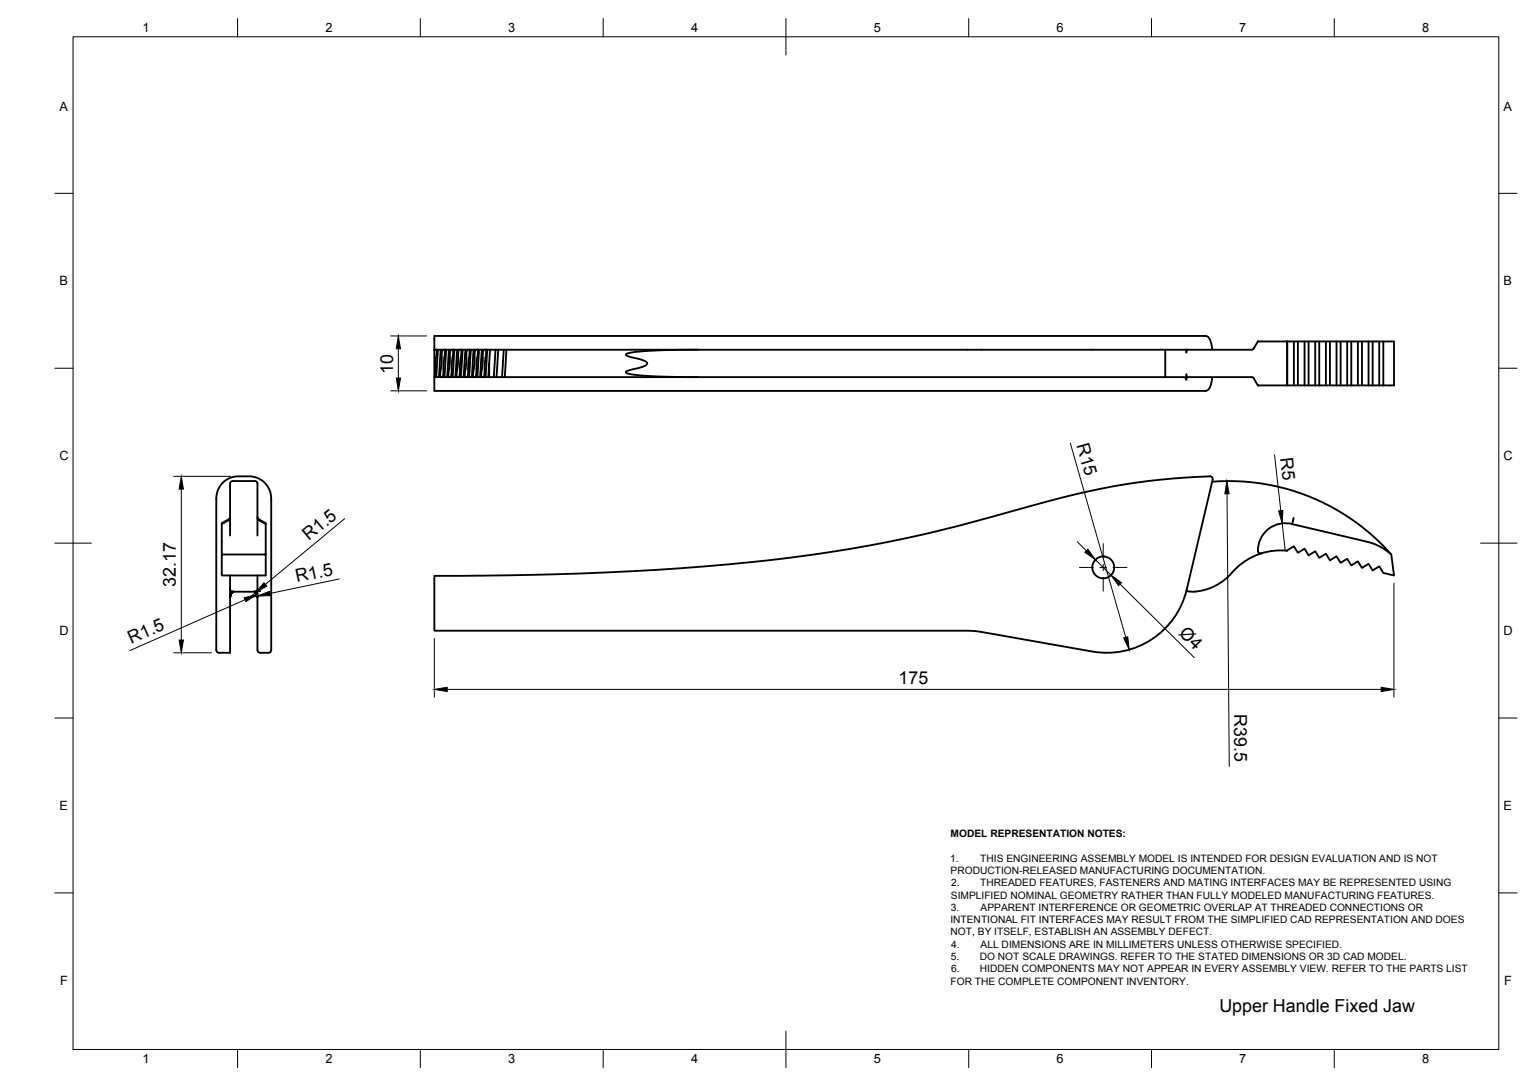
ISO-10303-21;
HEADER;
/* Generated by software containing ST-Developer
 * from STEP Tools, Inc. (www.steptools.com) 
 */

FILE_DESCRIPTION(
/* description */ ('STEP AP214'),
/* implementation_level */ '2;1');

FILE_NAME(
/* name */ 'Upper Handle Fixed Jaw.step',
/* time_stamp */ '2026-10-06T11:11:25-07:00',
/* author */ (''),
/* organization */ (''),
/* preprocessor_version */ 'ST-DEVELOPER v20.2',
/* originating_system */ 'Autodesk Translation Framework v15.15.0.0',
/* authorisation */ '');

FILE_SCHEMA (('AUTOMOTIVE_DESIGN { 1 0 10303 214 3 1 1 }'));
ENDSEC;

DATA;
#10=MECHANICAL_DESIGN_GEOMETRIC_PRESENTATION_REPRESENTATION('',(#701),#47717);
#59=(
BOUNDED_CURVE()
B_SPLINE_CURVE(2,(#17840,#17841,#17842,#17843,#17844),.UNSPECIFIED.,.F.,
 .F.)
B_SPLINE_CURVE_WITH_KNOTS((3,2,3),(0.0782086527637745,0.0875,0.0968862157575747),
 .UNSPECIFIED.)
CURVE()
GEOMETRIC_REPRESENTATION_ITEM()
RATIONAL_B_SPLINE_CURVE((0.970952227928523,0.943419064382284,1.,0.942841349486679,
0.971523247154132))
REPRESENTATION_ITEM('')
);
#60=(
BOUNDED_CURVE()
B_SPLINE_CURVE(2,(#17845,#17846,#17847,#17848,#17849),.UNSPECIFIED.,.F.,
 .F.)
B_SPLINE_CURVE_WITH_KNOTS((3,2,3),(0.803114463635883,0.8125,0.821791347236166),
 .UNSPECIFIED.)
CURVE()
GEOMETRIC_REPRESENTATION_ITEM()
RATIONAL_B_SPLINE_CURVE((0.971519095495255,0.942845486746487,1.,0.943419064382644,
0.970952227928172))
REPRESENTATION_ITEM('')
);
#61=(
BOUNDED_CURVE()
B_SPLINE_CURVE(2,(#17851,#17852,#17853,#17854,#17855),.UNSPECIFIED.,.F.,
 .F.)
B_SPLINE_CURVE_WITH_KNOTS((3,2,3),(0.178208652763774,0.1875,0.196882250682148),
 .UNSPECIFIED.)
CURVE()
GEOMETRIC_REPRESENTATION_ITEM()
RATIONAL_B_SPLINE_CURVE((0.970952227928523,0.943419064382284,1.,0.942865495358289,
0.971499029940397))
REPRESENTATION_ITEM('')
);
#62=(
BOUNDED_CURVE()
B_SPLINE_CURVE(2,(#17856,#17857,#17858,#17859,#17860),.UNSPECIFIED.,.F.,
 .F.)
B_SPLINE_CURVE_WITH_KNOTS((3,2,3),(0.703119206263016,0.7125,0.721791347236166),
 .UNSPECIFIED.)
CURVE()
GEOMETRIC_REPRESENTATION_ITEM()
RATIONAL_B_SPLINE_CURVE((0.971490139155267,0.942874367626047,1.,0.943419064382644,
0.970952227928173))
REPRESENTATION_ITEM('')
);
#63=(
BOUNDED_CURVE()
B_SPLINE_CURVE(2,(#17862,#17863,#17864,#17865,#17866),.UNSPECIFIED.,.F.,
 .F.)
B_SPLINE_CURVE_WITH_KNOTS((3,2,3),(0.278208652763774,0.2875,0.296875230169318),
 .UNSPECIFIED.)
CURVE()
GEOMETRIC_REPRESENTATION_ITEM()
RATIONAL_B_SPLINE_CURVE((0.970952227928523,0.943419064382284,1.,0.94290824773578,
0.971456226391036))
REPRESENTATION_ITEM('')
);
#64=(
BOUNDED_CURVE()
B_SPLINE_CURVE(2,(#17867,#17868,#17869,#17870,#17871),.UNSPECIFIED.,.F.,
 .F.)
B_SPLINE_CURVE_WITH_KNOTS((3,2,3),(0.603126927215252,0.6125,0.621791347236166),
 .UNSPECIFIED.)
CURVE()
GEOMETRIC_REPRESENTATION_ITEM()
RATIONAL_B_SPLINE_CURVE((0.971443092268521,0.942921385425537,1.,0.943419064382644,
0.970952227928173))
REPRESENTATION_ITEM('')
);
#65=(
BOUNDED_CURVE()
B_SPLINE_CURVE(2,(#17873,#17874,#17875,#17876,#17877),.UNSPECIFIED.,.F.,
 .F.)
B_SPLINE_CURVE_WITH_KNOTS((3,2,3),(0.378208652763774,0.3875,0.396865543999395),
 .UNSPECIFIED.)
CURVE()
GEOMETRIC_REPRESENTATION_ITEM()
RATIONAL_B_SPLINE_CURVE((0.970952227928524,0.943419064382284,1.,0.942967232998394,
0.971397328198516))
REPRESENTATION_ITEM('')
);
#66=(
BOUNDED_CURVE()
B_SPLINE_CURVE(2,(#17878,#17879,#17880,#17881,#17882),.UNSPECIFIED.,.F.,
 .F.)
B_SPLINE_CURVE_WITH_KNOTS((3,2,3),(0.50313718714112,0.5125,0.521791347236167),
 .UNSPECIFIED.)
CURVE()
GEOMETRIC_REPRESENTATION_ITEM()
RATIONAL_B_SPLINE_CURVE((0.971380754136894,0.94298386465382,1.,0.943419064382643,
0.970952227928174))
REPRESENTATION_ITEM('')
);
#67=(
BOUNDED_CURVE()
B_SPLINE_CURVE(2,(#17884,#17885,#17886,#17887,#17888),.UNSPECIFIED.,.F.,
 .F.)
B_SPLINE_CURVE_WITH_KNOTS((3,2,3),(0.478208652763774,0.4875,0.496853778396117),
 .UNSPECIFIED.)
CURVE()
GEOMETRIC_REPRESENTATION_ITEM()
RATIONAL_B_SPLINE_CURVE((0.970952227928524,0.943419064382283,1.,0.94303888125614,
0.971326031620276))
REPRESENTATION_ITEM('')
);
#68=(
BOUNDED_CURVE()
B_SPLINE_CURVE(2,(#17889,#17890,#17891,#17892,#17893),.UNSPECIFIED.,.F.,
 .F.)
B_SPLINE_CURVE_WITH_KNOTS((3,2,3),(0.403149353858237,0.4125,0.421791347236167),
 .UNSPECIFIED.)
CURVE()
GEOMETRIC_REPRESENTATION_ITEM()
RATIONAL_B_SPLINE_CURVE((0.971307096418175,0.943057955549397,1.,0.943419064382643,
0.970952227928173))
REPRESENTATION_ITEM('')
);
#69=(
BOUNDED_CURVE()
B_SPLINE_CURVE(2,(#17895,#17896,#17897,#17898,#17899),.UNSPECIFIED.,.F.,
 .F.)
B_SPLINE_CURVE_WITH_KNOTS((3,2,3),(0.578208652763774,0.5875,0.596840698287781),
 .UNSPECIFIED.)
CURVE()
GEOMETRIC_REPRESENTATION_ITEM()
RATIONAL_B_SPLINE_CURVE((0.970952227928523,0.943419064382284,1.,0.943118534373046,
0.971247086120199))
REPRESENTATION_ITEM('')
);
#70=(
BOUNDED_CURVE()
B_SPLINE_CURVE(2,(#17900,#17901,#17902,#17903,#17904),.UNSPECIFIED.,.F.,
 .F.)
B_SPLINE_CURVE_WITH_KNOTS((3,2,3),(0.303162621990297,0.3125,0.321791347236167),
 .UNSPECIFIED.)
CURVE()
GEOMETRIC_REPRESENTATION_ITEM()
RATIONAL_B_SPLINE_CURVE((0.971227099510026,0.943138753662606,1.,0.943419064382643,
0.970952227928174))
REPRESENTATION_ITEM('')
);
#71=(
BOUNDED_CURVE()
B_SPLINE_CURVE(2,(#17907,#17908,#17909,#17910,#17911),.UNSPECIFIED.,.F.,
 .F.)
B_SPLINE_CURVE_WITH_KNOTS((3,2,3),(0.678208652763775,0.6875,0.691555825853902),
 .UNSPECIFIED.)
CURVE()
GEOMETRIC_REPRESENTATION_ITEM()
RATIONAL_B_SPLINE_CURVE((0.970952227928523,0.943419064382284,1.,0.975301491195852,
0.966630638481416))
REPRESENTATION_ITEM('')
);
#72=(
BOUNDED_CURVE()
B_SPLINE_CURVE(2,(#19973,#19974,#19975,#19976,#19977),.UNSPECIFIED.,.F.,
 .F.)
B_SPLINE_CURVE_WITH_KNOTS((3,2,3),(0.745762259902575,0.75,0.751783130051315),
 .UNSPECIFIED.)
CURVE()
GEOMETRIC_REPRESENTATION_ITEM()
RATIONAL_B_SPLINE_CURVE((0.965885061990929,0.974193699415065,1.,0.989141384552057,
0.981380740867458))
REPRESENTATION_ITEM('')
);
#73=(
BOUNDED_CURVE()
B_SPLINE_CURVE(2,(#20440,#20441,#20442,#20443,#20444,#20445,#20446,#20447,
#20448,#20449,#20450,#20451,#20452,#20453,#20454),.UNSPECIFIED.,.F.,.F.)
B_SPLINE_CURVE_WITH_KNOTS((3,2,2,2,2,2,2,3),(0.673216868607369,0.675,0.6875,
0.7,0.7125,0.725,0.7375,0.745762259902575),.UNSPECIFIED.)
CURVE()
GEOMETRIC_REPRESENTATION_ITEM()
RATIONAL_B_SPLINE_CURVE((0.981380729191956,0.989141376383933,1.,0.923879532511287,
1.,0.923879532511287,1.,0.923879532511287,1.,0.923879532511287,1.,0.923879532511287,
1.,0.949685833096222,0.965885061990929))
REPRESENTATION_ITEM('')
);
#74=(
BOUNDED_CURVE()
B_SPLINE_CURVE(2,(#20777,#20778,#20779,#20780,#20781,#20782,#20783,#20784,
#20785),.UNSPECIFIED.,.F.,.F.)
B_SPLINE_CURVE_WITH_KNOTS((3,2,2,2,3),(0.673216868607369,0.675,0.6875,0.7,
0.712499999279178),.UNSPECIFIED.)
CURVE()
GEOMETRIC_REPRESENTATION_ITEM()
RATIONAL_B_SPLINE_CURVE((0.981380729191956,0.989141376383933,1.,0.923879532511287,
1.,0.923879532511287,1.,0.923879536900831,0.999999991220912))
REPRESENTATION_ITEM('')
);
#75=(
BOUNDED_CURVE()
B_SPLINE_CURVE(2,(#23686,#23687,#23688,#23689,#23690,#23691,#23692,#23693,
#23694,#23695,#23696,#23697,#23698,#23699,#23700,#23701,#23702),
 .UNSPECIFIED.,.F.,.F.)
B_SPLINE_CURVE_WITH_KNOTS((3,2,2,2,2,2,2,2,3),(0.0732168686073693,0.075,
0.0875,0.1,0.1125,0.125,0.1375,0.15,0.151783130051315),.UNSPECIFIED.)
CURVE()
GEOMETRIC_REPRESENTATION_ITEM()
RATIONAL_B_SPLINE_CURVE((0.981380729191956,0.989141376383932,1.,0.923879532511287,
1.,0.923879532511287,1.,0.923879532511287,1.,0.923879532511287,1.,0.923879532511287,
1.,0.923879532511287,1.,0.989141384552058,0.981380740867459))
REPRESENTATION_ITEM('')
);
#76=(
BOUNDED_CURVE()
B_SPLINE_CURVE(2,(#24025,#24026,#24027,#24028,#24029,#24030,#24031,#24032,
#24033,#24034,#24035,#24036,#24037,#24038,#24039),.UNSPECIFIED.,.F.,.F.)
B_SPLINE_CURVE_WITH_KNOTS((3,2,2,2,2,2,2,3),(0.0792377388003687,0.0875,
0.1,0.1125,0.125,0.1375,0.15,0.151783130051315),.UNSPECIFIED.)
CURVE()
GEOMETRIC_REPRESENTATION_ITEM()
RATIONAL_B_SPLINE_CURVE((0.965885067077025,0.949685825197617,1.,0.923879532511287,
1.,0.923879532511287,1.,0.923879532511287,1.,0.923879532511287,1.,0.923879532511287,
1.,0.989141384552057,0.981380740867458))
REPRESENTATION_ITEM('')
);
#77=(
BOUNDED_CURVE()
B_SPLINE_CURVE(2,(#25006,#25007,#25008,#25009,#25010,#25011,#25012,#25013,
#25014,#25015,#25016,#25017,#25018,#25019,#25020,#25021,#25022),
 .UNSPECIFIED.,.F.,.F.)
B_SPLINE_CURVE_WITH_KNOTS((3,2,2,2,2,2,2,2,3),(0.173216868607369,0.175,
0.1875,0.2,0.2125,0.225,0.2375,0.25,0.251783130051315),.UNSPECIFIED.)
CURVE()
GEOMETRIC_REPRESENTATION_ITEM()
RATIONAL_B_SPLINE_CURVE((0.981380729191956,0.989141376383932,1.,0.923879532511287,
1.,0.923879532511287,1.,0.923879532511287,1.,0.923879532511287,1.,0.923879532511287,
1.,0.923879532511287,1.,0.989141384552057,0.981380740867459))
REPRESENTATION_ITEM('')
);
#78=(
BOUNDED_CURVE()
B_SPLINE_CURVE(2,(#25345,#25346,#25347,#25348,#25349,#25350,#25351,#25352,
#25353,#25354,#25355,#25356,#25357,#25358,#25359,#25360,#25361),
 .UNSPECIFIED.,.F.,.F.)
B_SPLINE_CURVE_WITH_KNOTS((3,2,2,2,2,2,2,2,3),(0.173216868607369,0.175,
0.1875,0.2,0.2125,0.225,0.2375,0.25,0.251783130051315),.UNSPECIFIED.)
CURVE()
GEOMETRIC_REPRESENTATION_ITEM()
RATIONAL_B_SPLINE_CURVE((0.981380729191957,0.989141376383933,1.,0.923879532511287,
1.,0.923879532511287,1.,0.923879532511287,1.,0.923879532511287,1.,0.923879532511287,
1.,0.923879532511287,1.,0.989141384552057,0.981380740867459))
REPRESENTATION_ITEM('')
);
#79=(
BOUNDED_CURVE()
B_SPLINE_CURVE(2,(#26328,#26329,#26330,#26331,#26332,#26333,#26334,#26335,
#26336,#26337,#26338,#26339,#26340,#26341,#26342,#26343,#26344),
 .UNSPECIFIED.,.F.,.F.)
B_SPLINE_CURVE_WITH_KNOTS((3,2,2,2,2,2,2,2,3),(0.273216868607369,0.275,
0.2875,0.3,0.3125,0.325,0.3375,0.35,0.351783130051315),.UNSPECIFIED.)
CURVE()
GEOMETRIC_REPRESENTATION_ITEM()
RATIONAL_B_SPLINE_CURVE((0.981380729191956,0.989141376383932,1.,0.923879532511287,
1.,0.923879532511287,1.,0.923879532511287,1.,0.923879532511287,1.,0.923879532511287,
1.,0.923879532511287,1.,0.989141384552056,0.981380740867458))
REPRESENTATION_ITEM('')
);
#80=(
BOUNDED_CURVE()
B_SPLINE_CURVE(2,(#26667,#26668,#26669,#26670,#26671,#26672,#26673,#26674,
#26675,#26676,#26677,#26678,#26679,#26680,#26681,#26682,#26683),
 .UNSPECIFIED.,.F.,.F.)
B_SPLINE_CURVE_WITH_KNOTS((3,2,2,2,2,2,2,2,3),(0.273216868607369,0.275,
0.2875,0.3,0.3125,0.325,0.3375,0.35,0.351783130051315),.UNSPECIFIED.)
CURVE()
GEOMETRIC_REPRESENTATION_ITEM()
RATIONAL_B_SPLINE_CURVE((0.981380729191955,0.989141376383932,1.,0.923879532511287,
1.,0.923879532511287,1.,0.923879532511287,1.,0.923879532511287,1.,0.923879532511287,
1.,0.923879532511287,1.,0.989141384552056,0.981380740867458))
REPRESENTATION_ITEM('')
);
#81=(
BOUNDED_CURVE()
B_SPLINE_CURVE(2,(#27650,#27651,#27652,#27653,#27654,#27655,#27656,#27657,
#27658,#27659,#27660,#27661,#27662,#27663,#27664,#27665,#27666),
 .UNSPECIFIED.,.F.,.F.)
B_SPLINE_CURVE_WITH_KNOTS((3,2,2,2,2,2,2,2,3),(0.373216868607369,0.375,
0.3875,0.4,0.4125,0.425,0.4375,0.45,0.451783130051315),.UNSPECIFIED.)
CURVE()
GEOMETRIC_REPRESENTATION_ITEM()
RATIONAL_B_SPLINE_CURVE((0.981380729191956,0.989141376383932,1.,0.923879532511287,
1.,0.923879532511287,1.,0.923879532511287,1.,0.923879532511287,1.,0.923879532511287,
1.,0.923879532511287,1.,0.989141384552057,0.981380740867459))
REPRESENTATION_ITEM('')
);
#82=(
BOUNDED_CURVE()
B_SPLINE_CURVE(2,(#27989,#27990,#27991,#27992,#27993,#27994,#27995,#27996,
#27997,#27998,#27999,#28000,#28001,#28002,#28003,#28004,#28005),
 .UNSPECIFIED.,.F.,.F.)
B_SPLINE_CURVE_WITH_KNOTS((3,2,2,2,2,2,2,2,3),(0.373216868607369,0.375,
0.3875,0.4,0.4125,0.425,0.4375,0.45,0.451783130051315),.UNSPECIFIED.)
CURVE()
GEOMETRIC_REPRESENTATION_ITEM()
RATIONAL_B_SPLINE_CURVE((0.981380729191956,0.989141376383932,1.,0.923879532511287,
1.,0.923879532511287,1.,0.923879532511287,1.,0.923879532511287,1.,0.923879532511287,
1.,0.923879532511287,1.,0.989141384552056,0.981380740867458))
REPRESENTATION_ITEM('')
);
#83=(
BOUNDED_CURVE()
B_SPLINE_CURVE(2,(#28972,#28973,#28974,#28975,#28976,#28977,#28978,#28979,
#28980,#28981,#28982,#28983,#28984,#28985,#28986,#28987,#28988),
 .UNSPECIFIED.,.F.,.F.)
B_SPLINE_CURVE_WITH_KNOTS((3,2,2,2,2,2,2,2,3),(0.473216868607369,0.475,
0.4875,0.5,0.5125,0.525,0.5375,0.55,0.551783130051315),.UNSPECIFIED.)
CURVE()
GEOMETRIC_REPRESENTATION_ITEM()
RATIONAL_B_SPLINE_CURVE((0.981380729191957,0.989141376383933,1.,0.923879532511287,
1.,0.923879532511287,1.,0.923879532511287,1.,0.923879532511287,1.,0.923879532511287,
1.,0.923879532511287,1.,0.989141384552057,0.981380740867459))
REPRESENTATION_ITEM('')
);
#84=(
BOUNDED_CURVE()
B_SPLINE_CURVE(2,(#29311,#29312,#29313,#29314,#29315,#29316,#29317,#29318,
#29319,#29320,#29321,#29322,#29323,#29324,#29325,#29326,#29327),
 .UNSPECIFIED.,.F.,.F.)
B_SPLINE_CURVE_WITH_KNOTS((3,2,2,2,2,2,2,2,3),(0.473216868607369,0.475,
0.4875,0.5,0.5125,0.525,0.5375,0.55,0.551783130051315),.UNSPECIFIED.)
CURVE()
GEOMETRIC_REPRESENTATION_ITEM()
RATIONAL_B_SPLINE_CURVE((0.981380729191956,0.989141376383932,1.,0.923879532511287,
1.,0.923879532511287,1.,0.923879532511287,1.,0.923879532511287,1.,0.923879532511287,
1.,0.923879532511287,1.,0.989141384552057,0.981380740867459))
REPRESENTATION_ITEM('')
);
#85=(
BOUNDED_CURVE()
B_SPLINE_CURVE(2,(#30294,#30295,#30296,#30297,#30298,#30299,#30300,#30301,
#30302,#30303,#30304,#30305,#30306,#30307,#30308,#30309,#30310),
 .UNSPECIFIED.,.F.,.F.)
B_SPLINE_CURVE_WITH_KNOTS((3,2,2,2,2,2,2,2,3),(0.573216868607369,0.575,
0.5875,0.6,0.6125,0.625,0.6375,0.65,0.651783130051315),.UNSPECIFIED.)
CURVE()
GEOMETRIC_REPRESENTATION_ITEM()
RATIONAL_B_SPLINE_CURVE((0.981380729191957,0.989141376383933,1.,0.923879532511287,
1.,0.923879532511287,1.,0.923879532511287,1.,0.923879532511287,1.,0.923879532511287,
1.,0.923879532511287,1.,0.989141384552057,0.981380740867459))
REPRESENTATION_ITEM('')
);
#86=(
BOUNDED_CURVE()
B_SPLINE_CURVE(2,(#30633,#30634,#30635,#30636,#30637,#30638,#30639,#30640,
#30641,#30642,#30643,#30644,#30645,#30646,#30647,#30648,#30649),
 .UNSPECIFIED.,.F.,.F.)
B_SPLINE_CURVE_WITH_KNOTS((3,2,2,2,2,2,2,2,3),(0.573216868607369,0.575,
0.5875,0.6,0.6125,0.625,0.6375,0.65,0.651783130051315),.UNSPECIFIED.)
CURVE()
GEOMETRIC_REPRESENTATION_ITEM()
RATIONAL_B_SPLINE_CURVE((0.981380729191956,0.989141376383932,1.,0.923879532511287,
1.,0.923879532511287,1.,0.923879532511287,1.,0.923879532511287,1.,0.923879532511287,
1.,0.923879532511287,1.,0.989141384552057,0.981380740867458))
REPRESENTATION_ITEM('')
);
#87=(
BOUNDED_CURVE()
B_SPLINE_CURVE(2,(#31616,#31617,#31618,#31619,#31620),.UNSPECIFIED.,.F.,
 .F.)
B_SPLINE_CURVE_WITH_KNOTS((3,2,3),(0.0457622599025745,0.05,0.0517831300513152),
 .UNSPECIFIED.)
CURVE()
GEOMETRIC_REPRESENTATION_ITEM()
RATIONAL_B_SPLINE_CURVE((0.965885061990928,0.974193699415064,1.,0.989141384552057,
0.981380740867459))
REPRESENTATION_ITEM('')
);
#90=ELLIPSE('',#9174,3.18617762455186,3.07129968234925);
#91=ELLIPSE('',#9175,3.18617761845016,3.07129967669361);
#92=ELLIPSE('',#9176,3.18617759547738,3.07129965523857);
#93=ELLIPSE('',#9177,3.18617760733856,3.07129966633831);
#94=ELLIPSE('',#9178,3.18617760230713,3.07129966147478);
#95=ELLIPSE('',#9179,3.18617759636938,3.07129965601913);
#96=ELLIPSE('',#9180,3.18617760025713,3.07129965960386);
#97=ELLIPSE('',#9183,3.18617762276224,3.07129968128518);
#98=ELLIPSE('',#9184,3.18617761431604,3.07129967288479);
#99=ELLIPSE('',#9226,3.15483183585312,3.04022344912707);
#100=ELLIPSE('',#9227,3.15483182592464,3.04022343859094);
#101=ELLIPSE('',#9228,3.15483183621962,3.04022344977534);
#102=ELLIPSE('',#9229,3.53219078069322,3.28486872276377);
#103=ELLIPSE('',#9230,3.15483183030471,3.04022344355871);
#104=ELLIPSE('',#9231,3.15483182288516,3.04022343561688);
#105=ELLIPSE('',#9232,3.15483181972163,3.04022343210884);
#106=ELLIPSE('',#9233,3.1548318236625,3.04022343652648);
#107=ELLIPSE('',#9234,3.15483184138826,3.04022345552491);
#108=ELLIPSE('',#9235,3.15483182239517,3.04022343496998);
#109=ELLIPSE('',#9281,18.0380987508663,8.93352299302603);
#110=ELLIPSE('',#9284,18.0200745312909,8.92797473607996);
#124=B_SPLINE_SURFACE_WITH_KNOTS('',3,1,((#16524,#16525),(#16526,#16527),
(#16528,#16529),(#16530,#16531)),.UNSPECIFIED.,.F.,.F.,.F.,(4,4),(2,2),
(0.,1.),(0.,0.239999999999999),.UNSPECIFIED.);
#125=B_SPLINE_SURFACE_WITH_KNOTS('',3,1,((#16618,#16619),(#16620,#16621),
(#16622,#16623),(#16624,#16625)),.UNSPECIFIED.,.F.,.F.,.F.,(4,4),(2,2),
(0.,1.),(0.,0.239999999999999),.UNSPECIFIED.);
#126=B_SPLINE_SURFACE_WITH_KNOTS('',3,1,((#16715,#16716),(#16717,#16718),
(#16719,#16720),(#16721,#16722)),.UNSPECIFIED.,.F.,.F.,.F.,(4,4),(2,2),
(0.,1.),(0.,0.239999999999999),.UNSPECIFIED.);
#127=B_SPLINE_SURFACE_WITH_KNOTS('',3,1,((#16803,#16804),(#16805,#16806),
(#16807,#16808),(#16809,#16810)),.UNSPECIFIED.,.F.,.F.,.F.,(4,4),(2,2),
(0.,1.),(0.,0.239999999999999),.UNSPECIFIED.);
#128=B_SPLINE_SURFACE_WITH_KNOTS('',3,1,((#16894,#16895),(#16896,#16897),
(#16898,#16899),(#16900,#16901)),.UNSPECIFIED.,.F.,.F.,.F.,(4,4),(2,2),
(0.,1.),(0.,0.240000000000008),.UNSPECIFIED.);
#129=B_SPLINE_SURFACE_WITH_KNOTS('',3,1,((#16985,#16986),(#16987,#16988),
(#16989,#16990),(#16991,#16992)),.UNSPECIFIED.,.F.,.F.,.F.,(4,4),(2,2),
(0.,1.),(0.,0.239999999999999),.UNSPECIFIED.);
#130=B_SPLINE_SURFACE_WITH_KNOTS('',3,1,((#17924,#17925),(#17926,#17927),
(#17928,#17929),(#17930,#17931),(#17932,#17933),(#17934,#17935),(#17936,
#17937),(#17938,#17939),(#17940,#17941),(#17942,#17943),(#17944,#17945),
(#17946,#17947)),.UNSPECIFIED.,.F.,.F.,.F.,(4,2,2,2,2,4),(2,2),(0.,0.25,
0.5,0.625,0.75,1.),(0.,0.240000000000451),.UNSPECIFIED.);
#131=B_SPLINE_SURFACE_WITH_KNOTS('',3,1,((#18513,#18514),(#18515,#18516),
(#18517,#18518),(#18519,#18520)),.UNSPECIFIED.,.F.,.F.,.F.,(4,4),(2,2),
(0.,0.994738905317126),(0.,0.239999999999999),.UNSPECIFIED.);
#132=B_SPLINE_SURFACE_WITH_KNOTS('',3,1,((#19117,#19118),(#19119,#19120),
(#19121,#19122),(#19123,#19124)),.UNSPECIFIED.,.F.,.F.,.F.,(4,4),(2,2),
(0.,1.),(0.,1.),.UNSPECIFIED.);
#137=CONICAL_SURFACE('',#9144,5.,0.5235987755983);
#138=CONICAL_SURFACE('',#9146,5.,0.5235987755983);
#139=CONICAL_SURFACE('',#9256,10.,0.5235987755983);
#140=CONICAL_SURFACE('',#9258,10.,0.5235987755983);
#154=B_SPLINE_CURVE_WITH_KNOTS('',3,(#15707,#15708,#15709,#15710,#15711,
#15712,#15713,#15714,#15715,#15716,#15717,#15718),.UNSPECIFIED.,.F.,.F.,
(4,2,2,2,2,4),(-0.315861705869912,-0.304504739480588,-0.293147577229122,
-0.273654264741298,-0.254199478143445,-0.237067099008455),.UNSPECIFIED.);
#155=B_SPLINE_CURVE_WITH_KNOTS('',3,(#15728,#15729,#15730,#15731,#15732,
#15733,#15734,#15735,#15736,#15737),.UNSPECIFIED.,.F.,.F.,(4,2,2,2,4),(-0.075918388998373,
-0.0561637881777793,-0.0369076925566084,-0.0182249521533977,0.),
 .UNSPECIFIED.);
#156=B_SPLINE_CURVE_WITH_KNOTS('',3,(#15746,#15747,#15748,#15749,#15750,
#15751,#15752,#15753,#15754,#15755),.UNSPECIFIED.,.F.,.F.,(4,2,2,2,4),(-0.303763540065855,
-0.285538587912457,-0.266855847509246,-0.247599751888075,-0.227845151067482),
 .UNSPECIFIED.);
#157=B_SPLINE_CURVE_WITH_KNOTS('',3,(#15761,#15762,#15763,#15764,#15765,
#15766,#15767,#15768,#15769,#15770,#15771,#15772,#15773,#15774,#15775,#15776,
#15777,#15778,#15779,#15780,#15781,#15782,#15783,#15784,#15785,#15786,#15787,
#15788,#15789,#15790,#15791),.UNSPECIFIED.,.F.,.F.,(4,3,3,3,3,3,3,3,3,3,
4),(0.,6.43812390587994E-5,0.000133462758091886,0.000205560683863588,0.000281692284478665,
0.000294258926984526,0.00030196027953542,0.000382573776850771,0.000466187556446014,
0.000551165178275843,0.000603920559070841),.UNSPECIFIED.);
#158=B_SPLINE_CURVE_WITH_KNOTS('',3,(#15800,#15801,#15802,#15803,#15804,
#15805,#15806,#15807,#15808,#15809,#15810,#15811,#15812,#15813,#15814,#15815,
#15816,#15817,#15818,#15819,#15820,#15821,#15822,#15823,#15824,#15825,#15826,
#15827,#15828,#15829,#15830),.UNSPECIFIED.,.F.,.F.,(4,3,3,3,3,3,3,3,3,3,
4),(0.,8.03828939616283E-5,0.00016094681871393,0.000237477837746124,0.000302706001391965,
0.000310398285264662,0.000384832659816502,0.000456089108430895,0.000524203185115278,
0.000588293662717843,0.00060541200278393),.UNSPECIFIED.);
#159=B_SPLINE_CURVE_WITH_KNOTS('',3,(#15838,#15839,#15840,#15841),
 .UNSPECIFIED.,.F.,.F.,(4,4),(0.000288679049704741,0.00173207592567418),
 .UNSPECIFIED.);
#160=B_SPLINE_CURVE_WITH_KNOTS('',3,(#15842,#15843,#15844,#15845),
 .UNSPECIFIED.,.F.,.F.,(4,4),(0.,0.00146452330146534),.UNSPECIFIED.);
#161=B_SPLINE_CURVE_WITH_KNOTS('',3,(#15850,#15851,#15852,#15853),
 .UNSPECIFIED.,.F.,.F.,(4,4),(3.99819120664141E-10,0.0014645237012841),
 .UNSPECIFIED.);
#162=B_SPLINE_CURVE_WITH_KNOTS('',3,(#15854,#15855,#15856,#15857),
 .UNSPECIFIED.,.F.,.F.,(4,4),(0.,0.00144339687596949),.UNSPECIFIED.);
#163=B_SPLINE_CURVE_WITH_KNOTS('',3,(#15874,#15875,#15876,#15877,#15878,
#15879,#15880,#15881),.UNSPECIFIED.,.F.,.F.,(4,2,2,4),(0.,0.0195287994608885,
0.039060798714645,0.058407685727557),.UNSPECIFIED.);
#164=B_SPLINE_CURVE_WITH_KNOTS('',3,(#15893,#15894,#15895,#15896,#15897,
#15898,#15899,#15900,#15901,#15902),.UNSPECIFIED.,.F.,.F.,(4,2,2,2,4),(0.25677760841793,
0.273427822422786,0.292959602080408,0.30405126303756,0.315142780478787),
 .UNSPECIFIED.);
#165=B_SPLINE_CURVE_WITH_KNOTS('',3,(#15909,#15910,#15911,#15912,#15913,
#15914,#15915,#15916,#15917,#15918,#15919,#15920),.UNSPECIFIED.,.F.,.F.,
(4,2,2,2,2,4),(-0.675172633386201,-0.576849455741665,-0.476321267640776,
-0.315506903735809,-0.160746606147669,-9.99999996698087E-7),
 .UNSPECIFIED.);
#166=B_SPLINE_CURVE_WITH_KNOTS('',3,(#15924,#15925,#15926,#15927,#15928,
#15929,#15930,#15931,#15932,#15933,#15934,#15935),.UNSPECIFIED.,.F.,.F.,
(4,2,2,2,2,4),(-0.675693768666456,-0.514824382991667,-0.359943941875025,
-0.199004734580793,-0.0983990080529495,0.),.UNSPECIFIED.);
#167=B_SPLINE_CURVE_WITH_KNOTS('',3,(#15943,#15944,#15945,#15946,#15947,
#15948,#15949,#15950,#15951,#15952,#15953,#15954,#15955,#15956,#15957,#15958,
#15959,#15960,#15961,#15962,#15963,#15964,#15965,#15966,#15967,#15968,#15969,
#15970,#15971,#15972,#15973,#15974,#15975,#15976,#15977,#15978,#15979,#15980,
#15981,#15982,#15983,#15984,#15985,#15986,#15987,#15988,#15989,#15990,#15991,
#15992,#15993,#15994,#15995,#15996,#15997,#15998,#15999,#16000,#16001,#16002,
#16003,#16004,#16005,#16006,#16007,#16008,#16009,#16010,#16011,#16012,#16013,
#16014,#16015,#16016,#16017,#16018,#16019,#16020,#16021,#16022,#16023,#16024,
#16025,#16026,#16027,#16028,#16029,#16030,#16031,#16032,#16033,#16034,#16035,
#16036,#16037,#16038,#16039,#16040,#16041,#16042,#16043,#16044,#16045,#16046,
#16047,#16048,#16049,#16050,#16051,#16052,#16053,#16054,#16055,#16056,#16057,
#16058,#16059,#16060,#16061,#16062,#16063,#16064,#16065,#16066,#16067,#16068,
#16069,#16070,#16071,#16072,#16073,#16074,#16075,#16076,#16077,#16078,#16079,
#16080,#16081),.UNSPECIFIED.,.F.,.F.,(4,3,3,3,3,3,3,3,3,3,3,3,3,3,3,3,3,
3,3,3,3,3,3,3,3,3,3,3,3,3,3,3,3,3,3,3,3,3,3,3,3,3,3,3,3,3,4),(0.,0.000256348549033948,
0.000502816100424785,0.000732686647454628,0.000929586010325689,0.00106762170514576,
0.00119927302827119,0.00132084179949912,0.00139437901548853,0.00146772785131755,
0.00153687262127654,0.00160013903578677,0.00162677551806997,0.00169883608742252,
0.00174297376936069,0.0017904732714029,0.00184301110341694,0.00185917202065141,
0.00192000576784545,0.00198442832044501,0.00205463066127626,0.00209156852323289,
0.00219804885243176,0.00231204074056505,0.00232396502581438,0.00249108586559547,
0.00266994389318095,0.00278875803097735,0.00305416840235674,0.00333025398384524,
0.00362172008319921,0.00371834404130334,0.00415146712302494,0.00461037575263192,
0.00509524559958469,0.00557751606195529,0.00625060925148138,0.00695696807124114,
0.00743668808260725,0.00838353573023607,0.0093594221448559,0.0103800307872189,
0.0111550321239112,0.0124465160053231,0.013791250312021,0.0141155747496086,
0.0148733761652151),.UNSPECIFIED.);
#168=B_SPLINE_CURVE_WITH_KNOTS('',3,(#16083,#16084,#16085,#16086,#16087,
#16088,#16089,#16090,#16091,#16092,#16093,#16094,#16095,#16096,#16097,#16098,
#16099,#16100,#16101,#16102,#16103,#16104,#16105,#16106,#16107,#16108,#16109,
#16110,#16111,#16112,#16113,#16114,#16115,#16116,#16117,#16118,#16119,#16120,
#16121,#16122,#16123,#16124,#16125,#16126,#16127,#16128,#16129,#16130,#16131,
#16132,#16133,#16134,#16135,#16136,#16137,#16138,#16139,#16140,#16141,#16142,
#16143,#16144,#16145,#16146,#16147,#16148,#16149),.UNSPECIFIED.,.F.,.F.,
(4,3,3,3,3,3,3,3,3,3,3,3,3,3,3,3,3,3,3,3,3,3,4),(9.27910111233108E-7,0.0388272496183639,
0.0772841574679648,0.116619782957044,0.132707521806239,0.162001548301887,
0.193238852575001,0.208023910010697,0.229368195915971,0.235345838936746,
0.249459717687539,0.259976239169003,0.270396540144426,0.283622627082234,
0.304570284853286,0.307925338554378,0.339393568656544,0.367134413731198,
0.37086179875871,0.40826291529972,0.444819006483458,0.481815249493331,0.517800460191241),
 .UNSPECIFIED.);
#169=B_SPLINE_CURVE_WITH_KNOTS('',3,(#16151,#16152,#16153,#16154,#16155,
#16156,#16157,#16158,#16159,#16160,#16161,#16162,#16163,#16164,#16165,#16166,
#16167,#16168,#16169,#16170,#16171,#16172),.UNSPECIFIED.,.F.,.F.,(4,2,2,
2,2,2,2,2,2,2,4),(9.99999880946701E-7,0.740968356548999,1.10803447596115,
1.13297439899924,1.143721929787,1.15062153269268,1.15675184018037,1.16426475270422,
1.17757025555378,1.20996329596376,1.34291541565289),.UNSPECIFIED.);
#170=B_SPLINE_CURVE_WITH_KNOTS('',3,(#16180,#16181,#16182,#16183,#16184,
#16185,#16186,#16187,#16188,#16189,#16190,#16191,#16192,#16193,#16194,#16195,
#16196,#16197,#16198,#16199,#16200,#16201,#16202,#16203,#16204,#16205,#16206,
#16207,#16208,#16209),.UNSPECIFIED.,.F.,.F.,(4,2,2,2,2,2,2,2,2,2,2,2,2,
2,4),(-1.98444564130913,-1.89114422425201,-1.7958177380882,-1.6349790573507,
-1.48026754058274,-1.31955477667618,-1.16495234940928,-1.00932603631617,
-0.850222812514903,-0.69461661564959,-0.535710588189596,-0.380118368783108,
-0.221411746164279,-0.109438295410394,0.),.UNSPECIFIED.);
#171=B_SPLINE_CURVE_WITH_KNOTS('',3,(#16214,#16215,#16216,#16217,#16218,
#16219,#16220,#16221,#16222,#16223,#16224,#16225,#16226,#16227,#16228,#16229,
#16230,#16231,#16232,#16233,#16234,#16235,#16236,#16237,#16238,#16239,#16240,
#16241,#16242,#16243),.UNSPECIFIED.,.F.,.F.,(4,2,2,2,2,2,2,2,2,2,2,2,2,
2,4),(-1.984820426919,-1.88639492736602,-1.78576272266909,-1.6246808184501,
-1.46967790916084,-1.30845849556702,-1.15333170836285,-0.992039524704425,
-0.83081389910288,-0.675813195226356,-0.514724822116692,-0.359847895242116,
-0.198896919906624,-0.0983465039006042,-9.9999998770528E-7),
 .UNSPECIFIED.);
#172=B_SPLINE_CURVE_WITH_KNOTS('',3,(#16247,#16248,#16249,#16250,#16251,
#16252,#16253,#16254,#16255,#16256,#16257,#16258,#16259,#16260,#16261,#16262,
#16263,#16264,#16265,#16266,#16267,#16268,#16269,#16270,#16271,#16272,#16273,
#16274,#16275,#16276),.UNSPECIFIED.,.F.,.F.,(4,2,2,2,2,2,2,2,2,2,2,2,2,
2,4),(-1.98444666250816,-1.89114483728254,-1.79581794294083,-1.63497942337504,
-1.48026806163894,-1.31955545877792,-1.16495318643358,-1.00932702928904,
-0.850223964920479,-0.694617923983521,-0.535712055758561,-0.380119992266497,
-0.221413528682937,-0.109439684369395,-1.00000005098799E-6),
 .UNSPECIFIED.);
#173=B_SPLINE_CURVE_WITH_KNOTS('',3,(#16281,#16282,#16283,#16284,#16285,
#16286,#16287,#16288,#16289,#16290,#16291,#16292,#16293,#16294,#16295,#16296,
#16297,#16298,#16299,#16300,#16301,#16302,#16303,#16304,#16305,#16306,#16307,
#16308,#16309,#16310),.UNSPECIFIED.,.F.,.F.,(4,2,2,2,2,2,2,2,2,2,2,2,2,
2,4),(-1.98481940872555,-1.88639386031479,-1.78576160566468,-1.62467962148561,
-1.46967663525383,-1.30845714163163,-1.15333027742346,-0.99203801370059,
-0.830812308067643,-0.675811527249796,-0.514723074176976,-0.359846070422441,
-0.198895015191813,-0.0983450528749099,0.),.UNSPECIFIED.);
#174=B_SPLINE_CURVE_WITH_KNOTS('',3,(#16314,#16315,#16316,#16317,#16318,
#16319,#16320,#16321,#16322,#16323,#16324,#16325,#16326,#16327,#16328,#16329,
#16330,#16331),.UNSPECIFIED.,.F.,.F.,(4,2,2,2,2,2,2,2,4),(-0.99035866670182,
-0.901126137518957,-0.810017339813086,-0.64988238649248,-0.495708568742823,
-0.340066262368237,-0.18191477126192,-0.0901037457175406,-1.00000003533385E-6),
 .UNSPECIFIED.);
#175=B_SPLINE_CURVE_WITH_KNOTS('',3,(#16338,#16339,#16340,#16341,#16342,
#16343,#16344,#16345,#16346,#16347),.UNSPECIFIED.,.F.,.F.,(4,2,2,2,4),(-0.354263984936231,
-0.264994680361422,-0.177037652566582,-0.0891610114015905,-1.00000006514334E-6),
 .UNSPECIFIED.);
#176=B_SPLINE_CURVE_WITH_KNOTS('',3,(#16351,#16352,#16353,#16354,#16355,
#16356,#16357,#16358,#16359,#16360),.UNSPECIFIED.,.F.,.F.,(4,2,2,2,4),(-0.353824542748299,
-0.264774556195651,-0.177007347690013,-0.0891585628061826,-9.99999994089062E-7),
 .UNSPECIFIED.);
#177=B_SPLINE_CURVE_WITH_KNOTS('',3,(#16365,#16366,#16367,#16368,#16369,
#16370,#16371,#16372,#16373,#16374),.UNSPECIFIED.,.F.,.F.,(4,2,2,2,4),(-0.354518502107395,
-0.265189138567669,-0.177165433052852,-0.0892273778761162,-1.00000006419965E-6),
 .UNSPECIFIED.);
#178=B_SPLINE_CURVE_WITH_KNOTS('',3,(#16378,#16379,#16380,#16381,#16382,
#16383,#16384,#16385,#16386,#16387),.UNSPECIFIED.,.F.,.F.,(4,2,2,2,4),(-0.354079537268672,
-0.264963089010901,-0.177134329509822,-0.0892187800375224,-1.00000006381107E-6),
 .UNSPECIFIED.);
#179=B_SPLINE_CURVE_WITH_KNOTS('',3,(#16392,#16393,#16394,#16395,#16396,
#16397,#16398,#16399,#16400,#16401),.UNSPECIFIED.,.F.,.F.,(4,2,2,2,4),(-0.354757463555714,
-0.265371721316049,-0.17728540199176,-0.0892896807913005,-1.00000006364453E-6),
 .UNSPECIFIED.);
#180=B_SPLINE_CURVE_WITH_KNOTS('',3,(#16405,#16406,#16407,#16408,#16409,
#16410,#16411,#16412,#16413,#16414),.UNSPECIFIED.,.F.,.F.,(4,2,2,2,4),(-0.354314501807183,
-0.265136819335046,-0.177251338508511,-0.0892742578316736,-1.00000006514334E-6),
 .UNSPECIFIED.);
#181=B_SPLINE_CURVE_WITH_KNOTS('',3,(#16419,#16420,#16421,#16422,#16423,
#16424,#16425,#16426,#16427,#16428),.UNSPECIFIED.,.F.,.F.,(4,2,2,2,4),(-0.354964666048056,
-0.26553004556308,-0.177389425165517,-0.0893436976482566,-9.99999990924927E-7),
 .UNSPECIFIED.);
#182=B_SPLINE_CURVE_WITH_KNOTS('',3,(#16432,#16433,#16434,#16435,#16436,
#16437,#16438,#16439,#16440,#16441),.UNSPECIFIED.,.F.,.F.,(4,2,2,2,4),(-0.354513805707218,
-0.265284187720151,-0.177350590270964,-0.0893213087125481,-1.0000000654764E-6),
 .UNSPECIFIED.);
#183=B_SPLINE_CURVE_WITH_KNOTS('',3,(#16446,#16447,#16448,#16449,#16450,
#16451,#16452,#16453,#16454,#16455),.UNSPECIFIED.,.F.,.F.,(4,2,2,2,4),(-0.355127057597616,
-0.265654134459916,-0.17747095070662,-0.0893860287446967,-9.99999999196088E-7),
 .UNSPECIFIED.);
#184=B_SPLINE_CURVE_WITH_KNOTS('',3,(#16459,#16460,#16461,#16462,#16463,
#16464,#16465,#16466,#16467,#16468),.UNSPECIFIED.,.F.,.F.,(4,2,2,2,4),(-0.354665118474449,
-0.265396073885442,-0.177425943603115,-0.0893570257229319,-9.99999998974044E-7),
 .UNSPECIFIED.);
#185=B_SPLINE_CURVE_WITH_KNOTS('',3,(#16473,#16474,#16475,#16476,#16477,
#16478,#16479,#16480,#16481,#16482),.UNSPECIFIED.,.F.,.F.,(4,2,2,2,4),(-0.355235150205187,
-0.265736734067912,-0.177525216072434,-0.0894142037588925,-1.00000006714174E-6),
 .UNSPECIFIED.);
#186=B_SPLINE_CURVE_WITH_KNOTS('',3,(#16486,#16487,#16488,#16489,#16490,
#16491,#16492,#16493,#16494,#16495),.UNSPECIFIED.,.F.,.F.,(4,2,2,2,4),(-0.354759791686021,
-0.265466080089346,-0.177473090931424,-0.0893793712074604,-9.99999999695689E-7),
 .UNSPECIFIED.);
#187=B_SPLINE_CURVE_WITH_KNOTS('',3,(#16500,#16501,#16502,#16503,#16504,
#16505,#16506,#16507,#16508,#16509),.UNSPECIFIED.,.F.,.F.,(4,2,2,2,4),(-0.355283282513423,
-0.26577351527105,-0.177549379663897,-0.0894267492827573,-1.00000006569845E-6),
 .UNSPECIFIED.);
#188=B_SPLINE_CURVE_WITH_KNOTS('',3,(#16513,#16514,#16515,#16516,#16517,
#16518,#16519,#16520,#16521,#16522),.UNSPECIFIED.,.F.,.F.,(4,2,2,2,4),(-0.354793080478592,
-0.265490695774362,-0.177489668834524,-0.0893872279312292,-9.99999999584666E-7),
 .UNSPECIFIED.);
#189=B_SPLINE_CURVE_WITH_KNOTS('',3,(#16534,#16535,#16536,#16537,#16538,
#16539,#16540,#16541,#16542,#16543,#16544,#16545,#16546,#16547,#16548,#16549,
#16550,#16551,#16552,#16553,#16554,#16555,#16556,#16557,#16558,#16559,#16560,
#16561,#16562,#16563,#16564,#16565,#16566,#16567,#16568,#16569,#16570),
 .UNSPECIFIED.,.F.,.F.,(4,3,3,3,3,3,3,3,3,3,3,3,4),(-0.195598306843679,
-0.123264481538882,-0.110045864193155,-0.103002447810529,-0.10157695259272,
-0.100794703875248,-0.100424012566965,-0.100190257704989,-0.0993931570989621,
-0.0980296806446515,-0.0926181161151234,-0.0743843579378517,-1.00000019162542E-6),
 .UNSPECIFIED.);
#190=B_SPLINE_CURVE_WITH_KNOTS('',3,(#16572,#16573,#16574,#16575),
 .UNSPECIFIED.,.F.,.F.,(4,4),(0.141911553477537,0.142385482367034),
 .UNSPECIFIED.);
#191=B_SPLINE_CURVE_WITH_KNOTS('',3,(#16577,#16578,#16579,#16580,#16581,
#16582,#16583,#16584,#16585,#16586,#16587,#16588,#16589,#16590,#16591,#16592,
#16593,#16594,#16595,#16596,#16597,#16598,#16599,#16600,#16601,#16602,#16603,
#16604,#16605,#16606,#16607,#16608,#16609,#16610,#16611,#16612,#16613),
 .UNSPECIFIED.,.F.,.F.,(4,3,3,3,3,3,3,3,3,3,3,3,4),(-0.194458103761094,
-0.134684129317144,-0.113068646531483,-0.103143192107291,-0.101588268397981,
-0.100784238137842,-0.100418705769013,-0.100119304646258,-0.0993246176591243,
-0.0979697747936403,-0.0926478893950155,-0.074330571228443,0.),
 .UNSPECIFIED.);
#192=B_SPLINE_CURVE_WITH_KNOTS('',3,(#16614,#16615,#16616,#16617),
 .UNSPECIFIED.,.F.,.F.,(4,4),(0.00134009499830981,0.00181261238932178),
 .UNSPECIFIED.);
#193=B_SPLINE_CURVE_WITH_KNOTS('',3,(#16628,#16629,#16630,#16631,#16632,
#16633,#16634,#16635,#16636,#16637,#16638,#16639,#16640,#16641,#16642,#16643,
#16644,#16645,#16646,#16647,#16648,#16649,#16650,#16651,#16652,#16653,#16654,
#16655,#16656,#16657,#16658,#16659,#16660,#16661,#16662,#16663,#16664,#16665,
#16666,#16667),.UNSPECIFIED.,.F.,.F.,(4,3,3,3,3,3,3,3,3,3,3,3,3,4),(-0.194494028891387,
-0.162125908018411,-0.119536045329343,-0.108846565940067,-0.102885128703993,
-0.101541265474887,-0.100781691030153,-0.100417518665575,-0.10012302828061,
-0.0992855890259592,-0.0977398411588879,-0.0897084819313687,-0.0744225582376583,
-1.00000019873092E-6),.UNSPECIFIED.);
#194=B_SPLINE_CURVE_WITH_KNOTS('',3,(#16669,#16670,#16671,#16672),
 .UNSPECIFIED.,.F.,.F.,(4,4),(0.140405475149255,0.140881603915338),
 .UNSPECIFIED.);
#195=B_SPLINE_CURVE_WITH_KNOTS('',3,(#16674,#16675,#16676,#16677,#16678,
#16679,#16680,#16681,#16682,#16683,#16684,#16685,#16686,#16687,#16688,#16689,
#16690,#16691,#16692,#16693,#16694,#16695,#16696,#16697,#16698,#16699,#16700,
#16701,#16702,#16703,#16704,#16705,#16706,#16707,#16708,#16709,#16710),
 .UNSPECIFIED.,.F.,.F.,(4,3,3,3,3,3,3,3,3,3,3,3,4),(-0.194436193946118,
-0.144932886173553,-0.115563305609625,-0.103254995613247,-0.101617470978299,
-0.100796695496138,-0.100431864202833,-0.10013062822708,-0.099348493432612,
-0.098048610059559,-0.0933182996091218,-0.0753172897329091,0.),
 .UNSPECIFIED.);
#196=B_SPLINE_CURVE_WITH_KNOTS('',3,(#16711,#16712,#16713,#16714),
 .UNSPECIFIED.,.F.,.F.,(4,4),(0.002838891359255,0.0033137097483393),
 .UNSPECIFIED.);
#197=B_SPLINE_CURVE_WITH_KNOTS('',3,(#16725,#16726,#16727,#16728,#16729,
#16730,#16731,#16732,#16733,#16734,#16735,#16736,#16737,#16738,#16739,#16740,
#16741,#16742,#16743,#16744,#16745,#16746,#16747,#16748,#16749,#16750,#16751,
#16752,#16753,#16754,#16755,#16756,#16757,#16758),.UNSPECIFIED.,.F.,.F.,
(4,3,3,3,3,3,3,3,3,3,3,4),(-0.19435323528279,-0.124535619715197,-0.106070197067798,
-0.102599335626109,-0.101487874003443,-0.100780098417182,-0.100427674373929,
-0.10010644945315,-0.0991724103632078,-0.0971568831920127,-0.0759588650073846,
-1.00000018861696E-6),.UNSPECIFIED.);
#198=B_SPLINE_CURVE_WITH_KNOTS('',3,(#16760,#16761,#16762,#16763),
 .UNSPECIFIED.,.F.,.F.,(4,4),(0.134372093107689,0.134872686417409),
 .UNSPECIFIED.);
#199=B_SPLINE_CURVE_WITH_KNOTS('',3,(#16765,#16766,#16767,#16768,#16769,
#16770,#16771,#16772,#16773,#16774,#16775,#16776,#16777,#16778,#16779,#16780,
#16781,#16782,#16783,#16784,#16785,#16786,#16787,#16788,#16789,#16790,#16791,
#16792,#16793,#16794,#16795,#16796,#16797,#16798),.UNSPECIFIED.,.F.,.F.,
(4,3,3,3,3,3,3,3,3,3,3,4),(-0.194392555335661,-0.123344459486231,-0.103739879120015,
-0.101678198852006,-0.100778062576977,-0.100422358916701,-0.10010239570925,
-0.0993609150724121,-0.0982389457672826,-0.0950358831823619,-0.075424087699,
0.),.UNSPECIFIED.);
#200=B_SPLINE_CURVE_WITH_KNOTS('',3,(#16799,#16800,#16801,#16802),
 .UNSPECIFIED.,.F.,.F.,(4,4),(0.00882605152059419,0.00932569413867771),
 .UNSPECIFIED.);
#201=B_SPLINE_CURVE_WITH_KNOTS('',3,(#16813,#16814,#16815,#16816,#16817,
#16818,#16819,#16820,#16821,#16822,#16823,#16824,#16825,#16826,#16827,#16828,
#16829,#16830,#16831,#16832,#16833,#16834,#16835,#16836,#16837,#16838,#16839,
#16840,#16841,#16842,#16843,#16844,#16845,#16846,#16847,#16848,#16849),
 .UNSPECIFIED.,.F.,.F.,(4,3,3,3,3,3,3,3,3,3,3,3,4),(-0.194157876185446,
-0.124533044815514,-0.106352198581866,-0.102421387170606,-0.101257165736826,
-0.100537645142505,-0.100181415933288,-0.0998675692180962,-0.0989614751107034,
-0.0970886950782979,-0.0795114673901098,-0.0324255403862385,-1.00000007903258E-6),
 .UNSPECIFIED.);
#202=B_SPLINE_CURVE_WITH_KNOTS('',3,(#16851,#16852,#16853,#16854),
 .UNSPECIFIED.,.F.,.F.,(4,4),(0.13588184021166,0.136373897134007),
 .UNSPECIFIED.);
#203=B_SPLINE_CURVE_WITH_KNOTS('',3,(#16856,#16857,#16858,#16859,#16860,
#16861,#16862,#16863,#16864,#16865,#16866,#16867,#16868,#16869,#16870,#16871,
#16872,#16873,#16874,#16875,#16876,#16877,#16878,#16879,#16880,#16881,#16882,
#16883,#16884,#16885,#16886,#16887,#16888,#16889),.UNSPECIFIED.,.F.,.F.,
(4,3,3,3,3,3,3,3,3,3,3,4),(-0.194441151898413,-0.123303248261605,-0.103612149587876,
-0.101673331691855,-0.100795113504573,-0.100436213890763,-0.100122644799755,
-0.0993723218297423,-0.0982113052533252,-0.0947158338413571,-0.076129474606578,
0.),.UNSPECIFIED.);
#204=B_SPLINE_CURVE_WITH_KNOTS('',3,(#16890,#16891,#16892,#16893),
 .UNSPECIFIED.,.F.,.F.,(4,4),(0.00733049598192872,0.0078215204041217),
 .UNSPECIFIED.);
#205=B_SPLINE_CURVE_WITH_KNOTS('',3,(#16904,#16905,#16906,#16907,#16908,
#16909,#16910,#16911,#16912,#16913,#16914,#16915,#16916,#16917,#16918,#16919,
#16920,#16921,#16922,#16923,#16924,#16925,#16926,#16927,#16928,#16929,#16930,
#16931,#16932,#16933,#16934,#16935,#16936,#16937,#16938,#16939,#16940),
 .UNSPECIFIED.,.F.,.F.,(4,3,3,3,3,3,3,3,3,3,3,3,4),(-0.195323898017394,
-0.124294804269522,-0.107255118396146,-0.102731117250133,-0.101499027233354,
-0.100759964465065,-0.100395632571243,-0.100153343276803,-0.0993052369896065,
-0.0977122022557945,-0.0888118939699463,-0.0729373309057275,-1.00000018948831E-6),
 .UNSPECIFIED.);
#206=B_SPLINE_CURVE_WITH_KNOTS('',3,(#16942,#16943,#16944,#16945),
 .UNSPECIFIED.,.F.,.F.,(4,4),(0.137390638838294,0.137875797145181),
 .UNSPECIFIED.);
#207=B_SPLINE_CURVE_WITH_KNOTS('',3,(#16947,#16948,#16949,#16950,#16951,
#16952,#16953,#16954,#16955,#16956,#16957,#16958,#16959,#16960,#16961,#16962,
#16963,#16964,#16965,#16966,#16967,#16968,#16969,#16970,#16971,#16972,#16973,
#16974,#16975,#16976,#16977,#16978,#16979,#16980),.UNSPECIFIED.,.F.,.F.,
(4,3,3,3,3,3,3,3,3,3,3,4),(-0.194460770152194,-0.123138826518747,-0.103467518298517,
-0.101639305168327,-0.100781542294932,-0.100420043418356,-0.100111728380133,
-0.0993517235744529,-0.0981483078455959,-0.0943102495859858,-0.0747206712961253,
0.),.UNSPECIFIED.);
#208=B_SPLINE_CURVE_WITH_KNOTS('',3,(#16981,#16982,#16983,#16984),
 .UNSPECIFIED.,.F.,.F.,(4,4),(0.00583410702683465,0.00631814513922487),
 .UNSPECIFIED.);
#209=B_SPLINE_CURVE_WITH_KNOTS('',3,(#16995,#16996,#16997,#16998,#16999,
#17000,#17001,#17002,#17003,#17004,#17005,#17006,#17007,#17008,#17009,#17010,
#17011,#17012,#17013,#17014,#17015,#17016,#17017,#17018,#17019,#17020,#17021,
#17022,#17023,#17024,#17025,#17026,#17027,#17028,#17029,#17030,#17031),
 .UNSPECIFIED.,.F.,.F.,(4,3,3,3,3,3,3,3,3,3,3,3,4),(-0.194354595634486,
-0.124820448572211,-0.107845859548302,-0.102700952796982,-0.101421142037528,
-0.100675980132718,-0.100314095496492,-0.100010428444396,-0.0991509263640827,
-0.0975029450999708,-0.0874063402276625,-0.0661239178086379,-1.00000017532684E-6),
 .UNSPECIFIED.);
#210=B_SPLINE_CURVE_WITH_KNOTS('',3,(#17033,#17034,#17035,#17036),
 .UNSPECIFIED.,.F.,.F.,(4,4),(0.138898510273107,0.139378370938015),
 .UNSPECIFIED.);
#211=B_SPLINE_CURVE_WITH_KNOTS('',3,(#17038,#17039,#17040,#17041,#17042,
#17043,#17044,#17045,#17046,#17047,#17048,#17049,#17050,#17051,#17052,#17053,
#17054,#17055,#17056,#17057,#17058,#17059,#17060,#17061,#17062,#17063,#17064,
#17065,#17066,#17067,#17068,#17069,#17070,#17071,#17072,#17073,#17074),
 .UNSPECIFIED.,.F.,.F.,(4,3,3,3,3,3,3,3,3,3,3,3,4),(-0.19441619914366,-0.161480406225361,
-0.119240121158241,-0.103349474438416,-0.101621236163409,-0.100782583552426,
-0.100419101429683,-0.100114896575942,-0.099344306124858,-0.0980947432494325,
-0.093850925665231,-0.0744872008833497,0.),.UNSPECIFIED.);
#212=B_SPLINE_CURVE_WITH_KNOTS('',3,(#17075,#17076,#17077,#17078),
 .UNSPECIFIED.,.F.,.F.,(4,4),(0.00433690036911171,0.00481554798135458),
 .UNSPECIFIED.);
#213=B_SPLINE_CURVE_WITH_KNOTS('',3,(#17086,#17087,#17088,#17089,#17090,
#17091),.UNSPECIFIED.,.F.,.F.,(4,2,4),(-0.14333107944773,-0.0736159262229404,
0.),.UNSPECIFIED.);
#214=B_SPLINE_CURVE_WITH_KNOTS('',3,(#17095,#17096,#17097,#17098,#17099,
#17100),.UNSPECIFIED.,.F.,.F.,(4,2,4),(-0.147015175052716,-0.0741905379943431,
-9.99999944489849E-7),.UNSPECIFIED.);
#215=B_SPLINE_CURVE_WITH_KNOTS('',3,(#17104,#17105,#17106,#17107,#17108,
#17109),.UNSPECIFIED.,.F.,.F.,(4,2,4),(-0.143331079447973,-0.0736164030416013,
0.),.UNSPECIFIED.);
#216=B_SPLINE_CURVE_WITH_KNOTS('',3,(#17113,#17114,#17115,#17116,#17117,
#17118),.UNSPECIFIED.,.F.,.F.,(4,2,4),(-0.147015175052249,-0.0741900426363321,
-9.99999949590951E-7),.UNSPECIFIED.);
#217=B_SPLINE_CURVE_WITH_KNOTS('',3,(#17122,#17123,#17124,#17125,#17126,
#17127),.UNSPECIFIED.,.F.,.F.,(4,2,4),(-0.143331079446318,-0.07361640304082,
0.),.UNSPECIFIED.);
#218=B_SPLINE_CURVE_WITH_KNOTS('',3,(#17131,#17132,#17133,#17134,#17135,
#17136),.UNSPECIFIED.,.F.,.F.,(4,2,4),(-0.147015175052338,-0.0741905379942694,
-9.99999947848274E-7),.UNSPECIFIED.);
#219=B_SPLINE_CURVE_WITH_KNOTS('',3,(#17140,#17141,#17142,#17143,#17144,
#17145),.UNSPECIFIED.,.F.,.F.,(4,2,4),(-0.143331079445893,-0.0736164030406679,
0.),.UNSPECIFIED.);
#220=B_SPLINE_CURVE_WITH_KNOTS('',3,(#17149,#17150,#17151,#17152,#17153,
#17154),.UNSPECIFIED.,.F.,.F.,(4,2,4),(-0.147015175052675,-0.074190537994313,
-9.99999944878427E-7),.UNSPECIFIED.);
#221=B_SPLINE_CURVE_WITH_KNOTS('',3,(#17158,#17159,#17160,#17161,#17162,
#17163),.UNSPECIFIED.,.F.,.F.,(4,2,4),(-0.143331079449217,-0.0736164030425967,
0.),.UNSPECIFIED.);
#222=B_SPLINE_CURVE_WITH_KNOTS('',3,(#17167,#17168,#17169,#17170,#17171,
#17172),.UNSPECIFIED.,.F.,.F.,(4,2,4),(-0.147015175052563,-0.0741905379943041,
-9.99999946987851E-7),.UNSPECIFIED.);
#223=B_SPLINE_CURVE_WITH_KNOTS('',3,(#17176,#17177,#17178,#17179,#17180,
#17181),.UNSPECIFIED.,.F.,.F.,(4,2,4),(-0.143331079448333,-0.0736159262229434,
0.),.UNSPECIFIED.);
#224=B_SPLINE_CURVE_WITH_KNOTS('',3,(#17185,#17186,#17187,#17188,#17189,
#17190),.UNSPECIFIED.,.F.,.F.,(4,2,4),(-0.147015175052789,-0.0741900426364876,
-9.99999946378767E-7),.UNSPECIFIED.);
#225=B_SPLINE_CURVE_WITH_KNOTS('',3,(#17194,#17195,#17196,#17197,#17198,
#17199),.UNSPECIFIED.,.F.,.F.,(4,2,4),(-0.143331079447819,-0.0736164030417104,
0.),.UNSPECIFIED.);
#226=B_SPLINE_CURVE_WITH_KNOTS('',3,(#17201,#17202,#17203,#17204,#17205,
#17206),.UNSPECIFIED.,.F.,.F.,(4,2,4),(-0.0412408216537853,-0.0206214941513466,
-1.00000001180406E-6),.UNSPECIFIED.);
#227=B_SPLINE_CURVE_WITH_KNOTS('',3,(#17218,#17219,#17220,#17221,#17222,
#17223,#17224,#17225,#17226,#17227,#17228,#17229,#17230,#17231,#17232,#17233,
#17234,#17235,#17236,#17237,#17238,#17239,#17240,#17241,#17242,#17243,#17244,
#17245,#17246,#17247,#17248,#17249,#17250,#17251,#17252,#17253,#17254,#17255,
#17256,#17257,#17258,#17259,#17260,#17261,#17262,#17263,#17264,#17265,#17266,
#17267,#17268,#17269,#17270,#17271,#17272,#17273,#17274,#17275,#17276,#17277,
#17278,#17279,#17280,#17281,#17282,#17283,#17284,#17285,#17286,#17287),
 .UNSPECIFIED.,.F.,.F.,(4,3,3,3,3,3,3,3,3,3,3,3,3,3,3,3,3,3,3,3,3,3,3,4),
(0.0481874539974375,0.0604511794446379,0.070528500825075,0.0734860385296239,
0.0816990242388937,0.0865209011059417,0.0928695476527125,0.0930383208706332,
0.0984548093596218,0.0995557664417368,0.104040071066531,0.106073179694452,
0.112590606795416,0.11521059448035,0.119108035899913,0.120795856187259,
0.124177092586103,0.125625561625231,0.126381117894169,0.128882895010381,
0.131966379601078,0.132137852941708,0.136965611308967,0.137551641307987),
 .UNSPECIFIED.);
#228=B_SPLINE_CURVE_WITH_KNOTS('',3,(#17303,#17304,#17305,#17306,#17307,
#17308,#17309,#17310,#17311,#17312,#17313,#17314,#17315,#17316,#17317,#17318),
 .UNSPECIFIED.,.F.,.F.,(4,2,2,2,2,2,2,4),(1.00000015767795E-6,0.0566419671564676,
0.112784425720308,0.12743749066151,0.133720994177815,0.139633617857089,
0.183920433299157,0.225783248401836),.UNSPECIFIED.);
#229=B_SPLINE_CURVE_WITH_KNOTS('',3,(#17319,#17320,#17321,#17322,#17323,
#17324,#17325,#17326,#17327,#17328,#17329,#17330,#17331,#17332,#17333,#17334,
#17335,#17336),.UNSPECIFIED.,.F.,.F.,(4,2,2,2,2,2,2,2,4),(0.,0.0401671331759944,
0.0854041510983084,0.088451528257622,0.0916096770996849,0.0983906908764339,
0.112644364639411,0.170245279340444,0.225566054832859),.UNSPECIFIED.);
#230=B_SPLINE_CURVE_WITH_KNOTS('',3,(#17349,#17350,#17351,#17352,#17353,
#17354,#17355,#17356,#17357,#17358,#17359,#17360,#17361,#17362,#17363,#17364,
#17365,#17366),.UNSPECIFIED.,.F.,.F.,(4,2,2,2,2,2,2,2,4),(1.00000015378182E-6,
0.0558033364890031,0.111947159620381,0.126596830926891,0.132828265004497,
0.135756028209409,0.138596448354699,0.182551382377112,0.224108739412938),
 .UNSPECIFIED.);
#231=B_SPLINE_CURVE_WITH_KNOTS('',3,(#17367,#17368,#17369,#17370,#17371,
#17372,#17373,#17374,#17375,#17376,#17377,#17378,#17379,#17380,#17381,#17382),
 .UNSPECIFIED.,.F.,.F.,(4,2,2,2,2,2,2,4),(0.,0.0397861978551001,0.084544977734077,
0.0907978235304521,0.0975212072539927,0.111776839943134,0.169529074612989,
0.223835312885583),.UNSPECIFIED.);
#232=B_SPLINE_CURVE_WITH_KNOTS('',3,(#17395,#17396,#17397,#17398,#17399,
#17400,#17401,#17402,#17403,#17404,#17405,#17406,#17407,#17408,#17409,#17410),
 .UNSPECIFIED.,.F.,.F.,(4,2,2,2,2,2,2,4),(1.00000015458341E-6,0.0551170619821043,
0.111258895694281,0.125906053027141,0.132093950533861,0.137915824051536,
0.181508333049727,0.22273106176126),.UNSPECIFIED.);
#233=B_SPLINE_CURVE_WITH_KNOTS('',3,(#17411,#17412,#17413,#17414,#17415,
#17416,#17417,#17418,#17419,#17420,#17421,#17422,#17423,#17424,#17425,#17426),
 .UNSPECIFIED.,.F.,.F.,(4,2,2,2,2,2,2,4),(0.,0.0409142927088161,0.0870329656864442,
0.090140402195948,0.0968150072471416,0.11107376451763,0.168959944123858,
0.222415697934881),.UNSPECIFIED.);
#234=B_SPLINE_CURVE_WITH_KNOTS('',3,(#17439,#17440,#17441,#17442,#17443,
#17444,#17445,#17446,#17447,#17448,#17449,#17450,#17451,#17452,#17453,#17454),
 .UNSPECIFIED.,.F.,.F.,(4,2,2,2,2,2,2,4),(1.00000015245565E-6,0.0545871826959916,
0.110723454503288,0.125369052976213,0.131522194169781,0.137311275351113,
0.18065802848448,0.221659371342439),.UNSPECIFIED.);
#235=B_SPLINE_CURVE_WITH_KNOTS('',3,(#17455,#17456,#17457,#17458,#17459,
#17460,#17461,#17462,#17463,#17464,#17465,#17466,#17467,#17468,#17469,#17470),
 .UNSPECIFIED.,.F.,.F.,(4,2,2,2,2,2,2,4),(0.,0.0406903828664926,0.0865151821863462,
0.0896037483126215,0.0962386252435175,0.110500789147319,0.168500019068009,
0.221271398664186),.UNSPECIFIED.);
#236=B_SPLINE_CURVE_WITH_KNOTS('',3,(#17483,#17484,#17485,#17486,#17487,
#17488,#17489,#17490,#17491,#17492,#17493,#17494,#17495,#17496,#17497,#17498),
 .UNSPECIFIED.,.F.,.F.,(4,2,2,2,2,2,2,4),(1.00000015268294E-6,0.0542163947487819,
0.110343410733279,0.124212476892867,0.130385053869933,0.136193595788229,
0.179714725892929,0.220902014754228),.UNSPECIFIED.);
#237=B_SPLINE_CURVE_WITH_KNOTS('',3,(#17499,#17500,#17501,#17502,#17503,
#17504,#17505,#17506,#17507,#17508,#17509,#17510,#17511,#17512,#17513,#17514),
 .UNSPECIFIED.,.F.,.F.,(4,2,2,2,2,2,2,4),(0.,0.039140602667914,0.0830524217192137,
0.0891911669334346,0.095795784554504,0.110061497078605,0.168152629570437,
0.220408984280307),.UNSPECIFIED.);
#238=B_SPLINE_CURVE_WITH_KNOTS('',3,(#17527,#17528,#17529,#17530,#17531,
#17532,#17533,#17534,#17535,#17536,#17537,#17538,#17539,#17540,#17541,#17542),
 .UNSPECIFIED.,.F.,.F.,(4,2,2,2,2,2,2,4),(9.9999962800122E-7,0.0540058272398856,
0.110119887130061,0.123968789679388,0.130125700954026,0.135919865126588,
0.179343774956579,0.220454906422694),.UNSPECIFIED.);
#239=B_SPLINE_CURVE_WITH_KNOTS('',3,(#17543,#17544,#17545,#17546,#17547,
#17548,#17549,#17550,#17551,#17552,#17553,#17554,#17555,#17556),
 .UNSPECIFIED.,.F.,.F.,(4,2,2,2,2,2,4),(0.,0.0388549911094784,0.0823949291517112,
0.0955223331063072,0.109792272136123,0.167956881450626,0.21987139248006),
 .UNSPECIFIED.);
#240=B_SPLINE_CURVE_WITH_KNOTS('',3,(#17570,#17571,#17572,#17573,#17574,
#17575,#17576,#17577,#17578,#17579,#17580,#17581,#17582,#17583),
 .UNSPECIFIED.,.F.,.F.,(4,2,2,2,2,2,4),(0.,0.038846670414078,0.0823248638019488,
0.0954305814969146,0.109709621306899,0.167964127673705,0.219706780889003),
 .UNSPECIFIED.);
#241=B_SPLINE_CURVE_WITH_KNOTS('',3,(#17586,#17587,#17588,#17589,#17590,
#17591,#17592,#17593,#17594,#17595,#17596,#17597,#17598,#17599,#17600,#17601),
 .UNSPECIFIED.,.F.,.F.,(4,2,2,2,2,2,2,4),(1.00000015172994E-6,0.0540638821572014,
0.11014021259305,0.124011364716217,0.130159885420681,0.135947500297997,
0.179358237230156,0.220496798577425),.UNSPECIFIED.);
#242=B_SPLINE_CURVE_WITH_KNOTS('',3,(#17615,#17616,#17617,#17618,#17619,
#17620,#17621,#17622,#17623,#17624,#17625,#17626,#17627,#17628),
 .UNSPECIFIED.,.F.,.F.,(4,2,2,2,2,2,4),(0.,0.0389316508749848,0.0824851666861475,
0.0956106643644333,0.109894565357363,0.168167665939653,0.220077044238227),
 .UNSPECIFIED.);
#243=B_SPLINE_CURVE_WITH_KNOTS('',3,(#17631,#17632,#17633,#17634,#17635,
#17636,#17637,#17638,#17639,#17640,#17641,#17642,#17643,#17644,#17645,#17646),
 .UNSPECIFIED.,.F.,.F.,(4,2,2,2,2,2,2,4),(9.99999733883172E-7,0.0543338500939956,
0.110384986534261,0.124299234975658,0.130454753460029,0.136249978201543,
0.179744351784844,0.220987670436901),.UNSPECIFIED.);
#244=B_SPLINE_CURVE_WITH_KNOTS('',3,(#17660,#17661,#17662,#17663,#17664,
#17665,#17666,#17667,#17668,#17669,#17670,#17671,#17672,#17673,#17674,#17675),
 .UNSPECIFIED.,.F.,.F.,(4,2,2,2,2,2,2,4),(0.,0.0392686346462967,0.0832009038398811,
0.0893387848744381,0.0959430114101636,0.110232011346826,0.168506578804678,
0.220751898189097),.UNSPECIFIED.);
#245=B_SPLINE_CURVE_WITH_KNOTS('',3,(#17678,#17679,#17680,#17681,#17682,
#17683,#17684,#17685,#17686,#17687,#17688,#17689,#17690,#17691,#17692,#17693),
 .UNSPECIFIED.,.F.,.F.,(4,2,2,2,2,2,2,4),(9.99999694798638E-7,0.054765186443432,
0.110787756000683,0.124766747937571,0.130936736325675,0.136746840437026,
0.180385329895753,0.221794905871534),.UNSPECIFIED.);
#246=B_SPLINE_CURVE_WITH_KNOTS('',3,(#17707,#17708,#17709,#17710,#17711,
#17712,#17713,#17714,#17715,#17716,#17717,#17718,#17719,#17720,#17721,#17722),
 .UNSPECIFIED.,.F.,.F.,(4,2,2,2,2,2,2,4),(0.,0.0408739056675736,0.0867208225315575,
0.0898091363774199,0.0964435146083802,0.110738149517396,0.168998361491458,
0.221749184254011),.UNSPECIFIED.);
#247=B_SPLINE_CURVE_WITH_KNOTS('',3,(#17725,#17726,#17727,#17728,#17729,
#17730,#17731,#17732,#17733,#17734,#17735,#17736,#17737,#17738,#17739,#17740,
#17741,#17742),.UNSPECIFIED.,.F.,.F.,(4,2,2,2,2,2,2,2,4),(1.0000001542254E-6,
0.0553562490243362,0.111347973454671,0.125413378119285,0.13160524711844,
0.134516642372091,0.140176624201263,0.182626732587682,0.222901923225939),
 .UNSPECIFIED.);
#248=B_SPLINE_CURVE_WITH_KNOTS('',3,(#17756,#17757,#17758,#17759,#17760,
#17761,#17762,#17763,#17764,#17765,#17766,#17767,#17768,#17769,#17770,#17771),
 .UNSPECIFIED.,.F.,.F.,(4,2,2,2,2,2,2,4),(0.,0.0397423041374614,0.0841800463334577,
0.0903840838386645,0.0970580150081825,0.111357802402403,0.169584115209849,
0.223003636179411),.UNSPECIFIED.);
#249=B_SPLINE_CURVE_WITH_KNOTS('',3,(#17774,#17775,#17776,#17777,#17778,
#17779,#17780,#17781,#17782,#17783,#17784,#17785,#17786,#17787,#17788,#17789,
#17790,#17791),.UNSPECIFIED.,.F.,.F.,(4,2,2,2,2,2,2,2,4),(1.00000015667271E-6,
0.05610406193974,0.112063656979094,0.1267391800453,0.132931491224511,0.135843444218188,
0.138670210782974,0.182598137801834,0.2243485614711),.UNSPECIFIED.);
#250=B_SPLINE_CURVE_WITH_KNOTS('',3,(#17805,#17806,#17807,#17808,#17809,
#17810,#17811,#17812,#17813,#17814,#17815,#17816,#17817,#17818,#17819,#17820,
#17821,#17822),.UNSPECIFIED.,.F.,.F.,(4,2,2,2,2,2,2,2,4),(0.,0.0401135485226958,
0.0849628399941787,0.0879826739139531,0.0911130528346559,0.0978362772912048,
0.112141694870289,0.170319870714651,0.224570333252864),.UNSPECIFIED.);
#251=B_SPLINE_CURVE_WITH_KNOTS('',3,(#17825,#17826,#17827,#17828,#17829,
#17830,#17831,#17832,#17833,#17834,#17835,#17836,#17837,#17838),
 .UNSPECIFIED.,.F.,.F.,(4,2,2,2,2,2,4),(1.00000015712895E-6,0.0570055155829236,
0.112931585188432,0.127617025456474,0.152457956486069,0.190231269095715,
0.226037592522236),.UNSPECIFIED.);
#252=B_SPLINE_CURVE_WITH_KNOTS('',3,(#17914,#17915,#17916,#17917,#17918,
#17919,#17920,#17921,#17922,#17923),.UNSPECIFIED.,.F.,.F.,(4,2,2,2,4),(-0.585264524702013,
-0.413512903650657,-0.255832772201376,-0.111462969969327,-1.00000008418366E-6),
 .UNSPECIFIED.);
#253=B_SPLINE_CURVE_WITH_KNOTS('',3,(#17949,#17950,#17951,#17952,#17953,
#17954,#17955,#17956,#17957,#17958,#17959,#17960,#17961,#17962,#17963,#17964,
#17965,#17966,#17967,#17968,#17969,#17970,#17971,#17972,#17973,#17974,#17975,
#17976,#17977,#17978,#17979,#17980,#17981,#17982,#17983,#17984,#17985,#17986,
#17987,#17988,#17989,#17990,#17991,#17992,#17993,#17994,#17995,#17996,#17997,
#17998,#17999,#18000,#18001,#18002,#18003,#18004,#18005,#18006,#18007,#18008,
#18009,#18010,#18011,#18012,#18013,#18014,#18015,#18016,#18017,#18018,#18019,
#18020,#18021,#18022,#18023,#18024,#18025,#18026,#18027,#18028,#18029,#18030,
#18031,#18032,#18033,#18034,#18035,#18036,#18037,#18038,#18039,#18040,#18041,
#18042,#18043,#18044,#18045),.UNSPECIFIED.,.F.,.F.,(4,3,3,3,3,3,3,3,3,3,
3,3,3,3,3,3,3,3,3,3,3,3,3,3,3,3,3,3,3,3,3,3,4),(0.00520390849053931,0.0111835548209164,
0.012118997686005,0.0144941590703358,0.0175378069916795,0.0178073866881133,
0.0184477217574606,0.0215855252002216,0.0237812844703456,0.0244250135230592,
0.0277183120730455,0.0302238583774399,0.0310116106230319,0.034285860301359,
0.0369003334813381,0.0375601099796862,0.0419321400689772,0.0440789397487643,
0.0473302468073634,0.0488344027844652,0.050350039614148,0.0505815538659626,
0.0545489282567866,0.056285549733304,0.0570785274976558,0.0635772982300868,
0.0675410633768119,0.0700760689625178,0.07874287737638,0.0830884508286058,
0.0925219281812085,0.0961152797092054,0.10693113025843),.UNSPECIFIED.);
#254=B_SPLINE_CURVE_WITH_KNOTS('',3,(#18048,#18049,#18050,#18051,#18052,
#18053,#18054,#18055,#18056,#18057,#18058,#18059,#18060,#18061,#18062,#18063,
#18064,#18065,#18066,#18067,#18068,#18069,#18070,#18071,#18072,#18073),
 .UNSPECIFIED.,.F.,.F.,(4,2,2,2,2,2,2,2,2,2,2,2,4),(0.0365380202373312,
0.04920852331164,0.0618790595466603,0.0745495957816805,0.0872201320167008,
0.093555400134211,0.0998906682517212,0.106225936369231,0.112561204486741,
0.118896472604252,0.125231740721762,0.131567008839272,0.137902275881919),
 .UNSPECIFIED.);
#255=B_SPLINE_CURVE_WITH_KNOTS('',3,(#18153,#18154,#18155,#18156,#18157,
#18158,#18159,#18160,#18161,#18162,#18163,#18164,#18165,#18166,#18167,#18168,
#18169,#18170,#18171,#18172,#18173,#18174,#18175,#18176,#18177,#18178,#18179,
#18180,#18181,#18182,#18183,#18184,#18185,#18186,#18187,#18188,#18189,#18190,
#18191,#18192,#18193,#18194,#18195,#18196,#18197,#18198,#18199,#18200,#18201,
#18202,#18203,#18204,#18205,#18206,#18207,#18208,#18209,#18210,#18211,#18212,
#18213,#18214,#18215,#18216,#18217,#18218,#18219,#18220,#18221,#18222,#18223,
#18224,#18225),.UNSPECIFIED.,.F.,.F.,(4,3,3,3,3,3,3,3,3,3,3,3,3,3,3,3,3,
3,3,3,3,3,3,3,4),(0.00520886345403039,0.00970120603013346,0.0106439945563895,
0.0108154787072623,0.0139735509194556,0.0164220939604942,0.0171820088000305,
0.0204031582895172,0.0220287092137261,0.0237260172021366,0.0276353244669579,
0.030270007008701,0.0368139948663752,0.0388485549734217,0.043357966798868,
0.0444551702266536,0.0495865075309555,0.0499019750475477,0.0500617854798855,
0.05644595420659,0.0612750159863493,0.06953393868509,0.0724882464928131,
0.0826219208929852,0.0949147075057406),.UNSPECIFIED.);
#256=B_SPLINE_CURVE_WITH_KNOTS('',3,(#18226,#18227,#18228,#18229,#18230,
#18231,#18232,#18233,#18234,#18235,#18236,#18237),.UNSPECIFIED.,.F.,.F.,
(4,2,2,2,2,4),(0.,0.0299527642720166,0.0619423015472164,0.120911888659585,
0.180698800964258,0.241792534958426),.UNSPECIFIED.);
#257=B_SPLINE_CURVE_WITH_KNOTS('',3,(#18322,#18323,#18324,#18325,#18326,
#18327,#18328,#18329,#18330,#18331,#18332,#18333),.UNSPECIFIED.,.F.,.F.,
(4,2,2,2,2,4),(1.00000010262874E-6,0.0610883129182119,0.120980470221561,
0.180061968201615,0.212160232587823,0.242212526403015),.UNSPECIFIED.);
#258=B_SPLINE_CURVE_WITH_KNOTS('',3,(#18346,#18347,#18348,#18349,#18350,
#18351,#18352,#18353,#18354,#18355,#18356,#18357,#18358,#18359,#18360,#18361,
#18362,#18363,#18364,#18365,#18366,#18367,#18368,#18369,#18370,#18371,#18372,
#18373,#18374,#18375,#18376),.UNSPECIFIED.,.F.,.F.,(4,3,3,3,3,3,3,3,3,3,
4),(0.,0.000294988744227459,0.000591621339744572,0.000703775434139677,0.00140755086827935,
0.00211132630241903,0.00281510173655871,0.00351887717069839,0.00422265260483806,
0.00492642803897774,0.00563020347311742),.UNSPECIFIED.);
#259=B_SPLINE_CURVE_WITH_KNOTS('',3,(#18386,#18387,#18388,#18389,#18390,
#18391,#18392,#18393,#18394,#18395,#18396,#18397,#18398,#18399,#18400,#18401,
#18402,#18403,#18404,#18405,#18406,#18407,#18408,#18409,#18410,#18411,#18412,
#18413,#18414,#18415,#18416,#18417,#18418,#18419,#18420,#18421,#18422),
 .UNSPECIFIED.,.F.,.F.,(4,3,3,3,3,3,3,3,3,3,3,3,4),(0.,0.000230876498533257,
0.000465662459581963,0.000700448420630669,0.000975047322199287,0.00124663139837462,
0.00140089684126134,0.00210134526189201,0.00280179368252268,0.00350224210315334,
0.00420269052378401,0.00490313894441468,0.00560358736504535),
 .UNSPECIFIED.);
#260=B_SPLINE_CURVE_WITH_KNOTS('',3,(#18442,#18443,#18444,#18445,#18446,
#18447,#18448,#18449,#18450,#18451,#18452,#18453),.UNSPECIFIED.,.F.,.F.,
(4,2,2,2,2,4),(-0.426179478037512,-0.32445407038533,-0.214075470571974,
-0.161545733302206,-0.0817578221150203,0.),.UNSPECIFIED.);
#261=B_SPLINE_CURVE_WITH_KNOTS('',3,(#18455,#18456,#18457,#18458,#18459,
#18460),.UNSPECIFIED.,.F.,.F.,(4,2,4),(-0.150501180006049,-0.0752447108658683,
-1.00000001429512E-6),.UNSPECIFIED.);
#262=B_SPLINE_CURVE_WITH_KNOTS('',3,(#18480,#18481,#18482,#18483,#18484,
#18485),.UNSPECIFIED.,.F.,.F.,(4,2,4),(-0.150600801674249,-0.0756430925380589,
0.),.UNSPECIFIED.);
#263=B_SPLINE_CURVE_WITH_KNOTS('',3,(#18487,#18488,#18489,#18490,#18491,
#18492,#18493,#18494,#18495,#18496,#18497,#18498),.UNSPECIFIED.,.F.,.F.,
(4,2,2,2,2,4),(-0.43181117785828,-0.349168381037158,-0.268518618936436,
-0.215365450898843,-0.103278388757051,-8.24157489365263E-7),
 .UNSPECIFIED.);
#264=B_SPLINE_CURVE_WITH_KNOTS('',3,(#18522,#18523,#18524,#18525,#18526,
#18527,#18528,#18529,#18530,#18531,#18532,#18533,#18534,#18535,#18536,#18537,
#18538,#18539,#18540,#18541,#18542,#18543,#18544,#18545,#18546,#18547),
 .UNSPECIFIED.,.F.,.F.,(4,2,2,2,2,2,2,2,2,2,2,2,4),(0.,0.0178777739260339,
0.0357555478520677,0.0536333217781016,0.0715110957041355,0.0804499826671525,
0.0893888696301694,0.0983277565931864,0.107266643556203,0.11620553051922,
0.125144417482237,0.134083304445254,0.143022191408271),.UNSPECIFIED.);
#265=B_SPLINE_CURVE_WITH_KNOTS('',3,(#18550,#18551,#18552,#18553,#18554,
#18555,#18556,#18557,#18558,#18559,#18560,#18561,#18562,#18563,#18564,#18565,
#18566,#18567,#18568,#18569,#18570,#18571,#18572,#18573,#18574,#18575,#18576,
#18577),.UNSPECIFIED.,.F.,.F.,(4,2,2,2,2,2,2,2,2,2,2,2,2,4),(0.00065268600767223,
0.0096207910894088,0.0141048436302771,0.0185888961711454,0.0275570012528819,
0.0365251063346185,0.0454932114163551,0.0544613164980917,0.0634294215798282,
0.0723975266615648,0.090333736825038,0.108269946988511,0.126206157151984,
0.144142367315457),.UNSPECIFIED.);
#266=B_SPLINE_CURVE_WITH_KNOTS('',3,(#18586,#18587,#18588,#18589,#18590,
#18591,#18592,#18593,#18594,#18595,#18596,#18597,#18598,#18599,#18600,#18601,
#18602,#18603,#18604,#18605,#18606,#18607,#18608,#18609,#18610,#18611,#18612,
#18613,#18614,#18615,#18616,#18617,#18618,#18619,#18620,#18621,#18622,#18623,
#18624,#18625,#18626,#18627,#18628,#18629,#18630,#18631,#18632,#18633,#18634,
#18635,#18636,#18637,#18638,#18639,#18640,#18641,#18642,#18643,#18644,#18645,
#18646,#18647,#18648,#18649,#18650,#18651,#18652,#18653,#18654,#18655,#18656,
#18657,#18658,#18659,#18660,#18661,#18662,#18663,#18664,#18665,#18666,#18667,
#18668,#18669,#18670),.UNSPECIFIED.,.F.,.F.,(4,3,3,3,3,3,3,3,3,3,3,3,3,
3,3,3,3,3,3,3,3,3,3,3,3,3,3,3,4),(0.,0.0177783686920926,0.0180029436513539,
0.0270066186424758,0.0355567373841852,0.0360116560450794,0.0533351060762777,
0.0540227029497941,0.0711134747683703,0.0720337497834665,0.0810392838872481,
0.0888918434604629,0.0900447880456831,0.0977810278065092,0.099050320587819,
0.106670212152555,0.108055841493459,0.115559396498602,0.117061369410219,
0.121433958055277,0.124448580844648,0.126066766093759,0.128893173017671,
0.130566980042054,0.133337765190694,0.135060883634036,0.139548881847676,
0.141790875480166,0.142226949536741),.UNSPECIFIED.);
#267=B_SPLINE_CURVE_WITH_KNOTS('',3,(#18691,#18692,#18693,#18694,#18695,
#18696,#18697,#18698,#18699,#18700,#18701,#18702,#18703,#18704,#18705,#18706,
#18707,#18708,#18709,#18710,#18711,#18712,#18713,#18714,#18715,#18716,#18717,
#18718,#18719,#18720,#18721,#18722,#18723,#18724,#18725,#18726,#18727,#18728,
#18729,#18730,#18731,#18732,#18733,#18734,#18735,#18736,#18737,#18738,#18739,
#18740,#18741,#18742,#18743,#18744,#18745,#18746,#18747,#18748,#18749,#18750,
#18751,#18752,#18753,#18754,#18755,#18756,#18757,#18758,#18759,#18760,#18761,
#18762,#18763,#18764,#18765,#18766,#18767,#18768,#18769,#18770,#18771,#18772),
 .UNSPECIFIED.,.F.,.F.,(4,3,3,3,3,3,3,3,3,3,3,3,3,3,3,3,3,3,3,3,3,3,3,3,
3,3,3,4),(0.000517800053919739,0.000956159507782921,0.00320697463254193,
0.00771269228342838,0.00944404423079018,0.0134429504552714,0.0139071663192254,
0.0167424870504005,0.0183702884076606,0.0227455403801691,0.0257851780432227,
0.0272965325845311,0.0348279221194363,0.0362227767614015,0.0438706503327037,
0.045149020938272,0.0529133874777611,0.0540752651151424,0.0619560947171763,
0.070998836612136,0.0719277534688833,0.0890842949457832,0.0897802418226242,
0.107169748483184,0.107632730176365,0.125255111030166,0.125485218530106,
0.143337706883847),.UNSPECIFIED.);
#268=B_SPLINE_CURVE_WITH_KNOTS('',3,(#18872,#18873,#18874,#18875,#18876,
#18877,#18878,#18879,#18880,#18881,#18882,#18883,#18884,#18885,#18886,#18887,
#18888,#18889,#18890,#18891,#18892,#18893,#18894,#18895,#18896,#18897,#18898,
#18899,#18900,#18901,#18902,#18903,#18904,#18905,#18906,#18907,#18908,#18909,
#18910,#18911,#18912,#18913,#18914,#18915,#18916,#18917,#18918,#18919,#18920,
#18921,#18922,#18923,#18924,#18925,#18926,#18927,#18928,#18929,#18930,#18931,
#18932,#18933,#18934,#18935,#18936,#18937,#18938),.UNSPECIFIED.,.F.,.F.,
(4,3,3,3,3,3,3,3,3,3,3,3,3,3,3,3,3,3,3,3,3,3,4),(3.24873139256393E-12,0.000789113203271446,
0.000792375749127745,0.00141612050710302,0.00157874172054858,0.00158475149825549,
0.00222253730489919,0.00236930376886044,0.00237712724738323,0.00294445569018658,
0.00316101198412218,0.00316950299651097,0.00395398652820353,0.00396187874563871,
0.00461756528354283,0.00474818189970434,0.00475425449476645,0.0054660318604933,
0.00554328490870971,0.00554663024389419,0.00586525399963526,0.00618286705330126,
0.00633900599302193),.UNSPECIFIED.);
#269=B_SPLINE_CURVE_WITH_KNOTS('',3,(#19047,#19048,#19049,#19050,#19051,
#19052,#19053,#19054,#19055,#19056,#19057,#19058,#19059,#19060,#19061,#19062,
#19063,#19064,#19065,#19066,#19067,#19068,#19069,#19070,#19071,#19072,#19073,
#19074,#19075,#19076,#19077,#19078,#19079,#19080,#19081,#19082,#19083,#19084,
#19085,#19086,#19087,#19088,#19089,#19090,#19091,#19092,#19093,#19094,#19095,
#19096,#19097,#19098,#19099,#19100,#19101,#19102,#19103,#19104,#19105,#19106,
#19107,#19108,#19109,#19110,#19111,#19112,#19113,#19114,#19115,#19116),
 .UNSPECIFIED.,.F.,.F.,(4,3,3,3,3,3,3,3,3,3,3,3,3,3,3,3,3,3,3,3,3,3,3,4),
(0.,0.000792526143918412,0.000795787604514349,0.00142673915028219,0.00158505228783682,
0.00159109328876066,0.00237757843175524,0.00238542369538965,0.00299442831057784,
0.00317010457567365,0.0031785911693371,0.00375515851311093,0.00396263071959206,
0.00397045983119314,0.00448222397781173,0.00475515686351047,0.00476119515944008,
0.00506130515504216,0.0053643750105131,0.00554768300742888,0.00580423226308875,
0.00607222070558002,0.00632304467713367,0.0063402091480713),
 .UNSPECIFIED.);
#270=B_SPLINE_CURVE_WITH_KNOTS('',3,(#19127,#19128,#19129,#19130,#19131,
#19132,#19133,#19134,#19135,#19136,#19137,#19138,#19139,#19140,#19141,#19142,
#19143,#19144,#19145,#19146,#19147,#19148,#19149,#19150),.UNSPECIFIED.,
 .F.,.F.,(4,2,2,2,2,2,2,2,2,2,2,4),(-0.19450411922911,-0.126334189862308,
-0.111286464135786,-0.103050819900779,-0.10157129690467,-0.100782940759509,
-0.100118651209767,-0.0993103301884034,-0.0978953228319982,-0.0918418092473422,
-0.074264450184147,-3.29579807889502E-10),.UNSPECIFIED.);
#271=B_SPLINE_CURVE_WITH_KNOTS('',3,(#19151,#19152,#19153,#19154),
 .UNSPECIFIED.,.F.,.F.,(4,4),(0.,0.000312238933267578),.UNSPECIFIED.);
#272=B_SPLINE_CURVE_WITH_KNOTS('',3,(#19165,#19166,#19167,#19168,#19169,
#19170),.UNSPECIFIED.,.F.,.F.,(4,2,4),(-0.149813019636341,-0.0742119267126466,
0.),.UNSPECIFIED.);
#273=B_SPLINE_CURVE_WITH_KNOTS('',3,(#19172,#19173,#19174,#19175,#19176,
#19177),.UNSPECIFIED.,.F.,.F.,(4,2,4),(-0.154390811946475,-0.0750953953452426,
-9.99999601875023E-7),.UNSPECIFIED.);
#274=B_SPLINE_CURVE_WITH_KNOTS('',3,(#19180,#19181,#19182,#19183,#19184,
#19185),.UNSPECIFIED.,.F.,.F.,(4,2,4),(-0.149813019635849,-0.0742119267123349,
0.),.UNSPECIFIED.);
#275=B_SPLINE_CURVE_WITH_KNOTS('',3,(#19187,#19188,#19189,#19190,#19191,
#19192),.UNSPECIFIED.,.F.,.F.,(4,2,4),(-0.154390811945437,-0.0750948817400542,
-9.99999603170351E-7),.UNSPECIFIED.);
#276=B_SPLINE_CURVE_WITH_KNOTS('',3,(#19195,#19196,#19197,#19198,#19199,
#19200),.UNSPECIFIED.,.F.,.F.,(4,2,4),(-0.149813019635709,-0.0742114219215882,
0.),.UNSPECIFIED.);
#277=B_SPLINE_CURVE_WITH_KNOTS('',3,(#19202,#19203,#19204,#19205,#19206,
#19207),.UNSPECIFIED.,.F.,.F.,(4,2,4),(-0.154390811947745,-0.0750953953455204,
-9.99999601236645E-7),.UNSPECIFIED.);
#278=B_SPLINE_CURVE_WITH_KNOTS('',3,(#19210,#19211,#19212,#19213,#19214,
#19215),.UNSPECIFIED.,.F.,.F.,(4,2,4),(-0.149813019636192,-0.0742119267126041,
0.),.UNSPECIFIED.);
#279=B_SPLINE_CURVE_WITH_KNOTS('',3,(#19217,#19218,#19219,#19220,#19221,
#19222),.UNSPECIFIED.,.F.,.F.,(4,2,4),(-0.154390811946182,-0.0750948817402176,
-9.99999601734471E-7),.UNSPECIFIED.);
#280=B_SPLINE_CURVE_WITH_KNOTS('',3,(#19225,#19226,#19227,#19228,#19229,
#19230),.UNSPECIFIED.,.F.,.F.,(4,2,4),(-0.149813019636222,-0.0742119267126633,
0.),.UNSPECIFIED.);
#281=B_SPLINE_CURVE_WITH_KNOTS('',3,(#19232,#19233,#19234,#19235,#19236,
#19237),.UNSPECIFIED.,.F.,.F.,(4,2,4),(-0.154390811946885,-0.0750948817403378,
-9.99999602331216E-7),.UNSPECIFIED.);
#282=B_SPLINE_CURVE_WITH_KNOTS('',3,(#19240,#19241,#19242,#19243,#19244,
#19245),.UNSPECIFIED.,.F.,.F.,(4,2,4),(-0.149813019636188,-0.0742114219217932,
0.),.UNSPECIFIED.);
#283=B_SPLINE_CURVE_WITH_KNOTS('',3,(#19247,#19248,#19249,#19250,#19251,
#19252),.UNSPECIFIED.,.F.,.F.,(4,2,4),(-0.154390811947138,-0.0750948817403358,
-9.99999601842204E-7),.UNSPECIFIED.);
#284=B_SPLINE_CURVE_WITH_KNOTS('',3,(#19255,#19256,#19257,#19258,#19259,
#19260),.UNSPECIFIED.,.F.,.F.,(4,2,4),(-0.1498130196363,-0.0742119267124509,
0.),.UNSPECIFIED.);
#285=B_SPLINE_CURVE_WITH_KNOTS('',3,(#19262,#19263,#19264,#19265,#19266,
#19267),.UNSPECIFIED.,.F.,.F.,(4,2,4),(-0.1167939430675,-0.0559485367490526,
-9.9999970383513E-7),.UNSPECIFIED.);
#286=B_SPLINE_CURVE_WITH_KNOTS('',3,(#19283,#19284,#19285,#19286,#19287,
#19288),.UNSPECIFIED.,.F.,.F.,(4,2,4),(9.99999616665374E-7,0.0121034221554694,
0.0242049584783662),.UNSPECIFIED.);
#287=B_SPLINE_CURVE_WITH_KNOTS('',3,(#19289,#19290,#19291,#19292,#19293,
#19294,#19295,#19296,#19297,#19298,#19299,#19300,#19301,#19302),
 .UNSPECIFIED.,.F.,.F.,(4,2,2,2,2,2,4),(0.,0.0409644441214631,0.0887268040598564,
0.0955303651869036,0.109712942382492,0.168590020103833,0.219688229784175),
 .UNSPECIFIED.);
#288=B_SPLINE_CURVE_WITH_KNOTS('',3,(#19304,#19305,#19306,#19307,#19308,
#19309,#19310,#19311,#19312,#19313,#19314,#19315,#19316,#19317,#19318,#19319,
#19320,#19321,#19322,#19323,#19324,#19325,#19326,#19327,#19328,#19329,#19330,
#19331),.UNSPECIFIED.,.F.,.F.,(4,2,2,2,2,2,2,2,2,2,2,2,2,4),(-0.195818704088962,
-0.143355144115657,-0.110356347530556,-0.0979570470431692,-0.090786108819357,
-0.0895445881165381,-0.0888007558059985,-0.0882295747566688,-0.087617885883006,
-0.0866600191131884,-0.0836895532525834,-0.0674705918142883,-0.0363980900813506,
-9.99670535101194E-7),.UNSPECIFIED.);
#289=B_SPLINE_CURVE_WITH_KNOTS('',3,(#19345,#19346,#19347,#19348,#19349,
#19350,#19351,#19352,#19353,#19354,#19355,#19356,#19357,#19358,#19359,#19360,
#19361,#19362,#19363),.UNSPECIFIED.,.F.,.F.,(4,3,3,3,3,3,4),(5.81811766227498E-12,
0.000713015175406057,0.00148279719273555,0.0017944978017605,0.00183065943066078,
0.00325218021980356,0.00366131886132156),.UNSPECIFIED.);
#290=B_SPLINE_CURVE_WITH_KNOTS('',3,(#19365,#19366,#19367,#19368,#19369,
#19370,#19371,#19372,#19373,#19374,#19375,#19376,#19377,#19378,#19379,#19380,
#19381,#19382,#19383,#19384,#19385,#19386,#19387,#19388,#19389),
 .UNSPECIFIED.,.F.,.F.,(4,3,3,3,3,3,3,3,4),(0.,0.000282845373659893,0.000537791840235127,
0.000538908034209594,0.000878730315925117,0.00107558368047025,0.00107834483611328,
0.00176407748649149,0.00215116736094051),.UNSPECIFIED.);
#291=B_SPLINE_CURVE_WITH_KNOTS('',3,(#19390,#19391,#19392,#19393),
 .UNSPECIFIED.,.F.,.F.,(4,4),(0.,6.29047409436179E-5),.UNSPECIFIED.);
#292=B_SPLINE_CURVE_WITH_KNOTS('',3,(#19395,#19396,#19397,#19398),
 .UNSPECIFIED.,.F.,.F.,(4,4),(0.,6.29047409436508E-5),.UNSPECIFIED.);
#293=B_SPLINE_CURVE_WITH_KNOTS('',3,(#19400,#19401,#19402,#19403,#19404,
#19405,#19406,#19407,#19408,#19409,#19410,#19411,#19412,#19413,#19414,#19415,
#19416,#19417,#19418,#19419,#19420,#19421,#19422,#19423,#19424),
 .UNSPECIFIED.,.F.,.F.,(4,3,3,3,3,3,3,3,4),(0.,0.000685296287045248,0.00107213984073947,
0.00107489923933792,0.00141450527734773,0.0016112333753157,0.0016123488590069,
0.00191262071533291,0.00214979847867587),.UNSPECIFIED.);
#294=B_SPLINE_CURVE_WITH_KNOTS('',3,(#19425,#19426,#19427,#19428,#19429,
#19430,#19431,#19432,#19433,#19434,#19435,#19436,#19437,#19438,#19439,#19440,
#19441,#19442,#19443),.UNSPECIFIED.,.F.,.F.,(4,3,3,3,3,3,4),(0.,0.000899413916680641,
0.00174431342931246,0.00179882783336128,0.00256218526438471,0.00331004957902007,
0.00359765561291069),.UNSPECIFIED.);
#295=B_SPLINE_CURVE_WITH_KNOTS('',3,(#19448,#19449,#19450,#19451,#19452,
#19453),.UNSPECIFIED.,.F.,.F.,(4,2,4),(-0.0144436412707524,-0.00699620646723456,
-6.60336511512649E-9),.UNSPECIFIED.);
#296=B_SPLINE_CURVE_WITH_KNOTS('',3,(#19455,#19456,#19457,#19458,#19459,
#19460),.UNSPECIFIED.,.F.,.F.,(4,2,4),(-0.0144503347921917,-0.00745133852662736,
-1.00730609309307E-6),.UNSPECIFIED.);
#297=B_SPLINE_CURVE_WITH_KNOTS('',3,(#19475,#19476,#19477,#19478),
 .UNSPECIFIED.,.F.,.F.,(4,4),(0.,0.00173428636340849),.UNSPECIFIED.);
#298=B_SPLINE_CURVE_WITH_KNOTS('',3,(#19480,#19481,#19482,#19483,#19484,
#19485,#19486,#19487,#19488,#19489,#19490,#19491,#19492,#19493,#19494,#19495,
#19496,#19497,#19498,#19499,#19500,#19501,#19502,#19503,#19504,#19505,#19506,
#19507,#19508,#19509,#19510,#19511,#19512,#19513,#19514,#19515,#19516,#19517,
#19518,#19519,#19520,#19521,#19522,#19523,#19524,#19525),.UNSPECIFIED.,
 .F.,.F.,(4,3,3,3,3,3,3,3,3,3,3,3,3,3,3,4),(0.,9.12787148238181E-5,0.000183921671662766,
0.000256351757877802,0.000311479035290493,0.000328781844092839,0.000439888590826784,
0.000526050950548542,0.000530451527395148,0.000625111740468468,0.000657563688185677,
0.000756198241413529,0.000800848465156635,0.000892918501575997,0.000983117535815826,
0.00105210190109708),.UNSPECIFIED.);
#299=B_SPLINE_CURVE_WITH_KNOTS('',3,(#19533,#19534,#19535,#19536,#19537,
#19538,#19539,#19540,#19541,#19542,#19543,#19544,#19545,#19546,#19547,#19548,
#19549,#19550,#19551,#19552,#19553,#19554,#19555,#19556,#19557,#19558,#19559,
#19560,#19561,#19562,#19563,#19564,#19565,#19566,#19567,#19568,#19569,#19570,
#19571,#19572,#19573,#19574,#19575,#19576,#19577,#19578,#19579,#19580,#19581),
 .UNSPECIFIED.,.F.,.F.,(4,3,3,3,3,3,3,3,3,3,3,3,3,3,3,3,4),(0.,0.000112411075416676,
0.00022668855713591,0.000256939338114826,0.000281905681799926,0.00038239262866012,
0.000399717078062952,0.000493967094647472,0.000528483381613059,0.000532956104083936,
0.000646963423007012,0.00066619513010492,0.000766124399620658,0.000822145470081397,
0.000917119711214598,0.00101032641648309,0.00106591220816787),
 .UNSPECIFIED.);
#300=B_SPLINE_CURVE_WITH_KNOTS('',3,(#19583,#19584,#19585,#19586),
 .UNSPECIFIED.,.F.,.F.,(4,4),(0.,0.00173428636340849),.UNSPECIFIED.);
#301=B_SPLINE_CURVE_WITH_KNOTS('',3,(#19591,#19592,#19593,#19594,#19595,
#19596,#19597,#19598,#19599,#19600,#19601,#19602,#19603,#19604),
 .UNSPECIFIED.,.F.,.F.,(4,2,2,2,2,2,4),(-0.0976421838858201,-0.084189955512187,
-0.0697581457509971,-0.0491108456698284,-0.0297735319812699,-0.0141869021647831,
0.),.UNSPECIFIED.);
#302=B_SPLINE_CURVE_WITH_KNOTS('',3,(#19609,#19610,#19611,#19612,#19613,
#19614),.UNSPECIFIED.,.F.,.F.,(4,2,4),(-0.0567997771842775,-0.0284184953580656,
-1.01442404849064E-6),.UNSPECIFIED.);
#303=B_SPLINE_CURVE_WITH_KNOTS('',3,(#19663,#19664,#19665,#19666,#19667,
#19668,#19669,#19670,#19671,#19672,#19673,#19674,#19675,#19676),
 .UNSPECIFIED.,.F.,.F.,(4,2,2,2,2,2,4),(0.,0.0141504479466231,0.0296944189662601,
0.0490192876277638,0.0696539086346055,0.0841403129979988,0.0976417165566767),
 .UNSPECIFIED.);
#304=B_SPLINE_CURVE_WITH_KNOTS('',3,(#19715,#19716,#19717,#19718,#19719,
#19720),.UNSPECIFIED.,.F.,.F.,(4,2,4),(1.01442403287893E-6,0.0284184953584133,
0.0567997771849387),.UNSPECIFIED.);
#305=B_SPLINE_CURVE_WITH_KNOTS('',3,(#19724,#19725,#19726,#19727,#19728,
#19729,#19730,#19731,#19732,#19733),.UNSPECIFIED.,.F.,.F.,(4,3,3,4),(4.30118003192922E-9,
0.00131474961221221,0.00268758862115831,0.0031904227463795),
 .UNSPECIFIED.);
#306=B_SPLINE_CURVE_WITH_KNOTS('',3,(#19738,#19739,#19740,#19741,#19742,
#19743,#19744,#19745,#19746,#19747),.UNSPECIFIED.,.F.,.F.,(4,3,3,4),(0.,
0.00137283900902173,0.00187567313416777,0.00319041844519952),
 .UNSPECIFIED.);
#307=B_SPLINE_CURVE_WITH_KNOTS('',3,(#19790,#19791,#19792,#19793,#19794,
#19795,#19796,#19797,#19798,#19799,#19800,#19801,#19802,#19803,#19804,#19805,
#19806,#19807,#19808,#19809,#19810,#19811,#19812,#19813,#19814,#19815,#19816,
#19817,#19818,#19819,#19820),.UNSPECIFIED.,.F.,.F.,(4,3,3,3,3,3,3,3,3,3,
4),(0.,0.000157386647060973,0.000332445535114511,0.000489094642209349,0.000494201771608867,
0.000710151345833458,0.000951984363272296,0.000988403543217735,0.000989925971234007,
0.00149956601242565,0.00197680708643547),.UNSPECIFIED.);
#308=B_SPLINE_CURVE_WITH_KNOTS('',3,(#19826,#19827,#19828,#19829,#19830,
#19831,#19832,#19833,#19834,#19835,#19836,#19837,#19838,#19839,#19840,#19841,
#19842,#19843,#19844,#19845,#19846,#19847,#19848,#19849,#19850,#19851,#19852,
#19853,#19854,#19855,#19856),.UNSPECIFIED.,.F.,.F.,(4,3,3,3,3,3,3,3,3,3,
4),(0.,0.000509513490104227,0.000986636057298634,0.000988158107272369,0.00123519763409046,
0.00145109358469587,0.00148223716090855,0.00148734302212855,0.00166747975270183,
0.00182718054780211,0.00197631621454474),.UNSPECIFIED.);
#309=B_SPLINE_CURVE_WITH_KNOTS('',3,(#19979,#19980,#19981,#19982,#19983,
#19984),.UNSPECIFIED.,.F.,.F.,(4,2,4),(-0.107519161292799,-0.0637323978923038,
0.),.UNSPECIFIED.);
#532=(
BOUNDED_SURFACE()
B_SPLINE_SURFACE(3,2,((#17291,#17292,#17293),(#17294,#17295,#17296),(#17297,
#17298,#17299),(#17300,#17301,#17302)),.UNSPECIFIED.,.F.,.F.,.F.)
B_SPLINE_SURFACE_WITH_KNOTS((4,4),(3,3),(0.0596721496079926,0.060305624008707),
(0.0470793423724159,1.),.UNSPECIFIED.)
GEOMETRIC_REPRESENTATION_ITEM()
RATIONAL_B_SPLINE_SURFACE(((0.973719934576668,0.720896001313625,1.),(0.973719934576668,
0.720896001313625,1.),(0.973719934576668,0.720896001313625,1.),(0.973719934576668,
0.720896001313625,1.)))
REPRESENTATION_ITEM('')
SURFACE()
);
#533=(
BOUNDED_SURFACE()
B_SPLINE_SURFACE(3,2,((#17337,#17338,#17339),(#17340,#17341,#17342),(#17343,
#17344,#17345),(#17346,#17347,#17348)),.UNSPECIFIED.,.F.,.F.,.F.)
B_SPLINE_SURFACE_WITH_KNOTS((4,4),(3,3),(0.0581736933140078,0.0588009183988192),
(0.0549949072393295,1.),.UNSPECIFIED.)
GEOMETRIC_REPRESENTATION_ITEM()
RATIONAL_B_SPLINE_SURFACE(((0.969556405029951,0.723214416586222,1.),(0.969556405029951,
0.723214416586222,1.),(0.969556405029951,0.723214416586222,1.),(0.969556405029951,
0.723214416586222,1.)))
REPRESENTATION_ITEM('')
SURFACE()
);
#534=(
BOUNDED_SURFACE()
B_SPLINE_SURFACE(3,2,((#17383,#17384,#17385),(#17386,#17387,#17388),(#17389,
#17390,#17391),(#17392,#17393,#17394)),.UNSPECIFIED.,.F.,.F.,.F.)
B_SPLINE_SURFACE_WITH_KNOTS((4,4),(3,3),(0.0566744883899997,0.0572968072375656),
(0.0615688709473457,1.),.UNSPECIFIED.)
GEOMETRIC_REPRESENTATION_ITEM()
RATIONAL_B_SPLINE_SURFACE(((0.966154346222294,0.725139885977026,1.),(0.966154346222294,
0.725139885977026,1.),(0.966154346222294,0.725139885977026,1.),(0.966154346222294,
0.725139885977026,1.)))
REPRESENTATION_ITEM('')
SURFACE()
);
#535=(
BOUNDED_SURFACE()
B_SPLINE_SURFACE(3,2,((#17427,#17428,#17429),(#17430,#17431,#17432),(#17433,
#17434,#17435),(#17436,#17437,#17438)),.UNSPECIFIED.,.F.,.F.,.F.)
B_SPLINE_SURFACE_WITH_KNOTS((4,4),(3,3),(0.0551745403883536,0.0557932703572333),
(0.066777420683245,1.),.UNSPECIFIED.)
GEOMETRIC_REPRESENTATION_ITEM()
RATIONAL_B_SPLINE_SURFACE(((0.963494845514688,0.726665434874523,1.),(0.963494845514688,
0.726665434874523,1.),(0.963494845514688,0.726665434874523,1.),(0.963494845514688,
0.726665434874523,1.)))
REPRESENTATION_ITEM('')
SURFACE()
);
#536=(
BOUNDED_SURFACE()
B_SPLINE_SURFACE(3,2,((#17471,#17472,#17473),(#17474,#17475,#17476),(#17477,
#17478,#17479),(#17480,#17481,#17482)),.UNSPECIFIED.,.F.,.F.,.F.)
B_SPLINE_SURFACE_WITH_KNOTS((4,4),(3,3),(0.0536738567287748,0.0542902895645969),
(0.0706052509682322,1.),.UNSPECIFIED.)
GEOMETRIC_REPRESENTATION_ITEM()
RATIONAL_B_SPLINE_SURFACE(((0.961560606385539,0.727786580407766,1.),(0.961560606385539,
0.727786580407766,1.),(0.961560606385539,0.727786580407765,1.),(0.961560606385539,
0.727786580407765,1.)))
REPRESENTATION_ITEM('')
SURFACE()
);
#537=(
BOUNDED_SURFACE()
B_SPLINE_SURFACE(3,2,((#17515,#17516,#17517),(#17518,#17519,#17520),(#17521,
#17522,#17523),(#17524,#17525,#17526)),.UNSPECIFIED.,.F.,.F.,.F.)
B_SPLINE_SURFACE_WITH_KNOTS((4,4),(3,3),(0.0521724469311448,0.0527878485478844),
(0.073047320944285,1.),.UNSPECIFIED.)
GEOMETRIC_REPRESENTATION_ITEM()
RATIONAL_B_SPLINE_SURFACE(((0.960335574438944,0.728501846143617,1.),(0.960335574438944,
0.728501846143617,1.),(0.960335574438944,0.728501846143619,1.),(0.960335574438944,
0.728501846143619,1.)))
REPRESENTATION_ITEM('')
SURFACE()
);
#538=(
BOUNDED_SURFACE()
B_SPLINE_SURFACE(3,2,((#17557,#17558,#17559),(#17560,#17561,#17562),(#17563,
#17564,#17565),(#17566,#17567,#17568)),.UNSPECIFIED.,.F.,.F.,.F.)
B_SPLINE_SURFACE_WITH_KNOTS((4,4),(3,3),(0.15547618557744,0.156093772145324),
(0.073524259555501,1.),.UNSPECIFIED.)
GEOMETRIC_REPRESENTATION_ITEM()
RATIONAL_B_SPLINE_SURFACE(((0.960097140048281,0.728641538228635,1.),(0.960097140048281,
0.728641538228635,1.),(0.960097140048281,0.728641538228634,1.),(0.960097140048281,
0.728641538228634,1.)))
REPRESENTATION_ITEM('')
SURFACE()
);
#539=(
BOUNDED_SURFACE()
B_SPLINE_SURFACE(3,2,((#17602,#17603,#17604),(#17605,#17606,#17607),(#17608,
#17609,#17610),(#17611,#17612,#17613)),.UNSPECIFIED.,.F.,.F.,.F.)
B_SPLINE_SURFACE_WITH_KNOTS((4,4),(3,3),(0.153971233644507,0.154591580945739),
(0.0715119122999407,1.),.UNSPECIFIED.)
GEOMETRIC_REPRESENTATION_ITEM()
RATIONAL_B_SPLINE_SURFACE(((0.961104976307929,0.728052135363584,1.),(0.961104976307929,
0.728052135363584,1.),(0.961104976307929,0.728052135363584,1.),(0.961104976307929,
0.728052135363584,1.)))
REPRESENTATION_ITEM('')
SURFACE()
);
#540=(
BOUNDED_SURFACE()
B_SPLINE_SURFACE(3,2,((#17647,#17648,#17649),(#17650,#17651,#17652),(#17653,
#17654,#17655),(#17656,#17657,#17658)),.UNSPECIFIED.,.F.,.F.,.F.)
B_SPLINE_SURFACE_WITH_KNOTS((4,4),(3,3),(0.152465422311365,0.153089822150018),
(0.0681150405736641,1.),.UNSPECIFIED.)
GEOMETRIC_REPRESENTATION_ITEM()
RATIONAL_B_SPLINE_SURFACE(((0.962816982205886,0.727057214669775,1.),(0.962816982205886,
0.727057214669775,1.),(0.962816982205886,0.727057214669777,1.),(0.962816982205886,
0.727057214669777,1.)))
REPRESENTATION_ITEM('')
SURFACE()
);
#541=(
BOUNDED_SURFACE()
B_SPLINE_SURFACE(3,2,((#17694,#17695,#17696),(#17697,#17698,#17699),(#17700,
#17701,#17702),(#17703,#17704,#17705)),.UNSPECIFIED.,.F.,.F.,.F.)
B_SPLINE_SURFACE_WITH_KNOTS((4,4),(3,3),(0.150958741315287,0.151588591705843),
(0.0633354277393988,1.),.UNSPECIFIED.)
GEOMETRIC_REPRESENTATION_ITEM()
RATIONAL_B_SPLINE_SURFACE(((0.965248775304359,0.725657298482067,1.),(0.965248775304359,
0.725657298482067,1.),(0.965248775304359,0.725657298482067,1.),(0.965248775304359,
0.725657298482067,1.)))
REPRESENTATION_ITEM('')
SURFACE()
);
#542=(
BOUNDED_SURFACE()
B_SPLINE_SURFACE(3,2,((#17743,#17744,#17745),(#17746,#17747,#17748),(#17749,
#17750,#17751),(#17752,#17753,#17754)),.UNSPECIFIED.,.F.,.F.,.F.)
B_SPLINE_SURFACE_WITH_KNOTS((4,4),(3,3),(0.149451183265075,0.150087942103155),
(0.0571854695619357,1.),.UNSPECIFIED.)
GEOMETRIC_REPRESENTATION_ITEM()
RATIONAL_B_SPLINE_SURFACE(((0.968417153380738,0.723856017435902,1.),(0.968417153380738,
0.723856017435902,1.),(0.968417153380738,0.723856017435903,1.),(0.968417153380738,
0.723856017435903,1.)))
REPRESENTATION_ITEM('')
SURFACE()
);
#543=(
BOUNDED_SURFACE()
B_SPLINE_SURFACE(3,2,((#17792,#17793,#17794),(#17795,#17796,#17797),(#17798,
#17799,#17800),(#17801,#17802,#17803)),.UNSPECIFIED.,.F.,.F.,.F.)
B_SPLINE_SURFACE_WITH_KNOTS((4,4),(3,3),(0.147942744613282,0.148587704815656),
(0.0496865592693353,1.),.UNSPECIFIED.)
GEOMETRIC_REPRESENTATION_ITEM()
RATIONAL_B_SPLINE_SURFACE(((0.972340450159485,0.721659637462709,1.),(0.972340450159485,
0.721659637462709,1.),(0.972340450159485,0.721659637462709,1.),(0.972340450159485,
0.721659637462709,1.)))
REPRESENTATION_ITEM('')
SURFACE()
);
#544=(
BOUNDED_SURFACE()
B_SPLINE_SURFACE(3,2,((#18074,#18075,#18076),(#18077,#18078,#18079),(#18080,
#18081,#18082),(#18083,#18084,#18085),(#18086,#18087,#18088),(#18089,#18090,
#18091),(#18092,#18093,#18094),(#18095,#18096,#18097),(#18098,#18099,#18100),
(#18101,#18102,#18103),(#18104,#18105,#18106),(#18107,#18108,#18109),(#18110,
#18111,#18112),(#18113,#18114,#18115),(#18116,#18117,#18118),(#18119,#18120,
#18121),(#18122,#18123,#18124),(#18125,#18126,#18127),(#18128,#18129,#18130),
(#18131,#18132,#18133),(#18134,#18135,#18136),(#18137,#18138,#18139),(#18140,
#18141,#18142),(#18143,#18144,#18145),(#18146,#18147,#18148),(#18149,#18150,
#18151)),.UNSPECIFIED.,.F.,.F.,.F.)
B_SPLINE_SURFACE_WITH_KNOTS((4,2,2,2,2,2,2,2,2,2,2,2,4),(3,3),(0.0852283172250545,
0.098258593834224,0.111288870443393,0.124319147052563,0.137349423661732,
0.143864561966317,0.150379700270902,0.156894838575487,0.163409976880071,
0.169925115184656,0.176440253489241,0.182955391793825,0.18947053009841),
(0.,1.),.UNSPECIFIED.)
GEOMETRIC_REPRESENTATION_ITEM()
RATIONAL_B_SPLINE_SURFACE(((1.,0.707106781186546,1.),(1.,0.707106781186546,
1.),(1.,0.707106781186546,1.),(1.,0.707106781186546,1.),(1.,0.707106781186548,
1.),(1.,0.707106781186548,1.),(1.,0.707106781186548,1.),(1.,0.707106781186548,
1.),(1.,0.707106781186548,1.),(1.,0.707106781186548,1.),(1.,0.707106781186547,
1.),(1.,0.707106781186547,1.),(1.,0.707106781186548,1.),(1.,0.707106781186548,
1.),(1.,0.707106781186548,1.),(1.,0.707106781186548,1.),(1.,0.707106781186548,
1.),(1.,0.707106781186548,1.),(1.,0.707106781186547,1.),(1.,0.707106781186547,
1.),(1.,0.707106781186548,1.),(1.,0.707106781186548,1.),(1.,0.707106781186548,
1.),(1.,0.707106781186548,1.),(1.,0.707106781186548,1.),(1.,0.707106781186548,
1.)))
REPRESENTATION_ITEM('')
SURFACE()
);
#545=(
BOUNDED_SURFACE()
B_SPLINE_SURFACE(3,2,((#18238,#18239,#18240),(#18241,#18242,#18243),(#18244,
#18245,#18246),(#18247,#18248,#18249),(#18250,#18251,#18252),(#18253,#18254,
#18255),(#18256,#18257,#18258),(#18259,#18260,#18261),(#18262,#18263,#18264),
(#18265,#18266,#18267),(#18268,#18269,#18270),(#18271,#18272,#18273),(#18274,
#18275,#18276),(#18277,#18278,#18279),(#18280,#18281,#18282),(#18283,#18284,
#18285),(#18286,#18287,#18288),(#18289,#18290,#18291),(#18292,#18293,#18294),
(#18295,#18296,#18297),(#18298,#18299,#18300),(#18301,#18302,#18303),(#18304,
#18305,#18306),(#18307,#18308,#18309),(#18310,#18311,#18312),(#18313,#18314,
#18315),(#18316,#18317,#18318),(#18319,#18320,#18321)),.UNSPECIFIED.,.F.,
 .F.,.F.)
B_SPLINE_SURFACE_WITH_KNOTS((4,2,2,2,2,2,2,2,2,2,2,2,2,4),(3,3),(0.0184185986382119,
0.0249387797460936,0.0281988703000345,0.0314589608539753,0.037979141961857,
0.0444993230697387,0.0510195041776203,0.057539685285502,0.0640598663933837,
0.0705800475012654,0.0836204097170287,0.0966607719327921,0.109701134148555,
0.122741496364319),(0.,1.),.UNSPECIFIED.)
GEOMETRIC_REPRESENTATION_ITEM()
RATIONAL_B_SPLINE_SURFACE(((1.,0.707106781186548,1.),(1.,0.707106781186548,
1.),(1.,0.707106781186548,1.),(1.,0.707106781186548,1.),(1.,0.707106781186547,
1.),(1.,0.707106781186547,1.),(1.,0.707106781186548,1.),(1.,0.707106781186548,
1.),(1.,0.707106781186548,1.),(1.,0.707106781186548,1.),(1.,0.707106781186548,
1.),(1.,0.707106781186548,1.),(1.,0.707106781186548,1.),(1.,0.707106781186548,
1.),(1.,0.707106781186547,1.),(1.,0.707106781186547,1.),(1.,0.707106781186548,
1.),(1.,0.707106781186548,1.),(1.,0.707106781186548,1.),(1.,0.707106781186548,
1.),(1.,0.707106781186548,1.),(1.,0.707106781186548,1.),(1.,0.707106781186548,
1.),(1.,0.707106781186548,1.),(1.,0.707106781186548,1.),(1.,0.707106781186548,
1.),(1.,0.707106781186548,1.),(1.,0.707106781186548,1.)))
REPRESENTATION_ITEM('')
SURFACE()
);
#546=(
BOUNDED_SURFACE()
B_SPLINE_SURFACE(3,2,((#18776,#18777,#18778),(#18779,#18780,#18781),(#18782,
#18783,#18784),(#18785,#18786,#18787),(#18788,#18789,#18790),(#18791,#18792,
#18793),(#18794,#18795,#18796),(#18797,#18798,#18799),(#18800,#18801,#18802),
(#18803,#18804,#18805),(#18806,#18807,#18808),(#18809,#18810,#18811),(#18812,
#18813,#18814),(#18815,#18816,#18817),(#18818,#18819,#18820),(#18821,#18822,
#18823),(#18824,#18825,#18826),(#18827,#18828,#18829),(#18830,#18831,#18832),
(#18833,#18834,#18835),(#18836,#18837,#18838),(#18839,#18840,#18841),(#18842,
#18843,#18844),(#18845,#18846,#18847),(#18848,#18849,#18850),(#18851,#18852,
#18853),(#18854,#18855,#18856),(#18857,#18858,#18859),(#18860,#18861,#18862),
(#18863,#18864,#18865),(#18866,#18867,#18868),(#18869,#18870,#18871)),
 .UNSPECIFIED.,.F.,.F.,.F.)
B_SPLINE_SURFACE_WITH_KNOTS((4,2,2,2,2,2,2,2,2,2,2,2,2,2,2,4),(3,3),(0.0508378190163745,
0.0688435419383206,0.0868492648602666,0.104854987782213,0.122860710704159,
0.131863572165132,0.140866433626105,0.149869295087078,0.158872156548051,
0.167875018009024,0.176877879469997,0.18588074093097,0.190382171661456,
0.1926328870267,0.193758244709321,0.194883602391943),(0.,1.),
 .UNSPECIFIED.)
GEOMETRIC_REPRESENTATION_ITEM()
RATIONAL_B_SPLINE_SURFACE(((1.,0.707106781186548,1.),(1.,0.707106781186548,
1.),(1.,0.707106781186545,1.),(1.,0.707106781186545,1.),(1.,0.707106781186548,
1.),(1.,0.707106781186548,1.),(1.,0.707106781186548,1.),(1.,0.707106781186548,
1.),(1.,0.707106781186548,1.),(1.,0.707106781186548,1.),(1.,0.707106781186548,
1.),(1.,0.707106781186548,1.),(1.,0.707106781186548,1.),(1.,0.707106781186548,
1.),(1.,0.707106781186548,1.),(1.,0.707106781186548,1.),(1.,0.707106781186548,
1.),(1.,0.707106781186548,1.),(1.,0.707106781186548,1.),(1.,0.707106781186548,
1.),(1.,0.707106781186548,1.),(1.,0.707106781186548,1.),(1.,0.707106781186548,
1.),(1.,0.707106781186548,1.),(1.,0.707106781186547,1.),(1.,0.707106781186547,
1.),(1.,0.707106781186548,1.),(1.,0.707106781186548,1.),(1.,0.707106781186548,
1.),(1.,0.707106781186548,1.),(1.,0.707106781186548,1.),(1.,0.707106781186548,
1.)))
REPRESENTATION_ITEM('')
SURFACE()
);
#547=(
BOUNDED_SURFACE()
B_SPLINE_SURFACE(3,2,((#18939,#18940,#18941),(#18942,#18943,#18944),(#18945,
#18946,#18947),(#18948,#18949,#18950),(#18951,#18952,#18953),(#18954,#18955,
#18956),(#18957,#18958,#18959),(#18960,#18961,#18962),(#18963,#18964,#18965),
(#18966,#18967,#18968),(#18969,#18970,#18971),(#18972,#18973,#18974),(#18975,
#18976,#18977),(#18978,#18979,#18980),(#18981,#18982,#18983),(#18984,#18985,
#18986),(#18987,#18988,#18989),(#18990,#18991,#18992),(#18993,#18994,#18995),
(#18996,#18997,#18998),(#18999,#19000,#19001),(#19002,#19003,#19004),(#19005,
#19006,#19007),(#19008,#19009,#19010),(#19011,#19012,#19013),(#19014,#19015,
#19016),(#19017,#19018,#19019),(#19020,#19021,#19022),(#19023,#19024,#19025),
(#19026,#19027,#19028),(#19029,#19030,#19031),(#19032,#19033,#19034),(#19035,
#19036,#19037),(#19038,#19039,#19040),(#19041,#19042,#19043),(#19044,#19045,
#19046)),.UNSPECIFIED.,.F.,.F.,.F.)
B_SPLINE_SURFACE_WITH_KNOTS((4,2,2,2,2,2,2,2,2,2,2,2,2,2,2,2,2,4),(3,3),
(0.0129986978937602,0.0141248636966938,0.0152510294996274,0.0175033611054947,
0.0220080243172292,0.0265126875289637,0.0310173507406982,0.0400266771641672,
0.0490360035876362,0.0580453300111053,0.0670546564345743,0.0760639828580433,
0.0850733092815123,0.10309196212845,0.121110614975388,0.130119941398857,
0.139129267822326,0.157147920669264),(0.,1.),.UNSPECIFIED.)
GEOMETRIC_REPRESENTATION_ITEM()
RATIONAL_B_SPLINE_SURFACE(((1.,0.707106781186547,1.),(1.,0.707106781186547,
1.),(1.,0.707106781186548,1.),(1.,0.707106781186548,1.),(1.,0.707106781186548,
1.),(1.,0.707106781186548,1.),(1.,0.707106781186548,1.),(1.,0.707106781186548,
1.),(1.,0.707106781186548,1.),(1.,0.707106781186548,1.),(1.,0.707106781186548,
1.),(1.,0.707106781186548,1.),(1.,0.707106781186548,1.),(1.,0.707106781186548,
1.),(1.,0.707106781186548,1.),(1.,0.707106781186548,1.),(1.,0.707106781186548,
1.),(1.,0.707106781186548,1.),(1.,0.707106781186548,1.),(1.,0.707106781186548,
1.),(1.,0.707106781186548,1.),(1.,0.707106781186548,1.),(1.,0.707106781186548,
1.),(1.,0.707106781186548,1.),(1.,0.707106781186548,1.),(1.,0.707106781186548,
1.),(1.,0.707106781186548,1.),(1.,0.707106781186548,1.),(1.,0.707106781186549,
1.),(1.,0.707106781186549,1.),(1.,0.70710678118655,1.),(1.,0.70710678118655,
1.),(1.,0.707106781186551,1.),(1.,0.707106781186551,1.),(1.,0.707106781186548,
1.),(1.,0.707106781186548,1.)))
REPRESENTATION_ITEM('')
SURFACE()
);
#548=(
BOUNDED_SURFACE()
B_SPLINE_SURFACE(3,2,((#19271,#19272,#19273),(#19274,#19275,#19276),(#19277,
#19278,#19279),(#19280,#19281,#19282)),.UNSPECIFIED.,.F.,.F.,.F.)
B_SPLINE_SURFACE_WITH_KNOTS((4,4),(3,3),(0.0508378190163745,0.0512849497020778),
(0.0741100254049076,1.),.UNSPECIFIED.)
GEOMETRIC_REPRESENTATION_ITEM()
RATIONAL_B_SPLINE_SURFACE(((0.959804664655073,0.728813105073738,1.),(0.959804664655073,
0.728813105073738,1.),(0.959804664655073,0.728813105073736,1.),(0.959804664655073,
0.728813105073736,1.)))
REPRESENTATION_ITEM('')
SURFACE()
);
#549=(
BOUNDED_SURFACE()
B_SPLINE_SURFACE(3,2,((#19857,#19858,#19859),(#19860,#19861,#19862),(#19863,
#19864,#19865),(#19866,#19867,#19868)),.UNSPECIFIED.,.F.,.F.,.F.)
B_SPLINE_SURFACE_WITH_KNOTS((4,4),(3,3),(1.47451495458029E-17,6.21085125745449E-5),
(0.,1.),.UNSPECIFIED.)
GEOMETRIC_REPRESENTATION_ITEM()
RATIONAL_B_SPLINE_SURFACE(((1.,0.707106781186542,1.),(1.,0.710100066656328,
1.),(1.,0.713076333427087,1.),(1.,0.716036186282139,1.)))
REPRESENTATION_ITEM('')
SURFACE()
);
#550=(
BOUNDED_SURFACE()
B_SPLINE_SURFACE(3,2,((#19870,#19871,#19872),(#19873,#19874,#19875),(#19876,
#19877,#19878),(#19879,#19880,#19881),(#19882,#19883,#19884),(#19885,#19886,
#19887),(#19888,#19889,#19890),(#19891,#19892,#19893)),.UNSPECIFIED.,.F.,
 .F.,.F.)
B_SPLINE_SURFACE_WITH_KNOTS((4,2,2,4),(3,3),(0.00527160002528868,0.00580803552825251,
0.00634447103121634,0.00741734203714401),(0.,1.),.UNSPECIFIED.)
GEOMETRIC_REPRESENTATION_ITEM()
RATIONAL_B_SPLINE_SURFACE(((1.,0.951613498173813,1.),(1.,0.937509881703587,
1.),(1.,0.921891319389384,1.),(1.,0.887932805313032,1.),(1.,0.869471948377235,
1.),(1.,0.810569928220315,1.),(1.,0.766682605321705,1.),(1.,0.716036186282147,
1.)))
REPRESENTATION_ITEM('')
SURFACE()
);
#551=(
BOUNDED_SURFACE()
B_SPLINE_SURFACE(3,2,((#19895,#19896,#19897),(#19898,#19899,#19900),(#19901,
#19902,#19903),(#19904,#19905,#19906),(#19907,#19908,#19909),(#19910,#19911,
#19912)),.UNSPECIFIED.,.F.,.F.,.F.)
B_SPLINE_SURFACE_WITH_KNOTS((4,2,4),(3,3),(-2.60208521396521E-17,0.00181589083224653,
0.00363178166449308),(0.,1.),.UNSPECIFIED.)
GEOMETRIC_REPRESENTATION_ITEM()
RATIONAL_B_SPLINE_SURFACE(((1.,0.951613498173813,1.),(1.,0.954339600494346,
1.),(1.,0.956942012490788,1.),(1.,0.961426637855616,1.),(1.,0.963309297483902,
1.),(1.,0.964515574250421,1.)))
REPRESENTATION_ITEM('')
SURFACE()
);
#552=(
BOUNDED_SURFACE()
B_SPLINE_SURFACE(3,2,((#19913,#19914,#19915),(#19916,#19917,#19918),(#19919,
#19920,#19921),(#19922,#19923,#19924)),.UNSPECIFIED.,.F.,.F.,.F.)
B_SPLINE_SURFACE_WITH_KNOTS((4,4),(3,3),(1.24954300378954E-17,6.21085125745808E-5),
(0.,1.),.UNSPECIFIED.)
GEOMETRIC_REPRESENTATION_ITEM()
RATIONAL_B_SPLINE_SURFACE(((1.,0.707106781186542,1.),(1.,0.710100066656337,
1.),(1.,0.713076333427082,1.),(1.,0.716036186282145,1.)))
REPRESENTATION_ITEM('')
SURFACE()
);
#553=(
BOUNDED_SURFACE()
B_SPLINE_SURFACE(3,2,((#19926,#19927,#19928),(#19929,#19930,#19931),(#19932,
#19933,#19934),(#19935,#19936,#19937),(#19938,#19939,#19940),(#19941,#19942,
#19943),(#19944,#19945,#19946),(#19947,#19948,#19949)),.UNSPECIFIED.,.F.,
 .F.,.F.)
B_SPLINE_SURFACE_WITH_KNOTS((4,2,2,4),(3,3),(0.00527160002528845,0.00580803552825226,
0.00634447103121607,0.00741734203714369),(0.,1.),.UNSPECIFIED.)
GEOMETRIC_REPRESENTATION_ITEM()
RATIONAL_B_SPLINE_SURFACE(((1.,0.951613498173813,1.),(1.,0.937509881703887,
1.),(1.,0.921891319388982,1.),(1.,0.887932805313441,1.),(1.,0.869471948377343,
1.),(1.,0.810569928220099,1.),(1.,0.766682605321886,1.),(1.,0.716036186282151,
1.)))
REPRESENTATION_ITEM('')
SURFACE()
);
#554=(
BOUNDED_SURFACE()
B_SPLINE_SURFACE(3,2,((#19951,#19952,#19953),(#19954,#19955,#19956),(#19957,
#19958,#19959),(#19960,#19961,#19962),(#19963,#19964,#19965),(#19966,#19967,
#19968)),.UNSPECIFIED.,.F.,.F.,.F.)
B_SPLINE_SURFACE_WITH_KNOTS((4,2,4),(3,3),(-8.67361737988404E-18,0.00181589083224649,
0.00363178166449298),(0.,1.),.UNSPECIFIED.)
GEOMETRIC_REPRESENTATION_ITEM()
RATIONAL_B_SPLINE_SURFACE(((1.,0.951613498173814,1.),(1.,0.954339600494444,
1.),(1.,0.956942012490655,1.),(1.,0.961426637855752,1.),(1.,0.963309297483799,
1.),(1.,0.96451557425042,1.)))
REPRESENTATION_ITEM('')
SURFACE()
);
#555=(
BOUNDED_SURFACE()
B_SPLINE_SURFACE(3,2,((#20003,#20004,#20005),(#20006,#20007,#20008),(#20009,
#20010,#20011),(#20012,#20013,#20014),(#20015,#20016,#20017),(#20018,#20019,
#20020),(#20021,#20022,#20023),(#20024,#20025,#20026),(#20027,#20028,#20029),
(#20030,#20031,#20032),(#20033,#20034,#20035),(#20036,#20037,#20038),(#20039,
#20040,#20041),(#20042,#20043,#20044),(#20045,#20046,#20047),(#20048,#20049,
#20050)),.UNSPECIFIED.,.F.,.F.,.F.)
B_SPLINE_SURFACE_WITH_KNOTS((4,2,2,2,2,2,2,4),(3,3),(-9.54097911787244E-18,
0.000696349442505511,0.00139269888501103,0.00208904832751655,0.00278539777002207,
0.00348174721252759,0.00417809665503312,0.00557079554004416),(0.,1.),
 .UNSPECIFIED.)
GEOMETRIC_REPRESENTATION_ITEM()
RATIONAL_B_SPLINE_SURFACE(((1.,0.607054112111757,1.),(1.,0.607056484530443,
1.),(1.,0.607765985148788,1.),(1.,0.610539233834522,1.),(1.,0.612638008520617,
1.),(1.,0.618035047876937,1.),(1.,0.621317782228222,1.),(1.,0.628996523516187,
1.),(1.,0.633392405889998,1.),(1.,0.642875366219237,1.),(1.,0.648018732602713,
1.),(1.,0.658994978794232,1.),(1.,0.664685207841264,1.),(1.,0.682298653549566,
1.),(1.,0.69487665462171,1.),(1.,0.707106781186348,1.)))
REPRESENTATION_ITEM('')
SURFACE()
);
#556=(
BOUNDED_SURFACE()
B_SPLINE_SURFACE(3,2,((#20054,#20055,#20056),(#20057,#20058,#20059),(#20060,
#20061,#20062),(#20063,#20064,#20065),(#20066,#20067,#20068),(#20069,#20070,
#20071),(#20072,#20073,#20074),(#20075,#20076,#20077),(#20078,#20079,#20080),
(#20081,#20082,#20083),(#20084,#20085,#20086),(#20087,#20088,#20089),(#20090,
#20091,#20092),(#20093,#20094,#20095),(#20096,#20097,#20098),(#20099,#20100,
#20101),(#20102,#20103,#20104),(#20105,#20106,#20107)),.UNSPECIFIED.,.F.,
 .F.,.F.)
B_SPLINE_SURFACE_WITH_KNOTS((4,2,2,2,2,2,2,2,4),(3,3),(4.55364912443912E-18,
0.000696359701744999,0.00139271940348999,0.00208907910523499,0.00278543880697998,
0.00348179850872497,0.00417815821046997,0.00487451791221496,0.00557087761395996),
(0.,1.),.UNSPECIFIED.)
GEOMETRIC_REPRESENTATION_ITEM()
RATIONAL_B_SPLINE_SURFACE(((1.,0.707106781186528,1.),(1.,0.700938621263621,
1.),(1.,0.694814107318537,1.),(1.,0.682647727308077,1.),(1.,0.676551634194648,
1.),(1.,0.664717932169144,1.),(1.,0.659039302098822,1.),(1.,0.648178638212686,
1.),(1.,0.642945691912101,1.),(1.,0.633426835507387,1.),(1.,0.629110758092159,
1.),(1.,0.621426182814592,1.),(1.,0.618064223074675,1.),(1.,0.612677785681965,
1.),(1.,0.61060178483004,1.),(1.,0.607773091248028,1.),(1.,0.607052269837757,
1.),(1.,0.607054112111752,1.)))
REPRESENTATION_ITEM('')
SURFACE()
);
#557=(
BOUNDED_SURFACE()
B_SPLINE_SURFACE(1,2,((#20118,#20119,#20120,#20121,#20122,#20123,#20124,
#20125,#20126,#20127,#20128,#20129,#20130,#20131,#20132,#20133,#20134,#20135,
#20136,#20137,#20138,#20139,#20140,#20141,#20142,#20143,#20144,#20145,#20146,
#20147,#20148,#20149,#20150,#20151,#20152,#20153,#20154,#20155,#20156,#20157,
#20158,#20159,#20160,#20161,#20162,#20163,#20164,#20165,#20166,#20167,#20168,
#20169,#20170,#20171,#20172,#20173,#20174,#20175,#20176,#20177,#20178,#20179,
#20180,#20181,#20182,#20183,#20184,#20185,#20186,#20187,#20188,#20189,#20190,
#20191,#20192,#20193,#20194,#20195,#20196,#20197,#20198,#20199,#20200,#20201,
#20202,#20203,#20204,#20205,#20206,#20207,#20208,#20209,#20210,#20211,#20212,
#20213,#20214,#20215,#20216,#20217,#20218,#20219,#20220,#20221,#20222,#20223,
#20224,#20225,#20226,#20227,#20228,#20229,#20230,#20231,#20232,#20233,#20234,
#20235,#20236,#20237,#20238,#20239,#20240,#20241,#20242,#20243,#20244,#20245,
#20246,#20247,#20248,#20249,#20250,#20251,#20252,#20253,#20254,#20255,#20256,
#20257,#20258,#20259,#20260,#20261,#20262,#20263,#20264,#20265,#20266,#20267,
#20268,#20269,#20270,#20271,#20272,#20273,#20274,#20275,#20276,#20277,#20278),
(#20279,#20280,#20281,#20282,#20283,#20284,#20285,#20286,#20287,#20288,
#20289,#20290,#20291,#20292,#20293,#20294,#20295,#20296,#20297,#20298,#20299,
#20300,#20301,#20302,#20303,#20304,#20305,#20306,#20307,#20308,#20309,#20310,
#20311,#20312,#20313,#20314,#20315,#20316,#20317,#20318,#20319,#20320,#20321,
#20322,#20323,#20324,#20325,#20326,#20327,#20328,#20329,#20330,#20331,#20332,
#20333,#20334,#20335,#20336,#20337,#20338,#20339,#20340,#20341,#20342,#20343,
#20344,#20345,#20346,#20347,#20348,#20349,#20350,#20351,#20352,#20353,#20354,
#20355,#20356,#20357,#20358,#20359,#20360,#20361,#20362,#20363,#20364,#20365,
#20366,#20367,#20368,#20369,#20370,#20371,#20372,#20373,#20374,#20375,#20376,
#20377,#20378,#20379,#20380,#20381,#20382,#20383,#20384,#20385,#20386,#20387,
#20388,#20389,#20390,#20391,#20392,#20393,#20394,#20395,#20396,#20397,#20398,
#20399,#20400,#20401,#20402,#20403,#20404,#20405,#20406,#20407,#20408,#20409,
#20410,#20411,#20412,#20413,#20414,#20415,#20416,#20417,#20418,#20419,#20420,
#20421,#20422,#20423,#20424,#20425,#20426,#20427,#20428,#20429,#20430,#20431,
#20432,#20433,#20434,#20435,#20436,#20437,#20438,#20439)),.UNSPECIFIED.,
 .F.,.F.,.F.)
B_SPLINE_SURFACE_WITH_KNOTS((2,2),(3,2,2,2,2,2,2,2,2,2,2,2,2,2,2,2,2,2,
2,2,2,2,2,2,2,2,2,2,2,2,2,2,2,2,2,2,2,2,2,2,2,2,2,2,2,2,2,2,2,2,2,2,2,2,
2,2,2,2,2,2,2,2,2,2,2,2,2,2,2,2,2,2,2,2,2,2,2,2,2,2,3),(0.,1.),(0.,0.0125,
0.025,0.0375,0.05,0.0625,0.075,0.0875,0.1,0.1125,0.125,0.1375,0.15,0.1625,
0.175,0.1875,0.2,0.2125,0.225,0.2375,0.25,0.2625,0.275,0.2875,0.3,0.3125,
0.325,0.3375,0.35,0.3625,0.375,0.3875,0.4,0.4125,0.425,0.4375,0.45,0.4625,
0.475,0.4875,0.5,0.5125,0.525,0.5375,0.55,0.5625,0.575,0.5875,0.6,0.6125,
0.625,0.6375,0.65,0.6625,0.675,0.6875,0.7,0.7125,0.725,0.7375,0.75,0.7625,
0.775,0.7875,0.8,0.8125,0.825,0.8375,0.85,0.8625,0.875,0.8875,0.9,0.9125,
0.925,0.9375,0.95,0.9625,0.975,0.9875,1.),.UNSPECIFIED.)
GEOMETRIC_REPRESENTATION_ITEM()
RATIONAL_B_SPLINE_SURFACE(((1.,0.923879532511287,1.,0.923879532511287,1.,
0.923879532511287,1.,0.923879532511287,1.,0.923879532511287,1.,0.923879532511287,
1.,0.923879532511287,1.,0.923879532511287,1.,0.923879532511287,1.,0.923879532511287,
1.,0.923879532511287,1.,0.923879532511287,1.,0.923879532511287,1.,0.923879532511287,
1.,0.923879532511287,1.,0.923879532511287,1.,0.923879532511287,1.,0.923879532511287,
1.,0.923879532511287,1.,0.923879532511287,1.,0.923879532511287,1.,0.923879532511287,
1.,0.923879532511287,1.,0.923879532511287,1.,0.923879532511287,1.,0.923879532511287,
1.,0.923879532511287,1.,0.923879532511287,1.,0.923879532511287,1.,0.923879532511287,
1.,0.923879532511287,1.,0.923879532511287,1.,0.923879532511287,1.,0.923879532511287,
1.,0.923879532511287,1.,0.923879532511287,1.,0.923879532511287,1.,0.923879532511287,
1.,0.923879532511287,1.,0.923879532511287,1.,0.923879532511287,1.,0.923879532511287,
1.,0.923879532511287,1.,0.923879532511287,1.,0.923879532511287,1.,0.923879532511287,
1.,0.923879532511287,1.,0.923879532511287,1.,0.923879532511287,1.,0.923879532511287,
1.,0.923879532511287,1.,0.923879532511287,1.,0.923879532511287,1.,0.923879532511287,
1.,0.923879532511287,1.,0.923879532511287,1.,0.923879532511287,1.,0.923879532511287,
1.,0.923879532511287,1.,0.923879532511287,1.,0.923879532511287,1.,0.923879532511287,
1.,0.923879532511287,1.,0.923879532511287,1.,0.923879532511287,1.,0.923879532511287,
1.,0.923879532511287,1.,0.923879532511287,1.,0.923879532511287,1.,0.923879532511287,
1.,0.923879532511287,1.,0.923879532511287,1.,0.923879532511287,1.,0.923879532511287,
1.,0.923879532511287,1.,0.923879532511287,1.,0.923879532511287,1.,0.923879532511287,
1.,0.923879532511287,1.,0.923879532511287,1.),(1.,0.923879532511287,1.,
0.923879532511287,1.,0.923879532511287,1.,0.923879532511287,1.,0.923879532511287,
1.,0.923879532511287,1.,0.923879532511287,1.,0.923879532511287,1.,0.923879532511287,
1.,0.923879532511287,1.,0.923879532511287,1.,0.923879532511287,1.,0.923879532511287,
1.,0.923879532511287,1.,0.923879532511287,1.,0.923879532511287,1.,0.923879532511287,
1.,0.923879532511287,1.,0.923879532511287,1.,0.923879532511287,1.,0.923879532511287,
1.,0.923879532511287,1.,0.923879532511287,1.,0.923879532511287,1.,0.923879532511287,
1.,0.923879532511287,1.,0.923879532511287,1.,0.923879532511287,1.,0.923879532511287,
1.,0.923879532511287,1.,0.923879532511287,1.,0.923879532511287,1.,0.923879532511287,
1.,0.923879532511287,1.,0.923879532511287,1.,0.923879532511287,1.,0.923879532511287,
1.,0.923879532511287,1.,0.923879532511287,1.,0.923879532511287,1.,0.923879532511287,
1.,0.923879532511287,1.,0.923879532511287,1.,0.923879532511287,1.,0.923879532511287,
1.,0.923879532511287,1.,0.923879532511287,1.,0.923879532511287,1.,0.923879532511287,
1.,0.923879532511287,1.,0.923879532511287,1.,0.923879532511287,1.,0.923879532511287,
1.,0.923879532511287,1.,0.923879532511287,1.,0.923879532511287,1.,0.923879532511287,
1.,0.923879532511287,1.,0.923879532511287,1.,0.923879532511287,1.,0.923879532511287,
1.,0.923879532511287,1.,0.923879532511287,1.,0.923879532511287,1.,0.923879532511287,
1.,0.923879532511287,1.,0.923879532511287,1.,0.923879532511287,1.,0.923879532511287,
1.,0.923879532511287,1.,0.923879532511287,1.,0.923879532511287,1.,0.923879532511287,
1.,0.923879532511287,1.,0.923879532511287,1.,0.923879532511287,1.,0.923879532511287,
1.,0.923879532511287,1.,0.923879532511287,1.,0.923879532511287,1.)))
REPRESENTATION_ITEM('')
SURFACE()
);
#558=(
BOUNDED_SURFACE()
B_SPLINE_SURFACE(1,2,((#20455,#20456,#20457,#20458,#20459,#20460,#20461,
#20462,#20463,#20464,#20465,#20466,#20467,#20468,#20469,#20470,#20471,#20472,
#20473,#20474,#20475,#20476,#20477,#20478,#20479,#20480,#20481,#20482,#20483,
#20484,#20485,#20486,#20487,#20488,#20489,#20490,#20491,#20492,#20493,#20494,
#20495,#20496,#20497,#20498,#20499,#20500,#20501,#20502,#20503,#20504,#20505,
#20506,#20507,#20508,#20509,#20510,#20511,#20512,#20513,#20514,#20515,#20516,
#20517,#20518,#20519,#20520,#20521,#20522,#20523,#20524,#20525,#20526,#20527,
#20528,#20529,#20530,#20531,#20532,#20533,#20534,#20535,#20536,#20537,#20538,
#20539,#20540,#20541,#20542,#20543,#20544,#20545,#20546,#20547,#20548,#20549,
#20550,#20551,#20552,#20553,#20554,#20555,#20556,#20557,#20558,#20559,#20560,
#20561,#20562,#20563,#20564,#20565,#20566,#20567,#20568,#20569,#20570,#20571,
#20572,#20573,#20574,#20575,#20576,#20577,#20578,#20579,#20580,#20581,#20582,
#20583,#20584,#20585,#20586,#20587,#20588,#20589,#20590,#20591,#20592,#20593,
#20594,#20595,#20596,#20597,#20598,#20599,#20600,#20601,#20602,#20603,#20604,
#20605,#20606,#20607,#20608,#20609,#20610,#20611,#20612,#20613,#20614,#20615),
(#20616,#20617,#20618,#20619,#20620,#20621,#20622,#20623,#20624,#20625,
#20626,#20627,#20628,#20629,#20630,#20631,#20632,#20633,#20634,#20635,#20636,
#20637,#20638,#20639,#20640,#20641,#20642,#20643,#20644,#20645,#20646,#20647,
#20648,#20649,#20650,#20651,#20652,#20653,#20654,#20655,#20656,#20657,#20658,
#20659,#20660,#20661,#20662,#20663,#20664,#20665,#20666,#20667,#20668,#20669,
#20670,#20671,#20672,#20673,#20674,#20675,#20676,#20677,#20678,#20679,#20680,
#20681,#20682,#20683,#20684,#20685,#20686,#20687,#20688,#20689,#20690,#20691,
#20692,#20693,#20694,#20695,#20696,#20697,#20698,#20699,#20700,#20701,#20702,
#20703,#20704,#20705,#20706,#20707,#20708,#20709,#20710,#20711,#20712,#20713,
#20714,#20715,#20716,#20717,#20718,#20719,#20720,#20721,#20722,#20723,#20724,
#20725,#20726,#20727,#20728,#20729,#20730,#20731,#20732,#20733,#20734,#20735,
#20736,#20737,#20738,#20739,#20740,#20741,#20742,#20743,#20744,#20745,#20746,
#20747,#20748,#20749,#20750,#20751,#20752,#20753,#20754,#20755,#20756,#20757,
#20758,#20759,#20760,#20761,#20762,#20763,#20764,#20765,#20766,#20767,#20768,
#20769,#20770,#20771,#20772,#20773,#20774,#20775,#20776)),.UNSPECIFIED.,
 .F.,.F.,.F.)
B_SPLINE_SURFACE_WITH_KNOTS((2,2),(3,2,2,2,2,2,2,2,2,2,2,2,2,2,2,2,2,2,
2,2,2,2,2,2,2,2,2,2,2,2,2,2,2,2,2,2,2,2,2,2,2,2,2,2,2,2,2,2,2,2,2,2,2,2,
2,2,2,2,2,2,2,2,2,2,2,2,2,2,2,2,2,2,2,2,2,2,2,2,2,2,3),(0.,1.),(0.,0.0125,
0.025,0.0375,0.05,0.0625,0.075,0.0875,0.1,0.1125,0.125,0.1375,0.15,0.1625,
0.175,0.1875,0.2,0.2125,0.225,0.2375,0.25,0.2625,0.275,0.2875,0.3,0.3125,
0.325,0.3375,0.35,0.3625,0.375,0.3875,0.4,0.4125,0.425,0.4375,0.45,0.4625,
0.475,0.4875,0.5,0.5125,0.525,0.5375,0.55,0.5625,0.575,0.5875,0.6,0.6125,
0.625,0.6375,0.65,0.6625,0.675,0.6875,0.7,0.7125,0.725,0.7375,0.75,0.7625,
0.775,0.7875,0.8,0.8125,0.825,0.8375,0.85,0.8625,0.875,0.8875,0.9,0.9125,
0.925,0.9375,0.95,0.9625,0.975,0.9875,1.),.UNSPECIFIED.)
GEOMETRIC_REPRESENTATION_ITEM()
RATIONAL_B_SPLINE_SURFACE(((1.,0.923879532511287,1.,0.923879532511287,1.,
0.923879532511287,1.,0.923879532511287,1.,0.923879532511287,1.,0.923879532511287,
1.,0.923879532511287,1.,0.923879532511287,1.,0.923879532511287,1.,0.923879532511287,
1.,0.923879532511287,1.,0.923879532511287,1.,0.923879532511287,1.,0.923879532511287,
1.,0.923879532511287,1.,0.923879532511287,1.,0.923879532511287,1.,0.923879532511287,
1.,0.923879532511287,1.,0.923879532511287,1.,0.923879532511287,1.,0.923879532511287,
1.,0.923879532511287,1.,0.923879532511287,1.,0.923879532511287,1.,0.923879532511287,
1.,0.923879532511287,1.,0.923879532511287,1.,0.923879532511287,1.,0.923879532511287,
1.,0.923879532511287,1.,0.923879532511287,1.,0.923879532511287,1.,0.923879532511287,
1.,0.923879532511287,1.,0.923879532511287,1.,0.923879532511287,1.,0.923879532511287,
1.,0.923879532511287,1.,0.923879532511287,1.,0.923879532511287,1.,0.923879532511287,
1.,0.923879532511287,1.,0.923879532511287,1.,0.923879532511287,1.,0.923879532511287,
1.,0.923879532511287,1.,0.923879532511287,1.,0.923879532511287,1.,0.923879532511287,
1.,0.923879532511287,1.,0.923879532511287,1.,0.923879532511287,1.,0.923879532511287,
1.,0.923879532511287,1.,0.923879532511287,1.,0.923879532511287,1.,0.923879532511287,
1.,0.923879532511287,1.,0.923879532511287,1.,0.923879532511287,1.,0.923879532511287,
1.,0.923879532511287,1.,0.923879532511287,1.,0.923879532511287,1.,0.923879532511287,
1.,0.923879532511287,1.,0.923879532511287,1.,0.923879532511287,1.,0.923879532511287,
1.,0.923879532511287,1.,0.923879532511287,1.,0.923879532511287,1.,0.923879532511287,
1.,0.923879532511287,1.,0.923879532511287,1.,0.923879532511287,1.,0.923879532511287,
1.,0.923879532511287,1.,0.923879532511287,1.),(1.,0.923879532511287,1.,
0.923879532511287,1.,0.923879532511287,1.,0.923879532511287,1.,0.923879532511287,
1.,0.923879532511287,1.,0.923879532511287,1.,0.923879532511287,1.,0.923879532511287,
1.,0.923879532511287,1.,0.923879532511287,1.,0.923879532511287,1.,0.923879532511287,
1.,0.923879532511287,1.,0.923879532511287,1.,0.923879532511287,1.,0.923879532511287,
1.,0.923879532511287,1.,0.923879532511287,1.,0.923879532511287,1.,0.923879532511287,
1.,0.923879532511287,1.,0.923879532511287,1.,0.923879532511287,1.,0.923879532511287,
1.,0.923879532511287,1.,0.923879532511287,1.,0.923879532511287,1.,0.923879532511287,
1.,0.923879532511287,1.,0.923879532511287,1.,0.923879532511287,1.,0.923879532511287,
1.,0.923879532511287,1.,0.923879532511287,1.,0.923879532511287,1.,0.923879532511287,
1.,0.923879532511287,1.,0.923879532511287,1.,0.923879532511287,1.,0.923879532511287,
1.,0.923879532511287,1.,0.923879532511287,1.,0.923879532511287,1.,0.923879532511287,
1.,0.923879532511287,1.,0.923879532511287,1.,0.923879532511287,1.,0.923879532511287,
1.,0.923879532511287,1.,0.923879532511287,1.,0.923879532511287,1.,0.923879532511287,
1.,0.923879532511287,1.,0.923879532511287,1.,0.923879532511287,1.,0.923879532511287,
1.,0.923879532511287,1.,0.923879532511287,1.,0.923879532511287,1.,0.923879532511287,
1.,0.923879532511287,1.,0.923879532511287,1.,0.923879532511287,1.,0.923879532511287,
1.,0.923879532511287,1.,0.923879532511287,1.,0.923879532511287,1.,0.923879532511287,
1.,0.923879532511287,1.,0.923879532511287,1.,0.923879532511287,1.,0.923879532511287,
1.,0.923879532511287,1.,0.923879532511287,1.,0.923879532511287,1.,0.923879532511287,
1.,0.923879532511287,1.,0.923879532511287,1.,0.923879532511287,1.)))
REPRESENTATION_ITEM('')
SURFACE()
);
#559=(
BOUNDED_SURFACE()
B_SPLINE_SURFACE(3,2,((#20786,#20787,#20788,#20789,#20790,#20791,#20792,
#20793,#20794,#20795,#20796,#20797,#20798,#20799,#20800,#20801,#20802,#20803,
#20804,#20805,#20806,#20807,#20808,#20809,#20810,#20811,#20812,#20813,#20814,
#20815,#20816,#20817,#20818,#20819,#20820,#20821,#20822,#20823,#20824,#20825,
#20826,#20827,#20828,#20829,#20830,#20831,#20832,#20833,#20834,#20835,#20836,
#20837,#20838,#20839,#20840,#20841,#20842,#20843,#20844,#20845,#20846,#20847,
#20848,#20849,#20850,#20851,#20852,#20853,#20854,#20855,#20856,#20857,#20858,
#20859,#20860,#20861,#20862,#20863,#20864,#20865,#20866,#20867,#20868,#20869,
#20870,#20871,#20872,#20873,#20874,#20875,#20876,#20877,#20878,#20879,#20880,
#20881,#20882,#20883,#20884,#20885,#20886,#20887,#20888,#20889,#20890,#20891,
#20892,#20893,#20894,#20895,#20896,#20897,#20898,#20899,#20900,#20901,#20902,
#20903,#20904,#20905,#20906,#20907,#20908,#20909,#20910,#20911,#20912,#20913,
#20914,#20915,#20916,#20917,#20918,#20919,#20920,#20921,#20922,#20923,#20924,
#20925,#20926,#20927,#20928,#20929,#20930,#20931,#20932,#20933,#20934,#20935,
#20936,#20937,#20938,#20939,#20940,#20941,#20942,#20943,#20944,#20945,#20946),
(#20947,#20948,#20949,#20950,#20951,#20952,#20953,#20954,#20955,#20956,
#20957,#20958,#20959,#20960,#20961,#20962,#20963,#20964,#20965,#20966,#20967,
#20968,#20969,#20970,#20971,#20972,#20973,#20974,#20975,#20976,#20977,#20978,
#20979,#20980,#20981,#20982,#20983,#20984,#20985,#20986,#20987,#20988,#20989,
#20990,#20991,#20992,#20993,#20994,#20995,#20996,#20997,#20998,#20999,#21000,
#21001,#21002,#21003,#21004,#21005,#21006,#21007,#21008,#21009,#21010,#21011,
#21012,#21013,#21014,#21015,#21016,#21017,#21018,#21019,#21020,#21021,#21022,
#21023,#21024,#21025,#21026,#21027,#21028,#21029,#21030,#21031,#21032,#21033,
#21034,#21035,#21036,#21037,#21038,#21039,#21040,#21041,#21042,#21043,#21044,
#21045,#21046,#21047,#21048,#21049,#21050,#21051,#21052,#21053,#21054,#21055,
#21056,#21057,#21058,#21059,#21060,#21061,#21062,#21063,#21064,#21065,#21066,
#21067,#21068,#21069,#21070,#21071,#21072,#21073,#21074,#21075,#21076,#21077,
#21078,#21079,#21080,#21081,#21082,#21083,#21084,#21085,#21086,#21087,#21088,
#21089,#21090,#21091,#21092,#21093,#21094,#21095,#21096,#21097,#21098,#21099,
#21100,#21101,#21102,#21103,#21104,#21105,#21106,#21107),(#21108,#21109,
#21110,#21111,#21112,#21113,#21114,#21115,#21116,#21117,#21118,#21119,#21120,
#21121,#21122,#21123,#21124,#21125,#21126,#21127,#21128,#21129,#21130,#21131,
#21132,#21133,#21134,#21135,#21136,#21137,#21138,#21139,#21140,#21141,#21142,
#21143,#21144,#21145,#21146,#21147,#21148,#21149,#21150,#21151,#21152,#21153,
#21154,#21155,#21156,#21157,#21158,#21159,#21160,#21161,#21162,#21163,#21164,
#21165,#21166,#21167,#21168,#21169,#21170,#21171,#21172,#21173,#21174,#21175,
#21176,#21177,#21178,#21179,#21180,#21181,#21182,#21183,#21184,#21185,#21186,
#21187,#21188,#21189,#21190,#21191,#21192,#21193,#21194,#21195,#21196,#21197,
#21198,#21199,#21200,#21201,#21202,#21203,#21204,#21205,#21206,#21207,#21208,
#21209,#21210,#21211,#21212,#21213,#21214,#21215,#21216,#21217,#21218,#21219,
#21220,#21221,#21222,#21223,#21224,#21225,#21226,#21227,#21228,#21229,#21230,
#21231,#21232,#21233,#21234,#21235,#21236,#21237,#21238,#21239,#21240,#21241,
#21242,#21243,#21244,#21245,#21246,#21247,#21248,#21249,#21250,#21251,#21252,
#21253,#21254,#21255,#21256,#21257,#21258,#21259,#21260,#21261,#21262,#21263,
#21264,#21265,#21266,#21267,#21268),(#21269,#21270,#21271,#21272,#21273,
#21274,#21275,#21276,#21277,#21278,#21279,#21280,#21281,#21282,#21283,#21284,
#21285,#21286,#21287,#21288,#21289,#21290,#21291,#21292,#21293,#21294,#21295,
#21296,#21297,#21298,#21299,#21300,#21301,#21302,#21303,#21304,#21305,#21306,
#21307,#21308,#21309,#21310,#21311,#21312,#21313,#21314,#21315,#21316,#21317,
#21318,#21319,#21320,#21321,#21322,#21323,#21324,#21325,#21326,#21327,#21328,
#21329,#21330,#21331,#21332,#21333,#21334,#21335,#21336,#21337,#21338,#21339,
#21340,#21341,#21342,#21343,#21344,#21345,#21346,#21347,#21348,#21349,#21350,
#21351,#21352,#21353,#21354,#21355,#21356,#21357,#21358,#21359,#21360,#21361,
#21362,#21363,#21364,#21365,#21366,#21367,#21368,#21369,#21370,#21371,#21372,
#21373,#21374,#21375,#21376,#21377,#21378,#21379,#21380,#21381,#21382,#21383,
#21384,#21385,#21386,#21387,#21388,#21389,#21390,#21391,#21392,#21393,#21394,
#21395,#21396,#21397,#21398,#21399,#21400,#21401,#21402,#21403,#21404,#21405,
#21406,#21407,#21408,#21409,#21410,#21411,#21412,#21413,#21414,#21415,#21416,
#21417,#21418,#21419,#21420,#21421,#21422,#21423,#21424,#21425,#21426,#21427,
#21428,#21429)),.UNSPECIFIED.,.F.,.F.,.F.)
B_SPLINE_SURFACE_WITH_KNOTS((4,4),(3,2,2,2,2,2,2,2,2,2,2,2,2,2,2,2,2,2,
2,2,2,2,2,2,2,2,2,2,2,2,2,2,2,2,2,2,2,2,2,2,2,2,2,2,2,2,2,2,2,2,2,2,2,2,
2,2,2,2,2,2,2,2,2,2,2,2,2,2,2,2,2,2,2,2,2,2,2,2,2,2,3),(0.,1.),(0.,0.0125,
0.025,0.0375,0.05,0.0625,0.075,0.0875,0.1,0.1125,0.125,0.1375,0.15,0.1625,
0.175,0.1875,0.2,0.2125,0.225,0.2375,0.25,0.2625,0.275,0.2875,0.3,0.3125,
0.325,0.3375,0.35,0.3625,0.375,0.3875,0.4,0.4125,0.425,0.4375,0.45,0.4625,
0.475,0.4875,0.5,0.5125,0.525,0.5375,0.55,0.5625,0.575,0.5875,0.6,0.6125,
0.625,0.6375,0.65,0.6625,0.675,0.6875,0.7,0.7125,0.725,0.7375,0.75,0.7625,
0.775,0.7875,0.8,0.8125,0.825,0.8375,0.85,0.8625,0.875,0.8875,0.9,0.9125,
0.925,0.9375,0.95,0.9625,0.975,0.9875,1.),.UNSPECIFIED.)
GEOMETRIC_REPRESENTATION_ITEM()
RATIONAL_B_SPLINE_SURFACE(((1.,0.923879532511287,1.,0.923879532511287,1.,
0.923879532511287,1.,0.923879532511287,1.,0.923879532511287,1.,0.923879532511287,
1.,0.923879532511287,1.,0.923879532511287,1.,0.923879532511287,1.,0.923879532511287,
1.,0.923879532511287,1.,0.923879532511287,1.,0.923879532511287,1.,0.923879532511287,
1.,0.923879532511287,1.,0.923879532511287,1.,0.923879532511287,1.,0.923879532511287,
1.,0.923879532511287,1.,0.923879532511287,1.,0.923879532511287,1.,0.923879532511287,
1.,0.923879532511287,1.,0.923879532511287,1.,0.923879532511287,1.,0.923879532511287,
1.,0.923879532511287,1.,0.923879532511287,1.,0.923879532511287,1.,0.923879532511287,
1.,0.923879532511287,1.,0.923879532511287,1.,0.923879532511287,1.,0.923879532511287,
1.,0.923879532511287,1.,0.923879532511287,1.,0.923879532511287,1.,0.923879532511287,
1.,0.923879532511287,1.,0.923879532511287,1.,0.923879532511287,1.,0.923879532511287,
1.,0.923879532511287,1.,0.923879532511287,1.,0.923879532511287,1.,0.923879532511287,
1.,0.923879532511287,1.,0.923879532511287,1.,0.923879532511287,1.,0.923879532511287,
1.,0.923879532511287,1.,0.923879532511287,1.,0.923879532511287,1.,0.923879532511287,
1.,0.923879532511287,1.,0.923879532511287,1.,0.923879532511287,1.,0.923879532511287,
1.,0.923879532511287,1.,0.923879532511287,1.,0.923879532511287,1.,0.923879532511287,
1.,0.923879532511287,1.,0.923879532511287,1.,0.923879532511287,1.,0.923879532511287,
1.,0.923879532511287,1.,0.923879532511287,1.,0.923879532511287,1.,0.923879532511287,
1.,0.923879532511287,1.,0.923879532511287,1.,0.923879532511287,1.,0.923879532511287,
1.,0.923879532511287,1.,0.923879532511287,1.,0.923879532511287,1.,0.923879532511287,
1.,0.923879532511287,1.,0.923879532511287,1.),(0.998696642611305,0.922675387296324,
0.998696642611305,0.922675387296324,0.998696642611305,0.922675387296324,
0.998696642611305,0.922675387296324,0.998696642611305,0.922675387296324,
0.998696642611305,0.922675387296324,0.998696642611305,0.922675387296324,
0.998696642611305,0.922675387296324,0.998696642611305,0.922675387296324,
0.998696642611305,0.922675387296324,0.998696642611305,0.922675387296324,
0.998696642611305,0.922675387296324,0.998696642611305,0.922675387296324,
0.998696642611305,0.922675387296324,0.998696642611305,0.922675387296324,
0.998696642611305,0.922675387296324,0.998696642611305,0.922675387296324,
0.998696642611305,0.922675387296324,0.998696642611305,0.922675387296324,
0.998696642611305,0.922675387296324,0.998696642611305,0.922675387296324,
0.998696642611305,0.922675387296324,0.998696642611305,0.922675387296324,
0.998696642611305,0.922675387296324,0.998696642611305,0.922675387296324,
0.998696642611305,0.922675387296324,0.998696642611305,0.922675387296324,
0.998696642611305,0.922675387296324,0.998696642611305,0.922675387296324,
0.998696642611305,0.922675387296324,0.998696642611305,0.922675387296324,
0.998696642611305,0.922675387296324,0.998696642611305,0.922675387296324,
0.998696642611305,0.922675387296324,0.998696642611305,0.922675387296324,
0.998696642611305,0.922675387296324,0.998696642611305,0.922675387296324,
0.998696642611305,0.922675387296324,0.998696642611305,0.922675387296324,
0.998696642611305,0.922675387296324,0.998696642611305,0.922675387296324,
0.998696642611305,0.922675387296324,0.998696642611305,0.922675387296324,
0.998696642611305,0.922675387296324,0.998696642611305,0.922675387296324,
0.998696642611305,0.922675387296324,0.998696642611305,0.922675387296324,
0.998696642611305,0.922675387296324,0.998696642611305,0.922675387296324,
0.998696642611305,0.922675387296324,0.998696642611305,0.922675387296324,
0.998696642611305,0.922675387296324,0.998696642611305,0.922675387296324,
0.998696642611305,0.922675387296324,0.998696642611305,0.922675387296324,
0.998696642611305,0.922675387296324,0.998696642611305,0.922675387296324,
0.998696642611305,0.922675387296324,0.998696642611305,0.922675387296324,
0.998696642611305,0.922675387296324,0.998696642611305,0.922675387296324,
0.998696642611305,0.922675387296324,0.998696642611305,0.922675387296324,
0.998696642611305,0.922675387296324,0.998696642611305,0.922675387296324,
0.998696642611305,0.922675387296324,0.998696642611305,0.922675387296324,
0.998696642611305,0.922675387296324,0.998696642611305,0.922675387296324,
0.998696642611305,0.922675387296324,0.998696642611305,0.922675387296324,
0.998696642611305,0.922675387296324,0.998696642611305,0.922675387296324,
0.998696642611305,0.922675387296324,0.998696642611305,0.922675387296324,
0.998696642611305,0.922675387296324,0.998696642611305,0.922675387296324,
0.998696642611305,0.922675387296324,0.998696642611305,0.922675387296324,
0.998696642611305,0.922675387296324,0.998696642611305),(0.998696642611305,
0.922675387296324,0.998696642611305,0.922675387296324,0.998696642611305,
0.922675387296324,0.998696642611305,0.922675387296324,0.998696642611305,
0.922675387296324,0.998696642611305,0.922675387296324,0.998696642611305,
0.922675387296324,0.998696642611305,0.922675387296324,0.998696642611305,
0.922675387296324,0.998696642611305,0.922675387296324,0.998696642611305,
0.922675387296324,0.998696642611305,0.922675387296324,0.998696642611305,
0.922675387296324,0.998696642611305,0.922675387296324,0.998696642611305,
0.922675387296324,0.998696642611305,0.922675387296324,0.998696642611305,
0.922675387296324,0.998696642611305,0.922675387296324,0.998696642611305,
0.922675387296324,0.998696642611305,0.922675387296324,0.998696642611305,
0.922675387296324,0.998696642611305,0.922675387296324,0.998696642611305,
0.922675387296324,0.998696642611305,0.922675387296324,0.998696642611305,
0.922675387296324,0.998696642611305,0.922675387296324,0.998696642611305,
0.922675387296324,0.998696642611305,0.922675387296324,0.998696642611305,
0.922675387296324,0.998696642611305,0.922675387296324,0.998696642611305,
0.922675387296324,0.998696642611305,0.922675387296324,0.998696642611305,
0.922675387296324,0.998696642611305,0.922675387296324,0.998696642611305,
0.922675387296324,0.998696642611305,0.922675387296324,0.998696642611305,
0.922675387296324,0.998696642611305,0.922675387296324,0.998696642611305,
0.922675387296324,0.998696642611305,0.922675387296324,0.998696642611305,
0.922675387296324,0.998696642611305,0.922675387296324,0.998696642611305,
0.922675387296324,0.998696642611305,0.922675387296324,0.998696642611305,
0.922675387296324,0.998696642611305,0.922675387296324,0.998696642611305,
0.922675387296324,0.998696642611305,0.922675387296324,0.998696642611305,
0.922675387296324,0.998696642611305,0.922675387296324,0.998696642611305,
0.922675387296324,0.998696642611305,0.922675387296324,0.998696642611305,
0.922675387296324,0.998696642611305,0.922675387296324,0.998696642611305,
0.922675387296324,0.998696642611305,0.922675387296324,0.998696642611305,
0.922675387296324,0.998696642611305,0.922675387296324,0.998696642611305,
0.922675387296324,0.998696642611305,0.922675387296324,0.998696642611305,
0.922675387296324,0.998696642611305,0.922675387296324,0.998696642611305,
0.922675387296324,0.998696642611305,0.922675387296324,0.998696642611305,
0.922675387296324,0.998696642611305,0.922675387296324,0.998696642611305,
0.922675387296324,0.998696642611305,0.922675387296324,0.998696642611305,
0.922675387296324,0.998696642611305,0.922675387296324,0.998696642611305,
0.922675387296324,0.998696642611305,0.922675387296324,0.998696642611305,
0.922675387296324,0.998696642611305,0.922675387296324,0.998696642611305,
0.922675387296324,0.998696642611305,0.922675387296324,0.998696642611305,
0.922675387296324,0.998696642611305,0.922675387296324,0.998696642611305,
0.922675387296324,0.998696642611305,0.922675387296324,0.998696642611305),
(1.,0.923879532511287,1.,0.923879532511287,1.,0.923879532511287,1.,0.923879532511287,
1.,0.923879532511287,1.,0.923879532511287,1.,0.923879532511287,1.,0.923879532511287,
1.,0.923879532511287,1.,0.923879532511287,1.,0.923879532511287,1.,0.923879532511287,
1.,0.923879532511287,1.,0.923879532511287,1.,0.923879532511287,1.,0.923879532511287,
1.,0.923879532511287,1.,0.923879532511287,1.,0.923879532511287,1.,0.923879532511287,
1.,0.923879532511287,1.,0.923879532511287,1.,0.923879532511287,1.,0.923879532511287,
1.,0.923879532511287,1.,0.923879532511287,1.,0.923879532511287,1.,0.923879532511287,
1.,0.923879532511287,1.,0.923879532511287,1.,0.923879532511287,1.,0.923879532511287,
1.,0.923879532511287,1.,0.923879532511287,1.,0.923879532511287,1.,0.923879532511287,
1.,0.923879532511287,1.,0.923879532511287,1.,0.923879532511287,1.,0.923879532511287,
1.,0.923879532511287,1.,0.923879532511287,1.,0.923879532511287,1.,0.923879532511287,
1.,0.923879532511287,1.,0.923879532511287,1.,0.923879532511287,1.,0.923879532511287,
1.,0.923879532511287,1.,0.923879532511287,1.,0.923879532511287,1.,0.923879532511287,
1.,0.923879532511287,1.,0.923879532511287,1.,0.923879532511287,1.,0.923879532511287,
1.,0.923879532511287,1.,0.923879532511287,1.,0.923879532511287,1.,0.923879532511287,
1.,0.923879532511287,1.,0.923879532511287,1.,0.923879532511287,1.,0.923879532511287,
1.,0.923879532511287,1.,0.923879532511287,1.,0.923879532511287,1.,0.923879532511287,
1.,0.923879532511287,1.,0.923879532511287,1.,0.923879532511287,1.,0.923879532511287,
1.,0.923879532511287,1.,0.923879532511287,1.,0.923879532511287,1.,0.923879532511287,
1.,0.923879532511287,1.,0.923879532511287,1.,0.923879532511287,1.,0.923879532511287,
1.)))
REPRESENTATION_ITEM('')
SURFACE()
);
#560=(
BOUNDED_SURFACE()
B_SPLINE_SURFACE(3,2,((#21430,#21431,#21432,#21433,#21434,#21435,#21436,
#21437,#21438,#21439,#21440,#21441,#21442,#21443,#21444,#21445,#21446,#21447,
#21448,#21449,#21450,#21451,#21452,#21453,#21454,#21455,#21456,#21457,#21458,
#21459,#21460,#21461,#21462,#21463,#21464,#21465,#21466,#21467,#21468,#21469,
#21470,#21471,#21472,#21473,#21474,#21475,#21476,#21477,#21478,#21479,#21480,
#21481,#21482,#21483,#21484,#21485,#21486,#21487,#21488,#21489,#21490,#21491,
#21492,#21493,#21494,#21495,#21496,#21497,#21498,#21499,#21500,#21501,#21502,
#21503,#21504,#21505,#21506,#21507,#21508,#21509,#21510,#21511,#21512,#21513,
#21514,#21515,#21516,#21517,#21518,#21519,#21520,#21521,#21522,#21523,#21524,
#21525,#21526,#21527,#21528,#21529,#21530,#21531,#21532,#21533,#21534,#21535,
#21536,#21537,#21538,#21539,#21540,#21541,#21542,#21543,#21544,#21545,#21546,
#21547,#21548,#21549,#21550,#21551,#21552,#21553,#21554,#21555,#21556,#21557,
#21558,#21559,#21560,#21561,#21562,#21563,#21564,#21565,#21566,#21567,#21568,
#21569,#21570,#21571,#21572,#21573,#21574,#21575,#21576,#21577,#21578,#21579,
#21580,#21581,#21582,#21583,#21584,#21585,#21586,#21587,#21588,#21589,#21590),
(#21591,#21592,#21593,#21594,#21595,#21596,#21597,#21598,#21599,#21600,
#21601,#21602,#21603,#21604,#21605,#21606,#21607,#21608,#21609,#21610,#21611,
#21612,#21613,#21614,#21615,#21616,#21617,#21618,#21619,#21620,#21621,#21622,
#21623,#21624,#21625,#21626,#21627,#21628,#21629,#21630,#21631,#21632,#21633,
#21634,#21635,#21636,#21637,#21638,#21639,#21640,#21641,#21642,#21643,#21644,
#21645,#21646,#21647,#21648,#21649,#21650,#21651,#21652,#21653,#21654,#21655,
#21656,#21657,#21658,#21659,#21660,#21661,#21662,#21663,#21664,#21665,#21666,
#21667,#21668,#21669,#21670,#21671,#21672,#21673,#21674,#21675,#21676,#21677,
#21678,#21679,#21680,#21681,#21682,#21683,#21684,#21685,#21686,#21687,#21688,
#21689,#21690,#21691,#21692,#21693,#21694,#21695,#21696,#21697,#21698,#21699,
#21700,#21701,#21702,#21703,#21704,#21705,#21706,#21707,#21708,#21709,#21710,
#21711,#21712,#21713,#21714,#21715,#21716,#21717,#21718,#21719,#21720,#21721,
#21722,#21723,#21724,#21725,#21726,#21727,#21728,#21729,#21730,#21731,#21732,
#21733,#21734,#21735,#21736,#21737,#21738,#21739,#21740,#21741,#21742,#21743,
#21744,#21745,#21746,#21747,#21748,#21749,#21750,#21751),(#21752,#21753,
#21754,#21755,#21756,#21757,#21758,#21759,#21760,#21761,#21762,#21763,#21764,
#21765,#21766,#21767,#21768,#21769,#21770,#21771,#21772,#21773,#21774,#21775,
#21776,#21777,#21778,#21779,#21780,#21781,#21782,#21783,#21784,#21785,#21786,
#21787,#21788,#21789,#21790,#21791,#21792,#21793,#21794,#21795,#21796,#21797,
#21798,#21799,#21800,#21801,#21802,#21803,#21804,#21805,#21806,#21807,#21808,
#21809,#21810,#21811,#21812,#21813,#21814,#21815,#21816,#21817,#21818,#21819,
#21820,#21821,#21822,#21823,#21824,#21825,#21826,#21827,#21828,#21829,#21830,
#21831,#21832,#21833,#21834,#21835,#21836,#21837,#21838,#21839,#21840,#21841,
#21842,#21843,#21844,#21845,#21846,#21847,#21848,#21849,#21850,#21851,#21852,
#21853,#21854,#21855,#21856,#21857,#21858,#21859,#21860,#21861,#21862,#21863,
#21864,#21865,#21866,#21867,#21868,#21869,#21870,#21871,#21872,#21873,#21874,
#21875,#21876,#21877,#21878,#21879,#21880,#21881,#21882,#21883,#21884,#21885,
#21886,#21887,#21888,#21889,#21890,#21891,#21892,#21893,#21894,#21895,#21896,
#21897,#21898,#21899,#21900,#21901,#21902,#21903,#21904,#21905,#21906,#21907,
#21908,#21909,#21910,#21911,#21912),(#21913,#21914,#21915,#21916,#21917,
#21918,#21919,#21920,#21921,#21922,#21923,#21924,#21925,#21926,#21927,#21928,
#21929,#21930,#21931,#21932,#21933,#21934,#21935,#21936,#21937,#21938,#21939,
#21940,#21941,#21942,#21943,#21944,#21945,#21946,#21947,#21948,#21949,#21950,
#21951,#21952,#21953,#21954,#21955,#21956,#21957,#21958,#21959,#21960,#21961,
#21962,#21963,#21964,#21965,#21966,#21967,#21968,#21969,#21970,#21971,#21972,
#21973,#21974,#21975,#21976,#21977,#21978,#21979,#21980,#21981,#21982,#21983,
#21984,#21985,#21986,#21987,#21988,#21989,#21990,#21991,#21992,#21993,#21994,
#21995,#21996,#21997,#21998,#21999,#22000,#22001,#22002,#22003,#22004,#22005,
#22006,#22007,#22008,#22009,#22010,#22011,#22012,#22013,#22014,#22015,#22016,
#22017,#22018,#22019,#22020,#22021,#22022,#22023,#22024,#22025,#22026,#22027,
#22028,#22029,#22030,#22031,#22032,#22033,#22034,#22035,#22036,#22037,#22038,
#22039,#22040,#22041,#22042,#22043,#22044,#22045,#22046,#22047,#22048,#22049,
#22050,#22051,#22052,#22053,#22054,#22055,#22056,#22057,#22058,#22059,#22060,
#22061,#22062,#22063,#22064,#22065,#22066,#22067,#22068,#22069,#22070,#22071,
#22072,#22073)),.UNSPECIFIED.,.F.,.F.,.F.)
B_SPLINE_SURFACE_WITH_KNOTS((4,4),(3,2,2,2,2,2,2,2,2,2,2,2,2,2,2,2,2,2,
2,2,2,2,2,2,2,2,2,2,2,2,2,2,2,2,2,2,2,2,2,2,2,2,2,2,2,2,2,2,2,2,2,2,2,2,
2,2,2,2,2,2,2,2,2,2,2,2,2,2,2,2,2,2,2,2,2,2,2,2,2,2,3),(0.,1.00288579446161),
(0.,0.0125,0.025,0.0375,0.05,0.0625,0.075,0.0875,0.1,0.1125,0.125,0.1375,
0.15,0.1625,0.175,0.1875,0.2,0.2125,0.225,0.2375,0.25,0.2625,0.275,0.2875,
0.3,0.3125,0.325,0.3375,0.35,0.3625,0.375,0.3875,0.4,0.4125,0.425,0.4375,
0.45,0.4625,0.475,0.4875,0.5,0.5125,0.525,0.5375,0.55,0.5625,0.575,0.5875,
0.6,0.6125,0.625,0.6375,0.65,0.6625,0.675,0.6875,0.7,0.7125,0.725,0.7375,
0.75,0.7625,0.775,0.7875,0.8,0.8125,0.825,0.8375,0.85,0.8625,0.875,0.8875,
0.9,0.9125,0.925,0.9375,0.95,0.9625,0.975,0.9875,1.00288579446161),
 .UNSPECIFIED.)
GEOMETRIC_REPRESENTATION_ITEM()
RATIONAL_B_SPLINE_SURFACE(((1.,0.923879532511287,1.,0.923879532511287,1.,
0.923879532511287,1.,0.923879532511287,1.,0.923879532511287,1.,0.923879532511287,
1.,0.923879532511287,1.,0.923879532511287,1.,0.923879532511287,1.,0.923879532511287,
1.,0.923879532511287,1.,0.923879532511287,1.,0.923879532511287,1.,0.923879532511287,
1.,0.923879532511287,1.,0.923879532511287,1.,0.923879532511287,1.,0.923879532511287,
1.,0.923879532511287,1.,0.923879532511287,1.,0.923879532511287,1.,0.923879532511287,
1.,0.923879532511287,1.,0.923879532511287,1.,0.923879532511287,1.,0.923879532511287,
1.,0.923879532511287,1.,0.923879532511287,1.,0.923879532511287,1.,0.923879532511287,
1.,0.923879532511287,1.,0.923879532511287,1.,0.923879532511287,1.,0.923879532511287,
1.,0.923879532511287,1.,0.923879532511287,1.,0.923879532511287,1.,0.923879532511287,
1.,0.923879532511287,1.,0.923879532511287,1.,0.923879532511287,1.,0.923879532511287,
1.,0.923879532511287,1.,0.923879532511287,1.,0.923879532511287,1.,0.923879532511287,
1.,0.923879532511287,1.,0.923879532511287,1.,0.923879532511287,1.,0.923879532511287,
1.,0.923879532511287,1.,0.923879532511287,1.,0.923879532511287,1.,0.923879532511287,
1.,0.923879532511287,1.,0.923879532511287,1.,0.923879532511287,1.,0.923879532511287,
1.,0.923879532511287,1.,0.923879532511287,1.,0.923879532511287,1.,0.923879532511287,
1.,0.923879532511287,1.,0.923879532511287,1.,0.923879532511287,1.,0.923879532511287,
1.,0.923879532511287,1.,0.923879532511287,1.,0.923879532511287,1.,0.923879532511287,
1.,0.923879532511287,1.,0.923879532511287,1.,0.923879532511287,1.,0.923879532511287,
1.,0.923879532511287,1.,0.923879532511287,1.,0.923879532511287,1.,0.923879532511287,
1.,0.923879532511287,1.,0.90630609063176,1.04326101835863),(0.998692881389771,
0.922671912380731,0.998692881389771,0.922671912380731,0.998692881389771,
0.922671912380731,0.998692881389771,0.922671912380731,0.998692881389771,
0.922671912380731,0.998692881389771,0.922671912380731,0.998692881389771,
0.922671912380731,0.998692881389771,0.922671912380731,0.998692881389771,
0.922671912380731,0.998692881389771,0.922671912380731,0.998692881389771,
0.922671912380731,0.998692881389771,0.922671912380731,0.998692881389771,
0.922671912380731,0.998692881389771,0.922671912380731,0.998692881389771,
0.922671912380731,0.998692881389771,0.922671912380731,0.998692881389771,
0.922671912380731,0.998692881389771,0.922671912380731,0.998692881389771,
0.922671912380731,0.998692881389771,0.922671912380731,0.998692881389771,
0.922671912380731,0.998692881389771,0.922671912380731,0.998692881389771,
0.922671912380731,0.998692881389771,0.922671912380731,0.998692881389771,
0.922671912380731,0.998692881389771,0.922671912380731,0.998692881389771,
0.922671912380731,0.998692881389771,0.922671912380731,0.998692881389771,
0.922671912380731,0.998692881389771,0.922671912380731,0.998692881389771,
0.922671912380731,0.998692881389771,0.922671912380731,0.998692881389771,
0.922671912380731,0.998692881389771,0.922671912380731,0.998692881389771,
0.922671912380731,0.998692881389771,0.922671912380731,0.998692881389771,
0.922671912380731,0.998692881389771,0.922671912380731,0.998692881389771,
0.922671912380731,0.998692881389771,0.922671912380731,0.998692881389771,
0.922671912380731,0.998692881389771,0.922671912380731,0.998692881389771,
0.922671912380731,0.998692881389771,0.922671912380731,0.998692881389771,
0.922671912380731,0.998692881389771,0.922671912380731,0.998692881389771,
0.922671912380731,0.998692881389771,0.922671912380731,0.998692881389771,
0.922671912380731,0.998692881389771,0.922671912380731,0.998692881389771,
0.922671912380731,0.998692881389771,0.922671912380731,0.998692881389771,
0.922671912380731,0.998692881389771,0.922671912380731,0.998692881389771,
0.922671912380731,0.998692881389771,0.922671912380731,0.998692881389771,
0.922671912380731,0.998692881389771,0.922671912380731,0.998692881389771,
0.922671912380731,0.998692881389771,0.922671912380731,0.998692881389771,
0.922671912380731,0.998692881389771,0.922671912380731,0.998692881389771,
0.922671912380731,0.998692881389771,0.922671912380731,0.998692881389771,
0.922671912380731,0.998692881389771,0.922671912380731,0.998692881389771,
0.922671912380731,0.998692881389771,0.922671912380731,0.998692881389771,
0.922671912380731,0.998692881389771,0.922671912380731,0.998692881389771,
0.922671912380731,0.998692881389771,0.922671912380731,0.998692881389771,
0.922671912380731,0.998692881389771,0.922671912380731,0.998692881389771,
0.922671912380731,0.998692881389771,0.922671912380731,0.998692881389771,
0.922671912380731,0.998692881389771,0.922671912380731,0.998692881389771,
0.922671912380731,0.998692881389771,0.905121441074131,1.04189735246621),
(0.998696653465417,0.922675397324216,0.998696653465417,0.922675397324216,
0.998696653465417,0.922675397324216,0.998696653465417,0.922675397324216,
0.998696653465417,0.922675397324216,0.998696653465417,0.922675397324216,
0.998696653465417,0.922675397324216,0.998696653465417,0.922675397324216,
0.998696653465417,0.922675397324216,0.998696653465417,0.922675397324216,
0.998696653465417,0.922675397324216,0.998696653465417,0.922675397324216,
0.998696653465417,0.922675397324216,0.998696653465417,0.922675397324216,
0.998696653465417,0.922675397324216,0.998696653465417,0.922675397324216,
0.998696653465417,0.922675397324216,0.998696653465417,0.922675397324216,
0.998696653465417,0.922675397324216,0.998696653465417,0.922675397324216,
0.998696653465417,0.922675397324216,0.998696653465417,0.922675397324216,
0.998696653465417,0.922675397324216,0.998696653465417,0.922675397324216,
0.998696653465417,0.922675397324216,0.998696653465417,0.922675397324216,
0.998696653465417,0.922675397324216,0.998696653465417,0.922675397324216,
0.998696653465417,0.922675397324216,0.998696653465417,0.922675397324216,
0.998696653465417,0.922675397324216,0.998696653465417,0.922675397324216,
0.998696653465417,0.922675397324216,0.998696653465417,0.922675397324216,
0.998696653465417,0.922675397324216,0.998696653465417,0.922675397324216,
0.998696653465417,0.922675397324216,0.998696653465417,0.922675397324216,
0.998696653465417,0.922675397324216,0.998696653465417,0.922675397324216,
0.998696653465417,0.922675397324216,0.998696653465417,0.922675397324216,
0.998696653465417,0.922675397324216,0.998696653465417,0.922675397324216,
0.998696653465417,0.922675397324216,0.998696653465417,0.922675397324216,
0.998696653465417,0.922675397324216,0.998696653465417,0.922675397324216,
0.998696653465417,0.922675397324216,0.998696653465417,0.922675397324216,
0.998696653465417,0.922675397324216,0.998696653465417,0.922675397324216,
0.998696653465417,0.922675397324216,0.998696653465417,0.922675397324216,
0.998696653465417,0.922675397324216,0.998696653465417,0.922675397324216,
0.998696653465417,0.922675397324216,0.998696653465417,0.922675397324216,
0.998696653465417,0.922675397324216,0.998696653465417,0.922675397324216,
0.998696653465417,0.922675397324216,0.998696653465417,0.922675397324216,
0.998696653465417,0.922675397324216,0.998696653465417,0.922675397324216,
0.998696653465417,0.922675397324216,0.998696653465417,0.922675397324216,
0.998696653465417,0.922675397324216,0.998696653465417,0.922675397324216,
0.998696653465417,0.922675397324216,0.998696653465417,0.922675397324216,
0.998696653465417,0.922675397324216,0.998696653465417,0.922675397324216,
0.998696653465417,0.922675397324216,0.998696653465417,0.922675397324216,
0.998696653465417,0.922675397324216,0.998696653465417,0.922675397324216,
0.998696653465417,0.922675397324216,0.998696653465417,0.922675397324216,
0.998696653465417,0.922675397324216,0.998696653465417,0.905124859729264,
1.04190128772569),(1.00001131622694,0.92388998734174,1.00001131622694,0.92388998734174,
1.00001131622694,0.92388998734174,1.00001131622694,0.92388998734174,1.00001131622694,
0.92388998734174,1.00001131622694,0.92388998734174,1.00001131622694,0.92388998734174,
1.00001131622694,0.92388998734174,1.00001131622694,0.92388998734174,1.00001131622694,
0.92388998734174,1.00001131622694,0.92388998734174,1.00001131622694,0.92388998734174,
1.00001131622694,0.92388998734174,1.00001131622694,0.92388998734174,1.00001131622694,
0.92388998734174,1.00001131622694,0.92388998734174,1.00001131622694,0.92388998734174,
1.00001131622694,0.92388998734174,1.00001131622694,0.92388998734174,1.00001131622694,
0.92388998734174,1.00001131622694,0.92388998734174,1.00001131622694,0.92388998734174,
1.00001131622694,0.92388998734174,1.00001131622694,0.92388998734174,1.00001131622694,
0.92388998734174,1.00001131622694,0.92388998734174,1.00001131622694,0.92388998734174,
1.00001131622694,0.92388998734174,1.00001131622694,0.92388998734174,1.00001131622694,
0.92388998734174,1.00001131622694,0.92388998734174,1.00001131622694,0.92388998734174,
1.00001131622694,0.92388998734174,1.00001131622694,0.92388998734174,1.00001131622694,
0.92388998734174,1.00001131622694,0.92388998734174,1.00001131622694,0.92388998734174,
1.00001131622694,0.92388998734174,1.00001131622694,0.92388998734174,1.00001131622694,
0.92388998734174,1.00001131622694,0.92388998734174,1.00001131622694,0.92388998734174,
1.00001131622694,0.92388998734174,1.00001131622694,0.92388998734174,1.00001131622694,
0.92388998734174,1.00001131622694,0.92388998734174,1.00001131622694,0.92388998734174,
1.00001131622694,0.92388998734174,1.00001131622694,0.92388998734174,1.00001131622694,
0.92388998734174,1.00001131622694,0.92388998734174,1.00001131622694,0.92388998734174,
1.00001131622694,0.92388998734174,1.00001131622694,0.92388998734174,1.00001131622694,
0.92388998734174,1.00001131622694,0.92388998734174,1.00001131622694,0.92388998734174,
1.00001131622694,0.92388998734174,1.00001131622694,0.92388998734174,1.00001131622694,
0.92388998734174,1.00001131622694,0.92388998734174,1.00001131622694,0.92388998734174,
1.00001131622694,0.92388998734174,1.00001131622694,0.92388998734174,1.00001131622694,
0.92388998734174,1.00001131622694,0.92388998734174,1.00001131622694,0.92388998734174,
1.00001131622694,0.92388998734174,1.00001131622694,0.92388998734174,1.00001131622694,
0.92388998734174,1.00001131622694,0.92388998734174,1.00001131622694,0.92388998734174,
1.00001131622694,0.92388998734174,1.00001131622694,0.92388998734174,1.00001131622694,
0.92388998734174,1.00001131622694,0.92388998734174,1.00001131622694,0.92388998734174,
1.00001131622694,0.92388998734174,1.00001131622694,0.92388998734174,1.00001131622694,
0.906316346597157,1.04327282413707)))
REPRESENTATION_ITEM('')
SURFACE()
);
#561=(
BOUNDED_SURFACE()
B_SPLINE_SURFACE(3,2,((#22076,#22077,#22078,#22079,#22080,#22081,#22082,
#22083,#22084,#22085,#22086,#22087,#22088,#22089,#22090,#22091,#22092,#22093,
#22094,#22095,#22096,#22097,#22098,#22099,#22100,#22101,#22102,#22103,#22104,
#22105,#22106,#22107,#22108,#22109,#22110,#22111,#22112,#22113,#22114,#22115,
#22116,#22117,#22118,#22119,#22120,#22121,#22122,#22123,#22124,#22125,#22126,
#22127,#22128,#22129,#22130,#22131,#22132,#22133,#22134,#22135,#22136,#22137,
#22138,#22139,#22140,#22141,#22142,#22143,#22144,#22145,#22146,#22147,#22148,
#22149,#22150,#22151,#22152,#22153,#22154,#22155,#22156,#22157,#22158,#22159,
#22160,#22161,#22162,#22163,#22164,#22165,#22166,#22167,#22168,#22169,#22170,
#22171,#22172,#22173,#22174,#22175,#22176,#22177,#22178,#22179,#22180,#22181,
#22182,#22183,#22184,#22185,#22186,#22187,#22188,#22189,#22190,#22191,#22192,
#22193,#22194,#22195,#22196,#22197,#22198,#22199,#22200,#22201,#22202,#22203,
#22204,#22205,#22206,#22207,#22208,#22209,#22210,#22211,#22212,#22213,#22214,
#22215,#22216,#22217,#22218,#22219,#22220,#22221,#22222,#22223,#22224,#22225,
#22226,#22227,#22228,#22229,#22230,#22231,#22232,#22233,#22234,#22235,#22236),
(#22237,#22238,#22239,#22240,#22241,#22242,#22243,#22244,#22245,#22246,
#22247,#22248,#22249,#22250,#22251,#22252,#22253,#22254,#22255,#22256,#22257,
#22258,#22259,#22260,#22261,#22262,#22263,#22264,#22265,#22266,#22267,#22268,
#22269,#22270,#22271,#22272,#22273,#22274,#22275,#22276,#22277,#22278,#22279,
#22280,#22281,#22282,#22283,#22284,#22285,#22286,#22287,#22288,#22289,#22290,
#22291,#22292,#22293,#22294,#22295,#22296,#22297,#22298,#22299,#22300,#22301,
#22302,#22303,#22304,#22305,#22306,#22307,#22308,#22309,#22310,#22311,#22312,
#22313,#22314,#22315,#22316,#22317,#22318,#22319,#22320,#22321,#22322,#22323,
#22324,#22325,#22326,#22327,#22328,#22329,#22330,#22331,#22332,#22333,#22334,
#22335,#22336,#22337,#22338,#22339,#22340,#22341,#22342,#22343,#22344,#22345,
#22346,#22347,#22348,#22349,#22350,#22351,#22352,#22353,#22354,#22355,#22356,
#22357,#22358,#22359,#22360,#22361,#22362,#22363,#22364,#22365,#22366,#22367,
#22368,#22369,#22370,#22371,#22372,#22373,#22374,#22375,#22376,#22377,#22378,
#22379,#22380,#22381,#22382,#22383,#22384,#22385,#22386,#22387,#22388,#22389,
#22390,#22391,#22392,#22393,#22394,#22395,#22396,#22397),(#22398,#22399,
#22400,#22401,#22402,#22403,#22404,#22405,#22406,#22407,#22408,#22409,#22410,
#22411,#22412,#22413,#22414,#22415,#22416,#22417,#22418,#22419,#22420,#22421,
#22422,#22423,#22424,#22425,#22426,#22427,#22428,#22429,#22430,#22431,#22432,
#22433,#22434,#22435,#22436,#22437,#22438,#22439,#22440,#22441,#22442,#22443,
#22444,#22445,#22446,#22447,#22448,#22449,#22450,#22451,#22452,#22453,#22454,
#22455,#22456,#22457,#22458,#22459,#22460,#22461,#22462,#22463,#22464,#22465,
#22466,#22467,#22468,#22469,#22470,#22471,#22472,#22473,#22474,#22475,#22476,
#22477,#22478,#22479,#22480,#22481,#22482,#22483,#22484,#22485,#22486,#22487,
#22488,#22489,#22490,#22491,#22492,#22493,#22494,#22495,#22496,#22497,#22498,
#22499,#22500,#22501,#22502,#22503,#22504,#22505,#22506,#22507,#22508,#22509,
#22510,#22511,#22512,#22513,#22514,#22515,#22516,#22517,#22518,#22519,#22520,
#22521,#22522,#22523,#22524,#22525,#22526,#22527,#22528,#22529,#22530,#22531,
#22532,#22533,#22534,#22535,#22536,#22537,#22538,#22539,#22540,#22541,#22542,
#22543,#22544,#22545,#22546,#22547,#22548,#22549,#22550,#22551,#22552,#22553,
#22554,#22555,#22556,#22557,#22558),(#22559,#22560,#22561,#22562,#22563,
#22564,#22565,#22566,#22567,#22568,#22569,#22570,#22571,#22572,#22573,#22574,
#22575,#22576,#22577,#22578,#22579,#22580,#22581,#22582,#22583,#22584,#22585,
#22586,#22587,#22588,#22589,#22590,#22591,#22592,#22593,#22594,#22595,#22596,
#22597,#22598,#22599,#22600,#22601,#22602,#22603,#22604,#22605,#22606,#22607,
#22608,#22609,#22610,#22611,#22612,#22613,#22614,#22615,#22616,#22617,#22618,
#22619,#22620,#22621,#22622,#22623,#22624,#22625,#22626,#22627,#22628,#22629,
#22630,#22631,#22632,#22633,#22634,#22635,#22636,#22637,#22638,#22639,#22640,
#22641,#22642,#22643,#22644,#22645,#22646,#22647,#22648,#22649,#22650,#22651,
#22652,#22653,#22654,#22655,#22656,#22657,#22658,#22659,#22660,#22661,#22662,
#22663,#22664,#22665,#22666,#22667,#22668,#22669,#22670,#22671,#22672,#22673,
#22674,#22675,#22676,#22677,#22678,#22679,#22680,#22681,#22682,#22683,#22684,
#22685,#22686,#22687,#22688,#22689,#22690,#22691,#22692,#22693,#22694,#22695,
#22696,#22697,#22698,#22699,#22700,#22701,#22702,#22703,#22704,#22705,#22706,
#22707,#22708,#22709,#22710,#22711,#22712,#22713,#22714,#22715,#22716,#22717,
#22718,#22719)),.UNSPECIFIED.,.F.,.F.,.F.)
B_SPLINE_SURFACE_WITH_KNOTS((4,4),(3,2,2,2,2,2,2,2,2,2,2,2,2,2,2,2,2,2,
2,2,2,2,2,2,2,2,2,2,2,2,2,2,2,2,2,2,2,2,2,2,2,2,2,2,2,2,2,2,2,2,2,2,2,2,
2,2,2,2,2,2,2,2,2,2,2,2,2,2,2,2,2,2,2,2,2,2,2,2,2,2,3),(0.,1.),(0.,0.0125,
0.025,0.0375,0.05,0.0625,0.075,0.0875,0.1,0.1125,0.125,0.1375,0.15,0.1625,
0.175,0.1875,0.2,0.2125,0.225,0.2375,0.25,0.2625,0.275,0.2875,0.3,0.3125,
0.325,0.3375,0.35,0.3625,0.375,0.3875,0.4,0.4125,0.425,0.4375,0.45,0.4625,
0.475,0.4875,0.5,0.5125,0.525,0.5375,0.55,0.5625,0.575,0.5875,0.6,0.6125,
0.625,0.6375,0.65,0.6625,0.675,0.6875,0.7,0.7125,0.725,0.7375,0.75,0.7625,
0.775,0.7875,0.8,0.8125,0.825,0.8375,0.85,0.8625,0.875,0.8875,0.9,0.9125,
0.925,0.9375,0.95,0.9625,0.975,0.9875,1.),.UNSPECIFIED.)
GEOMETRIC_REPRESENTATION_ITEM()
RATIONAL_B_SPLINE_SURFACE(((1.,0.923879532511287,1.,0.923879532511287,1.,
0.923879532511287,1.,0.923879532511287,1.,0.923879532511287,1.,0.923879532511287,
1.,0.923879532511287,1.,0.923879532511287,1.,0.923879532511287,1.,0.923879532511287,
1.,0.923879532511287,1.,0.923879532511287,1.,0.923879532511287,1.,0.923879532511287,
1.,0.923879532511287,1.,0.923879532511287,1.,0.923879532511287,1.,0.923879532511287,
1.,0.923879532511287,1.,0.923879532511287,1.,0.923879532511287,1.,0.923879532511287,
1.,0.923879532511287,1.,0.923879532511287,1.,0.923879532511287,1.,0.923879532511287,
1.,0.923879532511287,1.,0.923879532511287,1.,0.923879532511287,1.,0.923879532511287,
1.,0.923879532511287,1.,0.923879532511287,1.,0.923879532511287,1.,0.923879532511287,
1.,0.923879532511287,1.,0.923879532511287,1.,0.923879532511287,1.,0.923879532511287,
1.,0.923879532511287,1.,0.923879532511287,1.,0.923879532511287,1.,0.923879532511287,
1.,0.923879532511287,1.,0.923879532511287,1.,0.923879532511287,1.,0.923879532511287,
1.,0.923879532511287,1.,0.923879532511287,1.,0.923879532511287,1.,0.923879532511287,
1.,0.923879532511287,1.,0.923879532511287,1.,0.923879532511287,1.,0.923879532511287,
1.,0.923879532511287,1.,0.923879532511287,1.,0.923879532511287,1.,0.923879532511287,
1.,0.923879532511287,1.,0.923879532511287,1.,0.923879532511287,1.,0.923879532511287,
1.,0.923879532511287,1.,0.923879532511287,1.,0.923879532511287,1.,0.923879532511287,
1.,0.923879532511287,1.,0.923879532511287,1.,0.923879532511287,1.,0.923879532511287,
1.,0.923879532511287,1.,0.923879532511287,1.,0.923879532511287,1.,0.923879532511287,
1.,0.923879532511287,1.,0.923879532511287,1.,0.923879532511287,1.,0.923879532511287,
1.,0.923879532511287,1.,0.923879532511287,1.),(0.998696642611305,0.922675387296324,
0.998696642611305,0.922675387296324,0.998696642611305,0.922675387296324,
0.998696642611305,0.922675387296324,0.998696642611305,0.922675387296324,
0.998696642611305,0.922675387296324,0.998696642611305,0.922675387296324,
0.998696642611305,0.922675387296324,0.998696642611305,0.922675387296324,
0.998696642611305,0.922675387296324,0.998696642611305,0.922675387296324,
0.998696642611305,0.922675387296324,0.998696642611305,0.922675387296324,
0.998696642611305,0.922675387296324,0.998696642611305,0.922675387296324,
0.998696642611305,0.922675387296324,0.998696642611305,0.922675387296324,
0.998696642611305,0.922675387296324,0.998696642611305,0.922675387296324,
0.998696642611305,0.922675387296324,0.998696642611305,0.922675387296324,
0.998696642611305,0.922675387296324,0.998696642611305,0.922675387296324,
0.998696642611305,0.922675387296324,0.998696642611305,0.922675387296324,
0.998696642611305,0.922675387296324,0.998696642611305,0.922675387296324,
0.998696642611305,0.922675387296324,0.998696642611305,0.922675387296324,
0.998696642611305,0.922675387296324,0.998696642611305,0.922675387296324,
0.998696642611305,0.922675387296324,0.998696642611305,0.922675387296324,
0.998696642611305,0.922675387296324,0.998696642611305,0.922675387296324,
0.998696642611305,0.922675387296324,0.998696642611305,0.922675387296324,
0.998696642611305,0.922675387296324,0.998696642611305,0.922675387296324,
0.998696642611305,0.922675387296324,0.998696642611305,0.922675387296324,
0.998696642611305,0.922675387296324,0.998696642611305,0.922675387296324,
0.998696642611305,0.922675387296324,0.998696642611305,0.922675387296324,
0.998696642611305,0.922675387296324,0.998696642611305,0.922675387296324,
0.998696642611305,0.922675387296324,0.998696642611305,0.922675387296324,
0.998696642611305,0.922675387296324,0.998696642611305,0.922675387296324,
0.998696642611305,0.922675387296324,0.998696642611305,0.922675387296324,
0.998696642611305,0.922675387296324,0.998696642611305,0.922675387296324,
0.998696642611305,0.922675387296324,0.998696642611305,0.922675387296324,
0.998696642611305,0.922675387296324,0.998696642611305,0.922675387296324,
0.998696642611305,0.922675387296324,0.998696642611305,0.922675387296324,
0.998696642611305,0.922675387296324,0.998696642611305,0.922675387296324,
0.998696642611305,0.922675387296324,0.998696642611305,0.922675387296324,
0.998696642611305,0.922675387296324,0.998696642611305,0.922675387296324,
0.998696642611305,0.922675387296324,0.998696642611305,0.922675387296324,
0.998696642611305,0.922675387296324,0.998696642611305,0.922675387296324,
0.998696642611305,0.922675387296324,0.998696642611305,0.922675387296324,
0.998696642611305,0.922675387296324,0.998696642611305,0.922675387296324,
0.998696642611305,0.922675387296324,0.998696642611305,0.922675387296324,
0.998696642611305,0.922675387296324,0.998696642611305,0.922675387296324,
0.998696642611305,0.922675387296324,0.998696642611305),(0.998696642611305,
0.922675387296324,0.998696642611305,0.922675387296324,0.998696642611305,
0.922675387296324,0.998696642611305,0.922675387296324,0.998696642611305,
0.922675387296324,0.998696642611305,0.922675387296324,0.998696642611305,
0.922675387296324,0.998696642611305,0.922675387296324,0.998696642611305,
0.922675387296324,0.998696642611305,0.922675387296324,0.998696642611305,
0.922675387296324,0.998696642611305,0.922675387296324,0.998696642611305,
0.922675387296324,0.998696642611305,0.922675387296324,0.998696642611305,
0.922675387296324,0.998696642611305,0.922675387296324,0.998696642611305,
0.922675387296324,0.998696642611305,0.922675387296324,0.998696642611305,
0.922675387296324,0.998696642611305,0.922675387296324,0.998696642611305,
0.922675387296324,0.998696642611305,0.922675387296324,0.998696642611305,
0.922675387296324,0.998696642611305,0.922675387296324,0.998696642611305,
0.922675387296324,0.998696642611305,0.922675387296324,0.998696642611305,
0.922675387296324,0.998696642611305,0.922675387296324,0.998696642611305,
0.922675387296324,0.998696642611305,0.922675387296324,0.998696642611305,
0.922675387296324,0.998696642611305,0.922675387296324,0.998696642611305,
0.922675387296324,0.998696642611305,0.922675387296324,0.998696642611305,
0.922675387296324,0.998696642611305,0.922675387296324,0.998696642611305,
0.922675387296324,0.998696642611305,0.922675387296324,0.998696642611305,
0.922675387296324,0.998696642611305,0.922675387296324,0.998696642611305,
0.922675387296324,0.998696642611305,0.922675387296324,0.998696642611305,
0.922675387296324,0.998696642611305,0.922675387296324,0.998696642611305,
0.922675387296324,0.998696642611305,0.922675387296324,0.998696642611305,
0.922675387296324,0.998696642611305,0.922675387296324,0.998696642611305,
0.922675387296324,0.998696642611305,0.922675387296324,0.998696642611305,
0.922675387296324,0.998696642611305,0.922675387296324,0.998696642611305,
0.922675387296324,0.998696642611305,0.922675387296324,0.998696642611305,
0.922675387296324,0.998696642611305,0.922675387296324,0.998696642611305,
0.922675387296324,0.998696642611305,0.922675387296324,0.998696642611305,
0.922675387296324,0.998696642611305,0.922675387296324,0.998696642611305,
0.922675387296324,0.998696642611305,0.922675387296324,0.998696642611305,
0.922675387296324,0.998696642611305,0.922675387296324,0.998696642611305,
0.922675387296324,0.998696642611305,0.922675387296324,0.998696642611305,
0.922675387296324,0.998696642611305,0.922675387296324,0.998696642611305,
0.922675387296324,0.998696642611305,0.922675387296324,0.998696642611305,
0.922675387296324,0.998696642611305,0.922675387296324,0.998696642611305,
0.922675387296324,0.998696642611305,0.922675387296324,0.998696642611305,
0.922675387296324,0.998696642611305,0.922675387296324,0.998696642611305,
0.922675387296324,0.998696642611305,0.922675387296324,0.998696642611305,
0.922675387296324,0.998696642611305,0.922675387296324,0.998696642611305),
(1.,0.923879532511287,1.,0.923879532511287,1.,0.923879532511287,1.,0.923879532511287,
1.,0.923879532511287,1.,0.923879532511287,1.,0.923879532511287,1.,0.923879532511287,
1.,0.923879532511287,1.,0.923879532511287,1.,0.923879532511287,1.,0.923879532511287,
1.,0.923879532511287,1.,0.923879532511287,1.,0.923879532511287,1.,0.923879532511287,
1.,0.923879532511287,1.,0.923879532511287,1.,0.923879532511287,1.,0.923879532511287,
1.,0.923879532511287,1.,0.923879532511287,1.,0.923879532511287,1.,0.923879532511287,
1.,0.923879532511287,1.,0.923879532511287,1.,0.923879532511287,1.,0.923879532511287,
1.,0.923879532511287,1.,0.923879532511287,1.,0.923879532511287,1.,0.923879532511287,
1.,0.923879532511287,1.,0.923879532511287,1.,0.923879532511287,1.,0.923879532511287,
1.,0.923879532511287,1.,0.923879532511287,1.,0.923879532511287,1.,0.923879532511287,
1.,0.923879532511287,1.,0.923879532511287,1.,0.923879532511287,1.,0.923879532511287,
1.,0.923879532511287,1.,0.923879532511287,1.,0.923879532511287,1.,0.923879532511287,
1.,0.923879532511287,1.,0.923879532511287,1.,0.923879532511287,1.,0.923879532511287,
1.,0.923879532511287,1.,0.923879532511287,1.,0.923879532511287,1.,0.923879532511287,
1.,0.923879532511287,1.,0.923879532511287,1.,0.923879532511287,1.,0.923879532511287,
1.,0.923879532511287,1.,0.923879532511287,1.,0.923879532511287,1.,0.923879532511287,
1.,0.923879532511287,1.,0.923879532511287,1.,0.923879532511287,1.,0.923879532511287,
1.,0.923879532511287,1.,0.923879532511287,1.,0.923879532511287,1.,0.923879532511287,
1.,0.923879532511287,1.,0.923879532511287,1.,0.923879532511287,1.,0.923879532511287,
1.,0.923879532511287,1.,0.923879532511287,1.,0.923879532511287,1.,0.923879532511287,
1.)))
REPRESENTATION_ITEM('')
SURFACE()
);
#562=(
BOUNDED_SURFACE()
B_SPLINE_SURFACE(3,2,((#22720,#22721,#22722,#22723,#22724,#22725,#22726,
#22727,#22728,#22729,#22730,#22731,#22732,#22733,#22734,#22735,#22736,#22737,
#22738,#22739,#22740,#22741,#22742,#22743,#22744,#22745,#22746,#22747,#22748,
#22749,#22750,#22751,#22752,#22753,#22754,#22755,#22756,#22757,#22758,#22759,
#22760,#22761,#22762,#22763,#22764,#22765,#22766,#22767,#22768,#22769,#22770,
#22771,#22772,#22773,#22774,#22775,#22776,#22777,#22778,#22779,#22780,#22781,
#22782,#22783,#22784,#22785,#22786,#22787,#22788,#22789,#22790,#22791,#22792,
#22793,#22794,#22795,#22796,#22797,#22798,#22799,#22800,#22801,#22802,#22803,
#22804,#22805,#22806,#22807,#22808,#22809,#22810,#22811,#22812,#22813,#22814,
#22815,#22816,#22817,#22818,#22819,#22820,#22821,#22822,#22823,#22824,#22825,
#22826,#22827,#22828,#22829,#22830,#22831,#22832,#22833,#22834,#22835,#22836,
#22837,#22838,#22839,#22840,#22841,#22842,#22843,#22844,#22845,#22846,#22847,
#22848,#22849,#22850,#22851,#22852,#22853,#22854,#22855,#22856,#22857,#22858,
#22859,#22860,#22861,#22862,#22863,#22864,#22865,#22866,#22867,#22868,#22869,
#22870,#22871,#22872,#22873,#22874,#22875,#22876,#22877,#22878,#22879,#22880),
(#22881,#22882,#22883,#22884,#22885,#22886,#22887,#22888,#22889,#22890,
#22891,#22892,#22893,#22894,#22895,#22896,#22897,#22898,#22899,#22900,#22901,
#22902,#22903,#22904,#22905,#22906,#22907,#22908,#22909,#22910,#22911,#22912,
#22913,#22914,#22915,#22916,#22917,#22918,#22919,#22920,#22921,#22922,#22923,
#22924,#22925,#22926,#22927,#22928,#22929,#22930,#22931,#22932,#22933,#22934,
#22935,#22936,#22937,#22938,#22939,#22940,#22941,#22942,#22943,#22944,#22945,
#22946,#22947,#22948,#22949,#22950,#22951,#22952,#22953,#22954,#22955,#22956,
#22957,#22958,#22959,#22960,#22961,#22962,#22963,#22964,#22965,#22966,#22967,
#22968,#22969,#22970,#22971,#22972,#22973,#22974,#22975,#22976,#22977,#22978,
#22979,#22980,#22981,#22982,#22983,#22984,#22985,#22986,#22987,#22988,#22989,
#22990,#22991,#22992,#22993,#22994,#22995,#22996,#22997,#22998,#22999,#23000,
#23001,#23002,#23003,#23004,#23005,#23006,#23007,#23008,#23009,#23010,#23011,
#23012,#23013,#23014,#23015,#23016,#23017,#23018,#23019,#23020,#23021,#23022,
#23023,#23024,#23025,#23026,#23027,#23028,#23029,#23030,#23031,#23032,#23033,
#23034,#23035,#23036,#23037,#23038,#23039,#23040,#23041),(#23042,#23043,
#23044,#23045,#23046,#23047,#23048,#23049,#23050,#23051,#23052,#23053,#23054,
#23055,#23056,#23057,#23058,#23059,#23060,#23061,#23062,#23063,#23064,#23065,
#23066,#23067,#23068,#23069,#23070,#23071,#23072,#23073,#23074,#23075,#23076,
#23077,#23078,#23079,#23080,#23081,#23082,#23083,#23084,#23085,#23086,#23087,
#23088,#23089,#23090,#23091,#23092,#23093,#23094,#23095,#23096,#23097,#23098,
#23099,#23100,#23101,#23102,#23103,#23104,#23105,#23106,#23107,#23108,#23109,
#23110,#23111,#23112,#23113,#23114,#23115,#23116,#23117,#23118,#23119,#23120,
#23121,#23122,#23123,#23124,#23125,#23126,#23127,#23128,#23129,#23130,#23131,
#23132,#23133,#23134,#23135,#23136,#23137,#23138,#23139,#23140,#23141,#23142,
#23143,#23144,#23145,#23146,#23147,#23148,#23149,#23150,#23151,#23152,#23153,
#23154,#23155,#23156,#23157,#23158,#23159,#23160,#23161,#23162,#23163,#23164,
#23165,#23166,#23167,#23168,#23169,#23170,#23171,#23172,#23173,#23174,#23175,
#23176,#23177,#23178,#23179,#23180,#23181,#23182,#23183,#23184,#23185,#23186,
#23187,#23188,#23189,#23190,#23191,#23192,#23193,#23194,#23195,#23196,#23197,
#23198,#23199,#23200,#23201,#23202),(#23203,#23204,#23205,#23206,#23207,
#23208,#23209,#23210,#23211,#23212,#23213,#23214,#23215,#23216,#23217,#23218,
#23219,#23220,#23221,#23222,#23223,#23224,#23225,#23226,#23227,#23228,#23229,
#23230,#23231,#23232,#23233,#23234,#23235,#23236,#23237,#23238,#23239,#23240,
#23241,#23242,#23243,#23244,#23245,#23246,#23247,#23248,#23249,#23250,#23251,
#23252,#23253,#23254,#23255,#23256,#23257,#23258,#23259,#23260,#23261,#23262,
#23263,#23264,#23265,#23266,#23267,#23268,#23269,#23270,#23271,#23272,#23273,
#23274,#23275,#23276,#23277,#23278,#23279,#23280,#23281,#23282,#23283,#23284,
#23285,#23286,#23287,#23288,#23289,#23290,#23291,#23292,#23293,#23294,#23295,
#23296,#23297,#23298,#23299,#23300,#23301,#23302,#23303,#23304,#23305,#23306,
#23307,#23308,#23309,#23310,#23311,#23312,#23313,#23314,#23315,#23316,#23317,
#23318,#23319,#23320,#23321,#23322,#23323,#23324,#23325,#23326,#23327,#23328,
#23329,#23330,#23331,#23332,#23333,#23334,#23335,#23336,#23337,#23338,#23339,
#23340,#23341,#23342,#23343,#23344,#23345,#23346,#23347,#23348,#23349,#23350,
#23351,#23352,#23353,#23354,#23355,#23356,#23357,#23358,#23359,#23360,#23361,
#23362,#23363)),.UNSPECIFIED.,.F.,.F.,.F.)
B_SPLINE_SURFACE_WITH_KNOTS((4,4),(3,2,2,2,2,2,2,2,2,2,2,2,2,2,2,2,2,2,
2,2,2,2,2,2,2,2,2,2,2,2,2,2,2,2,2,2,2,2,2,2,2,2,2,2,2,2,2,2,2,2,2,2,2,2,
2,2,2,2,2,2,2,2,2,2,2,2,2,2,2,2,2,2,2,2,2,2,2,2,2,2,3),(0.,1.),(0.,0.0125,
0.025,0.0375,0.05,0.0625,0.075,0.0875,0.1,0.1125,0.125,0.1375,0.15,0.1625,
0.175,0.1875,0.2,0.2125,0.225,0.2375,0.25,0.2625,0.275,0.2875,0.3,0.3125,
0.325,0.3375,0.35,0.3625,0.375,0.3875,0.4,0.4125,0.425,0.4375,0.45,0.4625,
0.475,0.4875,0.5,0.5125,0.525,0.5375,0.55,0.5625,0.575,0.5875,0.6,0.6125,
0.625,0.6375,0.65,0.6625,0.675,0.6875,0.7,0.7125,0.725,0.7375,0.75,0.7625,
0.775,0.7875,0.8,0.8125,0.825,0.8375,0.85,0.8625,0.875,0.8875,0.9,0.9125,
0.925,0.9375,0.95,0.9625,0.975,0.9875,1.),.UNSPECIFIED.)
GEOMETRIC_REPRESENTATION_ITEM()
RATIONAL_B_SPLINE_SURFACE(((1.,0.923879532511287,1.,0.923879532511287,1.,
0.923879532511287,1.,0.923879532511287,1.,0.923879532511287,1.,0.923879532511287,
1.,0.923879532511287,1.,0.923879532511287,1.,0.923879532511287,1.,0.923879532511287,
1.,0.923879532511287,1.,0.923879532511287,1.,0.923879532511287,1.,0.923879532511287,
1.,0.923879532511287,1.,0.923879532511287,1.,0.923879532511287,1.,0.923879532511287,
1.,0.923879532511287,1.,0.923879532511287,1.,0.923879532511287,1.,0.923879532511287,
1.,0.923879532511287,1.,0.923879532511287,1.,0.923879532511287,1.,0.923879532511287,
1.,0.923879532511287,1.,0.923879532511287,1.,0.923879532511287,1.,0.923879532511287,
1.,0.923879532511287,1.,0.923879532511287,1.,0.923879532511287,1.,0.923879532511287,
1.,0.923879532511287,1.,0.923879532511287,1.,0.923879532511287,1.,0.923879532511287,
1.,0.923879532511287,1.,0.923879532511287,1.,0.923879532511287,1.,0.923879532511287,
1.,0.923879532511287,1.,0.923879532511287,1.,0.923879532511287,1.,0.923879532511287,
1.,0.923879532511287,1.,0.923879532511287,1.,0.923879532511287,1.,0.923879532511287,
1.,0.923879532511287,1.,0.923879532511287,1.,0.923879532511287,1.,0.923879532511287,
1.,0.923879532511287,1.,0.923879532511287,1.,0.923879532511287,1.,0.923879532511287,
1.,0.923879532511287,1.,0.923879532511287,1.,0.923879532511287,1.,0.923879532511287,
1.,0.923879532511287,1.,0.923879532511287,1.,0.923879532511287,1.,0.923879532511287,
1.,0.923879532511287,1.,0.923879532511287,1.,0.923879532511287,1.,0.923879532511287,
1.,0.923879532511287,1.,0.923879532511287,1.,0.923879532511287,1.,0.923879532511287,
1.,0.923879532511287,1.,0.923879532511287,1.,0.923879532511287,1.,0.923879532511287,
1.,0.923879532511287,1.,0.923879532511287,1.),(0.998696642611305,0.922675387296324,
0.998696642611305,0.922675387296324,0.998696642611305,0.922675387296324,
0.998696642611305,0.922675387296324,0.998696642611305,0.922675387296324,
0.998696642611305,0.922675387296324,0.998696642611305,0.922675387296324,
0.998696642611305,0.922675387296324,0.998696642611305,0.922675387296324,
0.998696642611305,0.922675387296324,0.998696642611305,0.922675387296324,
0.998696642611305,0.922675387296324,0.998696642611305,0.922675387296324,
0.998696642611305,0.922675387296324,0.998696642611305,0.922675387296324,
0.998696642611305,0.922675387296324,0.998696642611305,0.922675387296324,
0.998696642611305,0.922675387296324,0.998696642611305,0.922675387296324,
0.998696642611305,0.922675387296324,0.998696642611305,0.922675387296324,
0.998696642611305,0.922675387296324,0.998696642611305,0.922675387296324,
0.998696642611305,0.922675387296324,0.998696642611305,0.922675387296324,
0.998696642611305,0.922675387296324,0.998696642611305,0.922675387296324,
0.998696642611305,0.922675387296324,0.998696642611305,0.922675387296324,
0.998696642611305,0.922675387296324,0.998696642611305,0.922675387296324,
0.998696642611305,0.922675387296324,0.998696642611305,0.922675387296324,
0.998696642611305,0.922675387296324,0.998696642611305,0.922675387296324,
0.998696642611305,0.922675387296324,0.998696642611305,0.922675387296324,
0.998696642611305,0.922675387296324,0.998696642611305,0.922675387296324,
0.998696642611305,0.922675387296324,0.998696642611305,0.922675387296324,
0.998696642611305,0.922675387296324,0.998696642611305,0.922675387296324,
0.998696642611305,0.922675387296324,0.998696642611305,0.922675387296324,
0.998696642611305,0.922675387296324,0.998696642611305,0.922675387296324,
0.998696642611305,0.922675387296324,0.998696642611305,0.922675387296324,
0.998696642611305,0.922675387296324,0.998696642611305,0.922675387296324,
0.998696642611305,0.922675387296324,0.998696642611305,0.922675387296324,
0.998696642611305,0.922675387296324,0.998696642611305,0.922675387296324,
0.998696642611305,0.922675387296324,0.998696642611305,0.922675387296324,
0.998696642611305,0.922675387296324,0.998696642611305,0.922675387296324,
0.998696642611305,0.922675387296324,0.998696642611305,0.922675387296324,
0.998696642611305,0.922675387296324,0.998696642611305,0.922675387296324,
0.998696642611305,0.922675387296324,0.998696642611305,0.922675387296324,
0.998696642611305,0.922675387296324,0.998696642611305,0.922675387296324,
0.998696642611305,0.922675387296324,0.998696642611305,0.922675387296324,
0.998696642611305,0.922675387296324,0.998696642611305,0.922675387296324,
0.998696642611305,0.922675387296324,0.998696642611305,0.922675387296324,
0.998696642611305,0.922675387296324,0.998696642611305,0.922675387296324,
0.998696642611305,0.922675387296324,0.998696642611305,0.922675387296324,
0.998696642611305,0.922675387296324,0.998696642611305,0.922675387296324,
0.998696642611305,0.922675387296324,0.998696642611305),(0.998696642611305,
0.922675387296324,0.998696642611305,0.922675387296324,0.998696642611305,
0.922675387296324,0.998696642611305,0.922675387296324,0.998696642611305,
0.922675387296324,0.998696642611305,0.922675387296324,0.998696642611305,
0.922675387296324,0.998696642611305,0.922675387296324,0.998696642611305,
0.922675387296324,0.998696642611305,0.922675387296324,0.998696642611305,
0.922675387296324,0.998696642611305,0.922675387296324,0.998696642611305,
0.922675387296324,0.998696642611305,0.922675387296324,0.998696642611305,
0.922675387296324,0.998696642611305,0.922675387296324,0.998696642611305,
0.922675387296324,0.998696642611305,0.922675387296324,0.998696642611305,
0.922675387296324,0.998696642611305,0.922675387296324,0.998696642611305,
0.922675387296324,0.998696642611305,0.922675387296324,0.998696642611305,
0.922675387296324,0.998696642611305,0.922675387296324,0.998696642611305,
0.922675387296324,0.998696642611305,0.922675387296324,0.998696642611305,
0.922675387296324,0.998696642611305,0.922675387296324,0.998696642611305,
0.922675387296324,0.998696642611305,0.922675387296324,0.998696642611305,
0.922675387296324,0.998696642611305,0.922675387296324,0.998696642611305,
0.922675387296324,0.998696642611305,0.922675387296324,0.998696642611305,
0.922675387296324,0.998696642611305,0.922675387296324,0.998696642611305,
0.922675387296324,0.998696642611305,0.922675387296324,0.998696642611305,
0.922675387296324,0.998696642611305,0.922675387296324,0.998696642611305,
0.922675387296324,0.998696642611305,0.922675387296324,0.998696642611305,
0.922675387296324,0.998696642611305,0.922675387296324,0.998696642611305,
0.922675387296324,0.998696642611305,0.922675387296324,0.998696642611305,
0.922675387296324,0.998696642611305,0.922675387296324,0.998696642611305,
0.922675387296324,0.998696642611305,0.922675387296324,0.998696642611305,
0.922675387296324,0.998696642611305,0.922675387296324,0.998696642611305,
0.922675387296324,0.998696642611305,0.922675387296324,0.998696642611305,
0.922675387296324,0.998696642611305,0.922675387296324,0.998696642611305,
0.922675387296324,0.998696642611305,0.922675387296324,0.998696642611305,
0.922675387296324,0.998696642611305,0.922675387296324,0.998696642611305,
0.922675387296324,0.998696642611305,0.922675387296324,0.998696642611305,
0.922675387296324,0.998696642611305,0.922675387296324,0.998696642611305,
0.922675387296324,0.998696642611305,0.922675387296324,0.998696642611305,
0.922675387296324,0.998696642611305,0.922675387296324,0.998696642611305,
0.922675387296324,0.998696642611305,0.922675387296324,0.998696642611305,
0.922675387296324,0.998696642611305,0.922675387296324,0.998696642611305,
0.922675387296324,0.998696642611305,0.922675387296324,0.998696642611305,
0.922675387296324,0.998696642611305,0.922675387296324,0.998696642611305,
0.922675387296324,0.998696642611305,0.922675387296324,0.998696642611305,
0.922675387296324,0.998696642611305,0.922675387296324,0.998696642611305),
(1.,0.923879532511287,1.,0.923879532511287,1.,0.923879532511287,1.,0.923879532511287,
1.,0.923879532511287,1.,0.923879532511287,1.,0.923879532511287,1.,0.923879532511287,
1.,0.923879532511287,1.,0.923879532511287,1.,0.923879532511287,1.,0.923879532511287,
1.,0.923879532511287,1.,0.923879532511287,1.,0.923879532511287,1.,0.923879532511287,
1.,0.923879532511287,1.,0.923879532511287,1.,0.923879532511287,1.,0.923879532511287,
1.,0.923879532511287,1.,0.923879532511287,1.,0.923879532511287,1.,0.923879532511287,
1.,0.923879532511287,1.,0.923879532511287,1.,0.923879532511287,1.,0.923879532511287,
1.,0.923879532511287,1.,0.923879532511287,1.,0.923879532511287,1.,0.923879532511287,
1.,0.923879532511287,1.,0.923879532511287,1.,0.923879532511287,1.,0.923879532511287,
1.,0.923879532511287,1.,0.923879532511287,1.,0.923879532511287,1.,0.923879532511287,
1.,0.923879532511287,1.,0.923879532511287,1.,0.923879532511287,1.,0.923879532511287,
1.,0.923879532511287,1.,0.923879532511287,1.,0.923879532511287,1.,0.923879532511287,
1.,0.923879532511287,1.,0.923879532511287,1.,0.923879532511287,1.,0.923879532511287,
1.,0.923879532511287,1.,0.923879532511287,1.,0.923879532511287,1.,0.923879532511287,
1.,0.923879532511287,1.,0.923879532511287,1.,0.923879532511287,1.,0.923879532511287,
1.,0.923879532511287,1.,0.923879532511287,1.,0.923879532511287,1.,0.923879532511287,
1.,0.923879532511287,1.,0.923879532511287,1.,0.923879532511287,1.,0.923879532511287,
1.,0.923879532511287,1.,0.923879532511287,1.,0.923879532511287,1.,0.923879532511287,
1.,0.923879532511287,1.,0.923879532511287,1.,0.923879532511287,1.,0.923879532511287,
1.,0.923879532511287,1.,0.923879532511287,1.,0.923879532511287,1.,0.923879532511287,
1.)))
REPRESENTATION_ITEM('')
SURFACE()
);
#563=(
BOUNDED_SURFACE()
B_SPLINE_SURFACE(1,2,((#23364,#23365,#23366,#23367,#23368,#23369,#23370,
#23371,#23372,#23373,#23374,#23375,#23376,#23377,#23378,#23379,#23380,#23381,
#23382,#23383,#23384,#23385,#23386,#23387,#23388,#23389,#23390,#23391,#23392,
#23393,#23394,#23395,#23396,#23397,#23398,#23399,#23400,#23401,#23402,#23403,
#23404,#23405,#23406,#23407,#23408,#23409,#23410,#23411,#23412,#23413,#23414,
#23415,#23416,#23417,#23418,#23419,#23420,#23421,#23422,#23423,#23424,#23425,
#23426,#23427,#23428,#23429,#23430,#23431,#23432,#23433,#23434,#23435,#23436,
#23437,#23438,#23439,#23440,#23441,#23442,#23443,#23444,#23445,#23446,#23447,
#23448,#23449,#23450,#23451,#23452,#23453,#23454,#23455,#23456,#23457,#23458,
#23459,#23460,#23461,#23462,#23463,#23464,#23465,#23466,#23467,#23468,#23469,
#23470,#23471,#23472,#23473,#23474,#23475,#23476,#23477,#23478,#23479,#23480,
#23481,#23482,#23483,#23484,#23485,#23486,#23487,#23488,#23489,#23490,#23491,
#23492,#23493,#23494,#23495,#23496,#23497,#23498,#23499,#23500,#23501,#23502,
#23503,#23504,#23505,#23506,#23507,#23508,#23509,#23510,#23511,#23512,#23513,
#23514,#23515,#23516,#23517,#23518,#23519,#23520,#23521,#23522,#23523,#23524),
(#23525,#23526,#23527,#23528,#23529,#23530,#23531,#23532,#23533,#23534,
#23535,#23536,#23537,#23538,#23539,#23540,#23541,#23542,#23543,#23544,#23545,
#23546,#23547,#23548,#23549,#23550,#23551,#23552,#23553,#23554,#23555,#23556,
#23557,#23558,#23559,#23560,#23561,#23562,#23563,#23564,#23565,#23566,#23567,
#23568,#23569,#23570,#23571,#23572,#23573,#23574,#23575,#23576,#23577,#23578,
#23579,#23580,#23581,#23582,#23583,#23584,#23585,#23586,#23587,#23588,#23589,
#23590,#23591,#23592,#23593,#23594,#23595,#23596,#23597,#23598,#23599,#23600,
#23601,#23602,#23603,#23604,#23605,#23606,#23607,#23608,#23609,#23610,#23611,
#23612,#23613,#23614,#23615,#23616,#23617,#23618,#23619,#23620,#23621,#23622,
#23623,#23624,#23625,#23626,#23627,#23628,#23629,#23630,#23631,#23632,#23633,
#23634,#23635,#23636,#23637,#23638,#23639,#23640,#23641,#23642,#23643,#23644,
#23645,#23646,#23647,#23648,#23649,#23650,#23651,#23652,#23653,#23654,#23655,
#23656,#23657,#23658,#23659,#23660,#23661,#23662,#23663,#23664,#23665,#23666,
#23667,#23668,#23669,#23670,#23671,#23672,#23673,#23674,#23675,#23676,#23677,
#23678,#23679,#23680,#23681,#23682,#23683,#23684,#23685)),.UNSPECIFIED.,
 .F.,.F.,.F.)
B_SPLINE_SURFACE_WITH_KNOTS((2,2),(3,2,2,2,2,2,2,2,2,2,2,2,2,2,2,2,2,2,
2,2,2,2,2,2,2,2,2,2,2,2,2,2,2,2,2,2,2,2,2,2,2,2,2,2,2,2,2,2,2,2,2,2,2,2,
2,2,2,2,2,2,2,2,2,2,2,2,2,2,2,2,2,2,2,2,2,2,2,2,2,2,3),(0.,1.),(0.,0.0125,
0.025,0.0375,0.05,0.0625,0.075,0.0875,0.1,0.1125,0.125,0.1375,0.15,0.1625,
0.175,0.1875,0.2,0.2125,0.225,0.2375,0.25,0.2625,0.275,0.2875,0.3,0.3125,
0.325,0.3375,0.35,0.3625,0.375,0.3875,0.4,0.4125,0.425,0.4375,0.45,0.4625,
0.475,0.4875,0.5,0.5125,0.525,0.5375,0.55,0.5625,0.575,0.5875,0.6,0.6125,
0.625,0.6375,0.65,0.6625,0.675,0.6875,0.7,0.7125,0.725,0.7375,0.75,0.7625,
0.775,0.7875,0.8,0.8125,0.825,0.8375,0.85,0.8625,0.875,0.8875,0.9,0.9125,
0.925,0.9375,0.95,0.9625,0.975,0.9875,1.),.UNSPECIFIED.)
GEOMETRIC_REPRESENTATION_ITEM()
RATIONAL_B_SPLINE_SURFACE(((1.,0.923879532511287,1.,0.923879532511287,1.,
0.923879532511287,1.,0.923879532511287,1.,0.923879532511287,1.,0.923879532511287,
1.,0.923879532511287,1.,0.923879532511287,1.,0.923879532511287,1.,0.923879532511287,
1.,0.923879532511287,1.,0.923879532511287,1.,0.923879532511287,1.,0.923879532511287,
1.,0.923879532511287,1.,0.923879532511287,1.,0.923879532511287,1.,0.923879532511287,
1.,0.923879532511287,1.,0.923879532511287,1.,0.923879532511287,1.,0.923879532511287,
1.,0.923879532511287,1.,0.923879532511287,1.,0.923879532511287,1.,0.923879532511287,
1.,0.923879532511287,1.,0.923879532511287,1.,0.923879532511287,1.,0.923879532511287,
1.,0.923879532511287,1.,0.923879532511287,1.,0.923879532511287,1.,0.923879532511287,
1.,0.923879532511287,1.,0.923879532511287,1.,0.923879532511287,1.,0.923879532511287,
1.,0.923879532511287,1.,0.923879532511287,1.,0.923879532511287,1.,0.923879532511287,
1.,0.923879532511287,1.,0.923879532511287,1.,0.923879532511287,1.,0.923879532511287,
1.,0.923879532511287,1.,0.923879532511287,1.,0.923879532511287,1.,0.923879532511287,
1.,0.923879532511287,1.,0.923879532511287,1.,0.923879532511287,1.,0.923879532511287,
1.,0.923879532511287,1.,0.923879532511287,1.,0.923879532511287,1.,0.923879532511287,
1.,0.923879532511287,1.,0.923879532511287,1.,0.923879532511287,1.,0.923879532511287,
1.,0.923879532511287,1.,0.923879532511287,1.,0.923879532511287,1.,0.923879532511287,
1.,0.923879532511287,1.,0.923879532511287,1.,0.923879532511287,1.,0.923879532511287,
1.,0.923879532511287,1.,0.923879532511287,1.,0.923879532511287,1.,0.923879532511287,
1.,0.923879532511287,1.,0.923879532511287,1.,0.923879532511287,1.,0.923879532511287,
1.,0.923879532511287,1.,0.923879532511287,1.),(1.,0.923879532511287,1.,
0.923879532511287,1.,0.923879532511287,1.,0.923879532511287,1.,0.923879532511287,
1.,0.923879532511287,1.,0.923879532511287,1.,0.923879532511287,1.,0.923879532511287,
1.,0.923879532511287,1.,0.923879532511287,1.,0.923879532511287,1.,0.923879532511287,
1.,0.923879532511287,1.,0.923879532511287,1.,0.923879532511287,1.,0.923879532511287,
1.,0.923879532511287,1.,0.923879532511287,1.,0.923879532511287,1.,0.923879532511287,
1.,0.923879532511287,1.,0.923879532511287,1.,0.923879532511287,1.,0.923879532511287,
1.,0.923879532511287,1.,0.923879532511287,1.,0.923879532511287,1.,0.923879532511287,
1.,0.923879532511287,1.,0.923879532511287,1.,0.923879532511287,1.,0.923879532511287,
1.,0.923879532511287,1.,0.923879532511287,1.,0.923879532511287,1.,0.923879532511287,
1.,0.923879532511287,1.,0.923879532511287,1.,0.923879532511287,1.,0.923879532511287,
1.,0.923879532511287,1.,0.923879532511287,1.,0.923879532511287,1.,0.923879532511287,
1.,0.923879532511287,1.,0.923879532511287,1.,0.923879532511287,1.,0.923879532511287,
1.,0.923879532511287,1.,0.923879532511287,1.,0.923879532511287,1.,0.923879532511287,
1.,0.923879532511287,1.,0.923879532511287,1.,0.923879532511287,1.,0.923879532511287,
1.,0.923879532511287,1.,0.923879532511287,1.,0.923879532511287,1.,0.923879532511287,
1.,0.923879532511287,1.,0.923879532511287,1.,0.923879532511287,1.,0.923879532511287,
1.,0.923879532511287,1.,0.923879532511287,1.,0.923879532511287,1.,0.923879532511287,
1.,0.923879532511287,1.,0.923879532511287,1.,0.923879532511287,1.,0.923879532511287,
1.,0.923879532511287,1.,0.923879532511287,1.,0.923879532511287,1.,0.923879532511287,
1.,0.923879532511287,1.,0.923879532511287,1.,0.923879532511287,1.)))
REPRESENTATION_ITEM('')
SURFACE()
);
#564=(
BOUNDED_SURFACE()
B_SPLINE_SURFACE(1,2,((#23703,#23704,#23705,#23706,#23707,#23708,#23709,
#23710,#23711,#23712,#23713,#23714,#23715,#23716,#23717,#23718,#23719,#23720,
#23721,#23722,#23723,#23724,#23725,#23726,#23727,#23728,#23729,#23730,#23731,
#23732,#23733,#23734,#23735,#23736,#23737,#23738,#23739,#23740,#23741,#23742,
#23743,#23744,#23745,#23746,#23747,#23748,#23749,#23750,#23751,#23752,#23753,
#23754,#23755,#23756,#23757,#23758,#23759,#23760,#23761,#23762,#23763,#23764,
#23765,#23766,#23767,#23768,#23769,#23770,#23771,#23772,#23773,#23774,#23775,
#23776,#23777,#23778,#23779,#23780,#23781,#23782,#23783,#23784,#23785,#23786,
#23787,#23788,#23789,#23790,#23791,#23792,#23793,#23794,#23795,#23796,#23797,
#23798,#23799,#23800,#23801,#23802,#23803,#23804,#23805,#23806,#23807,#23808,
#23809,#23810,#23811,#23812,#23813,#23814,#23815,#23816,#23817,#23818,#23819,
#23820,#23821,#23822,#23823,#23824,#23825,#23826,#23827,#23828,#23829,#23830,
#23831,#23832,#23833,#23834,#23835,#23836,#23837,#23838,#23839,#23840,#23841,
#23842,#23843,#23844,#23845,#23846,#23847,#23848,#23849,#23850,#23851,#23852,
#23853,#23854,#23855,#23856,#23857,#23858,#23859,#23860,#23861,#23862,#23863),
(#23864,#23865,#23866,#23867,#23868,#23869,#23870,#23871,#23872,#23873,
#23874,#23875,#23876,#23877,#23878,#23879,#23880,#23881,#23882,#23883,#23884,
#23885,#23886,#23887,#23888,#23889,#23890,#23891,#23892,#23893,#23894,#23895,
#23896,#23897,#23898,#23899,#23900,#23901,#23902,#23903,#23904,#23905,#23906,
#23907,#23908,#23909,#23910,#23911,#23912,#23913,#23914,#23915,#23916,#23917,
#23918,#23919,#23920,#23921,#23922,#23923,#23924,#23925,#23926,#23927,#23928,
#23929,#23930,#23931,#23932,#23933,#23934,#23935,#23936,#23937,#23938,#23939,
#23940,#23941,#23942,#23943,#23944,#23945,#23946,#23947,#23948,#23949,#23950,
#23951,#23952,#23953,#23954,#23955,#23956,#23957,#23958,#23959,#23960,#23961,
#23962,#23963,#23964,#23965,#23966,#23967,#23968,#23969,#23970,#23971,#23972,
#23973,#23974,#23975,#23976,#23977,#23978,#23979,#23980,#23981,#23982,#23983,
#23984,#23985,#23986,#23987,#23988,#23989,#23990,#23991,#23992,#23993,#23994,
#23995,#23996,#23997,#23998,#23999,#24000,#24001,#24002,#24003,#24004,#24005,
#24006,#24007,#24008,#24009,#24010,#24011,#24012,#24013,#24014,#24015,#24016,
#24017,#24018,#24019,#24020,#24021,#24022,#24023,#24024)),.UNSPECIFIED.,
 .F.,.F.,.F.)
B_SPLINE_SURFACE_WITH_KNOTS((2,2),(3,2,2,2,2,2,2,2,2,2,2,2,2,2,2,2,2,2,
2,2,2,2,2,2,2,2,2,2,2,2,2,2,2,2,2,2,2,2,2,2,2,2,2,2,2,2,2,2,2,2,2,2,2,2,
2,2,2,2,2,2,2,2,2,2,2,2,2,2,2,2,2,2,2,2,2,2,2,2,2,2,3),(0.,1.),(0.,0.0125,
0.025,0.0375,0.05,0.0625,0.075,0.0875,0.1,0.1125,0.125,0.1375,0.15,0.1625,
0.175,0.1875,0.2,0.2125,0.225,0.2375,0.25,0.2625,0.275,0.2875,0.3,0.3125,
0.325,0.3375,0.35,0.3625,0.375,0.3875,0.4,0.4125,0.425,0.4375,0.45,0.4625,
0.475,0.4875,0.5,0.5125,0.525,0.5375,0.55,0.5625,0.575,0.5875,0.6,0.6125,
0.625,0.6375,0.65,0.6625,0.675,0.6875,0.7,0.7125,0.725,0.7375,0.75,0.7625,
0.775,0.7875,0.8,0.8125,0.825,0.8375,0.85,0.8625,0.875,0.8875,0.9,0.9125,
0.925,0.9375,0.95,0.9625,0.975,0.9875,1.),.UNSPECIFIED.)
GEOMETRIC_REPRESENTATION_ITEM()
RATIONAL_B_SPLINE_SURFACE(((1.,0.923879532511287,1.,0.923879532511287,1.,
0.923879532511287,1.,0.923879532511287,1.,0.923879532511287,1.,0.923879532511287,
1.,0.923879532511287,1.,0.923879532511287,1.,0.923879532511287,1.,0.923879532511287,
1.,0.923879532511287,1.,0.923879532511287,1.,0.923879532511287,1.,0.923879532511287,
1.,0.923879532511287,1.,0.923879532511287,1.,0.923879532511287,1.,0.923879532511287,
1.,0.923879532511287,1.,0.923879532511287,1.,0.923879532511287,1.,0.923879532511287,
1.,0.923879532511287,1.,0.923879532511287,1.,0.923879532511287,1.,0.923879532511287,
1.,0.923879532511287,1.,0.923879532511287,1.,0.923879532511287,1.,0.923879532511287,
1.,0.923879532511287,1.,0.923879532511287,1.,0.923879532511287,1.,0.923879532511287,
1.,0.923879532511287,1.,0.923879532511287,1.,0.923879532511287,1.,0.923879532511287,
1.,0.923879532511287,1.,0.923879532511287,1.,0.923879532511287,1.,0.923879532511287,
1.,0.923879532511287,1.,0.923879532511287,1.,0.923879532511287,1.,0.923879532511287,
1.,0.923879532511287,1.,0.923879532511287,1.,0.923879532511287,1.,0.923879532511287,
1.,0.923879532511287,1.,0.923879532511287,1.,0.923879532511287,1.,0.923879532511287,
1.,0.923879532511287,1.,0.923879532511287,1.,0.923879532511287,1.,0.923879532511287,
1.,0.923879532511287,1.,0.923879532511287,1.,0.923879532511287,1.,0.923879532511287,
1.,0.923879532511287,1.,0.923879532511287,1.,0.923879532511287,1.,0.923879532511287,
1.,0.923879532511287,1.,0.923879532511287,1.,0.923879532511287,1.,0.923879532511287,
1.,0.923879532511287,1.,0.923879532511287,1.,0.923879532511287,1.,0.923879532511287,
1.,0.923879532511287,1.,0.923879532511287,1.,0.923879532511287,1.,0.923879532511287,
1.,0.923879532511287,1.,0.923879532511287,1.),(1.,0.923879532511287,1.,
0.923879532511287,1.,0.923879532511287,1.,0.923879532511287,1.,0.923879532511287,
1.,0.923879532511287,1.,0.923879532511287,1.,0.923879532511287,1.,0.923879532511287,
1.,0.923879532511287,1.,0.923879532511287,1.,0.923879532511287,1.,0.923879532511287,
1.,0.923879532511287,1.,0.923879532511287,1.,0.923879532511287,1.,0.923879532511287,
1.,0.923879532511287,1.,0.923879532511287,1.,0.923879532511287,1.,0.923879532511287,
1.,0.923879532511287,1.,0.923879532511287,1.,0.923879532511287,1.,0.923879532511287,
1.,0.923879532511287,1.,0.923879532511287,1.,0.923879532511287,1.,0.923879532511287,
1.,0.923879532511287,1.,0.923879532511287,1.,0.923879532511287,1.,0.923879532511287,
1.,0.923879532511287,1.,0.923879532511287,1.,0.923879532511287,1.,0.923879532511287,
1.,0.923879532511287,1.,0.923879532511287,1.,0.923879532511287,1.,0.923879532511287,
1.,0.923879532511287,1.,0.923879532511287,1.,0.923879532511287,1.,0.923879532511287,
1.,0.923879532511287,1.,0.923879532511287,1.,0.923879532511287,1.,0.923879532511287,
1.,0.923879532511287,1.,0.923879532511287,1.,0.923879532511287,1.,0.923879532511287,
1.,0.923879532511287,1.,0.923879532511287,1.,0.923879532511287,1.,0.923879532511287,
1.,0.923879532511287,1.,0.923879532511287,1.,0.923879532511287,1.,0.923879532511287,
1.,0.923879532511287,1.,0.923879532511287,1.,0.923879532511287,1.,0.923879532511287,
1.,0.923879532511287,1.,0.923879532511287,1.,0.923879532511287,1.,0.923879532511287,
1.,0.923879532511287,1.,0.923879532511287,1.,0.923879532511287,1.,0.923879532511287,
1.,0.923879532511287,1.,0.923879532511287,1.,0.923879532511287,1.,0.923879532511287,
1.,0.923879532511287,1.,0.923879532511287,1.,0.923879532511287,1.)))
REPRESENTATION_ITEM('')
SURFACE()
);
#565=(
BOUNDED_SURFACE()
B_SPLINE_SURFACE(3,2,((#24040,#24041,#24042,#24043,#24044,#24045,#24046,
#24047,#24048,#24049,#24050,#24051,#24052,#24053,#24054,#24055,#24056,#24057,
#24058,#24059,#24060,#24061,#24062,#24063,#24064,#24065,#24066,#24067,#24068,
#24069,#24070,#24071,#24072,#24073,#24074,#24075,#24076,#24077,#24078,#24079,
#24080,#24081,#24082,#24083,#24084,#24085,#24086,#24087,#24088,#24089,#24090,
#24091,#24092,#24093,#24094,#24095,#24096,#24097,#24098,#24099,#24100,#24101,
#24102,#24103,#24104,#24105,#24106,#24107,#24108,#24109,#24110,#24111,#24112,
#24113,#24114,#24115,#24116,#24117,#24118,#24119,#24120,#24121,#24122,#24123,
#24124,#24125,#24126,#24127,#24128,#24129,#24130,#24131,#24132,#24133,#24134,
#24135,#24136,#24137,#24138,#24139,#24140,#24141,#24142,#24143,#24144,#24145,
#24146,#24147,#24148,#24149,#24150,#24151,#24152,#24153,#24154,#24155,#24156,
#24157,#24158,#24159,#24160,#24161,#24162,#24163,#24164,#24165,#24166,#24167,
#24168,#24169,#24170,#24171,#24172,#24173,#24174,#24175,#24176,#24177,#24178,
#24179,#24180,#24181,#24182,#24183,#24184,#24185,#24186,#24187,#24188,#24189,
#24190,#24191,#24192,#24193,#24194,#24195,#24196,#24197,#24198,#24199,#24200),
(#24201,#24202,#24203,#24204,#24205,#24206,#24207,#24208,#24209,#24210,
#24211,#24212,#24213,#24214,#24215,#24216,#24217,#24218,#24219,#24220,#24221,
#24222,#24223,#24224,#24225,#24226,#24227,#24228,#24229,#24230,#24231,#24232,
#24233,#24234,#24235,#24236,#24237,#24238,#24239,#24240,#24241,#24242,#24243,
#24244,#24245,#24246,#24247,#24248,#24249,#24250,#24251,#24252,#24253,#24254,
#24255,#24256,#24257,#24258,#24259,#24260,#24261,#24262,#24263,#24264,#24265,
#24266,#24267,#24268,#24269,#24270,#24271,#24272,#24273,#24274,#24275,#24276,
#24277,#24278,#24279,#24280,#24281,#24282,#24283,#24284,#24285,#24286,#24287,
#24288,#24289,#24290,#24291,#24292,#24293,#24294,#24295,#24296,#24297,#24298,
#24299,#24300,#24301,#24302,#24303,#24304,#24305,#24306,#24307,#24308,#24309,
#24310,#24311,#24312,#24313,#24314,#24315,#24316,#24317,#24318,#24319,#24320,
#24321,#24322,#24323,#24324,#24325,#24326,#24327,#24328,#24329,#24330,#24331,
#24332,#24333,#24334,#24335,#24336,#24337,#24338,#24339,#24340,#24341,#24342,
#24343,#24344,#24345,#24346,#24347,#24348,#24349,#24350,#24351,#24352,#24353,
#24354,#24355,#24356,#24357,#24358,#24359,#24360,#24361),(#24362,#24363,
#24364,#24365,#24366,#24367,#24368,#24369,#24370,#24371,#24372,#24373,#24374,
#24375,#24376,#24377,#24378,#24379,#24380,#24381,#24382,#24383,#24384,#24385,
#24386,#24387,#24388,#24389,#24390,#24391,#24392,#24393,#24394,#24395,#24396,
#24397,#24398,#24399,#24400,#24401,#24402,#24403,#24404,#24405,#24406,#24407,
#24408,#24409,#24410,#24411,#24412,#24413,#24414,#24415,#24416,#24417,#24418,
#24419,#24420,#24421,#24422,#24423,#24424,#24425,#24426,#24427,#24428,#24429,
#24430,#24431,#24432,#24433,#24434,#24435,#24436,#24437,#24438,#24439,#24440,
#24441,#24442,#24443,#24444,#24445,#24446,#24447,#24448,#24449,#24450,#24451,
#24452,#24453,#24454,#24455,#24456,#24457,#24458,#24459,#24460,#24461,#24462,
#24463,#24464,#24465,#24466,#24467,#24468,#24469,#24470,#24471,#24472,#24473,
#24474,#24475,#24476,#24477,#24478,#24479,#24480,#24481,#24482,#24483,#24484,
#24485,#24486,#24487,#24488,#24489,#24490,#24491,#24492,#24493,#24494,#24495,
#24496,#24497,#24498,#24499,#24500,#24501,#24502,#24503,#24504,#24505,#24506,
#24507,#24508,#24509,#24510,#24511,#24512,#24513,#24514,#24515,#24516,#24517,
#24518,#24519,#24520,#24521,#24522),(#24523,#24524,#24525,#24526,#24527,
#24528,#24529,#24530,#24531,#24532,#24533,#24534,#24535,#24536,#24537,#24538,
#24539,#24540,#24541,#24542,#24543,#24544,#24545,#24546,#24547,#24548,#24549,
#24550,#24551,#24552,#24553,#24554,#24555,#24556,#24557,#24558,#24559,#24560,
#24561,#24562,#24563,#24564,#24565,#24566,#24567,#24568,#24569,#24570,#24571,
#24572,#24573,#24574,#24575,#24576,#24577,#24578,#24579,#24580,#24581,#24582,
#24583,#24584,#24585,#24586,#24587,#24588,#24589,#24590,#24591,#24592,#24593,
#24594,#24595,#24596,#24597,#24598,#24599,#24600,#24601,#24602,#24603,#24604,
#24605,#24606,#24607,#24608,#24609,#24610,#24611,#24612,#24613,#24614,#24615,
#24616,#24617,#24618,#24619,#24620,#24621,#24622,#24623,#24624,#24625,#24626,
#24627,#24628,#24629,#24630,#24631,#24632,#24633,#24634,#24635,#24636,#24637,
#24638,#24639,#24640,#24641,#24642,#24643,#24644,#24645,#24646,#24647,#24648,
#24649,#24650,#24651,#24652,#24653,#24654,#24655,#24656,#24657,#24658,#24659,
#24660,#24661,#24662,#24663,#24664,#24665,#24666,#24667,#24668,#24669,#24670,
#24671,#24672,#24673,#24674,#24675,#24676,#24677,#24678,#24679,#24680,#24681,
#24682,#24683)),.UNSPECIFIED.,.F.,.F.,.F.)
B_SPLINE_SURFACE_WITH_KNOTS((4,4),(3,2,2,2,2,2,2,2,2,2,2,2,2,2,2,2,2,2,
2,2,2,2,2,2,2,2,2,2,2,2,2,2,2,2,2,2,2,2,2,2,2,2,2,2,2,2,2,2,2,2,2,2,2,2,
2,2,2,2,2,2,2,2,2,2,2,2,2,2,2,2,2,2,2,2,2,2,2,2,2,2,3),(0.,1.),(0.,0.0125,
0.025,0.0375,0.05,0.0625,0.075,0.0875,0.1,0.1125,0.125,0.1375,0.15,0.1625,
0.175,0.1875,0.2,0.2125,0.225,0.2375,0.25,0.2625,0.275,0.2875,0.3,0.3125,
0.325,0.3375,0.35,0.3625,0.375,0.3875,0.4,0.4125,0.425,0.4375,0.45,0.4625,
0.475,0.4875,0.5,0.5125,0.525,0.5375,0.55,0.5625,0.575,0.5875,0.6,0.6125,
0.625,0.6375,0.65,0.6625,0.675,0.6875,0.7,0.7125,0.725,0.7375,0.75,0.7625,
0.775,0.7875,0.8,0.8125,0.825,0.8375,0.85,0.8625,0.875,0.8875,0.9,0.9125,
0.925,0.9375,0.95,0.9625,0.975,0.9875,1.),.UNSPECIFIED.)
GEOMETRIC_REPRESENTATION_ITEM()
RATIONAL_B_SPLINE_SURFACE(((1.,0.923879532511287,1.,0.923879532511287,1.,
0.923879532511287,1.,0.923879532511287,1.,0.923879532511287,1.,0.923879532511287,
1.,0.923879532511287,1.,0.923879532511287,1.,0.923879532511287,1.,0.923879532511287,
1.,0.923879532511287,1.,0.923879532511287,1.,0.923879532511287,1.,0.923879532511287,
1.,0.923879532511287,1.,0.923879532511287,1.,0.923879532511287,1.,0.923879532511287,
1.,0.923879532511287,1.,0.923879532511287,1.,0.923879532511287,1.,0.923879532511287,
1.,0.923879532511287,1.,0.923879532511287,1.,0.923879532511287,1.,0.923879532511287,
1.,0.923879532511287,1.,0.923879532511287,1.,0.923879532511287,1.,0.923879532511287,
1.,0.923879532511287,1.,0.923879532511287,1.,0.923879532511287,1.,0.923879532511287,
1.,0.923879532511287,1.,0.923879532511287,1.,0.923879532511287,1.,0.923879532511287,
1.,0.923879532511287,1.,0.923879532511287,1.,0.923879532511287,1.,0.923879532511287,
1.,0.923879532511287,1.,0.923879532511287,1.,0.923879532511287,1.,0.923879532511287,
1.,0.923879532511287,1.,0.923879532511287,1.,0.923879532511287,1.,0.923879532511287,
1.,0.923879532511287,1.,0.923879532511287,1.,0.923879532511287,1.,0.923879532511287,
1.,0.923879532511287,1.,0.923879532511287,1.,0.923879532511287,1.,0.923879532511287,
1.,0.923879532511287,1.,0.923879532511287,1.,0.923879532511287,1.,0.923879532511287,
1.,0.923879532511287,1.,0.923879532511287,1.,0.923879532511287,1.,0.923879532511287,
1.,0.923879532511287,1.,0.923879532511287,1.,0.923879532511287,1.,0.923879532511287,
1.,0.923879532511287,1.,0.923879532511287,1.,0.923879532511287,1.,0.923879532511287,
1.,0.923879532511287,1.,0.923879532511287,1.,0.923879532511287,1.,0.923879532511287,
1.,0.923879532511287,1.,0.923879532511287,1.),(0.998696642611305,0.922675387296324,
0.998696642611305,0.922675387296324,0.998696642611305,0.922675387296324,
0.998696642611305,0.922675387296324,0.998696642611305,0.922675387296324,
0.998696642611305,0.922675387296324,0.998696642611305,0.922675387296324,
0.998696642611305,0.922675387296324,0.998696642611305,0.922675387296324,
0.998696642611305,0.922675387296324,0.998696642611305,0.922675387296324,
0.998696642611305,0.922675387296324,0.998696642611305,0.922675387296324,
0.998696642611305,0.922675387296324,0.998696642611305,0.922675387296324,
0.998696642611305,0.922675387296324,0.998696642611305,0.922675387296324,
0.998696642611305,0.922675387296324,0.998696642611305,0.922675387296324,
0.998696642611305,0.922675387296324,0.998696642611305,0.922675387296324,
0.998696642611305,0.922675387296324,0.998696642611305,0.922675387296324,
0.998696642611305,0.922675387296324,0.998696642611305,0.922675387296324,
0.998696642611305,0.922675387296324,0.998696642611305,0.922675387296324,
0.998696642611305,0.922675387296324,0.998696642611305,0.922675387296324,
0.998696642611305,0.922675387296324,0.998696642611305,0.922675387296324,
0.998696642611305,0.922675387296324,0.998696642611305,0.922675387296324,
0.998696642611305,0.922675387296324,0.998696642611305,0.922675387296324,
0.998696642611305,0.922675387296324,0.998696642611305,0.922675387296324,
0.998696642611305,0.922675387296324,0.998696642611305,0.922675387296324,
0.998696642611305,0.922675387296324,0.998696642611305,0.922675387296324,
0.998696642611305,0.922675387296324,0.998696642611305,0.922675387296324,
0.998696642611305,0.922675387296324,0.998696642611305,0.922675387296324,
0.998696642611305,0.922675387296324,0.998696642611305,0.922675387296324,
0.998696642611305,0.922675387296324,0.998696642611305,0.922675387296324,
0.998696642611305,0.922675387296324,0.998696642611305,0.922675387296324,
0.998696642611305,0.922675387296324,0.998696642611305,0.922675387296324,
0.998696642611305,0.922675387296324,0.998696642611305,0.922675387296324,
0.998696642611305,0.922675387296324,0.998696642611305,0.922675387296324,
0.998696642611305,0.922675387296324,0.998696642611305,0.922675387296324,
0.998696642611305,0.922675387296324,0.998696642611305,0.922675387296324,
0.998696642611305,0.922675387296324,0.998696642611305,0.922675387296324,
0.998696642611305,0.922675387296324,0.998696642611305,0.922675387296324,
0.998696642611305,0.922675387296324,0.998696642611305,0.922675387296324,
0.998696642611305,0.922675387296324,0.998696642611305,0.922675387296324,
0.998696642611305,0.922675387296324,0.998696642611305,0.922675387296324,
0.998696642611305,0.922675387296324,0.998696642611305,0.922675387296324,
0.998696642611305,0.922675387296324,0.998696642611305,0.922675387296324,
0.998696642611305,0.922675387296324,0.998696642611305,0.922675387296324,
0.998696642611305,0.922675387296324,0.998696642611305,0.922675387296324,
0.998696642611305,0.922675387296324,0.998696642611305),(0.998696642611305,
0.922675387296324,0.998696642611305,0.922675387296324,0.998696642611305,
0.922675387296324,0.998696642611305,0.922675387296324,0.998696642611305,
0.922675387296324,0.998696642611305,0.922675387296324,0.998696642611305,
0.922675387296324,0.998696642611305,0.922675387296324,0.998696642611305,
0.922675387296324,0.998696642611305,0.922675387296324,0.998696642611305,
0.922675387296324,0.998696642611305,0.922675387296324,0.998696642611305,
0.922675387296324,0.998696642611305,0.922675387296324,0.998696642611305,
0.922675387296324,0.998696642611305,0.922675387296324,0.998696642611305,
0.922675387296324,0.998696642611305,0.922675387296324,0.998696642611305,
0.922675387296324,0.998696642611305,0.922675387296324,0.998696642611305,
0.922675387296324,0.998696642611305,0.922675387296324,0.998696642611305,
0.922675387296324,0.998696642611305,0.922675387296324,0.998696642611305,
0.922675387296324,0.998696642611305,0.922675387296324,0.998696642611305,
0.922675387296324,0.998696642611305,0.922675387296324,0.998696642611305,
0.922675387296324,0.998696642611305,0.922675387296324,0.998696642611305,
0.922675387296324,0.998696642611305,0.922675387296324,0.998696642611305,
0.922675387296324,0.998696642611305,0.922675387296324,0.998696642611305,
0.922675387296324,0.998696642611305,0.922675387296324,0.998696642611305,
0.922675387296324,0.998696642611305,0.922675387296324,0.998696642611305,
0.922675387296324,0.998696642611305,0.922675387296324,0.998696642611305,
0.922675387296324,0.998696642611305,0.922675387296324,0.998696642611305,
0.922675387296324,0.998696642611305,0.922675387296324,0.998696642611305,
0.922675387296324,0.998696642611305,0.922675387296324,0.998696642611305,
0.922675387296324,0.998696642611305,0.922675387296324,0.998696642611305,
0.922675387296324,0.998696642611305,0.922675387296324,0.998696642611305,
0.922675387296324,0.998696642611305,0.922675387296324,0.998696642611305,
0.922675387296324,0.998696642611305,0.922675387296324,0.998696642611305,
0.922675387296324,0.998696642611305,0.922675387296324,0.998696642611305,
0.922675387296324,0.998696642611305,0.922675387296324,0.998696642611305,
0.922675387296324,0.998696642611305,0.922675387296324,0.998696642611305,
0.922675387296324,0.998696642611305,0.922675387296324,0.998696642611305,
0.922675387296324,0.998696642611305,0.922675387296324,0.998696642611305,
0.922675387296324,0.998696642611305,0.922675387296324,0.998696642611305,
0.922675387296324,0.998696642611305,0.922675387296324,0.998696642611305,
0.922675387296324,0.998696642611305,0.922675387296324,0.998696642611305,
0.922675387296324,0.998696642611305,0.922675387296324,0.998696642611305,
0.922675387296324,0.998696642611305,0.922675387296324,0.998696642611305,
0.922675387296324,0.998696642611305,0.922675387296324,0.998696642611305,
0.922675387296324,0.998696642611305,0.922675387296324,0.998696642611305,
0.922675387296324,0.998696642611305,0.922675387296324,0.998696642611305),
(1.,0.923879532511287,1.,0.923879532511287,1.,0.923879532511287,1.,0.923879532511287,
1.,0.923879532511287,1.,0.923879532511287,1.,0.923879532511287,1.,0.923879532511287,
1.,0.923879532511287,1.,0.923879532511287,1.,0.923879532511287,1.,0.923879532511287,
1.,0.923879532511287,1.,0.923879532511287,1.,0.923879532511287,1.,0.923879532511287,
1.,0.923879532511287,1.,0.923879532511287,1.,0.923879532511287,1.,0.923879532511287,
1.,0.923879532511287,1.,0.923879532511287,1.,0.923879532511287,1.,0.923879532511287,
1.,0.923879532511287,1.,0.923879532511287,1.,0.923879532511287,1.,0.923879532511287,
1.,0.923879532511287,1.,0.923879532511287,1.,0.923879532511287,1.,0.923879532511287,
1.,0.923879532511287,1.,0.923879532511287,1.,0.923879532511287,1.,0.923879532511287,
1.,0.923879532511287,1.,0.923879532511287,1.,0.923879532511287,1.,0.923879532511287,
1.,0.923879532511287,1.,0.923879532511287,1.,0.923879532511287,1.,0.923879532511287,
1.,0.923879532511287,1.,0.923879532511287,1.,0.923879532511287,1.,0.923879532511287,
1.,0.923879532511287,1.,0.923879532511287,1.,0.923879532511287,1.,0.923879532511287,
1.,0.923879532511287,1.,0.923879532511287,1.,0.923879532511287,1.,0.923879532511287,
1.,0.923879532511287,1.,0.923879532511287,1.,0.923879532511287,1.,0.923879532511287,
1.,0.923879532511287,1.,0.923879532511287,1.,0.923879532511287,1.,0.923879532511287,
1.,0.923879532511287,1.,0.923879532511287,1.,0.923879532511287,1.,0.923879532511287,
1.,0.923879532511287,1.,0.923879532511287,1.,0.923879532511287,1.,0.923879532511287,
1.,0.923879532511287,1.,0.923879532511287,1.,0.923879532511287,1.,0.923879532511287,
1.,0.923879532511287,1.,0.923879532511287,1.,0.923879532511287,1.,0.923879532511287,
1.)))
REPRESENTATION_ITEM('')
SURFACE()
);
#566=(
BOUNDED_SURFACE()
B_SPLINE_SURFACE(1,2,((#24684,#24685,#24686,#24687,#24688,#24689,#24690,
#24691,#24692,#24693,#24694,#24695,#24696,#24697,#24698,#24699,#24700,#24701,
#24702,#24703,#24704,#24705,#24706,#24707,#24708,#24709,#24710,#24711,#24712,
#24713,#24714,#24715,#24716,#24717,#24718,#24719,#24720,#24721,#24722,#24723,
#24724,#24725,#24726,#24727,#24728,#24729,#24730,#24731,#24732,#24733,#24734,
#24735,#24736,#24737,#24738,#24739,#24740,#24741,#24742,#24743,#24744,#24745,
#24746,#24747,#24748,#24749,#24750,#24751,#24752,#24753,#24754,#24755,#24756,
#24757,#24758,#24759,#24760,#24761,#24762,#24763,#24764,#24765,#24766,#24767,
#24768,#24769,#24770,#24771,#24772,#24773,#24774,#24775,#24776,#24777,#24778,
#24779,#24780,#24781,#24782,#24783,#24784,#24785,#24786,#24787,#24788,#24789,
#24790,#24791,#24792,#24793,#24794,#24795,#24796,#24797,#24798,#24799,#24800,
#24801,#24802,#24803,#24804,#24805,#24806,#24807,#24808,#24809,#24810,#24811,
#24812,#24813,#24814,#24815,#24816,#24817,#24818,#24819,#24820,#24821,#24822,
#24823,#24824,#24825,#24826,#24827,#24828,#24829,#24830,#24831,#24832,#24833,
#24834,#24835,#24836,#24837,#24838,#24839,#24840,#24841,#24842,#24843,#24844),
(#24845,#24846,#24847,#24848,#24849,#24850,#24851,#24852,#24853,#24854,
#24855,#24856,#24857,#24858,#24859,#24860,#24861,#24862,#24863,#24864,#24865,
#24866,#24867,#24868,#24869,#24870,#24871,#24872,#24873,#24874,#24875,#24876,
#24877,#24878,#24879,#24880,#24881,#24882,#24883,#24884,#24885,#24886,#24887,
#24888,#24889,#24890,#24891,#24892,#24893,#24894,#24895,#24896,#24897,#24898,
#24899,#24900,#24901,#24902,#24903,#24904,#24905,#24906,#24907,#24908,#24909,
#24910,#24911,#24912,#24913,#24914,#24915,#24916,#24917,#24918,#24919,#24920,
#24921,#24922,#24923,#24924,#24925,#24926,#24927,#24928,#24929,#24930,#24931,
#24932,#24933,#24934,#24935,#24936,#24937,#24938,#24939,#24940,#24941,#24942,
#24943,#24944,#24945,#24946,#24947,#24948,#24949,#24950,#24951,#24952,#24953,
#24954,#24955,#24956,#24957,#24958,#24959,#24960,#24961,#24962,#24963,#24964,
#24965,#24966,#24967,#24968,#24969,#24970,#24971,#24972,#24973,#24974,#24975,
#24976,#24977,#24978,#24979,#24980,#24981,#24982,#24983,#24984,#24985,#24986,
#24987,#24988,#24989,#24990,#24991,#24992,#24993,#24994,#24995,#24996,#24997,
#24998,#24999,#25000,#25001,#25002,#25003,#25004,#25005)),.UNSPECIFIED.,
 .F.,.F.,.F.)
B_SPLINE_SURFACE_WITH_KNOTS((2,2),(3,2,2,2,2,2,2,2,2,2,2,2,2,2,2,2,2,2,
2,2,2,2,2,2,2,2,2,2,2,2,2,2,2,2,2,2,2,2,2,2,2,2,2,2,2,2,2,2,2,2,2,2,2,2,
2,2,2,2,2,2,2,2,2,2,2,2,2,2,2,2,2,2,2,2,2,2,2,2,2,2,3),(0.,1.),(0.,0.0125,
0.025,0.0375,0.05,0.0625,0.075,0.0875,0.1,0.1125,0.125,0.1375,0.15,0.1625,
0.175,0.1875,0.2,0.2125,0.225,0.2375,0.25,0.2625,0.275,0.2875,0.3,0.3125,
0.325,0.3375,0.35,0.3625,0.375,0.3875,0.4,0.4125,0.425,0.4375,0.45,0.4625,
0.475,0.4875,0.5,0.5125,0.525,0.5375,0.55,0.5625,0.575,0.5875,0.6,0.6125,
0.625,0.6375,0.65,0.6625,0.675,0.6875,0.7,0.7125,0.725,0.7375,0.75,0.7625,
0.775,0.7875,0.8,0.8125,0.825,0.8375,0.85,0.8625,0.875,0.8875,0.9,0.9125,
0.925,0.9375,0.95,0.9625,0.975,0.9875,1.),.UNSPECIFIED.)
GEOMETRIC_REPRESENTATION_ITEM()
RATIONAL_B_SPLINE_SURFACE(((1.,0.923879532511287,1.,0.923879532511287,1.,
0.923879532511287,1.,0.923879532511287,1.,0.923879532511287,1.,0.923879532511287,
1.,0.923879532511287,1.,0.923879532511287,1.,0.923879532511287,1.,0.923879532511287,
1.,0.923879532511287,1.,0.923879532511287,1.,0.923879532511287,1.,0.923879532511287,
1.,0.923879532511287,1.,0.923879532511287,1.,0.923879532511287,1.,0.923879532511287,
1.,0.923879532511287,1.,0.923879532511287,1.,0.923879532511287,1.,0.923879532511287,
1.,0.923879532511287,1.,0.923879532511287,1.,0.923879532511287,1.,0.923879532511287,
1.,0.923879532511287,1.,0.923879532511287,1.,0.923879532511287,1.,0.923879532511287,
1.,0.923879532511287,1.,0.923879532511287,1.,0.923879532511287,1.,0.923879532511287,
1.,0.923879532511287,1.,0.923879532511287,1.,0.923879532511287,1.,0.923879532511287,
1.,0.923879532511287,1.,0.923879532511287,1.,0.923879532511287,1.,0.923879532511287,
1.,0.923879532511287,1.,0.923879532511287,1.,0.923879532511287,1.,0.923879532511287,
1.,0.923879532511287,1.,0.923879532511287,1.,0.923879532511287,1.,0.923879532511287,
1.,0.923879532511287,1.,0.923879532511287,1.,0.923879532511287,1.,0.923879532511287,
1.,0.923879532511287,1.,0.923879532511287,1.,0.923879532511287,1.,0.923879532511287,
1.,0.923879532511287,1.,0.923879532511287,1.,0.923879532511287,1.,0.923879532511287,
1.,0.923879532511287,1.,0.923879532511287,1.,0.923879532511287,1.,0.923879532511287,
1.,0.923879532511287,1.,0.923879532511287,1.,0.923879532511287,1.,0.923879532511287,
1.,0.923879532511287,1.,0.923879532511287,1.,0.923879532511287,1.,0.923879532511287,
1.,0.923879532511287,1.,0.923879532511287,1.,0.923879532511287,1.,0.923879532511287,
1.,0.923879532511287,1.,0.923879532511287,1.),(1.,0.923879532511287,1.,
0.923879532511287,1.,0.923879532511287,1.,0.923879532511287,1.,0.923879532511287,
1.,0.923879532511287,1.,0.923879532511287,1.,0.923879532511287,1.,0.923879532511287,
1.,0.923879532511287,1.,0.923879532511287,1.,0.923879532511287,1.,0.923879532511287,
1.,0.923879532511287,1.,0.923879532511287,1.,0.923879532511287,1.,0.923879532511287,
1.,0.923879532511287,1.,0.923879532511287,1.,0.923879532511287,1.,0.923879532511287,
1.,0.923879532511287,1.,0.923879532511287,1.,0.923879532511287,1.,0.923879532511287,
1.,0.923879532511287,1.,0.923879532511287,1.,0.923879532511287,1.,0.923879532511287,
1.,0.923879532511287,1.,0.923879532511287,1.,0.923879532511287,1.,0.923879532511287,
1.,0.923879532511287,1.,0.923879532511287,1.,0.923879532511287,1.,0.923879532511287,
1.,0.923879532511287,1.,0.923879532511287,1.,0.923879532511287,1.,0.923879532511287,
1.,0.923879532511287,1.,0.923879532511287,1.,0.923879532511287,1.,0.923879532511287,
1.,0.923879532511287,1.,0.923879532511287,1.,0.923879532511287,1.,0.923879532511287,
1.,0.923879532511287,1.,0.923879532511287,1.,0.923879532511287,1.,0.923879532511287,
1.,0.923879532511287,1.,0.923879532511287,1.,0.923879532511287,1.,0.923879532511287,
1.,0.923879532511287,1.,0.923879532511287,1.,0.923879532511287,1.,0.923879532511287,
1.,0.923879532511287,1.,0.923879532511287,1.,0.923879532511287,1.,0.923879532511287,
1.,0.923879532511287,1.,0.923879532511287,1.,0.923879532511287,1.,0.923879532511287,
1.,0.923879532511287,1.,0.923879532511287,1.,0.923879532511287,1.,0.923879532511287,
1.,0.923879532511287,1.,0.923879532511287,1.,0.923879532511287,1.,0.923879532511287,
1.,0.923879532511287,1.,0.923879532511287,1.,0.923879532511287,1.)))
REPRESENTATION_ITEM('')
SURFACE()
);
#567=(
BOUNDED_SURFACE()
B_SPLINE_SURFACE(1,2,((#25023,#25024,#25025,#25026,#25027,#25028,#25029,
#25030,#25031,#25032,#25033,#25034,#25035,#25036,#25037,#25038,#25039,#25040,
#25041,#25042,#25043,#25044,#25045,#25046,#25047,#25048,#25049,#25050,#25051,
#25052,#25053,#25054,#25055,#25056,#25057,#25058,#25059,#25060,#25061,#25062,
#25063,#25064,#25065,#25066,#25067,#25068,#25069,#25070,#25071,#25072,#25073,
#25074,#25075,#25076,#25077,#25078,#25079,#25080,#25081,#25082,#25083,#25084,
#25085,#25086,#25087,#25088,#25089,#25090,#25091,#25092,#25093,#25094,#25095,
#25096,#25097,#25098,#25099,#25100,#25101,#25102,#25103,#25104,#25105,#25106,
#25107,#25108,#25109,#25110,#25111,#25112,#25113,#25114,#25115,#25116,#25117,
#25118,#25119,#25120,#25121,#25122,#25123,#25124,#25125,#25126,#25127,#25128,
#25129,#25130,#25131,#25132,#25133,#25134,#25135,#25136,#25137,#25138,#25139,
#25140,#25141,#25142,#25143,#25144,#25145,#25146,#25147,#25148,#25149,#25150,
#25151,#25152,#25153,#25154,#25155,#25156,#25157,#25158,#25159,#25160,#25161,
#25162,#25163,#25164,#25165,#25166,#25167,#25168,#25169,#25170,#25171,#25172,
#25173,#25174,#25175,#25176,#25177,#25178,#25179,#25180,#25181,#25182,#25183),
(#25184,#25185,#25186,#25187,#25188,#25189,#25190,#25191,#25192,#25193,
#25194,#25195,#25196,#25197,#25198,#25199,#25200,#25201,#25202,#25203,#25204,
#25205,#25206,#25207,#25208,#25209,#25210,#25211,#25212,#25213,#25214,#25215,
#25216,#25217,#25218,#25219,#25220,#25221,#25222,#25223,#25224,#25225,#25226,
#25227,#25228,#25229,#25230,#25231,#25232,#25233,#25234,#25235,#25236,#25237,
#25238,#25239,#25240,#25241,#25242,#25243,#25244,#25245,#25246,#25247,#25248,
#25249,#25250,#25251,#25252,#25253,#25254,#25255,#25256,#25257,#25258,#25259,
#25260,#25261,#25262,#25263,#25264,#25265,#25266,#25267,#25268,#25269,#25270,
#25271,#25272,#25273,#25274,#25275,#25276,#25277,#25278,#25279,#25280,#25281,
#25282,#25283,#25284,#25285,#25286,#25287,#25288,#25289,#25290,#25291,#25292,
#25293,#25294,#25295,#25296,#25297,#25298,#25299,#25300,#25301,#25302,#25303,
#25304,#25305,#25306,#25307,#25308,#25309,#25310,#25311,#25312,#25313,#25314,
#25315,#25316,#25317,#25318,#25319,#25320,#25321,#25322,#25323,#25324,#25325,
#25326,#25327,#25328,#25329,#25330,#25331,#25332,#25333,#25334,#25335,#25336,
#25337,#25338,#25339,#25340,#25341,#25342,#25343,#25344)),.UNSPECIFIED.,
 .F.,.F.,.F.)
B_SPLINE_SURFACE_WITH_KNOTS((2,2),(3,2,2,2,2,2,2,2,2,2,2,2,2,2,2,2,2,2,
2,2,2,2,2,2,2,2,2,2,2,2,2,2,2,2,2,2,2,2,2,2,2,2,2,2,2,2,2,2,2,2,2,2,2,2,
2,2,2,2,2,2,2,2,2,2,2,2,2,2,2,2,2,2,2,2,2,2,2,2,2,2,3),(0.,1.),(0.,0.0125,
0.025,0.0375,0.05,0.0625,0.075,0.0875,0.1,0.1125,0.125,0.1375,0.15,0.1625,
0.175,0.1875,0.2,0.2125,0.225,0.2375,0.25,0.2625,0.275,0.2875,0.3,0.3125,
0.325,0.3375,0.35,0.3625,0.375,0.3875,0.4,0.4125,0.425,0.4375,0.45,0.4625,
0.475,0.4875,0.5,0.5125,0.525,0.5375,0.55,0.5625,0.575,0.5875,0.6,0.6125,
0.625,0.6375,0.65,0.6625,0.675,0.6875,0.7,0.7125,0.725,0.7375,0.75,0.7625,
0.775,0.7875,0.8,0.8125,0.825,0.8375,0.85,0.8625,0.875,0.8875,0.9,0.9125,
0.925,0.9375,0.95,0.9625,0.975,0.9875,1.),.UNSPECIFIED.)
GEOMETRIC_REPRESENTATION_ITEM()
RATIONAL_B_SPLINE_SURFACE(((1.,0.923879532511287,1.,0.923879532511287,1.,
0.923879532511287,1.,0.923879532511287,1.,0.923879532511287,1.,0.923879532511287,
1.,0.923879532511287,1.,0.923879532511287,1.,0.923879532511287,1.,0.923879532511287,
1.,0.923879532511287,1.,0.923879532511287,1.,0.923879532511287,1.,0.923879532511287,
1.,0.923879532511287,1.,0.923879532511287,1.,0.923879532511287,1.,0.923879532511287,
1.,0.923879532511287,1.,0.923879532511287,1.,0.923879532511287,1.,0.923879532511287,
1.,0.923879532511287,1.,0.923879532511287,1.,0.923879532511287,1.,0.923879532511287,
1.,0.923879532511287,1.,0.923879532511287,1.,0.923879532511287,1.,0.923879532511287,
1.,0.923879532511287,1.,0.923879532511287,1.,0.923879532511287,1.,0.923879532511287,
1.,0.923879532511287,1.,0.923879532511287,1.,0.923879532511287,1.,0.923879532511287,
1.,0.923879532511287,1.,0.923879532511287,1.,0.923879532511287,1.,0.923879532511287,
1.,0.923879532511287,1.,0.923879532511287,1.,0.923879532511287,1.,0.923879532511287,
1.,0.923879532511287,1.,0.923879532511287,1.,0.923879532511287,1.,0.923879532511287,
1.,0.923879532511287,1.,0.923879532511287,1.,0.923879532511287,1.,0.923879532511287,
1.,0.923879532511287,1.,0.923879532511287,1.,0.923879532511287,1.,0.923879532511287,
1.,0.923879532511287,1.,0.923879532511287,1.,0.923879532511287,1.,0.923879532511287,
1.,0.923879532511287,1.,0.923879532511287,1.,0.923879532511287,1.,0.923879532511287,
1.,0.923879532511287,1.,0.923879532511287,1.,0.923879532511287,1.,0.923879532511287,
1.,0.923879532511287,1.,0.923879532511287,1.,0.923879532511287,1.,0.923879532511287,
1.,0.923879532511287,1.,0.923879532511287,1.,0.923879532511287,1.,0.923879532511287,
1.,0.923879532511287,1.,0.923879532511287,1.),(1.,0.923879532511287,1.,
0.923879532511287,1.,0.923879532511287,1.,0.923879532511287,1.,0.923879532511287,
1.,0.923879532511287,1.,0.923879532511287,1.,0.923879532511287,1.,0.923879532511287,
1.,0.923879532511287,1.,0.923879532511287,1.,0.923879532511287,1.,0.923879532511287,
1.,0.923879532511287,1.,0.923879532511287,1.,0.923879532511287,1.,0.923879532511287,
1.,0.923879532511287,1.,0.923879532511287,1.,0.923879532511287,1.,0.923879532511287,
1.,0.923879532511287,1.,0.923879532511287,1.,0.923879532511287,1.,0.923879532511287,
1.,0.923879532511287,1.,0.923879532511287,1.,0.923879532511287,1.,0.923879532511287,
1.,0.923879532511287,1.,0.923879532511287,1.,0.923879532511287,1.,0.923879532511287,
1.,0.923879532511287,1.,0.923879532511287,1.,0.923879532511287,1.,0.923879532511287,
1.,0.923879532511287,1.,0.923879532511287,1.,0.923879532511287,1.,0.923879532511287,
1.,0.923879532511287,1.,0.923879532511287,1.,0.923879532511287,1.,0.923879532511287,
1.,0.923879532511287,1.,0.923879532511287,1.,0.923879532511287,1.,0.923879532511287,
1.,0.923879532511287,1.,0.923879532511287,1.,0.923879532511287,1.,0.923879532511287,
1.,0.923879532511287,1.,0.923879532511287,1.,0.923879532511287,1.,0.923879532511287,
1.,0.923879532511287,1.,0.923879532511287,1.,0.923879532511287,1.,0.923879532511287,
1.,0.923879532511287,1.,0.923879532511287,1.,0.923879532511287,1.,0.923879532511287,
1.,0.923879532511287,1.,0.923879532511287,1.,0.923879532511287,1.,0.923879532511287,
1.,0.923879532511287,1.,0.923879532511287,1.,0.923879532511287,1.,0.923879532511287,
1.,0.923879532511287,1.,0.923879532511287,1.,0.923879532511287,1.,0.923879532511287,
1.,0.923879532511287,1.,0.923879532511287,1.,0.923879532511287,1.)))
REPRESENTATION_ITEM('')
SURFACE()
);
#568=(
BOUNDED_SURFACE()
B_SPLINE_SURFACE(3,2,((#25362,#25363,#25364,#25365,#25366,#25367,#25368,
#25369,#25370,#25371,#25372,#25373,#25374,#25375,#25376,#25377,#25378,#25379,
#25380,#25381,#25382,#25383,#25384,#25385,#25386,#25387,#25388,#25389,#25390,
#25391,#25392,#25393,#25394,#25395,#25396,#25397,#25398,#25399,#25400,#25401,
#25402,#25403,#25404,#25405,#25406,#25407,#25408,#25409,#25410,#25411,#25412,
#25413,#25414,#25415,#25416,#25417,#25418,#25419,#25420,#25421,#25422,#25423,
#25424,#25425,#25426,#25427,#25428,#25429,#25430,#25431,#25432,#25433,#25434,
#25435,#25436,#25437,#25438,#25439,#25440,#25441,#25442,#25443,#25444,#25445,
#25446,#25447,#25448,#25449,#25450,#25451,#25452,#25453,#25454,#25455,#25456,
#25457,#25458,#25459,#25460,#25461,#25462,#25463,#25464,#25465,#25466,#25467,
#25468,#25469,#25470,#25471,#25472,#25473,#25474,#25475,#25476,#25477,#25478,
#25479,#25480,#25481,#25482,#25483,#25484,#25485,#25486,#25487,#25488,#25489,
#25490,#25491,#25492,#25493,#25494,#25495,#25496,#25497,#25498,#25499,#25500,
#25501,#25502,#25503,#25504,#25505,#25506,#25507,#25508,#25509,#25510,#25511,
#25512,#25513,#25514,#25515,#25516,#25517,#25518,#25519,#25520,#25521,#25522),
(#25523,#25524,#25525,#25526,#25527,#25528,#25529,#25530,#25531,#25532,
#25533,#25534,#25535,#25536,#25537,#25538,#25539,#25540,#25541,#25542,#25543,
#25544,#25545,#25546,#25547,#25548,#25549,#25550,#25551,#25552,#25553,#25554,
#25555,#25556,#25557,#25558,#25559,#25560,#25561,#25562,#25563,#25564,#25565,
#25566,#25567,#25568,#25569,#25570,#25571,#25572,#25573,#25574,#25575,#25576,
#25577,#25578,#25579,#25580,#25581,#25582,#25583,#25584,#25585,#25586,#25587,
#25588,#25589,#25590,#25591,#25592,#25593,#25594,#25595,#25596,#25597,#25598,
#25599,#25600,#25601,#25602,#25603,#25604,#25605,#25606,#25607,#25608,#25609,
#25610,#25611,#25612,#25613,#25614,#25615,#25616,#25617,#25618,#25619,#25620,
#25621,#25622,#25623,#25624,#25625,#25626,#25627,#25628,#25629,#25630,#25631,
#25632,#25633,#25634,#25635,#25636,#25637,#25638,#25639,#25640,#25641,#25642,
#25643,#25644,#25645,#25646,#25647,#25648,#25649,#25650,#25651,#25652,#25653,
#25654,#25655,#25656,#25657,#25658,#25659,#25660,#25661,#25662,#25663,#25664,
#25665,#25666,#25667,#25668,#25669,#25670,#25671,#25672,#25673,#25674,#25675,
#25676,#25677,#25678,#25679,#25680,#25681,#25682,#25683),(#25684,#25685,
#25686,#25687,#25688,#25689,#25690,#25691,#25692,#25693,#25694,#25695,#25696,
#25697,#25698,#25699,#25700,#25701,#25702,#25703,#25704,#25705,#25706,#25707,
#25708,#25709,#25710,#25711,#25712,#25713,#25714,#25715,#25716,#25717,#25718,
#25719,#25720,#25721,#25722,#25723,#25724,#25725,#25726,#25727,#25728,#25729,
#25730,#25731,#25732,#25733,#25734,#25735,#25736,#25737,#25738,#25739,#25740,
#25741,#25742,#25743,#25744,#25745,#25746,#25747,#25748,#25749,#25750,#25751,
#25752,#25753,#25754,#25755,#25756,#25757,#25758,#25759,#25760,#25761,#25762,
#25763,#25764,#25765,#25766,#25767,#25768,#25769,#25770,#25771,#25772,#25773,
#25774,#25775,#25776,#25777,#25778,#25779,#25780,#25781,#25782,#25783,#25784,
#25785,#25786,#25787,#25788,#25789,#25790,#25791,#25792,#25793,#25794,#25795,
#25796,#25797,#25798,#25799,#25800,#25801,#25802,#25803,#25804,#25805,#25806,
#25807,#25808,#25809,#25810,#25811,#25812,#25813,#25814,#25815,#25816,#25817,
#25818,#25819,#25820,#25821,#25822,#25823,#25824,#25825,#25826,#25827,#25828,
#25829,#25830,#25831,#25832,#25833,#25834,#25835,#25836,#25837,#25838,#25839,
#25840,#25841,#25842,#25843,#25844),(#25845,#25846,#25847,#25848,#25849,
#25850,#25851,#25852,#25853,#25854,#25855,#25856,#25857,#25858,#25859,#25860,
#25861,#25862,#25863,#25864,#25865,#25866,#25867,#25868,#25869,#25870,#25871,
#25872,#25873,#25874,#25875,#25876,#25877,#25878,#25879,#25880,#25881,#25882,
#25883,#25884,#25885,#25886,#25887,#25888,#25889,#25890,#25891,#25892,#25893,
#25894,#25895,#25896,#25897,#25898,#25899,#25900,#25901,#25902,#25903,#25904,
#25905,#25906,#25907,#25908,#25909,#25910,#25911,#25912,#25913,#25914,#25915,
#25916,#25917,#25918,#25919,#25920,#25921,#25922,#25923,#25924,#25925,#25926,
#25927,#25928,#25929,#25930,#25931,#25932,#25933,#25934,#25935,#25936,#25937,
#25938,#25939,#25940,#25941,#25942,#25943,#25944,#25945,#25946,#25947,#25948,
#25949,#25950,#25951,#25952,#25953,#25954,#25955,#25956,#25957,#25958,#25959,
#25960,#25961,#25962,#25963,#25964,#25965,#25966,#25967,#25968,#25969,#25970,
#25971,#25972,#25973,#25974,#25975,#25976,#25977,#25978,#25979,#25980,#25981,
#25982,#25983,#25984,#25985,#25986,#25987,#25988,#25989,#25990,#25991,#25992,
#25993,#25994,#25995,#25996,#25997,#25998,#25999,#26000,#26001,#26002,#26003,
#26004,#26005)),.UNSPECIFIED.,.F.,.F.,.F.)
B_SPLINE_SURFACE_WITH_KNOTS((4,4),(3,2,2,2,2,2,2,2,2,2,2,2,2,2,2,2,2,2,
2,2,2,2,2,2,2,2,2,2,2,2,2,2,2,2,2,2,2,2,2,2,2,2,2,2,2,2,2,2,2,2,2,2,2,2,
2,2,2,2,2,2,2,2,2,2,2,2,2,2,2,2,2,2,2,2,2,2,2,2,2,2,3),(0.,1.),(0.,0.0125,
0.025,0.0375,0.05,0.0625,0.075,0.0875,0.1,0.1125,0.125,0.1375,0.15,0.1625,
0.175,0.1875,0.2,0.2125,0.225,0.2375,0.25,0.2625,0.275,0.2875,0.3,0.3125,
0.325,0.3375,0.35,0.3625,0.375,0.3875,0.4,0.4125,0.425,0.4375,0.45,0.4625,
0.475,0.4875,0.5,0.5125,0.525,0.5375,0.55,0.5625,0.575,0.5875,0.6,0.6125,
0.625,0.6375,0.65,0.6625,0.675,0.6875,0.7,0.7125,0.725,0.7375,0.75,0.7625,
0.775,0.7875,0.8,0.8125,0.825,0.8375,0.85,0.8625,0.875,0.8875,0.9,0.9125,
0.925,0.9375,0.95,0.9625,0.975,0.9875,1.),.UNSPECIFIED.)
GEOMETRIC_REPRESENTATION_ITEM()
RATIONAL_B_SPLINE_SURFACE(((1.,0.923879532511287,1.,0.923879532511287,1.,
0.923879532511287,1.,0.923879532511287,1.,0.923879532511287,1.,0.923879532511287,
1.,0.923879532511287,1.,0.923879532511287,1.,0.923879532511287,1.,0.923879532511287,
1.,0.923879532511287,1.,0.923879532511287,1.,0.923879532511287,1.,0.923879532511287,
1.,0.923879532511287,1.,0.923879532511287,1.,0.923879532511287,1.,0.923879532511287,
1.,0.923879532511287,1.,0.923879532511287,1.,0.923879532511287,1.,0.923879532511287,
1.,0.923879532511287,1.,0.923879532511287,1.,0.923879532511287,1.,0.923879532511287,
1.,0.923879532511287,1.,0.923879532511287,1.,0.923879532511287,1.,0.923879532511287,
1.,0.923879532511287,1.,0.923879532511287,1.,0.923879532511287,1.,0.923879532511287,
1.,0.923879532511287,1.,0.923879532511287,1.,0.923879532511287,1.,0.923879532511287,
1.,0.923879532511287,1.,0.923879532511287,1.,0.923879532511287,1.,0.923879532511287,
1.,0.923879532511287,1.,0.923879532511287,1.,0.923879532511287,1.,0.923879532511287,
1.,0.923879532511287,1.,0.923879532511287,1.,0.923879532511287,1.,0.923879532511287,
1.,0.923879532511287,1.,0.923879532511287,1.,0.923879532511287,1.,0.923879532511287,
1.,0.923879532511287,1.,0.923879532511287,1.,0.923879532511287,1.,0.923879532511287,
1.,0.923879532511287,1.,0.923879532511287,1.,0.923879532511287,1.,0.923879532511287,
1.,0.923879532511287,1.,0.923879532511287,1.,0.923879532511287,1.,0.923879532511287,
1.,0.923879532511287,1.,0.923879532511287,1.,0.923879532511287,1.,0.923879532511287,
1.,0.923879532511287,1.,0.923879532511287,1.,0.923879532511287,1.,0.923879532511287,
1.,0.923879532511287,1.,0.923879532511287,1.,0.923879532511287,1.,0.923879532511287,
1.,0.923879532511287,1.,0.923879532511287,1.),(0.998696642611305,0.922675387296324,
0.998696642611305,0.922675387296324,0.998696642611305,0.922675387296324,
0.998696642611305,0.922675387296324,0.998696642611305,0.922675387296324,
0.998696642611305,0.922675387296324,0.998696642611305,0.922675387296324,
0.998696642611305,0.922675387296324,0.998696642611305,0.922675387296324,
0.998696642611305,0.922675387296324,0.998696642611305,0.922675387296324,
0.998696642611305,0.922675387296324,0.998696642611305,0.922675387296324,
0.998696642611305,0.922675387296324,0.998696642611305,0.922675387296324,
0.998696642611305,0.922675387296324,0.998696642611305,0.922675387296324,
0.998696642611305,0.922675387296324,0.998696642611305,0.922675387296324,
0.998696642611305,0.922675387296324,0.998696642611305,0.922675387296324,
0.998696642611305,0.922675387296324,0.998696642611305,0.922675387296324,
0.998696642611305,0.922675387296324,0.998696642611305,0.922675387296324,
0.998696642611305,0.922675387296324,0.998696642611305,0.922675387296324,
0.998696642611305,0.922675387296324,0.998696642611305,0.922675387296324,
0.998696642611305,0.922675387296324,0.998696642611305,0.922675387296324,
0.998696642611305,0.922675387296324,0.998696642611305,0.922675387296324,
0.998696642611305,0.922675387296324,0.998696642611305,0.922675387296324,
0.998696642611305,0.922675387296324,0.998696642611305,0.922675387296324,
0.998696642611305,0.922675387296324,0.998696642611305,0.922675387296324,
0.998696642611305,0.922675387296324,0.998696642611305,0.922675387296324,
0.998696642611305,0.922675387296324,0.998696642611305,0.922675387296324,
0.998696642611305,0.922675387296324,0.998696642611305,0.922675387296324,
0.998696642611305,0.922675387296324,0.998696642611305,0.922675387296324,
0.998696642611305,0.922675387296324,0.998696642611305,0.922675387296324,
0.998696642611305,0.922675387296324,0.998696642611305,0.922675387296324,
0.998696642611305,0.922675387296324,0.998696642611305,0.922675387296324,
0.998696642611305,0.922675387296324,0.998696642611305,0.922675387296324,
0.998696642611305,0.922675387296324,0.998696642611305,0.922675387296324,
0.998696642611305,0.922675387296324,0.998696642611305,0.922675387296324,
0.998696642611305,0.922675387296324,0.998696642611305,0.922675387296324,
0.998696642611305,0.922675387296324,0.998696642611305,0.922675387296324,
0.998696642611305,0.922675387296324,0.998696642611305,0.922675387296324,
0.998696642611305,0.922675387296324,0.998696642611305,0.922675387296324,
0.998696642611305,0.922675387296324,0.998696642611305,0.922675387296324,
0.998696642611305,0.922675387296324,0.998696642611305,0.922675387296324,
0.998696642611305,0.922675387296324,0.998696642611305,0.922675387296324,
0.998696642611305,0.922675387296324,0.998696642611305,0.922675387296324,
0.998696642611305,0.922675387296324,0.998696642611305,0.922675387296324,
0.998696642611305,0.922675387296324,0.998696642611305,0.922675387296324,
0.998696642611305,0.922675387296324,0.998696642611305),(0.998696642611305,
0.922675387296324,0.998696642611305,0.922675387296324,0.998696642611305,
0.922675387296324,0.998696642611305,0.922675387296324,0.998696642611305,
0.922675387296324,0.998696642611305,0.922675387296324,0.998696642611305,
0.922675387296324,0.998696642611305,0.922675387296324,0.998696642611305,
0.922675387296324,0.998696642611305,0.922675387296324,0.998696642611305,
0.922675387296324,0.998696642611305,0.922675387296324,0.998696642611305,
0.922675387296324,0.998696642611305,0.922675387296324,0.998696642611305,
0.922675387296324,0.998696642611305,0.922675387296324,0.998696642611305,
0.922675387296324,0.998696642611305,0.922675387296324,0.998696642611305,
0.922675387296324,0.998696642611305,0.922675387296324,0.998696642611305,
0.922675387296324,0.998696642611305,0.922675387296324,0.998696642611305,
0.922675387296324,0.998696642611305,0.922675387296324,0.998696642611305,
0.922675387296324,0.998696642611305,0.922675387296324,0.998696642611305,
0.922675387296324,0.998696642611305,0.922675387296324,0.998696642611305,
0.922675387296324,0.998696642611305,0.922675387296324,0.998696642611305,
0.922675387296324,0.998696642611305,0.922675387296324,0.998696642611305,
0.922675387296324,0.998696642611305,0.922675387296324,0.998696642611305,
0.922675387296324,0.998696642611305,0.922675387296324,0.998696642611305,
0.922675387296324,0.998696642611305,0.922675387296324,0.998696642611305,
0.922675387296324,0.998696642611305,0.922675387296324,0.998696642611305,
0.922675387296324,0.998696642611305,0.922675387296324,0.998696642611305,
0.922675387296324,0.998696642611305,0.922675387296324,0.998696642611305,
0.922675387296324,0.998696642611305,0.922675387296324,0.998696642611305,
0.922675387296324,0.998696642611305,0.922675387296324,0.998696642611305,
0.922675387296324,0.998696642611305,0.922675387296324,0.998696642611305,
0.922675387296324,0.998696642611305,0.922675387296324,0.998696642611305,
0.922675387296324,0.998696642611305,0.922675387296324,0.998696642611305,
0.922675387296324,0.998696642611305,0.922675387296324,0.998696642611305,
0.922675387296324,0.998696642611305,0.922675387296324,0.998696642611305,
0.922675387296324,0.998696642611305,0.922675387296324,0.998696642611305,
0.922675387296324,0.998696642611305,0.922675387296324,0.998696642611305,
0.922675387296324,0.998696642611305,0.922675387296324,0.998696642611305,
0.922675387296324,0.998696642611305,0.922675387296324,0.998696642611305,
0.922675387296324,0.998696642611305,0.922675387296324,0.998696642611305,
0.922675387296324,0.998696642611305,0.922675387296324,0.998696642611305,
0.922675387296324,0.998696642611305,0.922675387296324,0.998696642611305,
0.922675387296324,0.998696642611305,0.922675387296324,0.998696642611305,
0.922675387296324,0.998696642611305,0.922675387296324,0.998696642611305,
0.922675387296324,0.998696642611305,0.922675387296324,0.998696642611305,
0.922675387296324,0.998696642611305,0.922675387296324,0.998696642611305),
(1.,0.923879532511287,1.,0.923879532511287,1.,0.923879532511287,1.,0.923879532511287,
1.,0.923879532511287,1.,0.923879532511287,1.,0.923879532511287,1.,0.923879532511287,
1.,0.923879532511287,1.,0.923879532511287,1.,0.923879532511287,1.,0.923879532511287,
1.,0.923879532511287,1.,0.923879532511287,1.,0.923879532511287,1.,0.923879532511287,
1.,0.923879532511287,1.,0.923879532511287,1.,0.923879532511287,1.,0.923879532511287,
1.,0.923879532511287,1.,0.923879532511287,1.,0.923879532511287,1.,0.923879532511287,
1.,0.923879532511287,1.,0.923879532511287,1.,0.923879532511287,1.,0.923879532511287,
1.,0.923879532511287,1.,0.923879532511287,1.,0.923879532511287,1.,0.923879532511287,
1.,0.923879532511287,1.,0.923879532511287,1.,0.923879532511287,1.,0.923879532511287,
1.,0.923879532511287,1.,0.923879532511287,1.,0.923879532511287,1.,0.923879532511287,
1.,0.923879532511287,1.,0.923879532511287,1.,0.923879532511287,1.,0.923879532511287,
1.,0.923879532511287,1.,0.923879532511287,1.,0.923879532511287,1.,0.923879532511287,
1.,0.923879532511287,1.,0.923879532511287,1.,0.923879532511287,1.,0.923879532511287,
1.,0.923879532511287,1.,0.923879532511287,1.,0.923879532511287,1.,0.923879532511287,
1.,0.923879532511287,1.,0.923879532511287,1.,0.923879532511287,1.,0.923879532511287,
1.,0.923879532511287,1.,0.923879532511287,1.,0.923879532511287,1.,0.923879532511287,
1.,0.923879532511287,1.,0.923879532511287,1.,0.923879532511287,1.,0.923879532511287,
1.,0.923879532511287,1.,0.923879532511287,1.,0.923879532511287,1.,0.923879532511287,
1.,0.923879532511287,1.,0.923879532511287,1.,0.923879532511287,1.,0.923879532511287,
1.,0.923879532511287,1.,0.923879532511287,1.,0.923879532511287,1.,0.923879532511287,
1.)))
REPRESENTATION_ITEM('')
SURFACE()
);
#569=(
BOUNDED_SURFACE()
B_SPLINE_SURFACE(1,2,((#26006,#26007,#26008,#26009,#26010,#26011,#26012,
#26013,#26014,#26015,#26016,#26017,#26018,#26019,#26020,#26021,#26022,#26023,
#26024,#26025,#26026,#26027,#26028,#26029,#26030,#26031,#26032,#26033,#26034,
#26035,#26036,#26037,#26038,#26039,#26040,#26041,#26042,#26043,#26044,#26045,
#26046,#26047,#26048,#26049,#26050,#26051,#26052,#26053,#26054,#26055,#26056,
#26057,#26058,#26059,#26060,#26061,#26062,#26063,#26064,#26065,#26066,#26067,
#26068,#26069,#26070,#26071,#26072,#26073,#26074,#26075,#26076,#26077,#26078,
#26079,#26080,#26081,#26082,#26083,#26084,#26085,#26086,#26087,#26088,#26089,
#26090,#26091,#26092,#26093,#26094,#26095,#26096,#26097,#26098,#26099,#26100,
#26101,#26102,#26103,#26104,#26105,#26106,#26107,#26108,#26109,#26110,#26111,
#26112,#26113,#26114,#26115,#26116,#26117,#26118,#26119,#26120,#26121,#26122,
#26123,#26124,#26125,#26126,#26127,#26128,#26129,#26130,#26131,#26132,#26133,
#26134,#26135,#26136,#26137,#26138,#26139,#26140,#26141,#26142,#26143,#26144,
#26145,#26146,#26147,#26148,#26149,#26150,#26151,#26152,#26153,#26154,#26155,
#26156,#26157,#26158,#26159,#26160,#26161,#26162,#26163,#26164,#26165,#26166),
(#26167,#26168,#26169,#26170,#26171,#26172,#26173,#26174,#26175,#26176,
#26177,#26178,#26179,#26180,#26181,#26182,#26183,#26184,#26185,#26186,#26187,
#26188,#26189,#26190,#26191,#26192,#26193,#26194,#26195,#26196,#26197,#26198,
#26199,#26200,#26201,#26202,#26203,#26204,#26205,#26206,#26207,#26208,#26209,
#26210,#26211,#26212,#26213,#26214,#26215,#26216,#26217,#26218,#26219,#26220,
#26221,#26222,#26223,#26224,#26225,#26226,#26227,#26228,#26229,#26230,#26231,
#26232,#26233,#26234,#26235,#26236,#26237,#26238,#26239,#26240,#26241,#26242,
#26243,#26244,#26245,#26246,#26247,#26248,#26249,#26250,#26251,#26252,#26253,
#26254,#26255,#26256,#26257,#26258,#26259,#26260,#26261,#26262,#26263,#26264,
#26265,#26266,#26267,#26268,#26269,#26270,#26271,#26272,#26273,#26274,#26275,
#26276,#26277,#26278,#26279,#26280,#26281,#26282,#26283,#26284,#26285,#26286,
#26287,#26288,#26289,#26290,#26291,#26292,#26293,#26294,#26295,#26296,#26297,
#26298,#26299,#26300,#26301,#26302,#26303,#26304,#26305,#26306,#26307,#26308,
#26309,#26310,#26311,#26312,#26313,#26314,#26315,#26316,#26317,#26318,#26319,
#26320,#26321,#26322,#26323,#26324,#26325,#26326,#26327)),.UNSPECIFIED.,
 .F.,.F.,.F.)
B_SPLINE_SURFACE_WITH_KNOTS((2,2),(3,2,2,2,2,2,2,2,2,2,2,2,2,2,2,2,2,2,
2,2,2,2,2,2,2,2,2,2,2,2,2,2,2,2,2,2,2,2,2,2,2,2,2,2,2,2,2,2,2,2,2,2,2,2,
2,2,2,2,2,2,2,2,2,2,2,2,2,2,2,2,2,2,2,2,2,2,2,2,2,2,3),(0.,1.),(0.,0.0125,
0.025,0.0375,0.05,0.0625,0.075,0.0875,0.1,0.1125,0.125,0.1375,0.15,0.1625,
0.175,0.1875,0.2,0.2125,0.225,0.2375,0.25,0.2625,0.275,0.2875,0.3,0.3125,
0.325,0.3375,0.35,0.3625,0.375,0.3875,0.4,0.4125,0.425,0.4375,0.45,0.4625,
0.475,0.4875,0.5,0.5125,0.525,0.5375,0.55,0.5625,0.575,0.5875,0.6,0.6125,
0.625,0.6375,0.65,0.6625,0.675,0.6875,0.7,0.7125,0.725,0.7375,0.75,0.7625,
0.775,0.7875,0.8,0.8125,0.825,0.8375,0.85,0.8625,0.875,0.8875,0.9,0.9125,
0.925,0.9375,0.95,0.9625,0.975,0.9875,1.),.UNSPECIFIED.)
GEOMETRIC_REPRESENTATION_ITEM()
RATIONAL_B_SPLINE_SURFACE(((1.,0.923879532511287,1.,0.923879532511287,1.,
0.923879532511287,1.,0.923879532511287,1.,0.923879532511287,1.,0.923879532511287,
1.,0.923879532511287,1.,0.923879532511287,1.,0.923879532511287,1.,0.923879532511287,
1.,0.923879532511287,1.,0.923879532511287,1.,0.923879532511287,1.,0.923879532511287,
1.,0.923879532511287,1.,0.923879532511287,1.,0.923879532511287,1.,0.923879532511287,
1.,0.923879532511287,1.,0.923879532511287,1.,0.923879532511287,1.,0.923879532511287,
1.,0.923879532511287,1.,0.923879532511287,1.,0.923879532511287,1.,0.923879532511287,
1.,0.923879532511287,1.,0.923879532511287,1.,0.923879532511287,1.,0.923879532511287,
1.,0.923879532511287,1.,0.923879532511287,1.,0.923879532511287,1.,0.923879532511287,
1.,0.923879532511287,1.,0.923879532511287,1.,0.923879532511287,1.,0.923879532511287,
1.,0.923879532511287,1.,0.923879532511287,1.,0.923879532511287,1.,0.923879532511287,
1.,0.923879532511287,1.,0.923879532511287,1.,0.923879532511287,1.,0.923879532511287,
1.,0.923879532511287,1.,0.923879532511287,1.,0.923879532511287,1.,0.923879532511287,
1.,0.923879532511287,1.,0.923879532511287,1.,0.923879532511287,1.,0.923879532511287,
1.,0.923879532511287,1.,0.923879532511287,1.,0.923879532511287,1.,0.923879532511287,
1.,0.923879532511287,1.,0.923879532511287,1.,0.923879532511287,1.,0.923879532511287,
1.,0.923879532511287,1.,0.923879532511287,1.,0.923879532511287,1.,0.923879532511287,
1.,0.923879532511287,1.,0.923879532511287,1.,0.923879532511287,1.,0.923879532511287,
1.,0.923879532511287,1.,0.923879532511287,1.,0.923879532511287,1.,0.923879532511287,
1.,0.923879532511287,1.,0.923879532511287,1.,0.923879532511287,1.,0.923879532511287,
1.,0.923879532511287,1.,0.923879532511287,1.),(1.,0.923879532511287,1.,
0.923879532511287,1.,0.923879532511287,1.,0.923879532511287,1.,0.923879532511287,
1.,0.923879532511287,1.,0.923879532511287,1.,0.923879532511287,1.,0.923879532511287,
1.,0.923879532511287,1.,0.923879532511287,1.,0.923879532511287,1.,0.923879532511287,
1.,0.923879532511287,1.,0.923879532511287,1.,0.923879532511287,1.,0.923879532511287,
1.,0.923879532511287,1.,0.923879532511287,1.,0.923879532511287,1.,0.923879532511287,
1.,0.923879532511287,1.,0.923879532511287,1.,0.923879532511287,1.,0.923879532511287,
1.,0.923879532511287,1.,0.923879532511287,1.,0.923879532511287,1.,0.923879532511287,
1.,0.923879532511287,1.,0.923879532511287,1.,0.923879532511287,1.,0.923879532511287,
1.,0.923879532511287,1.,0.923879532511287,1.,0.923879532511287,1.,0.923879532511287,
1.,0.923879532511287,1.,0.923879532511287,1.,0.923879532511287,1.,0.923879532511287,
1.,0.923879532511287,1.,0.923879532511287,1.,0.923879532511287,1.,0.923879532511287,
1.,0.923879532511287,1.,0.923879532511287,1.,0.923879532511287,1.,0.923879532511287,
1.,0.923879532511287,1.,0.923879532511287,1.,0.923879532511287,1.,0.923879532511287,
1.,0.923879532511287,1.,0.923879532511287,1.,0.923879532511287,1.,0.923879532511287,
1.,0.923879532511287,1.,0.923879532511287,1.,0.923879532511287,1.,0.923879532511287,
1.,0.923879532511287,1.,0.923879532511287,1.,0.923879532511287,1.,0.923879532511287,
1.,0.923879532511287,1.,0.923879532511287,1.,0.923879532511287,1.,0.923879532511287,
1.,0.923879532511287,1.,0.923879532511287,1.,0.923879532511287,1.,0.923879532511287,
1.,0.923879532511287,1.,0.923879532511287,1.,0.923879532511287,1.,0.923879532511287,
1.,0.923879532511287,1.,0.923879532511287,1.,0.923879532511287,1.)))
REPRESENTATION_ITEM('')
SURFACE()
);
#570=(
BOUNDED_SURFACE()
B_SPLINE_SURFACE(1,2,((#26345,#26346,#26347,#26348,#26349,#26350,#26351,
#26352,#26353,#26354,#26355,#26356,#26357,#26358,#26359,#26360,#26361,#26362,
#26363,#26364,#26365,#26366,#26367,#26368,#26369,#26370,#26371,#26372,#26373,
#26374,#26375,#26376,#26377,#26378,#26379,#26380,#26381,#26382,#26383,#26384,
#26385,#26386,#26387,#26388,#26389,#26390,#26391,#26392,#26393,#26394,#26395,
#26396,#26397,#26398,#26399,#26400,#26401,#26402,#26403,#26404,#26405,#26406,
#26407,#26408,#26409,#26410,#26411,#26412,#26413,#26414,#26415,#26416,#26417,
#26418,#26419,#26420,#26421,#26422,#26423,#26424,#26425,#26426,#26427,#26428,
#26429,#26430,#26431,#26432,#26433,#26434,#26435,#26436,#26437,#26438,#26439,
#26440,#26441,#26442,#26443,#26444,#26445,#26446,#26447,#26448,#26449,#26450,
#26451,#26452,#26453,#26454,#26455,#26456,#26457,#26458,#26459,#26460,#26461,
#26462,#26463,#26464,#26465,#26466,#26467,#26468,#26469,#26470,#26471,#26472,
#26473,#26474,#26475,#26476,#26477,#26478,#26479,#26480,#26481,#26482,#26483,
#26484,#26485,#26486,#26487,#26488,#26489,#26490,#26491,#26492,#26493,#26494,
#26495,#26496,#26497,#26498,#26499,#26500,#26501,#26502,#26503,#26504,#26505),
(#26506,#26507,#26508,#26509,#26510,#26511,#26512,#26513,#26514,#26515,
#26516,#26517,#26518,#26519,#26520,#26521,#26522,#26523,#26524,#26525,#26526,
#26527,#26528,#26529,#26530,#26531,#26532,#26533,#26534,#26535,#26536,#26537,
#26538,#26539,#26540,#26541,#26542,#26543,#26544,#26545,#26546,#26547,#26548,
#26549,#26550,#26551,#26552,#26553,#26554,#26555,#26556,#26557,#26558,#26559,
#26560,#26561,#26562,#26563,#26564,#26565,#26566,#26567,#26568,#26569,#26570,
#26571,#26572,#26573,#26574,#26575,#26576,#26577,#26578,#26579,#26580,#26581,
#26582,#26583,#26584,#26585,#26586,#26587,#26588,#26589,#26590,#26591,#26592,
#26593,#26594,#26595,#26596,#26597,#26598,#26599,#26600,#26601,#26602,#26603,
#26604,#26605,#26606,#26607,#26608,#26609,#26610,#26611,#26612,#26613,#26614,
#26615,#26616,#26617,#26618,#26619,#26620,#26621,#26622,#26623,#26624,#26625,
#26626,#26627,#26628,#26629,#26630,#26631,#26632,#26633,#26634,#26635,#26636,
#26637,#26638,#26639,#26640,#26641,#26642,#26643,#26644,#26645,#26646,#26647,
#26648,#26649,#26650,#26651,#26652,#26653,#26654,#26655,#26656,#26657,#26658,
#26659,#26660,#26661,#26662,#26663,#26664,#26665,#26666)),.UNSPECIFIED.,
 .F.,.F.,.F.)
B_SPLINE_SURFACE_WITH_KNOTS((2,2),(3,2,2,2,2,2,2,2,2,2,2,2,2,2,2,2,2,2,
2,2,2,2,2,2,2,2,2,2,2,2,2,2,2,2,2,2,2,2,2,2,2,2,2,2,2,2,2,2,2,2,2,2,2,2,
2,2,2,2,2,2,2,2,2,2,2,2,2,2,2,2,2,2,2,2,2,2,2,2,2,2,3),(0.,1.),(0.,0.0125,
0.025,0.0375,0.05,0.0625,0.075,0.0875,0.1,0.1125,0.125,0.1375,0.15,0.1625,
0.175,0.1875,0.2,0.2125,0.225,0.2375,0.25,0.2625,0.275,0.2875,0.3,0.3125,
0.325,0.3375,0.35,0.3625,0.375,0.3875,0.4,0.4125,0.425,0.4375,0.45,0.4625,
0.475,0.4875,0.5,0.5125,0.525,0.5375,0.55,0.5625,0.575,0.5875,0.6,0.6125,
0.625,0.6375,0.65,0.6625,0.675,0.6875,0.7,0.7125,0.725,0.7375,0.75,0.7625,
0.775,0.7875,0.8,0.8125,0.825,0.8375,0.85,0.8625,0.875,0.8875,0.9,0.9125,
0.925,0.9375,0.95,0.9625,0.975,0.9875,1.),.UNSPECIFIED.)
GEOMETRIC_REPRESENTATION_ITEM()
RATIONAL_B_SPLINE_SURFACE(((1.,0.923879532511287,1.,0.923879532511287,1.,
0.923879532511287,1.,0.923879532511287,1.,0.923879532511287,1.,0.923879532511287,
1.,0.923879532511287,1.,0.923879532511287,1.,0.923879532511287,1.,0.923879532511287,
1.,0.923879532511287,1.,0.923879532511287,1.,0.923879532511287,1.,0.923879532511287,
1.,0.923879532511287,1.,0.923879532511287,1.,0.923879532511287,1.,0.923879532511287,
1.,0.923879532511287,1.,0.923879532511287,1.,0.923879532511287,1.,0.923879532511287,
1.,0.923879532511287,1.,0.923879532511287,1.,0.923879532511287,1.,0.923879532511287,
1.,0.923879532511287,1.,0.923879532511287,1.,0.923879532511287,1.,0.923879532511287,
1.,0.923879532511287,1.,0.923879532511287,1.,0.923879532511287,1.,0.923879532511287,
1.,0.923879532511287,1.,0.923879532511287,1.,0.923879532511287,1.,0.923879532511287,
1.,0.923879532511287,1.,0.923879532511287,1.,0.923879532511287,1.,0.923879532511287,
1.,0.923879532511287,1.,0.923879532511287,1.,0.923879532511287,1.,0.923879532511287,
1.,0.923879532511287,1.,0.923879532511287,1.,0.923879532511287,1.,0.923879532511287,
1.,0.923879532511287,1.,0.923879532511287,1.,0.923879532511287,1.,0.923879532511287,
1.,0.923879532511287,1.,0.923879532511287,1.,0.923879532511287,1.,0.923879532511287,
1.,0.923879532511287,1.,0.923879532511287,1.,0.923879532511287,1.,0.923879532511287,
1.,0.923879532511287,1.,0.923879532511287,1.,0.923879532511287,1.,0.923879532511287,
1.,0.923879532511287,1.,0.923879532511287,1.,0.923879532511287,1.,0.923879532511287,
1.,0.923879532511287,1.,0.923879532511287,1.,0.923879532511287,1.,0.923879532511287,
1.,0.923879532511287,1.,0.923879532511287,1.,0.923879532511287,1.,0.923879532511287,
1.,0.923879532511287,1.,0.923879532511287,1.),(1.,0.923879532511287,1.,
0.923879532511287,1.,0.923879532511287,1.,0.923879532511287,1.,0.923879532511287,
1.,0.923879532511287,1.,0.923879532511287,1.,0.923879532511287,1.,0.923879532511287,
1.,0.923879532511287,1.,0.923879532511287,1.,0.923879532511287,1.,0.923879532511287,
1.,0.923879532511287,1.,0.923879532511287,1.,0.923879532511287,1.,0.923879532511287,
1.,0.923879532511287,1.,0.923879532511287,1.,0.923879532511287,1.,0.923879532511287,
1.,0.923879532511287,1.,0.923879532511287,1.,0.923879532511287,1.,0.923879532511287,
1.,0.923879532511287,1.,0.923879532511287,1.,0.923879532511287,1.,0.923879532511287,
1.,0.923879532511287,1.,0.923879532511287,1.,0.923879532511287,1.,0.923879532511287,
1.,0.923879532511287,1.,0.923879532511287,1.,0.923879532511287,1.,0.923879532511287,
1.,0.923879532511287,1.,0.923879532511287,1.,0.923879532511287,1.,0.923879532511287,
1.,0.923879532511287,1.,0.923879532511287,1.,0.923879532511287,1.,0.923879532511287,
1.,0.923879532511287,1.,0.923879532511287,1.,0.923879532511287,1.,0.923879532511287,
1.,0.923879532511287,1.,0.923879532511287,1.,0.923879532511287,1.,0.923879532511287,
1.,0.923879532511287,1.,0.923879532511287,1.,0.923879532511287,1.,0.923879532511287,
1.,0.923879532511287,1.,0.923879532511287,1.,0.923879532511287,1.,0.923879532511287,
1.,0.923879532511287,1.,0.923879532511287,1.,0.923879532511287,1.,0.923879532511287,
1.,0.923879532511287,1.,0.923879532511287,1.,0.923879532511287,1.,0.923879532511287,
1.,0.923879532511287,1.,0.923879532511287,1.,0.923879532511287,1.,0.923879532511287,
1.,0.923879532511287,1.,0.923879532511287,1.,0.923879532511287,1.,0.923879532511287,
1.,0.923879532511287,1.,0.923879532511287,1.,0.923879532511287,1.)))
REPRESENTATION_ITEM('')
SURFACE()
);
#571=(
BOUNDED_SURFACE()
B_SPLINE_SURFACE(3,2,((#26684,#26685,#26686,#26687,#26688,#26689,#26690,
#26691,#26692,#26693,#26694,#26695,#26696,#26697,#26698,#26699,#26700,#26701,
#26702,#26703,#26704,#26705,#26706,#26707,#26708,#26709,#26710,#26711,#26712,
#26713,#26714,#26715,#26716,#26717,#26718,#26719,#26720,#26721,#26722,#26723,
#26724,#26725,#26726,#26727,#26728,#26729,#26730,#26731,#26732,#26733,#26734,
#26735,#26736,#26737,#26738,#26739,#26740,#26741,#26742,#26743,#26744,#26745,
#26746,#26747,#26748,#26749,#26750,#26751,#26752,#26753,#26754,#26755,#26756,
#26757,#26758,#26759,#26760,#26761,#26762,#26763,#26764,#26765,#26766,#26767,
#26768,#26769,#26770,#26771,#26772,#26773,#26774,#26775,#26776,#26777,#26778,
#26779,#26780,#26781,#26782,#26783,#26784,#26785,#26786,#26787,#26788,#26789,
#26790,#26791,#26792,#26793,#26794,#26795,#26796,#26797,#26798,#26799,#26800,
#26801,#26802,#26803,#26804,#26805,#26806,#26807,#26808,#26809,#26810,#26811,
#26812,#26813,#26814,#26815,#26816,#26817,#26818,#26819,#26820,#26821,#26822,
#26823,#26824,#26825,#26826,#26827,#26828,#26829,#26830,#26831,#26832,#26833,
#26834,#26835,#26836,#26837,#26838,#26839,#26840,#26841,#26842,#26843,#26844),
(#26845,#26846,#26847,#26848,#26849,#26850,#26851,#26852,#26853,#26854,
#26855,#26856,#26857,#26858,#26859,#26860,#26861,#26862,#26863,#26864,#26865,
#26866,#26867,#26868,#26869,#26870,#26871,#26872,#26873,#26874,#26875,#26876,
#26877,#26878,#26879,#26880,#26881,#26882,#26883,#26884,#26885,#26886,#26887,
#26888,#26889,#26890,#26891,#26892,#26893,#26894,#26895,#26896,#26897,#26898,
#26899,#26900,#26901,#26902,#26903,#26904,#26905,#26906,#26907,#26908,#26909,
#26910,#26911,#26912,#26913,#26914,#26915,#26916,#26917,#26918,#26919,#26920,
#26921,#26922,#26923,#26924,#26925,#26926,#26927,#26928,#26929,#26930,#26931,
#26932,#26933,#26934,#26935,#26936,#26937,#26938,#26939,#26940,#26941,#26942,
#26943,#26944,#26945,#26946,#26947,#26948,#26949,#26950,#26951,#26952,#26953,
#26954,#26955,#26956,#26957,#26958,#26959,#26960,#26961,#26962,#26963,#26964,
#26965,#26966,#26967,#26968,#26969,#26970,#26971,#26972,#26973,#26974,#26975,
#26976,#26977,#26978,#26979,#26980,#26981,#26982,#26983,#26984,#26985,#26986,
#26987,#26988,#26989,#26990,#26991,#26992,#26993,#26994,#26995,#26996,#26997,
#26998,#26999,#27000,#27001,#27002,#27003,#27004,#27005),(#27006,#27007,
#27008,#27009,#27010,#27011,#27012,#27013,#27014,#27015,#27016,#27017,#27018,
#27019,#27020,#27021,#27022,#27023,#27024,#27025,#27026,#27027,#27028,#27029,
#27030,#27031,#27032,#27033,#27034,#27035,#27036,#27037,#27038,#27039,#27040,
#27041,#27042,#27043,#27044,#27045,#27046,#27047,#27048,#27049,#27050,#27051,
#27052,#27053,#27054,#27055,#27056,#27057,#27058,#27059,#27060,#27061,#27062,
#27063,#27064,#27065,#27066,#27067,#27068,#27069,#27070,#27071,#27072,#27073,
#27074,#27075,#27076,#27077,#27078,#27079,#27080,#27081,#27082,#27083,#27084,
#27085,#27086,#27087,#27088,#27089,#27090,#27091,#27092,#27093,#27094,#27095,
#27096,#27097,#27098,#27099,#27100,#27101,#27102,#27103,#27104,#27105,#27106,
#27107,#27108,#27109,#27110,#27111,#27112,#27113,#27114,#27115,#27116,#27117,
#27118,#27119,#27120,#27121,#27122,#27123,#27124,#27125,#27126,#27127,#27128,
#27129,#27130,#27131,#27132,#27133,#27134,#27135,#27136,#27137,#27138,#27139,
#27140,#27141,#27142,#27143,#27144,#27145,#27146,#27147,#27148,#27149,#27150,
#27151,#27152,#27153,#27154,#27155,#27156,#27157,#27158,#27159,#27160,#27161,
#27162,#27163,#27164,#27165,#27166),(#27167,#27168,#27169,#27170,#27171,
#27172,#27173,#27174,#27175,#27176,#27177,#27178,#27179,#27180,#27181,#27182,
#27183,#27184,#27185,#27186,#27187,#27188,#27189,#27190,#27191,#27192,#27193,
#27194,#27195,#27196,#27197,#27198,#27199,#27200,#27201,#27202,#27203,#27204,
#27205,#27206,#27207,#27208,#27209,#27210,#27211,#27212,#27213,#27214,#27215,
#27216,#27217,#27218,#27219,#27220,#27221,#27222,#27223,#27224,#27225,#27226,
#27227,#27228,#27229,#27230,#27231,#27232,#27233,#27234,#27235,#27236,#27237,
#27238,#27239,#27240,#27241,#27242,#27243,#27244,#27245,#27246,#27247,#27248,
#27249,#27250,#27251,#27252,#27253,#27254,#27255,#27256,#27257,#27258,#27259,
#27260,#27261,#27262,#27263,#27264,#27265,#27266,#27267,#27268,#27269,#27270,
#27271,#27272,#27273,#27274,#27275,#27276,#27277,#27278,#27279,#27280,#27281,
#27282,#27283,#27284,#27285,#27286,#27287,#27288,#27289,#27290,#27291,#27292,
#27293,#27294,#27295,#27296,#27297,#27298,#27299,#27300,#27301,#27302,#27303,
#27304,#27305,#27306,#27307,#27308,#27309,#27310,#27311,#27312,#27313,#27314,
#27315,#27316,#27317,#27318,#27319,#27320,#27321,#27322,#27323,#27324,#27325,
#27326,#27327)),.UNSPECIFIED.,.F.,.F.,.F.)
B_SPLINE_SURFACE_WITH_KNOTS((4,4),(3,2,2,2,2,2,2,2,2,2,2,2,2,2,2,2,2,2,
2,2,2,2,2,2,2,2,2,2,2,2,2,2,2,2,2,2,2,2,2,2,2,2,2,2,2,2,2,2,2,2,2,2,2,2,
2,2,2,2,2,2,2,2,2,2,2,2,2,2,2,2,2,2,2,2,2,2,2,2,2,2,3),(0.,1.),(0.,0.0125,
0.025,0.0375,0.05,0.0625,0.075,0.0875,0.1,0.1125,0.125,0.1375,0.15,0.1625,
0.175,0.1875,0.2,0.2125,0.225,0.2375,0.25,0.2625,0.275,0.2875,0.3,0.3125,
0.325,0.3375,0.35,0.3625,0.375,0.3875,0.4,0.4125,0.425,0.4375,0.45,0.4625,
0.475,0.4875,0.5,0.5125,0.525,0.5375,0.55,0.5625,0.575,0.5875,0.6,0.6125,
0.625,0.6375,0.65,0.6625,0.675,0.6875,0.7,0.7125,0.725,0.7375,0.75,0.7625,
0.775,0.7875,0.8,0.8125,0.825,0.8375,0.85,0.8625,0.875,0.8875,0.9,0.9125,
0.925,0.9375,0.95,0.9625,0.975,0.9875,1.),.UNSPECIFIED.)
GEOMETRIC_REPRESENTATION_ITEM()
RATIONAL_B_SPLINE_SURFACE(((1.,0.923879532511287,1.,0.923879532511287,1.,
0.923879532511287,1.,0.923879532511287,1.,0.923879532511287,1.,0.923879532511287,
1.,0.923879532511287,1.,0.923879532511287,1.,0.923879532511287,1.,0.923879532511287,
1.,0.923879532511287,1.,0.923879532511287,1.,0.923879532511287,1.,0.923879532511287,
1.,0.923879532511287,1.,0.923879532511287,1.,0.923879532511287,1.,0.923879532511287,
1.,0.923879532511287,1.,0.923879532511287,1.,0.923879532511287,1.,0.923879532511287,
1.,0.923879532511287,1.,0.923879532511287,1.,0.923879532511287,1.,0.923879532511287,
1.,0.923879532511287,1.,0.923879532511287,1.,0.923879532511287,1.,0.923879532511287,
1.,0.923879532511287,1.,0.923879532511287,1.,0.923879532511287,1.,0.923879532511287,
1.,0.923879532511287,1.,0.923879532511287,1.,0.923879532511287,1.,0.923879532511287,
1.,0.923879532511287,1.,0.923879532511287,1.,0.923879532511287,1.,0.923879532511287,
1.,0.923879532511287,1.,0.923879532511287,1.,0.923879532511287,1.,0.923879532511287,
1.,0.923879532511287,1.,0.923879532511287,1.,0.923879532511287,1.,0.923879532511287,
1.,0.923879532511287,1.,0.923879532511287,1.,0.923879532511287,1.,0.923879532511287,
1.,0.923879532511287,1.,0.923879532511287,1.,0.923879532511287,1.,0.923879532511287,
1.,0.923879532511287,1.,0.923879532511287,1.,0.923879532511287,1.,0.923879532511287,
1.,0.923879532511287,1.,0.923879532511287,1.,0.923879532511287,1.,0.923879532511287,
1.,0.923879532511287,1.,0.923879532511287,1.,0.923879532511287,1.,0.923879532511287,
1.,0.923879532511287,1.,0.923879532511287,1.,0.923879532511287,1.,0.923879532511287,
1.,0.923879532511287,1.,0.923879532511287,1.,0.923879532511287,1.,0.923879532511287,
1.,0.923879532511287,1.,0.923879532511287,1.),(0.998696642611305,0.922675387296324,
0.998696642611305,0.922675387296324,0.998696642611305,0.922675387296324,
0.998696642611305,0.922675387296324,0.998696642611305,0.922675387296324,
0.998696642611305,0.922675387296324,0.998696642611305,0.922675387296324,
0.998696642611305,0.922675387296324,0.998696642611305,0.922675387296324,
0.998696642611305,0.922675387296324,0.998696642611305,0.922675387296324,
0.998696642611305,0.922675387296324,0.998696642611305,0.922675387296324,
0.998696642611305,0.922675387296324,0.998696642611305,0.922675387296324,
0.998696642611305,0.922675387296324,0.998696642611305,0.922675387296324,
0.998696642611305,0.922675387296324,0.998696642611305,0.922675387296324,
0.998696642611305,0.922675387296324,0.998696642611305,0.922675387296324,
0.998696642611305,0.922675387296324,0.998696642611305,0.922675387296324,
0.998696642611305,0.922675387296324,0.998696642611305,0.922675387296324,
0.998696642611305,0.922675387296324,0.998696642611305,0.922675387296324,
0.998696642611305,0.922675387296324,0.998696642611305,0.922675387296324,
0.998696642611305,0.922675387296324,0.998696642611305,0.922675387296324,
0.998696642611305,0.922675387296324,0.998696642611305,0.922675387296324,
0.998696642611305,0.922675387296324,0.998696642611305,0.922675387296324,
0.998696642611305,0.922675387296324,0.998696642611305,0.922675387296324,
0.998696642611305,0.922675387296324,0.998696642611305,0.922675387296324,
0.998696642611305,0.922675387296324,0.998696642611305,0.922675387296324,
0.998696642611305,0.922675387296324,0.998696642611305,0.922675387296324,
0.998696642611305,0.922675387296324,0.998696642611305,0.922675387296324,
0.998696642611305,0.922675387296324,0.998696642611305,0.922675387296324,
0.998696642611305,0.922675387296324,0.998696642611305,0.922675387296324,
0.998696642611305,0.922675387296324,0.998696642611305,0.922675387296324,
0.998696642611305,0.922675387296324,0.998696642611305,0.922675387296324,
0.998696642611305,0.922675387296324,0.998696642611305,0.922675387296324,
0.998696642611305,0.922675387296324,0.998696642611305,0.922675387296324,
0.998696642611305,0.922675387296324,0.998696642611305,0.922675387296324,
0.998696642611305,0.922675387296324,0.998696642611305,0.922675387296324,
0.998696642611305,0.922675387296324,0.998696642611305,0.922675387296324,
0.998696642611305,0.922675387296324,0.998696642611305,0.922675387296324,
0.998696642611305,0.922675387296324,0.998696642611305,0.922675387296324,
0.998696642611305,0.922675387296324,0.998696642611305,0.922675387296324,
0.998696642611305,0.922675387296324,0.998696642611305,0.922675387296324,
0.998696642611305,0.922675387296324,0.998696642611305,0.922675387296324,
0.998696642611305,0.922675387296324,0.998696642611305,0.922675387296324,
0.998696642611305,0.922675387296324,0.998696642611305,0.922675387296324,
0.998696642611305,0.922675387296324,0.998696642611305,0.922675387296324,
0.998696642611305,0.922675387296324,0.998696642611305),(0.998696642611305,
0.922675387296324,0.998696642611305,0.922675387296324,0.998696642611305,
0.922675387296324,0.998696642611305,0.922675387296324,0.998696642611305,
0.922675387296324,0.998696642611305,0.922675387296324,0.998696642611305,
0.922675387296324,0.998696642611305,0.922675387296324,0.998696642611305,
0.922675387296324,0.998696642611305,0.922675387296324,0.998696642611305,
0.922675387296324,0.998696642611305,0.922675387296324,0.998696642611305,
0.922675387296324,0.998696642611305,0.922675387296324,0.998696642611305,
0.922675387296324,0.998696642611305,0.922675387296324,0.998696642611305,
0.922675387296324,0.998696642611305,0.922675387296324,0.998696642611305,
0.922675387296324,0.998696642611305,0.922675387296324,0.998696642611305,
0.922675387296324,0.998696642611305,0.922675387296324,0.998696642611305,
0.922675387296324,0.998696642611305,0.922675387296324,0.998696642611305,
0.922675387296324,0.998696642611305,0.922675387296324,0.998696642611305,
0.922675387296324,0.998696642611305,0.922675387296324,0.998696642611305,
0.922675387296324,0.998696642611305,0.922675387296324,0.998696642611305,
0.922675387296324,0.998696642611305,0.922675387296324,0.998696642611305,
0.922675387296324,0.998696642611305,0.922675387296324,0.998696642611305,
0.922675387296324,0.998696642611305,0.922675387296324,0.998696642611305,
0.922675387296324,0.998696642611305,0.922675387296324,0.998696642611305,
0.922675387296324,0.998696642611305,0.922675387296324,0.998696642611305,
0.922675387296324,0.998696642611305,0.922675387296324,0.998696642611305,
0.922675387296324,0.998696642611305,0.922675387296324,0.998696642611305,
0.922675387296324,0.998696642611305,0.922675387296324,0.998696642611305,
0.922675387296324,0.998696642611305,0.922675387296324,0.998696642611305,
0.922675387296324,0.998696642611305,0.922675387296324,0.998696642611305,
0.922675387296324,0.998696642611305,0.922675387296324,0.998696642611305,
0.922675387296324,0.998696642611305,0.922675387296324,0.998696642611305,
0.922675387296324,0.998696642611305,0.922675387296324,0.998696642611305,
0.922675387296324,0.998696642611305,0.922675387296324,0.998696642611305,
0.922675387296324,0.998696642611305,0.922675387296324,0.998696642611305,
0.922675387296324,0.998696642611305,0.922675387296324,0.998696642611305,
0.922675387296324,0.998696642611305,0.922675387296324,0.998696642611305,
0.922675387296324,0.998696642611305,0.922675387296324,0.998696642611305,
0.922675387296324,0.998696642611305,0.922675387296324,0.998696642611305,
0.922675387296324,0.998696642611305,0.922675387296324,0.998696642611305,
0.922675387296324,0.998696642611305,0.922675387296324,0.998696642611305,
0.922675387296324,0.998696642611305,0.922675387296324,0.998696642611305,
0.922675387296324,0.998696642611305,0.922675387296324,0.998696642611305,
0.922675387296324,0.998696642611305,0.922675387296324,0.998696642611305,
0.922675387296324,0.998696642611305,0.922675387296324,0.998696642611305),
(1.,0.923879532511287,1.,0.923879532511287,1.,0.923879532511287,1.,0.923879532511287,
1.,0.923879532511287,1.,0.923879532511287,1.,0.923879532511287,1.,0.923879532511287,
1.,0.923879532511287,1.,0.923879532511287,1.,0.923879532511287,1.,0.923879532511287,
1.,0.923879532511287,1.,0.923879532511287,1.,0.923879532511287,1.,0.923879532511287,
1.,0.923879532511287,1.,0.923879532511287,1.,0.923879532511287,1.,0.923879532511287,
1.,0.923879532511287,1.,0.923879532511287,1.,0.923879532511287,1.,0.923879532511287,
1.,0.923879532511287,1.,0.923879532511287,1.,0.923879532511287,1.,0.923879532511287,
1.,0.923879532511287,1.,0.923879532511287,1.,0.923879532511287,1.,0.923879532511287,
1.,0.923879532511287,1.,0.923879532511287,1.,0.923879532511287,1.,0.923879532511287,
1.,0.923879532511287,1.,0.923879532511287,1.,0.923879532511287,1.,0.923879532511287,
1.,0.923879532511287,1.,0.923879532511287,1.,0.923879532511287,1.,0.923879532511287,
1.,0.923879532511287,1.,0.923879532511287,1.,0.923879532511287,1.,0.923879532511287,
1.,0.923879532511287,1.,0.923879532511287,1.,0.923879532511287,1.,0.923879532511287,
1.,0.923879532511287,1.,0.923879532511287,1.,0.923879532511287,1.,0.923879532511287,
1.,0.923879532511287,1.,0.923879532511287,1.,0.923879532511287,1.,0.923879532511287,
1.,0.923879532511287,1.,0.923879532511287,1.,0.923879532511287,1.,0.923879532511287,
1.,0.923879532511287,1.,0.923879532511287,1.,0.923879532511287,1.,0.923879532511287,
1.,0.923879532511287,1.,0.923879532511287,1.,0.923879532511287,1.,0.923879532511287,
1.,0.923879532511287,1.,0.923879532511287,1.,0.923879532511287,1.,0.923879532511287,
1.,0.923879532511287,1.,0.923879532511287,1.,0.923879532511287,1.,0.923879532511287,
1.)))
REPRESENTATION_ITEM('')
SURFACE()
);
#572=(
BOUNDED_SURFACE()
B_SPLINE_SURFACE(1,2,((#27328,#27329,#27330,#27331,#27332,#27333,#27334,
#27335,#27336,#27337,#27338,#27339,#27340,#27341,#27342,#27343,#27344,#27345,
#27346,#27347,#27348,#27349,#27350,#27351,#27352,#27353,#27354,#27355,#27356,
#27357,#27358,#27359,#27360,#27361,#27362,#27363,#27364,#27365,#27366,#27367,
#27368,#27369,#27370,#27371,#27372,#27373,#27374,#27375,#27376,#27377,#27378,
#27379,#27380,#27381,#27382,#27383,#27384,#27385,#27386,#27387,#27388,#27389,
#27390,#27391,#27392,#27393,#27394,#27395,#27396,#27397,#27398,#27399,#27400,
#27401,#27402,#27403,#27404,#27405,#27406,#27407,#27408,#27409,#27410,#27411,
#27412,#27413,#27414,#27415,#27416,#27417,#27418,#27419,#27420,#27421,#27422,
#27423,#27424,#27425,#27426,#27427,#27428,#27429,#27430,#27431,#27432,#27433,
#27434,#27435,#27436,#27437,#27438,#27439,#27440,#27441,#27442,#27443,#27444,
#27445,#27446,#27447,#27448,#27449,#27450,#27451,#27452,#27453,#27454,#27455,
#27456,#27457,#27458,#27459,#27460,#27461,#27462,#27463,#27464,#27465,#27466,
#27467,#27468,#27469,#27470,#27471,#27472,#27473,#27474,#27475,#27476,#27477,
#27478,#27479,#27480,#27481,#27482,#27483,#27484,#27485,#27486,#27487,#27488),
(#27489,#27490,#27491,#27492,#27493,#27494,#27495,#27496,#27497,#27498,
#27499,#27500,#27501,#27502,#27503,#27504,#27505,#27506,#27507,#27508,#27509,
#27510,#27511,#27512,#27513,#27514,#27515,#27516,#27517,#27518,#27519,#27520,
#27521,#27522,#27523,#27524,#27525,#27526,#27527,#27528,#27529,#27530,#27531,
#27532,#27533,#27534,#27535,#27536,#27537,#27538,#27539,#27540,#27541,#27542,
#27543,#27544,#27545,#27546,#27547,#27548,#27549,#27550,#27551,#27552,#27553,
#27554,#27555,#27556,#27557,#27558,#27559,#27560,#27561,#27562,#27563,#27564,
#27565,#27566,#27567,#27568,#27569,#27570,#27571,#27572,#27573,#27574,#27575,
#27576,#27577,#27578,#27579,#27580,#27581,#27582,#27583,#27584,#27585,#27586,
#27587,#27588,#27589,#27590,#27591,#27592,#27593,#27594,#27595,#27596,#27597,
#27598,#27599,#27600,#27601,#27602,#27603,#27604,#27605,#27606,#27607,#27608,
#27609,#27610,#27611,#27612,#27613,#27614,#27615,#27616,#27617,#27618,#27619,
#27620,#27621,#27622,#27623,#27624,#27625,#27626,#27627,#27628,#27629,#27630,
#27631,#27632,#27633,#27634,#27635,#27636,#27637,#27638,#27639,#27640,#27641,
#27642,#27643,#27644,#27645,#27646,#27647,#27648,#27649)),.UNSPECIFIED.,
 .F.,.F.,.F.)
B_SPLINE_SURFACE_WITH_KNOTS((2,2),(3,2,2,2,2,2,2,2,2,2,2,2,2,2,2,2,2,2,
2,2,2,2,2,2,2,2,2,2,2,2,2,2,2,2,2,2,2,2,2,2,2,2,2,2,2,2,2,2,2,2,2,2,2,2,
2,2,2,2,2,2,2,2,2,2,2,2,2,2,2,2,2,2,2,2,2,2,2,2,2,2,3),(0.,1.),(0.,0.0125,
0.025,0.0375,0.05,0.0625,0.075,0.0875,0.1,0.1125,0.125,0.1375,0.15,0.1625,
0.175,0.1875,0.2,0.2125,0.225,0.2375,0.25,0.2625,0.275,0.2875,0.3,0.3125,
0.325,0.3375,0.35,0.3625,0.375,0.3875,0.4,0.4125,0.425,0.4375,0.45,0.4625,
0.475,0.4875,0.5,0.5125,0.525,0.5375,0.55,0.5625,0.575,0.5875,0.6,0.6125,
0.625,0.6375,0.65,0.6625,0.675,0.6875,0.7,0.7125,0.725,0.7375,0.75,0.7625,
0.775,0.7875,0.8,0.8125,0.825,0.8375,0.85,0.8625,0.875,0.8875,0.9,0.9125,
0.925,0.9375,0.95,0.9625,0.975,0.9875,1.),.UNSPECIFIED.)
GEOMETRIC_REPRESENTATION_ITEM()
RATIONAL_B_SPLINE_SURFACE(((1.,0.923879532511287,1.,0.923879532511287,1.,
0.923879532511287,1.,0.923879532511287,1.,0.923879532511287,1.,0.923879532511287,
1.,0.923879532511287,1.,0.923879532511287,1.,0.923879532511287,1.,0.923879532511287,
1.,0.923879532511287,1.,0.923879532511287,1.,0.923879532511287,1.,0.923879532511287,
1.,0.923879532511287,1.,0.923879532511287,1.,0.923879532511287,1.,0.923879532511287,
1.,0.923879532511287,1.,0.923879532511287,1.,0.923879532511287,1.,0.923879532511287,
1.,0.923879532511287,1.,0.923879532511287,1.,0.923879532511287,1.,0.923879532511287,
1.,0.923879532511287,1.,0.923879532511287,1.,0.923879532511287,1.,0.923879532511287,
1.,0.923879532511287,1.,0.923879532511287,1.,0.923879532511287,1.,0.923879532511287,
1.,0.923879532511287,1.,0.923879532511287,1.,0.923879532511287,1.,0.923879532511287,
1.,0.923879532511287,1.,0.923879532511287,1.,0.923879532511287,1.,0.923879532511287,
1.,0.923879532511287,1.,0.923879532511287,1.,0.923879532511287,1.,0.923879532511287,
1.,0.923879532511287,1.,0.923879532511287,1.,0.923879532511287,1.,0.923879532511287,
1.,0.923879532511287,1.,0.923879532511287,1.,0.923879532511287,1.,0.923879532511287,
1.,0.923879532511287,1.,0.923879532511287,1.,0.923879532511287,1.,0.923879532511287,
1.,0.923879532511287,1.,0.923879532511287,1.,0.923879532511287,1.,0.923879532511287,
1.,0.923879532511287,1.,0.923879532511287,1.,0.923879532511287,1.,0.923879532511287,
1.,0.923879532511287,1.,0.923879532511287,1.,0.923879532511287,1.,0.923879532511287,
1.,0.923879532511287,1.,0.923879532511287,1.,0.923879532511287,1.,0.923879532511287,
1.,0.923879532511287,1.,0.923879532511287,1.,0.923879532511287,1.,0.923879532511287,
1.,0.923879532511287,1.,0.923879532511287,1.),(1.,0.923879532511287,1.,
0.923879532511287,1.,0.923879532511287,1.,0.923879532511287,1.,0.923879532511287,
1.,0.923879532511287,1.,0.923879532511287,1.,0.923879532511287,1.,0.923879532511287,
1.,0.923879532511287,1.,0.923879532511287,1.,0.923879532511287,1.,0.923879532511287,
1.,0.923879532511287,1.,0.923879532511287,1.,0.923879532511287,1.,0.923879532511287,
1.,0.923879532511287,1.,0.923879532511287,1.,0.923879532511287,1.,0.923879532511287,
1.,0.923879532511287,1.,0.923879532511287,1.,0.923879532511287,1.,0.923879532511287,
1.,0.923879532511287,1.,0.923879532511287,1.,0.923879532511287,1.,0.923879532511287,
1.,0.923879532511287,1.,0.923879532511287,1.,0.923879532511287,1.,0.923879532511287,
1.,0.923879532511287,1.,0.923879532511287,1.,0.923879532511287,1.,0.923879532511287,
1.,0.923879532511287,1.,0.923879532511287,1.,0.923879532511287,1.,0.923879532511287,
1.,0.923879532511287,1.,0.923879532511287,1.,0.923879532511287,1.,0.923879532511287,
1.,0.923879532511287,1.,0.923879532511287,1.,0.923879532511287,1.,0.923879532511287,
1.,0.923879532511287,1.,0.923879532511287,1.,0.923879532511287,1.,0.923879532511287,
1.,0.923879532511287,1.,0.923879532511287,1.,0.923879532511287,1.,0.923879532511287,
1.,0.923879532511287,1.,0.923879532511287,1.,0.923879532511287,1.,0.923879532511287,
1.,0.923879532511287,1.,0.923879532511287,1.,0.923879532511287,1.,0.923879532511287,
1.,0.923879532511287,1.,0.923879532511287,1.,0.923879532511287,1.,0.923879532511287,
1.,0.923879532511287,1.,0.923879532511287,1.,0.923879532511287,1.,0.923879532511287,
1.,0.923879532511287,1.,0.923879532511287,1.,0.923879532511287,1.,0.923879532511287,
1.,0.923879532511287,1.,0.923879532511287,1.,0.923879532511287,1.)))
REPRESENTATION_ITEM('')
SURFACE()
);
#573=(
BOUNDED_SURFACE()
B_SPLINE_SURFACE(1,2,((#27667,#27668,#27669,#27670,#27671,#27672,#27673,
#27674,#27675,#27676,#27677,#27678,#27679,#27680,#27681,#27682,#27683,#27684,
#27685,#27686,#27687,#27688,#27689,#27690,#27691,#27692,#27693,#27694,#27695,
#27696,#27697,#27698,#27699,#27700,#27701,#27702,#27703,#27704,#27705,#27706,
#27707,#27708,#27709,#27710,#27711,#27712,#27713,#27714,#27715,#27716,#27717,
#27718,#27719,#27720,#27721,#27722,#27723,#27724,#27725,#27726,#27727,#27728,
#27729,#27730,#27731,#27732,#27733,#27734,#27735,#27736,#27737,#27738,#27739,
#27740,#27741,#27742,#27743,#27744,#27745,#27746,#27747,#27748,#27749,#27750,
#27751,#27752,#27753,#27754,#27755,#27756,#27757,#27758,#27759,#27760,#27761,
#27762,#27763,#27764,#27765,#27766,#27767,#27768,#27769,#27770,#27771,#27772,
#27773,#27774,#27775,#27776,#27777,#27778,#27779,#27780,#27781,#27782,#27783,
#27784,#27785,#27786,#27787,#27788,#27789,#27790,#27791,#27792,#27793,#27794,
#27795,#27796,#27797,#27798,#27799,#27800,#27801,#27802,#27803,#27804,#27805,
#27806,#27807,#27808,#27809,#27810,#27811,#27812,#27813,#27814,#27815,#27816,
#27817,#27818,#27819,#27820,#27821,#27822,#27823,#27824,#27825,#27826,#27827),
(#27828,#27829,#27830,#27831,#27832,#27833,#27834,#27835,#27836,#27837,
#27838,#27839,#27840,#27841,#27842,#27843,#27844,#27845,#27846,#27847,#27848,
#27849,#27850,#27851,#27852,#27853,#27854,#27855,#27856,#27857,#27858,#27859,
#27860,#27861,#27862,#27863,#27864,#27865,#27866,#27867,#27868,#27869,#27870,
#27871,#27872,#27873,#27874,#27875,#27876,#27877,#27878,#27879,#27880,#27881,
#27882,#27883,#27884,#27885,#27886,#27887,#27888,#27889,#27890,#27891,#27892,
#27893,#27894,#27895,#27896,#27897,#27898,#27899,#27900,#27901,#27902,#27903,
#27904,#27905,#27906,#27907,#27908,#27909,#27910,#27911,#27912,#27913,#27914,
#27915,#27916,#27917,#27918,#27919,#27920,#27921,#27922,#27923,#27924,#27925,
#27926,#27927,#27928,#27929,#27930,#27931,#27932,#27933,#27934,#27935,#27936,
#27937,#27938,#27939,#27940,#27941,#27942,#27943,#27944,#27945,#27946,#27947,
#27948,#27949,#27950,#27951,#27952,#27953,#27954,#27955,#27956,#27957,#27958,
#27959,#27960,#27961,#27962,#27963,#27964,#27965,#27966,#27967,#27968,#27969,
#27970,#27971,#27972,#27973,#27974,#27975,#27976,#27977,#27978,#27979,#27980,
#27981,#27982,#27983,#27984,#27985,#27986,#27987,#27988)),.UNSPECIFIED.,
 .F.,.F.,.F.)
B_SPLINE_SURFACE_WITH_KNOTS((2,2),(3,2,2,2,2,2,2,2,2,2,2,2,2,2,2,2,2,2,
2,2,2,2,2,2,2,2,2,2,2,2,2,2,2,2,2,2,2,2,2,2,2,2,2,2,2,2,2,2,2,2,2,2,2,2,
2,2,2,2,2,2,2,2,2,2,2,2,2,2,2,2,2,2,2,2,2,2,2,2,2,2,3),(0.,1.),(0.,0.0125,
0.025,0.0375,0.05,0.0625,0.075,0.0875,0.1,0.1125,0.125,0.1375,0.15,0.1625,
0.175,0.1875,0.2,0.2125,0.225,0.2375,0.25,0.2625,0.275,0.2875,0.3,0.3125,
0.325,0.3375,0.35,0.3625,0.375,0.3875,0.4,0.4125,0.425,0.4375,0.45,0.4625,
0.475,0.4875,0.5,0.5125,0.525,0.5375,0.55,0.5625,0.575,0.5875,0.6,0.6125,
0.625,0.6375,0.65,0.6625,0.675,0.6875,0.7,0.7125,0.725,0.7375,0.75,0.7625,
0.775,0.7875,0.8,0.8125,0.825,0.8375,0.85,0.8625,0.875,0.8875,0.9,0.9125,
0.925,0.9375,0.95,0.9625,0.975,0.9875,1.),.UNSPECIFIED.)
GEOMETRIC_REPRESENTATION_ITEM()
RATIONAL_B_SPLINE_SURFACE(((1.,0.923879532511287,1.,0.923879532511287,1.,
0.923879532511287,1.,0.923879532511287,1.,0.923879532511287,1.,0.923879532511287,
1.,0.923879532511287,1.,0.923879532511287,1.,0.923879532511287,1.,0.923879532511287,
1.,0.923879532511287,1.,0.923879532511287,1.,0.923879532511287,1.,0.923879532511287,
1.,0.923879532511287,1.,0.923879532511287,1.,0.923879532511287,1.,0.923879532511287,
1.,0.923879532511287,1.,0.923879532511287,1.,0.923879532511287,1.,0.923879532511287,
1.,0.923879532511287,1.,0.923879532511287,1.,0.923879532511287,1.,0.923879532511287,
1.,0.923879532511287,1.,0.923879532511287,1.,0.923879532511287,1.,0.923879532511287,
1.,0.923879532511287,1.,0.923879532511287,1.,0.923879532511287,1.,0.923879532511287,
1.,0.923879532511287,1.,0.923879532511287,1.,0.923879532511287,1.,0.923879532511287,
1.,0.923879532511287,1.,0.923879532511287,1.,0.923879532511287,1.,0.923879532511287,
1.,0.923879532511287,1.,0.923879532511287,1.,0.923879532511287,1.,0.923879532511287,
1.,0.923879532511287,1.,0.923879532511287,1.,0.923879532511287,1.,0.923879532511287,
1.,0.923879532511287,1.,0.923879532511287,1.,0.923879532511287,1.,0.923879532511287,
1.,0.923879532511287,1.,0.923879532511287,1.,0.923879532511287,1.,0.923879532511287,
1.,0.923879532511287,1.,0.923879532511287,1.,0.923879532511287,1.,0.923879532511287,
1.,0.923879532511287,1.,0.923879532511287,1.,0.923879532511287,1.,0.923879532511287,
1.,0.923879532511287,1.,0.923879532511287,1.,0.923879532511287,1.,0.923879532511287,
1.,0.923879532511287,1.,0.923879532511287,1.,0.923879532511287,1.,0.923879532511287,
1.,0.923879532511287,1.,0.923879532511287,1.,0.923879532511287,1.,0.923879532511287,
1.,0.923879532511287,1.,0.923879532511287,1.),(1.,0.923879532511287,1.,
0.923879532511287,1.,0.923879532511287,1.,0.923879532511287,1.,0.923879532511287,
1.,0.923879532511287,1.,0.923879532511287,1.,0.923879532511287,1.,0.923879532511287,
1.,0.923879532511287,1.,0.923879532511287,1.,0.923879532511287,1.,0.923879532511287,
1.,0.923879532511287,1.,0.923879532511287,1.,0.923879532511287,1.,0.923879532511287,
1.,0.923879532511287,1.,0.923879532511287,1.,0.923879532511287,1.,0.923879532511287,
1.,0.923879532511287,1.,0.923879532511287,1.,0.923879532511287,1.,0.923879532511287,
1.,0.923879532511287,1.,0.923879532511287,1.,0.923879532511287,1.,0.923879532511287,
1.,0.923879532511287,1.,0.923879532511287,1.,0.923879532511287,1.,0.923879532511287,
1.,0.923879532511287,1.,0.923879532511287,1.,0.923879532511287,1.,0.923879532511287,
1.,0.923879532511287,1.,0.923879532511287,1.,0.923879532511287,1.,0.923879532511287,
1.,0.923879532511287,1.,0.923879532511287,1.,0.923879532511287,1.,0.923879532511287,
1.,0.923879532511287,1.,0.923879532511287,1.,0.923879532511287,1.,0.923879532511287,
1.,0.923879532511287,1.,0.923879532511287,1.,0.923879532511287,1.,0.923879532511287,
1.,0.923879532511287,1.,0.923879532511287,1.,0.923879532511287,1.,0.923879532511287,
1.,0.923879532511287,1.,0.923879532511287,1.,0.923879532511287,1.,0.923879532511287,
1.,0.923879532511287,1.,0.923879532511287,1.,0.923879532511287,1.,0.923879532511287,
1.,0.923879532511287,1.,0.923879532511287,1.,0.923879532511287,1.,0.923879532511287,
1.,0.923879532511287,1.,0.923879532511287,1.,0.923879532511287,1.,0.923879532511287,
1.,0.923879532511287,1.,0.923879532511287,1.,0.923879532511287,1.,0.923879532511287,
1.,0.923879532511287,1.,0.923879532511287,1.,0.923879532511287,1.)))
REPRESENTATION_ITEM('')
SURFACE()
);
#574=(
BOUNDED_SURFACE()
B_SPLINE_SURFACE(3,2,((#28006,#28007,#28008,#28009,#28010,#28011,#28012,
#28013,#28014,#28015,#28016,#28017,#28018,#28019,#28020,#28021,#28022,#28023,
#28024,#28025,#28026,#28027,#28028,#28029,#28030,#28031,#28032,#28033,#28034,
#28035,#28036,#28037,#28038,#28039,#28040,#28041,#28042,#28043,#28044,#28045,
#28046,#28047,#28048,#28049,#28050,#28051,#28052,#28053,#28054,#28055,#28056,
#28057,#28058,#28059,#28060,#28061,#28062,#28063,#28064,#28065,#28066,#28067,
#28068,#28069,#28070,#28071,#28072,#28073,#28074,#28075,#28076,#28077,#28078,
#28079,#28080,#28081,#28082,#28083,#28084,#28085,#28086,#28087,#28088,#28089,
#28090,#28091,#28092,#28093,#28094,#28095,#28096,#28097,#28098,#28099,#28100,
#28101,#28102,#28103,#28104,#28105,#28106,#28107,#28108,#28109,#28110,#28111,
#28112,#28113,#28114,#28115,#28116,#28117,#28118,#28119,#28120,#28121,#28122,
#28123,#28124,#28125,#28126,#28127,#28128,#28129,#28130,#28131,#28132,#28133,
#28134,#28135,#28136,#28137,#28138,#28139,#28140,#28141,#28142,#28143,#28144,
#28145,#28146,#28147,#28148,#28149,#28150,#28151,#28152,#28153,#28154,#28155,
#28156,#28157,#28158,#28159,#28160,#28161,#28162,#28163,#28164,#28165,#28166),
(#28167,#28168,#28169,#28170,#28171,#28172,#28173,#28174,#28175,#28176,
#28177,#28178,#28179,#28180,#28181,#28182,#28183,#28184,#28185,#28186,#28187,
#28188,#28189,#28190,#28191,#28192,#28193,#28194,#28195,#28196,#28197,#28198,
#28199,#28200,#28201,#28202,#28203,#28204,#28205,#28206,#28207,#28208,#28209,
#28210,#28211,#28212,#28213,#28214,#28215,#28216,#28217,#28218,#28219,#28220,
#28221,#28222,#28223,#28224,#28225,#28226,#28227,#28228,#28229,#28230,#28231,
#28232,#28233,#28234,#28235,#28236,#28237,#28238,#28239,#28240,#28241,#28242,
#28243,#28244,#28245,#28246,#28247,#28248,#28249,#28250,#28251,#28252,#28253,
#28254,#28255,#28256,#28257,#28258,#28259,#28260,#28261,#28262,#28263,#28264,
#28265,#28266,#28267,#28268,#28269,#28270,#28271,#28272,#28273,#28274,#28275,
#28276,#28277,#28278,#28279,#28280,#28281,#28282,#28283,#28284,#28285,#28286,
#28287,#28288,#28289,#28290,#28291,#28292,#28293,#28294,#28295,#28296,#28297,
#28298,#28299,#28300,#28301,#28302,#28303,#28304,#28305,#28306,#28307,#28308,
#28309,#28310,#28311,#28312,#28313,#28314,#28315,#28316,#28317,#28318,#28319,
#28320,#28321,#28322,#28323,#28324,#28325,#28326,#28327),(#28328,#28329,
#28330,#28331,#28332,#28333,#28334,#28335,#28336,#28337,#28338,#28339,#28340,
#28341,#28342,#28343,#28344,#28345,#28346,#28347,#28348,#28349,#28350,#28351,
#28352,#28353,#28354,#28355,#28356,#28357,#28358,#28359,#28360,#28361,#28362,
#28363,#28364,#28365,#28366,#28367,#28368,#28369,#28370,#28371,#28372,#28373,
#28374,#28375,#28376,#28377,#28378,#28379,#28380,#28381,#28382,#28383,#28384,
#28385,#28386,#28387,#28388,#28389,#28390,#28391,#28392,#28393,#28394,#28395,
#28396,#28397,#28398,#28399,#28400,#28401,#28402,#28403,#28404,#28405,#28406,
#28407,#28408,#28409,#28410,#28411,#28412,#28413,#28414,#28415,#28416,#28417,
#28418,#28419,#28420,#28421,#28422,#28423,#28424,#28425,#28426,#28427,#28428,
#28429,#28430,#28431,#28432,#28433,#28434,#28435,#28436,#28437,#28438,#28439,
#28440,#28441,#28442,#28443,#28444,#28445,#28446,#28447,#28448,#28449,#28450,
#28451,#28452,#28453,#28454,#28455,#28456,#28457,#28458,#28459,#28460,#28461,
#28462,#28463,#28464,#28465,#28466,#28467,#28468,#28469,#28470,#28471,#28472,
#28473,#28474,#28475,#28476,#28477,#28478,#28479,#28480,#28481,#28482,#28483,
#28484,#28485,#28486,#28487,#28488),(#28489,#28490,#28491,#28492,#28493,
#28494,#28495,#28496,#28497,#28498,#28499,#28500,#28501,#28502,#28503,#28504,
#28505,#28506,#28507,#28508,#28509,#28510,#28511,#28512,#28513,#28514,#28515,
#28516,#28517,#28518,#28519,#28520,#28521,#28522,#28523,#28524,#28525,#28526,
#28527,#28528,#28529,#28530,#28531,#28532,#28533,#28534,#28535,#28536,#28537,
#28538,#28539,#28540,#28541,#28542,#28543,#28544,#28545,#28546,#28547,#28548,
#28549,#28550,#28551,#28552,#28553,#28554,#28555,#28556,#28557,#28558,#28559,
#28560,#28561,#28562,#28563,#28564,#28565,#28566,#28567,#28568,#28569,#28570,
#28571,#28572,#28573,#28574,#28575,#28576,#28577,#28578,#28579,#28580,#28581,
#28582,#28583,#28584,#28585,#28586,#28587,#28588,#28589,#28590,#28591,#28592,
#28593,#28594,#28595,#28596,#28597,#28598,#28599,#28600,#28601,#28602,#28603,
#28604,#28605,#28606,#28607,#28608,#28609,#28610,#28611,#28612,#28613,#28614,
#28615,#28616,#28617,#28618,#28619,#28620,#28621,#28622,#28623,#28624,#28625,
#28626,#28627,#28628,#28629,#28630,#28631,#28632,#28633,#28634,#28635,#28636,
#28637,#28638,#28639,#28640,#28641,#28642,#28643,#28644,#28645,#28646,#28647,
#28648,#28649)),.UNSPECIFIED.,.F.,.F.,.F.)
B_SPLINE_SURFACE_WITH_KNOTS((4,4),(3,2,2,2,2,2,2,2,2,2,2,2,2,2,2,2,2,2,
2,2,2,2,2,2,2,2,2,2,2,2,2,2,2,2,2,2,2,2,2,2,2,2,2,2,2,2,2,2,2,2,2,2,2,2,
2,2,2,2,2,2,2,2,2,2,2,2,2,2,2,2,2,2,2,2,2,2,2,2,2,2,3),(0.,1.),(0.,0.0125,
0.025,0.0375,0.05,0.0625,0.075,0.0875,0.1,0.1125,0.125,0.1375,0.15,0.1625,
0.175,0.1875,0.2,0.2125,0.225,0.2375,0.25,0.2625,0.275,0.2875,0.3,0.3125,
0.325,0.3375,0.35,0.3625,0.375,0.3875,0.4,0.4125,0.425,0.4375,0.45,0.4625,
0.475,0.4875,0.5,0.5125,0.525,0.5375,0.55,0.5625,0.575,0.5875,0.6,0.6125,
0.625,0.6375,0.65,0.6625,0.675,0.6875,0.7,0.7125,0.725,0.7375,0.75,0.7625,
0.775,0.7875,0.8,0.8125,0.825,0.8375,0.85,0.8625,0.875,0.8875,0.9,0.9125,
0.925,0.9375,0.95,0.9625,0.975,0.9875,1.),.UNSPECIFIED.)
GEOMETRIC_REPRESENTATION_ITEM()
RATIONAL_B_SPLINE_SURFACE(((1.,0.923879532511287,1.,0.923879532511287,1.,
0.923879532511287,1.,0.923879532511287,1.,0.923879532511287,1.,0.923879532511287,
1.,0.923879532511287,1.,0.923879532511287,1.,0.923879532511287,1.,0.923879532511287,
1.,0.923879532511287,1.,0.923879532511287,1.,0.923879532511287,1.,0.923879532511287,
1.,0.923879532511287,1.,0.923879532511287,1.,0.923879532511287,1.,0.923879532511287,
1.,0.923879532511287,1.,0.923879532511287,1.,0.923879532511287,1.,0.923879532511287,
1.,0.923879532511287,1.,0.923879532511287,1.,0.923879532511287,1.,0.923879532511287,
1.,0.923879532511287,1.,0.923879532511287,1.,0.923879532511287,1.,0.923879532511287,
1.,0.923879532511287,1.,0.923879532511287,1.,0.923879532511287,1.,0.923879532511287,
1.,0.923879532511287,1.,0.923879532511287,1.,0.923879532511287,1.,0.923879532511287,
1.,0.923879532511287,1.,0.923879532511287,1.,0.923879532511287,1.,0.923879532511287,
1.,0.923879532511287,1.,0.923879532511287,1.,0.923879532511287,1.,0.923879532511287,
1.,0.923879532511287,1.,0.923879532511287,1.,0.923879532511287,1.,0.923879532511287,
1.,0.923879532511287,1.,0.923879532511287,1.,0.923879532511287,1.,0.923879532511287,
1.,0.923879532511287,1.,0.923879532511287,1.,0.923879532511287,1.,0.923879532511287,
1.,0.923879532511287,1.,0.923879532511287,1.,0.923879532511287,1.,0.923879532511287,
1.,0.923879532511287,1.,0.923879532511287,1.,0.923879532511287,1.,0.923879532511287,
1.,0.923879532511287,1.,0.923879532511287,1.,0.923879532511287,1.,0.923879532511287,
1.,0.923879532511287,1.,0.923879532511287,1.,0.923879532511287,1.,0.923879532511287,
1.,0.923879532511287,1.,0.923879532511287,1.,0.923879532511287,1.,0.923879532511287,
1.,0.923879532511287,1.,0.923879532511287,1.),(0.998696642611305,0.922675387296324,
0.998696642611305,0.922675387296324,0.998696642611305,0.922675387296324,
0.998696642611305,0.922675387296324,0.998696642611305,0.922675387296324,
0.998696642611305,0.922675387296324,0.998696642611305,0.922675387296324,
0.998696642611305,0.922675387296324,0.998696642611305,0.922675387296324,
0.998696642611305,0.922675387296324,0.998696642611305,0.922675387296324,
0.998696642611305,0.922675387296324,0.998696642611305,0.922675387296324,
0.998696642611305,0.922675387296324,0.998696642611305,0.922675387296324,
0.998696642611305,0.922675387296324,0.998696642611305,0.922675387296324,
0.998696642611305,0.922675387296324,0.998696642611305,0.922675387296324,
0.998696642611305,0.922675387296324,0.998696642611305,0.922675387296324,
0.998696642611305,0.922675387296324,0.998696642611305,0.922675387296324,
0.998696642611305,0.922675387296324,0.998696642611305,0.922675387296324,
0.998696642611305,0.922675387296324,0.998696642611305,0.922675387296324,
0.998696642611305,0.922675387296324,0.998696642611305,0.922675387296324,
0.998696642611305,0.922675387296324,0.998696642611305,0.922675387296324,
0.998696642611305,0.922675387296324,0.998696642611305,0.922675387296324,
0.998696642611305,0.922675387296324,0.998696642611305,0.922675387296324,
0.998696642611305,0.922675387296324,0.998696642611305,0.922675387296324,
0.998696642611305,0.922675387296324,0.998696642611305,0.922675387296324,
0.998696642611305,0.922675387296324,0.998696642611305,0.922675387296324,
0.998696642611305,0.922675387296324,0.998696642611305,0.922675387296324,
0.998696642611305,0.922675387296324,0.998696642611305,0.922675387296324,
0.998696642611305,0.922675387296324,0.998696642611305,0.922675387296324,
0.998696642611305,0.922675387296324,0.998696642611305,0.922675387296324,
0.998696642611305,0.922675387296324,0.998696642611305,0.922675387296324,
0.998696642611305,0.922675387296324,0.998696642611305,0.922675387296324,
0.998696642611305,0.922675387296324,0.998696642611305,0.922675387296324,
0.998696642611305,0.922675387296324,0.998696642611305,0.922675387296324,
0.998696642611305,0.922675387296324,0.998696642611305,0.922675387296324,
0.998696642611305,0.922675387296324,0.998696642611305,0.922675387296324,
0.998696642611305,0.922675387296324,0.998696642611305,0.922675387296324,
0.998696642611305,0.922675387296324,0.998696642611305,0.922675387296324,
0.998696642611305,0.922675387296324,0.998696642611305,0.922675387296324,
0.998696642611305,0.922675387296324,0.998696642611305,0.922675387296324,
0.998696642611305,0.922675387296324,0.998696642611305,0.922675387296324,
0.998696642611305,0.922675387296324,0.998696642611305,0.922675387296324,
0.998696642611305,0.922675387296324,0.998696642611305,0.922675387296324,
0.998696642611305,0.922675387296324,0.998696642611305,0.922675387296324,
0.998696642611305,0.922675387296324,0.998696642611305,0.922675387296324,
0.998696642611305,0.922675387296324,0.998696642611305),(0.998696642611305,
0.922675387296324,0.998696642611305,0.922675387296324,0.998696642611305,
0.922675387296324,0.998696642611305,0.922675387296324,0.998696642611305,
0.922675387296324,0.998696642611305,0.922675387296324,0.998696642611305,
0.922675387296324,0.998696642611305,0.922675387296324,0.998696642611305,
0.922675387296324,0.998696642611305,0.922675387296324,0.998696642611305,
0.922675387296324,0.998696642611305,0.922675387296324,0.998696642611305,
0.922675387296324,0.998696642611305,0.922675387296324,0.998696642611305,
0.922675387296324,0.998696642611305,0.922675387296324,0.998696642611305,
0.922675387296324,0.998696642611305,0.922675387296324,0.998696642611305,
0.922675387296324,0.998696642611305,0.922675387296324,0.998696642611305,
0.922675387296324,0.998696642611305,0.922675387296324,0.998696642611305,
0.922675387296324,0.998696642611305,0.922675387296324,0.998696642611305,
0.922675387296324,0.998696642611305,0.922675387296324,0.998696642611305,
0.922675387296324,0.998696642611305,0.922675387296324,0.998696642611305,
0.922675387296324,0.998696642611305,0.922675387296324,0.998696642611305,
0.922675387296324,0.998696642611305,0.922675387296324,0.998696642611305,
0.922675387296324,0.998696642611305,0.922675387296324,0.998696642611305,
0.922675387296324,0.998696642611305,0.922675387296324,0.998696642611305,
0.922675387296324,0.998696642611305,0.922675387296324,0.998696642611305,
0.922675387296324,0.998696642611305,0.922675387296324,0.998696642611305,
0.922675387296324,0.998696642611305,0.922675387296324,0.998696642611305,
0.922675387296324,0.998696642611305,0.922675387296324,0.998696642611305,
0.922675387296324,0.998696642611305,0.922675387296324,0.998696642611305,
0.922675387296324,0.998696642611305,0.922675387296324,0.998696642611305,
0.922675387296324,0.998696642611305,0.922675387296324,0.998696642611305,
0.922675387296324,0.998696642611305,0.922675387296324,0.998696642611305,
0.922675387296324,0.998696642611305,0.922675387296324,0.998696642611305,
0.922675387296324,0.998696642611305,0.922675387296324,0.998696642611305,
0.922675387296324,0.998696642611305,0.922675387296324,0.998696642611305,
0.922675387296324,0.998696642611305,0.922675387296324,0.998696642611305,
0.922675387296324,0.998696642611305,0.922675387296324,0.998696642611305,
0.922675387296324,0.998696642611305,0.922675387296324,0.998696642611305,
0.922675387296324,0.998696642611305,0.922675387296324,0.998696642611305,
0.922675387296324,0.998696642611305,0.922675387296324,0.998696642611305,
0.922675387296324,0.998696642611305,0.922675387296324,0.998696642611305,
0.922675387296324,0.998696642611305,0.922675387296324,0.998696642611305,
0.922675387296324,0.998696642611305,0.922675387296324,0.998696642611305,
0.922675387296324,0.998696642611305,0.922675387296324,0.998696642611305,
0.922675387296324,0.998696642611305,0.922675387296324,0.998696642611305,
0.922675387296324,0.998696642611305,0.922675387296324,0.998696642611305),
(1.,0.923879532511287,1.,0.923879532511287,1.,0.923879532511287,1.,0.923879532511287,
1.,0.923879532511287,1.,0.923879532511287,1.,0.923879532511287,1.,0.923879532511287,
1.,0.923879532511287,1.,0.923879532511287,1.,0.923879532511287,1.,0.923879532511287,
1.,0.923879532511287,1.,0.923879532511287,1.,0.923879532511287,1.,0.923879532511287,
1.,0.923879532511287,1.,0.923879532511287,1.,0.923879532511287,1.,0.923879532511287,
1.,0.923879532511287,1.,0.923879532511287,1.,0.923879532511287,1.,0.923879532511287,
1.,0.923879532511287,1.,0.923879532511287,1.,0.923879532511287,1.,0.923879532511287,
1.,0.923879532511287,1.,0.923879532511287,1.,0.923879532511287,1.,0.923879532511287,
1.,0.923879532511287,1.,0.923879532511287,1.,0.923879532511287,1.,0.923879532511287,
1.,0.923879532511287,1.,0.923879532511287,1.,0.923879532511287,1.,0.923879532511287,
1.,0.923879532511287,1.,0.923879532511287,1.,0.923879532511287,1.,0.923879532511287,
1.,0.923879532511287,1.,0.923879532511287,1.,0.923879532511287,1.,0.923879532511287,
1.,0.923879532511287,1.,0.923879532511287,1.,0.923879532511287,1.,0.923879532511287,
1.,0.923879532511287,1.,0.923879532511287,1.,0.923879532511287,1.,0.923879532511287,
1.,0.923879532511287,1.,0.923879532511287,1.,0.923879532511287,1.,0.923879532511287,
1.,0.923879532511287,1.,0.923879532511287,1.,0.923879532511287,1.,0.923879532511287,
1.,0.923879532511287,1.,0.923879532511287,1.,0.923879532511287,1.,0.923879532511287,
1.,0.923879532511287,1.,0.923879532511287,1.,0.923879532511287,1.,0.923879532511287,
1.,0.923879532511287,1.,0.923879532511287,1.,0.923879532511287,1.,0.923879532511287,
1.,0.923879532511287,1.,0.923879532511287,1.,0.923879532511287,1.,0.923879532511287,
1.)))
REPRESENTATION_ITEM('')
SURFACE()
);
#575=(
BOUNDED_SURFACE()
B_SPLINE_SURFACE(1,2,((#28650,#28651,#28652,#28653,#28654,#28655,#28656,
#28657,#28658,#28659,#28660,#28661,#28662,#28663,#28664,#28665,#28666,#28667,
#28668,#28669,#28670,#28671,#28672,#28673,#28674,#28675,#28676,#28677,#28678,
#28679,#28680,#28681,#28682,#28683,#28684,#28685,#28686,#28687,#28688,#28689,
#28690,#28691,#28692,#28693,#28694,#28695,#28696,#28697,#28698,#28699,#28700,
#28701,#28702,#28703,#28704,#28705,#28706,#28707,#28708,#28709,#28710,#28711,
#28712,#28713,#28714,#28715,#28716,#28717,#28718,#28719,#28720,#28721,#28722,
#28723,#28724,#28725,#28726,#28727,#28728,#28729,#28730,#28731,#28732,#28733,
#28734,#28735,#28736,#28737,#28738,#28739,#28740,#28741,#28742,#28743,#28744,
#28745,#28746,#28747,#28748,#28749,#28750,#28751,#28752,#28753,#28754,#28755,
#28756,#28757,#28758,#28759,#28760,#28761,#28762,#28763,#28764,#28765,#28766,
#28767,#28768,#28769,#28770,#28771,#28772,#28773,#28774,#28775,#28776,#28777,
#28778,#28779,#28780,#28781,#28782,#28783,#28784,#28785,#28786,#28787,#28788,
#28789,#28790,#28791,#28792,#28793,#28794,#28795,#28796,#28797,#28798,#28799,
#28800,#28801,#28802,#28803,#28804,#28805,#28806,#28807,#28808,#28809,#28810),
(#28811,#28812,#28813,#28814,#28815,#28816,#28817,#28818,#28819,#28820,
#28821,#28822,#28823,#28824,#28825,#28826,#28827,#28828,#28829,#28830,#28831,
#28832,#28833,#28834,#28835,#28836,#28837,#28838,#28839,#28840,#28841,#28842,
#28843,#28844,#28845,#28846,#28847,#28848,#28849,#28850,#28851,#28852,#28853,
#28854,#28855,#28856,#28857,#28858,#28859,#28860,#28861,#28862,#28863,#28864,
#28865,#28866,#28867,#28868,#28869,#28870,#28871,#28872,#28873,#28874,#28875,
#28876,#28877,#28878,#28879,#28880,#28881,#28882,#28883,#28884,#28885,#28886,
#28887,#28888,#28889,#28890,#28891,#28892,#28893,#28894,#28895,#28896,#28897,
#28898,#28899,#28900,#28901,#28902,#28903,#28904,#28905,#28906,#28907,#28908,
#28909,#28910,#28911,#28912,#28913,#28914,#28915,#28916,#28917,#28918,#28919,
#28920,#28921,#28922,#28923,#28924,#28925,#28926,#28927,#28928,#28929,#28930,
#28931,#28932,#28933,#28934,#28935,#28936,#28937,#28938,#28939,#28940,#28941,
#28942,#28943,#28944,#28945,#28946,#28947,#28948,#28949,#28950,#28951,#28952,
#28953,#28954,#28955,#28956,#28957,#28958,#28959,#28960,#28961,#28962,#28963,
#28964,#28965,#28966,#28967,#28968,#28969,#28970,#28971)),.UNSPECIFIED.,
 .F.,.F.,.F.)
B_SPLINE_SURFACE_WITH_KNOTS((2,2),(3,2,2,2,2,2,2,2,2,2,2,2,2,2,2,2,2,2,
2,2,2,2,2,2,2,2,2,2,2,2,2,2,2,2,2,2,2,2,2,2,2,2,2,2,2,2,2,2,2,2,2,2,2,2,
2,2,2,2,2,2,2,2,2,2,2,2,2,2,2,2,2,2,2,2,2,2,2,2,2,2,3),(0.,1.),(0.,0.0125,
0.025,0.0375,0.05,0.0625,0.075,0.0875,0.1,0.1125,0.125,0.1375,0.15,0.1625,
0.175,0.1875,0.2,0.2125,0.225,0.2375,0.25,0.2625,0.275,0.2875,0.3,0.3125,
0.325,0.3375,0.35,0.3625,0.375,0.3875,0.4,0.4125,0.425,0.4375,0.45,0.4625,
0.475,0.4875,0.5,0.5125,0.525,0.5375,0.55,0.5625,0.575,0.5875,0.6,0.6125,
0.625,0.6375,0.65,0.6625,0.675,0.6875,0.7,0.7125,0.725,0.7375,0.75,0.7625,
0.775,0.7875,0.8,0.8125,0.825,0.8375,0.85,0.8625,0.875,0.8875,0.9,0.9125,
0.925,0.9375,0.95,0.9625,0.975,0.9875,1.),.UNSPECIFIED.)
GEOMETRIC_REPRESENTATION_ITEM()
RATIONAL_B_SPLINE_SURFACE(((1.,0.923879532511287,1.,0.923879532511287,1.,
0.923879532511287,1.,0.923879532511287,1.,0.923879532511287,1.,0.923879532511287,
1.,0.923879532511287,1.,0.923879532511287,1.,0.923879532511287,1.,0.923879532511287,
1.,0.923879532511287,1.,0.923879532511287,1.,0.923879532511287,1.,0.923879532511287,
1.,0.923879532511287,1.,0.923879532511287,1.,0.923879532511287,1.,0.923879532511287,
1.,0.923879532511287,1.,0.923879532511287,1.,0.923879532511287,1.,0.923879532511287,
1.,0.923879532511287,1.,0.923879532511287,1.,0.923879532511287,1.,0.923879532511287,
1.,0.923879532511287,1.,0.923879532511287,1.,0.923879532511287,1.,0.923879532511287,
1.,0.923879532511287,1.,0.923879532511287,1.,0.923879532511287,1.,0.923879532511287,
1.,0.923879532511287,1.,0.923879532511287,1.,0.923879532511287,1.,0.923879532511287,
1.,0.923879532511287,1.,0.923879532511287,1.,0.923879532511287,1.,0.923879532511287,
1.,0.923879532511287,1.,0.923879532511287,1.,0.923879532511287,1.,0.923879532511287,
1.,0.923879532511287,1.,0.923879532511287,1.,0.923879532511287,1.,0.923879532511287,
1.,0.923879532511287,1.,0.923879532511287,1.,0.923879532511287,1.,0.923879532511287,
1.,0.923879532511287,1.,0.923879532511287,1.,0.923879532511287,1.,0.923879532511287,
1.,0.923879532511287,1.,0.923879532511287,1.,0.923879532511287,1.,0.923879532511287,
1.,0.923879532511287,1.,0.923879532511287,1.,0.923879532511287,1.,0.923879532511287,
1.,0.923879532511287,1.,0.923879532511287,1.,0.923879532511287,1.,0.923879532511287,
1.,0.923879532511287,1.,0.923879532511287,1.,0.923879532511287,1.,0.923879532511287,
1.,0.923879532511287,1.,0.923879532511287,1.,0.923879532511287,1.,0.923879532511287,
1.,0.923879532511287,1.,0.923879532511287,1.),(1.,0.923879532511287,1.,
0.923879532511287,1.,0.923879532511287,1.,0.923879532511287,1.,0.923879532511287,
1.,0.923879532511287,1.,0.923879532511287,1.,0.923879532511287,1.,0.923879532511287,
1.,0.923879532511287,1.,0.923879532511287,1.,0.923879532511287,1.,0.923879532511287,
1.,0.923879532511287,1.,0.923879532511287,1.,0.923879532511287,1.,0.923879532511287,
1.,0.923879532511287,1.,0.923879532511287,1.,0.923879532511287,1.,0.923879532511287,
1.,0.923879532511287,1.,0.923879532511287,1.,0.923879532511287,1.,0.923879532511287,
1.,0.923879532511287,1.,0.923879532511287,1.,0.923879532511287,1.,0.923879532511287,
1.,0.923879532511287,1.,0.923879532511287,1.,0.923879532511287,1.,0.923879532511287,
1.,0.923879532511287,1.,0.923879532511287,1.,0.923879532511287,1.,0.923879532511287,
1.,0.923879532511287,1.,0.923879532511287,1.,0.923879532511287,1.,0.923879532511287,
1.,0.923879532511287,1.,0.923879532511287,1.,0.923879532511287,1.,0.923879532511287,
1.,0.923879532511287,1.,0.923879532511287,1.,0.923879532511287,1.,0.923879532511287,
1.,0.923879532511287,1.,0.923879532511287,1.,0.923879532511287,1.,0.923879532511287,
1.,0.923879532511287,1.,0.923879532511287,1.,0.923879532511287,1.,0.923879532511287,
1.,0.923879532511287,1.,0.923879532511287,1.,0.923879532511287,1.,0.923879532511287,
1.,0.923879532511287,1.,0.923879532511287,1.,0.923879532511287,1.,0.923879532511287,
1.,0.923879532511287,1.,0.923879532511287,1.,0.923879532511287,1.,0.923879532511287,
1.,0.923879532511287,1.,0.923879532511287,1.,0.923879532511287,1.,0.923879532511287,
1.,0.923879532511287,1.,0.923879532511287,1.,0.923879532511287,1.,0.923879532511287,
1.,0.923879532511287,1.,0.923879532511287,1.,0.923879532511287,1.)))
REPRESENTATION_ITEM('')
SURFACE()
);
#576=(
BOUNDED_SURFACE()
B_SPLINE_SURFACE(1,2,((#28989,#28990,#28991,#28992,#28993,#28994,#28995,
#28996,#28997,#28998,#28999,#29000,#29001,#29002,#29003,#29004,#29005,#29006,
#29007,#29008,#29009,#29010,#29011,#29012,#29013,#29014,#29015,#29016,#29017,
#29018,#29019,#29020,#29021,#29022,#29023,#29024,#29025,#29026,#29027,#29028,
#29029,#29030,#29031,#29032,#29033,#29034,#29035,#29036,#29037,#29038,#29039,
#29040,#29041,#29042,#29043,#29044,#29045,#29046,#29047,#29048,#29049,#29050,
#29051,#29052,#29053,#29054,#29055,#29056,#29057,#29058,#29059,#29060,#29061,
#29062,#29063,#29064,#29065,#29066,#29067,#29068,#29069,#29070,#29071,#29072,
#29073,#29074,#29075,#29076,#29077,#29078,#29079,#29080,#29081,#29082,#29083,
#29084,#29085,#29086,#29087,#29088,#29089,#29090,#29091,#29092,#29093,#29094,
#29095,#29096,#29097,#29098,#29099,#29100,#29101,#29102,#29103,#29104,#29105,
#29106,#29107,#29108,#29109,#29110,#29111,#29112,#29113,#29114,#29115,#29116,
#29117,#29118,#29119,#29120,#29121,#29122,#29123,#29124,#29125,#29126,#29127,
#29128,#29129,#29130,#29131,#29132,#29133,#29134,#29135,#29136,#29137,#29138,
#29139,#29140,#29141,#29142,#29143,#29144,#29145,#29146,#29147,#29148,#29149),
(#29150,#29151,#29152,#29153,#29154,#29155,#29156,#29157,#29158,#29159,
#29160,#29161,#29162,#29163,#29164,#29165,#29166,#29167,#29168,#29169,#29170,
#29171,#29172,#29173,#29174,#29175,#29176,#29177,#29178,#29179,#29180,#29181,
#29182,#29183,#29184,#29185,#29186,#29187,#29188,#29189,#29190,#29191,#29192,
#29193,#29194,#29195,#29196,#29197,#29198,#29199,#29200,#29201,#29202,#29203,
#29204,#29205,#29206,#29207,#29208,#29209,#29210,#29211,#29212,#29213,#29214,
#29215,#29216,#29217,#29218,#29219,#29220,#29221,#29222,#29223,#29224,#29225,
#29226,#29227,#29228,#29229,#29230,#29231,#29232,#29233,#29234,#29235,#29236,
#29237,#29238,#29239,#29240,#29241,#29242,#29243,#29244,#29245,#29246,#29247,
#29248,#29249,#29250,#29251,#29252,#29253,#29254,#29255,#29256,#29257,#29258,
#29259,#29260,#29261,#29262,#29263,#29264,#29265,#29266,#29267,#29268,#29269,
#29270,#29271,#29272,#29273,#29274,#29275,#29276,#29277,#29278,#29279,#29280,
#29281,#29282,#29283,#29284,#29285,#29286,#29287,#29288,#29289,#29290,#29291,
#29292,#29293,#29294,#29295,#29296,#29297,#29298,#29299,#29300,#29301,#29302,
#29303,#29304,#29305,#29306,#29307,#29308,#29309,#29310)),.UNSPECIFIED.,
 .F.,.F.,.F.)
B_SPLINE_SURFACE_WITH_KNOTS((2,2),(3,2,2,2,2,2,2,2,2,2,2,2,2,2,2,2,2,2,
2,2,2,2,2,2,2,2,2,2,2,2,2,2,2,2,2,2,2,2,2,2,2,2,2,2,2,2,2,2,2,2,2,2,2,2,
2,2,2,2,2,2,2,2,2,2,2,2,2,2,2,2,2,2,2,2,2,2,2,2,2,2,3),(0.,1.),(0.,0.0125,
0.025,0.0375,0.05,0.0625,0.075,0.0875,0.1,0.1125,0.125,0.1375,0.15,0.1625,
0.175,0.1875,0.2,0.2125,0.225,0.2375,0.25,0.2625,0.275,0.2875,0.3,0.3125,
0.325,0.3375,0.35,0.3625,0.375,0.3875,0.4,0.4125,0.425,0.4375,0.45,0.4625,
0.475,0.4875,0.5,0.5125,0.525,0.5375,0.55,0.5625,0.575,0.5875,0.6,0.6125,
0.625,0.6375,0.65,0.6625,0.675,0.6875,0.7,0.7125,0.725,0.7375,0.75,0.7625,
0.775,0.7875,0.8,0.8125,0.825,0.8375,0.85,0.8625,0.875,0.8875,0.9,0.9125,
0.925,0.9375,0.95,0.9625,0.975,0.9875,1.),.UNSPECIFIED.)
GEOMETRIC_REPRESENTATION_ITEM()
RATIONAL_B_SPLINE_SURFACE(((1.,0.923879532511287,1.,0.923879532511287,1.,
0.923879532511287,1.,0.923879532511287,1.,0.923879532511287,1.,0.923879532511287,
1.,0.923879532511287,1.,0.923879532511287,1.,0.923879532511287,1.,0.923879532511287,
1.,0.923879532511287,1.,0.923879532511287,1.,0.923879532511287,1.,0.923879532511287,
1.,0.923879532511287,1.,0.923879532511287,1.,0.923879532511287,1.,0.923879532511287,
1.,0.923879532511287,1.,0.923879532511287,1.,0.923879532511287,1.,0.923879532511287,
1.,0.923879532511287,1.,0.923879532511287,1.,0.923879532511287,1.,0.923879532511287,
1.,0.923879532511287,1.,0.923879532511287,1.,0.923879532511287,1.,0.923879532511287,
1.,0.923879532511287,1.,0.923879532511287,1.,0.923879532511287,1.,0.923879532511287,
1.,0.923879532511287,1.,0.923879532511287,1.,0.923879532511287,1.,0.923879532511287,
1.,0.923879532511287,1.,0.923879532511287,1.,0.923879532511287,1.,0.923879532511287,
1.,0.923879532511287,1.,0.923879532511287,1.,0.923879532511287,1.,0.923879532511287,
1.,0.923879532511287,1.,0.923879532511287,1.,0.923879532511287,1.,0.923879532511287,
1.,0.923879532511287,1.,0.923879532511287,1.,0.923879532511287,1.,0.923879532511287,
1.,0.923879532511287,1.,0.923879532511287,1.,0.923879532511287,1.,0.923879532511287,
1.,0.923879532511287,1.,0.923879532511287,1.,0.923879532511287,1.,0.923879532511287,
1.,0.923879532511287,1.,0.923879532511287,1.,0.923879532511287,1.,0.923879532511287,
1.,0.923879532511287,1.,0.923879532511287,1.,0.923879532511287,1.,0.923879532511287,
1.,0.923879532511287,1.,0.923879532511287,1.,0.923879532511287,1.,0.923879532511287,
1.,0.923879532511287,1.,0.923879532511287,1.,0.923879532511287,1.,0.923879532511287,
1.,0.923879532511287,1.,0.923879532511287,1.),(1.,0.923879532511287,1.,
0.923879532511287,1.,0.923879532511287,1.,0.923879532511287,1.,0.923879532511287,
1.,0.923879532511287,1.,0.923879532511287,1.,0.923879532511287,1.,0.923879532511287,
1.,0.923879532511287,1.,0.923879532511287,1.,0.923879532511287,1.,0.923879532511287,
1.,0.923879532511287,1.,0.923879532511287,1.,0.923879532511287,1.,0.923879532511287,
1.,0.923879532511287,1.,0.923879532511287,1.,0.923879532511287,1.,0.923879532511287,
1.,0.923879532511287,1.,0.923879532511287,1.,0.923879532511287,1.,0.923879532511287,
1.,0.923879532511287,1.,0.923879532511287,1.,0.923879532511287,1.,0.923879532511287,
1.,0.923879532511287,1.,0.923879532511287,1.,0.923879532511287,1.,0.923879532511287,
1.,0.923879532511287,1.,0.923879532511287,1.,0.923879532511287,1.,0.923879532511287,
1.,0.923879532511287,1.,0.923879532511287,1.,0.923879532511287,1.,0.923879532511287,
1.,0.923879532511287,1.,0.923879532511287,1.,0.923879532511287,1.,0.923879532511287,
1.,0.923879532511287,1.,0.923879532511287,1.,0.923879532511287,1.,0.923879532511287,
1.,0.923879532511287,1.,0.923879532511287,1.,0.923879532511287,1.,0.923879532511287,
1.,0.923879532511287,1.,0.923879532511287,1.,0.923879532511287,1.,0.923879532511287,
1.,0.923879532511287,1.,0.923879532511287,1.,0.923879532511287,1.,0.923879532511287,
1.,0.923879532511287,1.,0.923879532511287,1.,0.923879532511287,1.,0.923879532511287,
1.,0.923879532511287,1.,0.923879532511287,1.,0.923879532511287,1.,0.923879532511287,
1.,0.923879532511287,1.,0.923879532511287,1.,0.923879532511287,1.,0.923879532511287,
1.,0.923879532511287,1.,0.923879532511287,1.,0.923879532511287,1.,0.923879532511287,
1.,0.923879532511287,1.,0.923879532511287,1.,0.923879532511287,1.)))
REPRESENTATION_ITEM('')
SURFACE()
);
#577=(
BOUNDED_SURFACE()
B_SPLINE_SURFACE(3,2,((#29328,#29329,#29330,#29331,#29332,#29333,#29334,
#29335,#29336,#29337,#29338,#29339,#29340,#29341,#29342,#29343,#29344,#29345,
#29346,#29347,#29348,#29349,#29350,#29351,#29352,#29353,#29354,#29355,#29356,
#29357,#29358,#29359,#29360,#29361,#29362,#29363,#29364,#29365,#29366,#29367,
#29368,#29369,#29370,#29371,#29372,#29373,#29374,#29375,#29376,#29377,#29378,
#29379,#29380,#29381,#29382,#29383,#29384,#29385,#29386,#29387,#29388,#29389,
#29390,#29391,#29392,#29393,#29394,#29395,#29396,#29397,#29398,#29399,#29400,
#29401,#29402,#29403,#29404,#29405,#29406,#29407,#29408,#29409,#29410,#29411,
#29412,#29413,#29414,#29415,#29416,#29417,#29418,#29419,#29420,#29421,#29422,
#29423,#29424,#29425,#29426,#29427,#29428,#29429,#29430,#29431,#29432,#29433,
#29434,#29435,#29436,#29437,#29438,#29439,#29440,#29441,#29442,#29443,#29444,
#29445,#29446,#29447,#29448,#29449,#29450,#29451,#29452,#29453,#29454,#29455,
#29456,#29457,#29458,#29459,#29460,#29461,#29462,#29463,#29464,#29465,#29466,
#29467,#29468,#29469,#29470,#29471,#29472,#29473,#29474,#29475,#29476,#29477,
#29478,#29479,#29480,#29481,#29482,#29483,#29484,#29485,#29486,#29487,#29488),
(#29489,#29490,#29491,#29492,#29493,#29494,#29495,#29496,#29497,#29498,
#29499,#29500,#29501,#29502,#29503,#29504,#29505,#29506,#29507,#29508,#29509,
#29510,#29511,#29512,#29513,#29514,#29515,#29516,#29517,#29518,#29519,#29520,
#29521,#29522,#29523,#29524,#29525,#29526,#29527,#29528,#29529,#29530,#29531,
#29532,#29533,#29534,#29535,#29536,#29537,#29538,#29539,#29540,#29541,#29542,
#29543,#29544,#29545,#29546,#29547,#29548,#29549,#29550,#29551,#29552,#29553,
#29554,#29555,#29556,#29557,#29558,#29559,#29560,#29561,#29562,#29563,#29564,
#29565,#29566,#29567,#29568,#29569,#29570,#29571,#29572,#29573,#29574,#29575,
#29576,#29577,#29578,#29579,#29580,#29581,#29582,#29583,#29584,#29585,#29586,
#29587,#29588,#29589,#29590,#29591,#29592,#29593,#29594,#29595,#29596,#29597,
#29598,#29599,#29600,#29601,#29602,#29603,#29604,#29605,#29606,#29607,#29608,
#29609,#29610,#29611,#29612,#29613,#29614,#29615,#29616,#29617,#29618,#29619,
#29620,#29621,#29622,#29623,#29624,#29625,#29626,#29627,#29628,#29629,#29630,
#29631,#29632,#29633,#29634,#29635,#29636,#29637,#29638,#29639,#29640,#29641,
#29642,#29643,#29644,#29645,#29646,#29647,#29648,#29649),(#29650,#29651,
#29652,#29653,#29654,#29655,#29656,#29657,#29658,#29659,#29660,#29661,#29662,
#29663,#29664,#29665,#29666,#29667,#29668,#29669,#29670,#29671,#29672,#29673,
#29674,#29675,#29676,#29677,#29678,#29679,#29680,#29681,#29682,#29683,#29684,
#29685,#29686,#29687,#29688,#29689,#29690,#29691,#29692,#29693,#29694,#29695,
#29696,#29697,#29698,#29699,#29700,#29701,#29702,#29703,#29704,#29705,#29706,
#29707,#29708,#29709,#29710,#29711,#29712,#29713,#29714,#29715,#29716,#29717,
#29718,#29719,#29720,#29721,#29722,#29723,#29724,#29725,#29726,#29727,#29728,
#29729,#29730,#29731,#29732,#29733,#29734,#29735,#29736,#29737,#29738,#29739,
#29740,#29741,#29742,#29743,#29744,#29745,#29746,#29747,#29748,#29749,#29750,
#29751,#29752,#29753,#29754,#29755,#29756,#29757,#29758,#29759,#29760,#29761,
#29762,#29763,#29764,#29765,#29766,#29767,#29768,#29769,#29770,#29771,#29772,
#29773,#29774,#29775,#29776,#29777,#29778,#29779,#29780,#29781,#29782,#29783,
#29784,#29785,#29786,#29787,#29788,#29789,#29790,#29791,#29792,#29793,#29794,
#29795,#29796,#29797,#29798,#29799,#29800,#29801,#29802,#29803,#29804,#29805,
#29806,#29807,#29808,#29809,#29810),(#29811,#29812,#29813,#29814,#29815,
#29816,#29817,#29818,#29819,#29820,#29821,#29822,#29823,#29824,#29825,#29826,
#29827,#29828,#29829,#29830,#29831,#29832,#29833,#29834,#29835,#29836,#29837,
#29838,#29839,#29840,#29841,#29842,#29843,#29844,#29845,#29846,#29847,#29848,
#29849,#29850,#29851,#29852,#29853,#29854,#29855,#29856,#29857,#29858,#29859,
#29860,#29861,#29862,#29863,#29864,#29865,#29866,#29867,#29868,#29869,#29870,
#29871,#29872,#29873,#29874,#29875,#29876,#29877,#29878,#29879,#29880,#29881,
#29882,#29883,#29884,#29885,#29886,#29887,#29888,#29889,#29890,#29891,#29892,
#29893,#29894,#29895,#29896,#29897,#29898,#29899,#29900,#29901,#29902,#29903,
#29904,#29905,#29906,#29907,#29908,#29909,#29910,#29911,#29912,#29913,#29914,
#29915,#29916,#29917,#29918,#29919,#29920,#29921,#29922,#29923,#29924,#29925,
#29926,#29927,#29928,#29929,#29930,#29931,#29932,#29933,#29934,#29935,#29936,
#29937,#29938,#29939,#29940,#29941,#29942,#29943,#29944,#29945,#29946,#29947,
#29948,#29949,#29950,#29951,#29952,#29953,#29954,#29955,#29956,#29957,#29958,
#29959,#29960,#29961,#29962,#29963,#29964,#29965,#29966,#29967,#29968,#29969,
#29970,#29971)),.UNSPECIFIED.,.F.,.F.,.F.)
B_SPLINE_SURFACE_WITH_KNOTS((4,4),(3,2,2,2,2,2,2,2,2,2,2,2,2,2,2,2,2,2,
2,2,2,2,2,2,2,2,2,2,2,2,2,2,2,2,2,2,2,2,2,2,2,2,2,2,2,2,2,2,2,2,2,2,2,2,
2,2,2,2,2,2,2,2,2,2,2,2,2,2,2,2,2,2,2,2,2,2,2,2,2,2,3),(0.,1.),(0.,0.0125,
0.025,0.0375,0.05,0.0625,0.075,0.0875,0.1,0.1125,0.125,0.1375,0.15,0.1625,
0.175,0.1875,0.2,0.2125,0.225,0.2375,0.25,0.2625,0.275,0.2875,0.3,0.3125,
0.325,0.3375,0.35,0.3625,0.375,0.3875,0.4,0.4125,0.425,0.4375,0.45,0.4625,
0.475,0.4875,0.5,0.5125,0.525,0.5375,0.55,0.5625,0.575,0.5875,0.6,0.6125,
0.625,0.6375,0.65,0.6625,0.675,0.6875,0.7,0.7125,0.725,0.7375,0.75,0.7625,
0.775,0.7875,0.8,0.8125,0.825,0.8375,0.85,0.8625,0.875,0.8875,0.9,0.9125,
0.925,0.9375,0.95,0.9625,0.975,0.9875,1.),.UNSPECIFIED.)
GEOMETRIC_REPRESENTATION_ITEM()
RATIONAL_B_SPLINE_SURFACE(((1.,0.923879532511287,1.,0.923879532511287,1.,
0.923879532511287,1.,0.923879532511287,1.,0.923879532511287,1.,0.923879532511287,
1.,0.923879532511287,1.,0.923879532511287,1.,0.923879532511287,1.,0.923879532511287,
1.,0.923879532511287,1.,0.923879532511287,1.,0.923879532511287,1.,0.923879532511287,
1.,0.923879532511287,1.,0.923879532511287,1.,0.923879532511287,1.,0.923879532511287,
1.,0.923879532511287,1.,0.923879532511287,1.,0.923879532511287,1.,0.923879532511287,
1.,0.923879532511287,1.,0.923879532511287,1.,0.923879532511287,1.,0.923879532511287,
1.,0.923879532511287,1.,0.923879532511287,1.,0.923879532511287,1.,0.923879532511287,
1.,0.923879532511287,1.,0.923879532511287,1.,0.923879532511287,1.,0.923879532511287,
1.,0.923879532511287,1.,0.923879532511287,1.,0.923879532511287,1.,0.923879532511287,
1.,0.923879532511287,1.,0.923879532511287,1.,0.923879532511287,1.,0.923879532511287,
1.,0.923879532511287,1.,0.923879532511287,1.,0.923879532511287,1.,0.923879532511287,
1.,0.923879532511287,1.,0.923879532511287,1.,0.923879532511287,1.,0.923879532511287,
1.,0.923879532511287,1.,0.923879532511287,1.,0.923879532511287,1.,0.923879532511287,
1.,0.923879532511287,1.,0.923879532511287,1.,0.923879532511287,1.,0.923879532511287,
1.,0.923879532511287,1.,0.923879532511287,1.,0.923879532511287,1.,0.923879532511287,
1.,0.923879532511287,1.,0.923879532511287,1.,0.923879532511287,1.,0.923879532511287,
1.,0.923879532511287,1.,0.923879532511287,1.,0.923879532511287,1.,0.923879532511287,
1.,0.923879532511287,1.,0.923879532511287,1.,0.923879532511287,1.,0.923879532511287,
1.,0.923879532511287,1.,0.923879532511287,1.,0.923879532511287,1.,0.923879532511287,
1.,0.923879532511287,1.,0.923879532511287,1.),(0.998696642611305,0.922675387296324,
0.998696642611305,0.922675387296324,0.998696642611305,0.922675387296324,
0.998696642611305,0.922675387296324,0.998696642611305,0.922675387296324,
0.998696642611305,0.922675387296324,0.998696642611305,0.922675387296324,
0.998696642611305,0.922675387296324,0.998696642611305,0.922675387296324,
0.998696642611305,0.922675387296324,0.998696642611305,0.922675387296324,
0.998696642611305,0.922675387296324,0.998696642611305,0.922675387296324,
0.998696642611305,0.922675387296324,0.998696642611305,0.922675387296324,
0.998696642611305,0.922675387296324,0.998696642611305,0.922675387296324,
0.998696642611305,0.922675387296324,0.998696642611305,0.922675387296324,
0.998696642611305,0.922675387296324,0.998696642611305,0.922675387296324,
0.998696642611305,0.922675387296324,0.998696642611305,0.922675387296324,
0.998696642611305,0.922675387296324,0.998696642611305,0.922675387296324,
0.998696642611305,0.922675387296324,0.998696642611305,0.922675387296324,
0.998696642611305,0.922675387296324,0.998696642611305,0.922675387296324,
0.998696642611305,0.922675387296324,0.998696642611305,0.922675387296324,
0.998696642611305,0.922675387296324,0.998696642611305,0.922675387296324,
0.998696642611305,0.922675387296324,0.998696642611305,0.922675387296324,
0.998696642611305,0.922675387296324,0.998696642611305,0.922675387296324,
0.998696642611305,0.922675387296324,0.998696642611305,0.922675387296324,
0.998696642611305,0.922675387296324,0.998696642611305,0.922675387296324,
0.998696642611305,0.922675387296324,0.998696642611305,0.922675387296324,
0.998696642611305,0.922675387296324,0.998696642611305,0.922675387296324,
0.998696642611305,0.922675387296324,0.998696642611305,0.922675387296324,
0.998696642611305,0.922675387296324,0.998696642611305,0.922675387296324,
0.998696642611305,0.922675387296324,0.998696642611305,0.922675387296324,
0.998696642611305,0.922675387296324,0.998696642611305,0.922675387296324,
0.998696642611305,0.922675387296324,0.998696642611305,0.922675387296324,
0.998696642611305,0.922675387296324,0.998696642611305,0.922675387296324,
0.998696642611305,0.922675387296324,0.998696642611305,0.922675387296324,
0.998696642611305,0.922675387296324,0.998696642611305,0.922675387296324,
0.998696642611305,0.922675387296324,0.998696642611305,0.922675387296324,
0.998696642611305,0.922675387296324,0.998696642611305,0.922675387296324,
0.998696642611305,0.922675387296324,0.998696642611305,0.922675387296324,
0.998696642611305,0.922675387296324,0.998696642611305,0.922675387296324,
0.998696642611305,0.922675387296324,0.998696642611305,0.922675387296324,
0.998696642611305,0.922675387296324,0.998696642611305,0.922675387296324,
0.998696642611305,0.922675387296324,0.998696642611305,0.922675387296324,
0.998696642611305,0.922675387296324,0.998696642611305,0.922675387296324,
0.998696642611305,0.922675387296324,0.998696642611305,0.922675387296324,
0.998696642611305,0.922675387296324,0.998696642611305),(0.998696642611305,
0.922675387296324,0.998696642611305,0.922675387296324,0.998696642611305,
0.922675387296324,0.998696642611305,0.922675387296324,0.998696642611305,
0.922675387296324,0.998696642611305,0.922675387296324,0.998696642611305,
0.922675387296324,0.998696642611305,0.922675387296324,0.998696642611305,
0.922675387296324,0.998696642611305,0.922675387296324,0.998696642611305,
0.922675387296324,0.998696642611305,0.922675387296324,0.998696642611305,
0.922675387296324,0.998696642611305,0.922675387296324,0.998696642611305,
0.922675387296324,0.998696642611305,0.922675387296324,0.998696642611305,
0.922675387296324,0.998696642611305,0.922675387296324,0.998696642611305,
0.922675387296324,0.998696642611305,0.922675387296324,0.998696642611305,
0.922675387296324,0.998696642611305,0.922675387296324,0.998696642611305,
0.922675387296324,0.998696642611305,0.922675387296324,0.998696642611305,
0.922675387296324,0.998696642611305,0.922675387296324,0.998696642611305,
0.922675387296324,0.998696642611305,0.922675387296324,0.998696642611305,
0.922675387296324,0.998696642611305,0.922675387296324,0.998696642611305,
0.922675387296324,0.998696642611305,0.922675387296324,0.998696642611305,
0.922675387296324,0.998696642611305,0.922675387296324,0.998696642611305,
0.922675387296324,0.998696642611305,0.922675387296324,0.998696642611305,
0.922675387296324,0.998696642611305,0.922675387296324,0.998696642611305,
0.922675387296324,0.998696642611305,0.922675387296324,0.998696642611305,
0.922675387296324,0.998696642611305,0.922675387296324,0.998696642611305,
0.922675387296324,0.998696642611305,0.922675387296324,0.998696642611305,
0.922675387296324,0.998696642611305,0.922675387296324,0.998696642611305,
0.922675387296324,0.998696642611305,0.922675387296324,0.998696642611305,
0.922675387296324,0.998696642611305,0.922675387296324,0.998696642611305,
0.922675387296324,0.998696642611305,0.922675387296324,0.998696642611305,
0.922675387296324,0.998696642611305,0.922675387296324,0.998696642611305,
0.922675387296324,0.998696642611305,0.922675387296324,0.998696642611305,
0.922675387296324,0.998696642611305,0.922675387296324,0.998696642611305,
0.922675387296324,0.998696642611305,0.922675387296324,0.998696642611305,
0.922675387296324,0.998696642611305,0.922675387296324,0.998696642611305,
0.922675387296324,0.998696642611305,0.922675387296324,0.998696642611305,
0.922675387296324,0.998696642611305,0.922675387296324,0.998696642611305,
0.922675387296324,0.998696642611305,0.922675387296324,0.998696642611305,
0.922675387296324,0.998696642611305,0.922675387296324,0.998696642611305,
0.922675387296324,0.998696642611305,0.922675387296324,0.998696642611305,
0.922675387296324,0.998696642611305,0.922675387296324,0.998696642611305,
0.922675387296324,0.998696642611305,0.922675387296324,0.998696642611305,
0.922675387296324,0.998696642611305,0.922675387296324,0.998696642611305,
0.922675387296324,0.998696642611305,0.922675387296324,0.998696642611305),
(1.,0.923879532511287,1.,0.923879532511287,1.,0.923879532511287,1.,0.923879532511287,
1.,0.923879532511287,1.,0.923879532511287,1.,0.923879532511287,1.,0.923879532511287,
1.,0.923879532511287,1.,0.923879532511287,1.,0.923879532511287,1.,0.923879532511287,
1.,0.923879532511287,1.,0.923879532511287,1.,0.923879532511287,1.,0.923879532511287,
1.,0.923879532511287,1.,0.923879532511287,1.,0.923879532511287,1.,0.923879532511287,
1.,0.923879532511287,1.,0.923879532511287,1.,0.923879532511287,1.,0.923879532511287,
1.,0.923879532511287,1.,0.923879532511287,1.,0.923879532511287,1.,0.923879532511287,
1.,0.923879532511287,1.,0.923879532511287,1.,0.923879532511287,1.,0.923879532511287,
1.,0.923879532511287,1.,0.923879532511287,1.,0.923879532511287,1.,0.923879532511287,
1.,0.923879532511287,1.,0.923879532511287,1.,0.923879532511287,1.,0.923879532511287,
1.,0.923879532511287,1.,0.923879532511287,1.,0.923879532511287,1.,0.923879532511287,
1.,0.923879532511287,1.,0.923879532511287,1.,0.923879532511287,1.,0.923879532511287,
1.,0.923879532511287,1.,0.923879532511287,1.,0.923879532511287,1.,0.923879532511287,
1.,0.923879532511287,1.,0.923879532511287,1.,0.923879532511287,1.,0.923879532511287,
1.,0.923879532511287,1.,0.923879532511287,1.,0.923879532511287,1.,0.923879532511287,
1.,0.923879532511287,1.,0.923879532511287,1.,0.923879532511287,1.,0.923879532511287,
1.,0.923879532511287,1.,0.923879532511287,1.,0.923879532511287,1.,0.923879532511287,
1.,0.923879532511287,1.,0.923879532511287,1.,0.923879532511287,1.,0.923879532511287,
1.,0.923879532511287,1.,0.923879532511287,1.,0.923879532511287,1.,0.923879532511287,
1.,0.923879532511287,1.,0.923879532511287,1.,0.923879532511287,1.,0.923879532511287,
1.)))
REPRESENTATION_ITEM('')
SURFACE()
);
#578=(
BOUNDED_SURFACE()
B_SPLINE_SURFACE(1,2,((#29972,#29973,#29974,#29975,#29976,#29977,#29978,
#29979,#29980,#29981,#29982,#29983,#29984,#29985,#29986,#29987,#29988,#29989,
#29990,#29991,#29992,#29993,#29994,#29995,#29996,#29997,#29998,#29999,#30000,
#30001,#30002,#30003,#30004,#30005,#30006,#30007,#30008,#30009,#30010,#30011,
#30012,#30013,#30014,#30015,#30016,#30017,#30018,#30019,#30020,#30021,#30022,
#30023,#30024,#30025,#30026,#30027,#30028,#30029,#30030,#30031,#30032,#30033,
#30034,#30035,#30036,#30037,#30038,#30039,#30040,#30041,#30042,#30043,#30044,
#30045,#30046,#30047,#30048,#30049,#30050,#30051,#30052,#30053,#30054,#30055,
#30056,#30057,#30058,#30059,#30060,#30061,#30062,#30063,#30064,#30065,#30066,
#30067,#30068,#30069,#30070,#30071,#30072,#30073,#30074,#30075,#30076,#30077,
#30078,#30079,#30080,#30081,#30082,#30083,#30084,#30085,#30086,#30087,#30088,
#30089,#30090,#30091,#30092,#30093,#30094,#30095,#30096,#30097,#30098,#30099,
#30100,#30101,#30102,#30103,#30104,#30105,#30106,#30107,#30108,#30109,#30110,
#30111,#30112,#30113,#30114,#30115,#30116,#30117,#30118,#30119,#30120,#30121,
#30122,#30123,#30124,#30125,#30126,#30127,#30128,#30129,#30130,#30131,#30132),
(#30133,#30134,#30135,#30136,#30137,#30138,#30139,#30140,#30141,#30142,
#30143,#30144,#30145,#30146,#30147,#30148,#30149,#30150,#30151,#30152,#30153,
#30154,#30155,#30156,#30157,#30158,#30159,#30160,#30161,#30162,#30163,#30164,
#30165,#30166,#30167,#30168,#30169,#30170,#30171,#30172,#30173,#30174,#30175,
#30176,#30177,#30178,#30179,#30180,#30181,#30182,#30183,#30184,#30185,#30186,
#30187,#30188,#30189,#30190,#30191,#30192,#30193,#30194,#30195,#30196,#30197,
#30198,#30199,#30200,#30201,#30202,#30203,#30204,#30205,#30206,#30207,#30208,
#30209,#30210,#30211,#30212,#30213,#30214,#30215,#30216,#30217,#30218,#30219,
#30220,#30221,#30222,#30223,#30224,#30225,#30226,#30227,#30228,#30229,#30230,
#30231,#30232,#30233,#30234,#30235,#30236,#30237,#30238,#30239,#30240,#30241,
#30242,#30243,#30244,#30245,#30246,#30247,#30248,#30249,#30250,#30251,#30252,
#30253,#30254,#30255,#30256,#30257,#30258,#30259,#30260,#30261,#30262,#30263,
#30264,#30265,#30266,#30267,#30268,#30269,#30270,#30271,#30272,#30273,#30274,
#30275,#30276,#30277,#30278,#30279,#30280,#30281,#30282,#30283,#30284,#30285,
#30286,#30287,#30288,#30289,#30290,#30291,#30292,#30293)),.UNSPECIFIED.,
 .F.,.F.,.F.)
B_SPLINE_SURFACE_WITH_KNOTS((2,2),(3,2,2,2,2,2,2,2,2,2,2,2,2,2,2,2,2,2,
2,2,2,2,2,2,2,2,2,2,2,2,2,2,2,2,2,2,2,2,2,2,2,2,2,2,2,2,2,2,2,2,2,2,2,2,
2,2,2,2,2,2,2,2,2,2,2,2,2,2,2,2,2,2,2,2,2,2,2,2,2,2,3),(0.,1.),(0.,0.0125,
0.025,0.0375,0.05,0.0625,0.075,0.0875,0.1,0.1125,0.125,0.1375,0.15,0.1625,
0.175,0.1875,0.2,0.2125,0.225,0.2375,0.25,0.2625,0.275,0.2875,0.3,0.3125,
0.325,0.3375,0.35,0.3625,0.375,0.3875,0.4,0.4125,0.425,0.4375,0.45,0.4625,
0.475,0.4875,0.5,0.5125,0.525,0.5375,0.55,0.5625,0.575,0.5875,0.6,0.6125,
0.625,0.6375,0.65,0.6625,0.675,0.6875,0.7,0.7125,0.725,0.7375,0.75,0.7625,
0.775,0.7875,0.8,0.8125,0.825,0.8375,0.85,0.8625,0.875,0.8875,0.9,0.9125,
0.925,0.9375,0.95,0.9625,0.975,0.9875,1.),.UNSPECIFIED.)
GEOMETRIC_REPRESENTATION_ITEM()
RATIONAL_B_SPLINE_SURFACE(((1.,0.923879532511287,1.,0.923879532511287,1.,
0.923879532511287,1.,0.923879532511287,1.,0.923879532511287,1.,0.923879532511287,
1.,0.923879532511287,1.,0.923879532511287,1.,0.923879532511287,1.,0.923879532511287,
1.,0.923879532511287,1.,0.923879532511287,1.,0.923879532511287,1.,0.923879532511287,
1.,0.923879532511287,1.,0.923879532511287,1.,0.923879532511287,1.,0.923879532511287,
1.,0.923879532511287,1.,0.923879532511287,1.,0.923879532511287,1.,0.923879532511287,
1.,0.923879532511287,1.,0.923879532511287,1.,0.923879532511287,1.,0.923879532511287,
1.,0.923879532511287,1.,0.923879532511287,1.,0.923879532511287,1.,0.923879532511287,
1.,0.923879532511287,1.,0.923879532511287,1.,0.923879532511287,1.,0.923879532511287,
1.,0.923879532511287,1.,0.923879532511287,1.,0.923879532511287,1.,0.923879532511287,
1.,0.923879532511287,1.,0.923879532511287,1.,0.923879532511287,1.,0.923879532511287,
1.,0.923879532511287,1.,0.923879532511287,1.,0.923879532511287,1.,0.923879532511287,
1.,0.923879532511287,1.,0.923879532511287,1.,0.923879532511287,1.,0.923879532511287,
1.,0.923879532511287,1.,0.923879532511287,1.,0.923879532511287,1.,0.923879532511287,
1.,0.923879532511287,1.,0.923879532511287,1.,0.923879532511287,1.,0.923879532511287,
1.,0.923879532511287,1.,0.923879532511287,1.,0.923879532511287,1.,0.923879532511287,
1.,0.923879532511287,1.,0.923879532511287,1.,0.923879532511287,1.,0.923879532511287,
1.,0.923879532511287,1.,0.923879532511287,1.,0.923879532511287,1.,0.923879532511287,
1.,0.923879532511287,1.,0.923879532511287,1.,0.923879532511287,1.,0.923879532511287,
1.,0.923879532511287,1.,0.923879532511287,1.,0.923879532511287,1.,0.923879532511287,
1.,0.923879532511287,1.,0.923879532511287,1.),(1.,0.923879532511287,1.,
0.923879532511287,1.,0.923879532511287,1.,0.923879532511287,1.,0.923879532511287,
1.,0.923879532511287,1.,0.923879532511287,1.,0.923879532511287,1.,0.923879532511287,
1.,0.923879532511287,1.,0.923879532511287,1.,0.923879532511287,1.,0.923879532511287,
1.,0.923879532511287,1.,0.923879532511287,1.,0.923879532511287,1.,0.923879532511287,
1.,0.923879532511287,1.,0.923879532511287,1.,0.923879532511287,1.,0.923879532511287,
1.,0.923879532511287,1.,0.923879532511287,1.,0.923879532511287,1.,0.923879532511287,
1.,0.923879532511287,1.,0.923879532511287,1.,0.923879532511287,1.,0.923879532511287,
1.,0.923879532511287,1.,0.923879532511287,1.,0.923879532511287,1.,0.923879532511287,
1.,0.923879532511287,1.,0.923879532511287,1.,0.923879532511287,1.,0.923879532511287,
1.,0.923879532511287,1.,0.923879532511287,1.,0.923879532511287,1.,0.923879532511287,
1.,0.923879532511287,1.,0.923879532511287,1.,0.923879532511287,1.,0.923879532511287,
1.,0.923879532511287,1.,0.923879532511287,1.,0.923879532511287,1.,0.923879532511287,
1.,0.923879532511287,1.,0.923879532511287,1.,0.923879532511287,1.,0.923879532511287,
1.,0.923879532511287,1.,0.923879532511287,1.,0.923879532511287,1.,0.923879532511287,
1.,0.923879532511287,1.,0.923879532511287,1.,0.923879532511287,1.,0.923879532511287,
1.,0.923879532511287,1.,0.923879532511287,1.,0.923879532511287,1.,0.923879532511287,
1.,0.923879532511287,1.,0.923879532511287,1.,0.923879532511287,1.,0.923879532511287,
1.,0.923879532511287,1.,0.923879532511287,1.,0.923879532511287,1.,0.923879532511287,
1.,0.923879532511287,1.,0.923879532511287,1.,0.923879532511287,1.,0.923879532511287,
1.,0.923879532511287,1.,0.923879532511287,1.,0.923879532511287,1.)))
REPRESENTATION_ITEM('')
SURFACE()
);
#579=(
BOUNDED_SURFACE()
B_SPLINE_SURFACE(1,2,((#30311,#30312,#30313,#30314,#30315,#30316,#30317,
#30318,#30319,#30320,#30321,#30322,#30323,#30324,#30325,#30326,#30327,#30328,
#30329,#30330,#30331,#30332,#30333,#30334,#30335,#30336,#30337,#30338,#30339,
#30340,#30341,#30342,#30343,#30344,#30345,#30346,#30347,#30348,#30349,#30350,
#30351,#30352,#30353,#30354,#30355,#30356,#30357,#30358,#30359,#30360,#30361,
#30362,#30363,#30364,#30365,#30366,#30367,#30368,#30369,#30370,#30371,#30372,
#30373,#30374,#30375,#30376,#30377,#30378,#30379,#30380,#30381,#30382,#30383,
#30384,#30385,#30386,#30387,#30388,#30389,#30390,#30391,#30392,#30393,#30394,
#30395,#30396,#30397,#30398,#30399,#30400,#30401,#30402,#30403,#30404,#30405,
#30406,#30407,#30408,#30409,#30410,#30411,#30412,#30413,#30414,#30415,#30416,
#30417,#30418,#30419,#30420,#30421,#30422,#30423,#30424,#30425,#30426,#30427,
#30428,#30429,#30430,#30431,#30432,#30433,#30434,#30435,#30436,#30437,#30438,
#30439,#30440,#30441,#30442,#30443,#30444,#30445,#30446,#30447,#30448,#30449,
#30450,#30451,#30452,#30453,#30454,#30455,#30456,#30457,#30458,#30459,#30460,
#30461,#30462,#30463,#30464,#30465,#30466,#30467,#30468,#30469,#30470,#30471),
(#30472,#30473,#30474,#30475,#30476,#30477,#30478,#30479,#30480,#30481,
#30482,#30483,#30484,#30485,#30486,#30487,#30488,#30489,#30490,#30491,#30492,
#30493,#30494,#30495,#30496,#30497,#30498,#30499,#30500,#30501,#30502,#30503,
#30504,#30505,#30506,#30507,#30508,#30509,#30510,#30511,#30512,#30513,#30514,
#30515,#30516,#30517,#30518,#30519,#30520,#30521,#30522,#30523,#30524,#30525,
#30526,#30527,#30528,#30529,#30530,#30531,#30532,#30533,#30534,#30535,#30536,
#30537,#30538,#30539,#30540,#30541,#30542,#30543,#30544,#30545,#30546,#30547,
#30548,#30549,#30550,#30551,#30552,#30553,#30554,#30555,#30556,#30557,#30558,
#30559,#30560,#30561,#30562,#30563,#30564,#30565,#30566,#30567,#30568,#30569,
#30570,#30571,#30572,#30573,#30574,#30575,#30576,#30577,#30578,#30579,#30580,
#30581,#30582,#30583,#30584,#30585,#30586,#30587,#30588,#30589,#30590,#30591,
#30592,#30593,#30594,#30595,#30596,#30597,#30598,#30599,#30600,#30601,#30602,
#30603,#30604,#30605,#30606,#30607,#30608,#30609,#30610,#30611,#30612,#30613,
#30614,#30615,#30616,#30617,#30618,#30619,#30620,#30621,#30622,#30623,#30624,
#30625,#30626,#30627,#30628,#30629,#30630,#30631,#30632)),.UNSPECIFIED.,
 .F.,.F.,.F.)
B_SPLINE_SURFACE_WITH_KNOTS((2,2),(3,2,2,2,2,2,2,2,2,2,2,2,2,2,2,2,2,2,
2,2,2,2,2,2,2,2,2,2,2,2,2,2,2,2,2,2,2,2,2,2,2,2,2,2,2,2,2,2,2,2,2,2,2,2,
2,2,2,2,2,2,2,2,2,2,2,2,2,2,2,2,2,2,2,2,2,2,2,2,2,2,3),(0.,1.),(0.,0.0125,
0.025,0.0375,0.05,0.0625,0.075,0.0875,0.1,0.1125,0.125,0.1375,0.15,0.1625,
0.175,0.1875,0.2,0.2125,0.225,0.2375,0.25,0.2625,0.275,0.2875,0.3,0.3125,
0.325,0.3375,0.35,0.3625,0.375,0.3875,0.4,0.4125,0.425,0.4375,0.45,0.4625,
0.475,0.4875,0.5,0.5125,0.525,0.5375,0.55,0.5625,0.575,0.5875,0.6,0.6125,
0.625,0.6375,0.65,0.6625,0.675,0.6875,0.7,0.7125,0.725,0.7375,0.75,0.7625,
0.775,0.7875,0.8,0.8125,0.825,0.8375,0.85,0.8625,0.875,0.8875,0.9,0.9125,
0.925,0.9375,0.95,0.9625,0.975,0.9875,1.),.UNSPECIFIED.)
GEOMETRIC_REPRESENTATION_ITEM()
RATIONAL_B_SPLINE_SURFACE(((1.,0.923879532511287,1.,0.923879532511287,1.,
0.923879532511287,1.,0.923879532511287,1.,0.923879532511287,1.,0.923879532511287,
1.,0.923879532511287,1.,0.923879532511287,1.,0.923879532511287,1.,0.923879532511287,
1.,0.923879532511287,1.,0.923879532511287,1.,0.923879532511287,1.,0.923879532511287,
1.,0.923879532511287,1.,0.923879532511287,1.,0.923879532511287,1.,0.923879532511287,
1.,0.923879532511287,1.,0.923879532511287,1.,0.923879532511287,1.,0.923879532511287,
1.,0.923879532511287,1.,0.923879532511287,1.,0.923879532511287,1.,0.923879532511287,
1.,0.923879532511287,1.,0.923879532511287,1.,0.923879532511287,1.,0.923879532511287,
1.,0.923879532511287,1.,0.923879532511287,1.,0.923879532511287,1.,0.923879532511287,
1.,0.923879532511287,1.,0.923879532511287,1.,0.923879532511287,1.,0.923879532511287,
1.,0.923879532511287,1.,0.923879532511287,1.,0.923879532511287,1.,0.923879532511287,
1.,0.923879532511287,1.,0.923879532511287,1.,0.923879532511287,1.,0.923879532511287,
1.,0.923879532511287,1.,0.923879532511287,1.,0.923879532511287,1.,0.923879532511287,
1.,0.923879532511287,1.,0.923879532511287,1.,0.923879532511287,1.,0.923879532511287,
1.,0.923879532511287,1.,0.923879532511287,1.,0.923879532511287,1.,0.923879532511287,
1.,0.923879532511287,1.,0.923879532511287,1.,0.923879532511287,1.,0.923879532511287,
1.,0.923879532511287,1.,0.923879532511287,1.,0.923879532511287,1.,0.923879532511287,
1.,0.923879532511287,1.,0.923879532511287,1.,0.923879532511287,1.,0.923879532511287,
1.,0.923879532511287,1.,0.923879532511287,1.,0.923879532511287,1.,0.923879532511287,
1.,0.923879532511287,1.,0.923879532511287,1.,0.923879532511287,1.,0.923879532511287,
1.,0.923879532511287,1.,0.923879532511287,1.),(1.,0.923879532511287,1.,
0.923879532511287,1.,0.923879532511287,1.,0.923879532511287,1.,0.923879532511287,
1.,0.923879532511287,1.,0.923879532511287,1.,0.923879532511287,1.,0.923879532511287,
1.,0.923879532511287,1.,0.923879532511287,1.,0.923879532511287,1.,0.923879532511287,
1.,0.923879532511287,1.,0.923879532511287,1.,0.923879532511287,1.,0.923879532511287,
1.,0.923879532511287,1.,0.923879532511287,1.,0.923879532511287,1.,0.923879532511287,
1.,0.923879532511287,1.,0.923879532511287,1.,0.923879532511287,1.,0.923879532511287,
1.,0.923879532511287,1.,0.923879532511287,1.,0.923879532511287,1.,0.923879532511287,
1.,0.923879532511287,1.,0.923879532511287,1.,0.923879532511287,1.,0.923879532511287,
1.,0.923879532511287,1.,0.923879532511287,1.,0.923879532511287,1.,0.923879532511287,
1.,0.923879532511287,1.,0.923879532511287,1.,0.923879532511287,1.,0.923879532511287,
1.,0.923879532511287,1.,0.923879532511287,1.,0.923879532511287,1.,0.923879532511287,
1.,0.923879532511287,1.,0.923879532511287,1.,0.923879532511287,1.,0.923879532511287,
1.,0.923879532511287,1.,0.923879532511287,1.,0.923879532511287,1.,0.923879532511287,
1.,0.923879532511287,1.,0.923879532511287,1.,0.923879532511287,1.,0.923879532511287,
1.,0.923879532511287,1.,0.923879532511287,1.,0.923879532511287,1.,0.923879532511287,
1.,0.923879532511287,1.,0.923879532511287,1.,0.923879532511287,1.,0.923879532511287,
1.,0.923879532511287,1.,0.923879532511287,1.,0.923879532511287,1.,0.923879532511287,
1.,0.923879532511287,1.,0.923879532511287,1.,0.923879532511287,1.,0.923879532511287,
1.,0.923879532511287,1.,0.923879532511287,1.,0.923879532511287,1.,0.923879532511287,
1.,0.923879532511287,1.,0.923879532511287,1.,0.923879532511287,1.)))
REPRESENTATION_ITEM('')
SURFACE()
);
#580=(
BOUNDED_SURFACE()
B_SPLINE_SURFACE(3,2,((#30650,#30651,#30652,#30653,#30654,#30655,#30656,
#30657,#30658,#30659,#30660,#30661,#30662,#30663,#30664,#30665,#30666,#30667,
#30668,#30669,#30670,#30671,#30672,#30673,#30674,#30675,#30676,#30677,#30678,
#30679,#30680,#30681,#30682,#30683,#30684,#30685,#30686,#30687,#30688,#30689,
#30690,#30691,#30692,#30693,#30694,#30695,#30696,#30697,#30698,#30699,#30700,
#30701,#30702,#30703,#30704,#30705,#30706,#30707,#30708,#30709,#30710,#30711,
#30712,#30713,#30714,#30715,#30716,#30717,#30718,#30719,#30720,#30721,#30722,
#30723,#30724,#30725,#30726,#30727,#30728,#30729,#30730,#30731,#30732,#30733,
#30734,#30735,#30736,#30737,#30738,#30739,#30740,#30741,#30742,#30743,#30744,
#30745,#30746,#30747,#30748,#30749,#30750,#30751,#30752,#30753,#30754,#30755,
#30756,#30757,#30758,#30759,#30760,#30761,#30762,#30763,#30764,#30765,#30766,
#30767,#30768,#30769,#30770,#30771,#30772,#30773,#30774,#30775,#30776,#30777,
#30778,#30779,#30780,#30781,#30782,#30783,#30784,#30785,#30786,#30787,#30788,
#30789,#30790,#30791,#30792,#30793,#30794,#30795,#30796,#30797,#30798,#30799,
#30800,#30801,#30802,#30803,#30804,#30805,#30806,#30807,#30808,#30809,#30810),
(#30811,#30812,#30813,#30814,#30815,#30816,#30817,#30818,#30819,#30820,
#30821,#30822,#30823,#30824,#30825,#30826,#30827,#30828,#30829,#30830,#30831,
#30832,#30833,#30834,#30835,#30836,#30837,#30838,#30839,#30840,#30841,#30842,
#30843,#30844,#30845,#30846,#30847,#30848,#30849,#30850,#30851,#30852,#30853,
#30854,#30855,#30856,#30857,#30858,#30859,#30860,#30861,#30862,#30863,#30864,
#30865,#30866,#30867,#30868,#30869,#30870,#30871,#30872,#30873,#30874,#30875,
#30876,#30877,#30878,#30879,#30880,#30881,#30882,#30883,#30884,#30885,#30886,
#30887,#30888,#30889,#30890,#30891,#30892,#30893,#30894,#30895,#30896,#30897,
#30898,#30899,#30900,#30901,#30902,#30903,#30904,#30905,#30906,#30907,#30908,
#30909,#30910,#30911,#30912,#30913,#30914,#30915,#30916,#30917,#30918,#30919,
#30920,#30921,#30922,#30923,#30924,#30925,#30926,#30927,#30928,#30929,#30930,
#30931,#30932,#30933,#30934,#30935,#30936,#30937,#30938,#30939,#30940,#30941,
#30942,#30943,#30944,#30945,#30946,#30947,#30948,#30949,#30950,#30951,#30952,
#30953,#30954,#30955,#30956,#30957,#30958,#30959,#30960,#30961,#30962,#30963,
#30964,#30965,#30966,#30967,#30968,#30969,#30970,#30971),(#30972,#30973,
#30974,#30975,#30976,#30977,#30978,#30979,#30980,#30981,#30982,#30983,#30984,
#30985,#30986,#30987,#30988,#30989,#30990,#30991,#30992,#30993,#30994,#30995,
#30996,#30997,#30998,#30999,#31000,#31001,#31002,#31003,#31004,#31005,#31006,
#31007,#31008,#31009,#31010,#31011,#31012,#31013,#31014,#31015,#31016,#31017,
#31018,#31019,#31020,#31021,#31022,#31023,#31024,#31025,#31026,#31027,#31028,
#31029,#31030,#31031,#31032,#31033,#31034,#31035,#31036,#31037,#31038,#31039,
#31040,#31041,#31042,#31043,#31044,#31045,#31046,#31047,#31048,#31049,#31050,
#31051,#31052,#31053,#31054,#31055,#31056,#31057,#31058,#31059,#31060,#31061,
#31062,#31063,#31064,#31065,#31066,#31067,#31068,#31069,#31070,#31071,#31072,
#31073,#31074,#31075,#31076,#31077,#31078,#31079,#31080,#31081,#31082,#31083,
#31084,#31085,#31086,#31087,#31088,#31089,#31090,#31091,#31092,#31093,#31094,
#31095,#31096,#31097,#31098,#31099,#31100,#31101,#31102,#31103,#31104,#31105,
#31106,#31107,#31108,#31109,#31110,#31111,#31112,#31113,#31114,#31115,#31116,
#31117,#31118,#31119,#31120,#31121,#31122,#31123,#31124,#31125,#31126,#31127,
#31128,#31129,#31130,#31131,#31132),(#31133,#31134,#31135,#31136,#31137,
#31138,#31139,#31140,#31141,#31142,#31143,#31144,#31145,#31146,#31147,#31148,
#31149,#31150,#31151,#31152,#31153,#31154,#31155,#31156,#31157,#31158,#31159,
#31160,#31161,#31162,#31163,#31164,#31165,#31166,#31167,#31168,#31169,#31170,
#31171,#31172,#31173,#31174,#31175,#31176,#31177,#31178,#31179,#31180,#31181,
#31182,#31183,#31184,#31185,#31186,#31187,#31188,#31189,#31190,#31191,#31192,
#31193,#31194,#31195,#31196,#31197,#31198,#31199,#31200,#31201,#31202,#31203,
#31204,#31205,#31206,#31207,#31208,#31209,#31210,#31211,#31212,#31213,#31214,
#31215,#31216,#31217,#31218,#31219,#31220,#31221,#31222,#31223,#31224,#31225,
#31226,#31227,#31228,#31229,#31230,#31231,#31232,#31233,#31234,#31235,#31236,
#31237,#31238,#31239,#31240,#31241,#31242,#31243,#31244,#31245,#31246,#31247,
#31248,#31249,#31250,#31251,#31252,#31253,#31254,#31255,#31256,#31257,#31258,
#31259,#31260,#31261,#31262,#31263,#31264,#31265,#31266,#31267,#31268,#31269,
#31270,#31271,#31272,#31273,#31274,#31275,#31276,#31277,#31278,#31279,#31280,
#31281,#31282,#31283,#31284,#31285,#31286,#31287,#31288,#31289,#31290,#31291,
#31292,#31293)),.UNSPECIFIED.,.F.,.F.,.F.)
B_SPLINE_SURFACE_WITH_KNOTS((4,4),(3,2,2,2,2,2,2,2,2,2,2,2,2,2,2,2,2,2,
2,2,2,2,2,2,2,2,2,2,2,2,2,2,2,2,2,2,2,2,2,2,2,2,2,2,2,2,2,2,2,2,2,2,2,2,
2,2,2,2,2,2,2,2,2,2,2,2,2,2,2,2,2,2,2,2,2,2,2,2,2,2,3),(0.,1.),(0.,0.0125,
0.025,0.0375,0.05,0.0625,0.075,0.0875,0.1,0.1125,0.125,0.1375,0.15,0.1625,
0.175,0.1875,0.2,0.2125,0.225,0.2375,0.25,0.2625,0.275,0.2875,0.3,0.3125,
0.325,0.3375,0.35,0.3625,0.375,0.3875,0.4,0.4125,0.425,0.4375,0.45,0.4625,
0.475,0.4875,0.5,0.5125,0.525,0.5375,0.55,0.5625,0.575,0.5875,0.6,0.6125,
0.625,0.6375,0.65,0.6625,0.675,0.6875,0.7,0.7125,0.725,0.7375,0.75,0.7625,
0.775,0.7875,0.8,0.8125,0.825,0.8375,0.85,0.8625,0.875,0.8875,0.9,0.9125,
0.925,0.9375,0.95,0.9625,0.975,0.9875,1.),.UNSPECIFIED.)
GEOMETRIC_REPRESENTATION_ITEM()
RATIONAL_B_SPLINE_SURFACE(((1.,0.923879532511287,1.,0.923879532511287,1.,
0.923879532511287,1.,0.923879532511287,1.,0.923879532511287,1.,0.923879532511287,
1.,0.923879532511287,1.,0.923879532511287,1.,0.923879532511287,1.,0.923879532511287,
1.,0.923879532511287,1.,0.923879532511287,1.,0.923879532511287,1.,0.923879532511287,
1.,0.923879532511287,1.,0.923879532511287,1.,0.923879532511287,1.,0.923879532511287,
1.,0.923879532511287,1.,0.923879532511287,1.,0.923879532511287,1.,0.923879532511287,
1.,0.923879532511287,1.,0.923879532511287,1.,0.923879532511287,1.,0.923879532511287,
1.,0.923879532511287,1.,0.923879532511287,1.,0.923879532511287,1.,0.923879532511287,
1.,0.923879532511287,1.,0.923879532511287,1.,0.923879532511287,1.,0.923879532511287,
1.,0.923879532511287,1.,0.923879532511287,1.,0.923879532511287,1.,0.923879532511287,
1.,0.923879532511287,1.,0.923879532511287,1.,0.923879532511287,1.,0.923879532511287,
1.,0.923879532511287,1.,0.923879532511287,1.,0.923879532511287,1.,0.923879532511287,
1.,0.923879532511287,1.,0.923879532511287,1.,0.923879532511287,1.,0.923879532511287,
1.,0.923879532511287,1.,0.923879532511287,1.,0.923879532511287,1.,0.923879532511287,
1.,0.923879532511287,1.,0.923879532511287,1.,0.923879532511287,1.,0.923879532511287,
1.,0.923879532511287,1.,0.923879532511287,1.,0.923879532511287,1.,0.923879532511287,
1.,0.923879532511287,1.,0.923879532511287,1.,0.923879532511287,1.,0.923879532511287,
1.,0.923879532511287,1.,0.923879532511287,1.,0.923879532511287,1.,0.923879532511287,
1.,0.923879532511287,1.,0.923879532511287,1.,0.923879532511287,1.,0.923879532511287,
1.,0.923879532511287,1.,0.923879532511287,1.,0.923879532511287,1.,0.923879532511287,
1.,0.923879532511287,1.,0.923879532511287,1.),(0.998696642611305,0.922675387296324,
0.998696642611305,0.922675387296324,0.998696642611305,0.922675387296324,
0.998696642611305,0.922675387296324,0.998696642611305,0.922675387296324,
0.998696642611305,0.922675387296324,0.998696642611305,0.922675387296324,
0.998696642611305,0.922675387296324,0.998696642611305,0.922675387296324,
0.998696642611305,0.922675387296324,0.998696642611305,0.922675387296324,
0.998696642611305,0.922675387296324,0.998696642611305,0.922675387296324,
0.998696642611305,0.922675387296324,0.998696642611305,0.922675387296324,
0.998696642611305,0.922675387296324,0.998696642611305,0.922675387296324,
0.998696642611305,0.922675387296324,0.998696642611305,0.922675387296324,
0.998696642611305,0.922675387296324,0.998696642611305,0.922675387296324,
0.998696642611305,0.922675387296324,0.998696642611305,0.922675387296324,
0.998696642611305,0.922675387296324,0.998696642611305,0.922675387296324,
0.998696642611305,0.922675387296324,0.998696642611305,0.922675387296324,
0.998696642611305,0.922675387296324,0.998696642611305,0.922675387296324,
0.998696642611305,0.922675387296324,0.998696642611305,0.922675387296324,
0.998696642611305,0.922675387296324,0.998696642611305,0.922675387296324,
0.998696642611305,0.922675387296324,0.998696642611305,0.922675387296324,
0.998696642611305,0.922675387296324,0.998696642611305,0.922675387296324,
0.998696642611305,0.922675387296324,0.998696642611305,0.922675387296324,
0.998696642611305,0.922675387296324,0.998696642611305,0.922675387296324,
0.998696642611305,0.922675387296324,0.998696642611305,0.922675387296324,
0.998696642611305,0.922675387296324,0.998696642611305,0.922675387296324,
0.998696642611305,0.922675387296324,0.998696642611305,0.922675387296324,
0.998696642611305,0.922675387296324,0.998696642611305,0.922675387296324,
0.998696642611305,0.922675387296324,0.998696642611305,0.922675387296324,
0.998696642611305,0.922675387296324,0.998696642611305,0.922675387296324,
0.998696642611305,0.922675387296324,0.998696642611305,0.922675387296324,
0.998696642611305,0.922675387296324,0.998696642611305,0.922675387296324,
0.998696642611305,0.922675387296324,0.998696642611305,0.922675387296324,
0.998696642611305,0.922675387296324,0.998696642611305,0.922675387296324,
0.998696642611305,0.922675387296324,0.998696642611305,0.922675387296324,
0.998696642611305,0.922675387296324,0.998696642611305,0.922675387296324,
0.998696642611305,0.922675387296324,0.998696642611305,0.922675387296324,
0.998696642611305,0.922675387296324,0.998696642611305,0.922675387296324,
0.998696642611305,0.922675387296324,0.998696642611305,0.922675387296324,
0.998696642611305,0.922675387296324,0.998696642611305,0.922675387296324,
0.998696642611305,0.922675387296324,0.998696642611305,0.922675387296324,
0.998696642611305,0.922675387296324,0.998696642611305,0.922675387296324,
0.998696642611305,0.922675387296324,0.998696642611305,0.922675387296324,
0.998696642611305,0.922675387296324,0.998696642611305),(0.998696642611305,
0.922675387296324,0.998696642611305,0.922675387296324,0.998696642611305,
0.922675387296324,0.998696642611305,0.922675387296324,0.998696642611305,
0.922675387296324,0.998696642611305,0.922675387296324,0.998696642611305,
0.922675387296324,0.998696642611305,0.922675387296324,0.998696642611305,
0.922675387296324,0.998696642611305,0.922675387296324,0.998696642611305,
0.922675387296324,0.998696642611305,0.922675387296324,0.998696642611305,
0.922675387296324,0.998696642611305,0.922675387296324,0.998696642611305,
0.922675387296324,0.998696642611305,0.922675387296324,0.998696642611305,
0.922675387296324,0.998696642611305,0.922675387296324,0.998696642611305,
0.922675387296324,0.998696642611305,0.922675387296324,0.998696642611305,
0.922675387296324,0.998696642611305,0.922675387296324,0.998696642611305,
0.922675387296324,0.998696642611305,0.922675387296324,0.998696642611305,
0.922675387296324,0.998696642611305,0.922675387296324,0.998696642611305,
0.922675387296324,0.998696642611305,0.922675387296324,0.998696642611305,
0.922675387296324,0.998696642611305,0.922675387296324,0.998696642611305,
0.922675387296324,0.998696642611305,0.922675387296324,0.998696642611305,
0.922675387296324,0.998696642611305,0.922675387296324,0.998696642611305,
0.922675387296324,0.998696642611305,0.922675387296324,0.998696642611305,
0.922675387296324,0.998696642611305,0.922675387296324,0.998696642611305,
0.922675387296324,0.998696642611305,0.922675387296324,0.998696642611305,
0.922675387296324,0.998696642611305,0.922675387296324,0.998696642611305,
0.922675387296324,0.998696642611305,0.922675387296324,0.998696642611305,
0.922675387296324,0.998696642611305,0.922675387296324,0.998696642611305,
0.922675387296324,0.998696642611305,0.922675387296324,0.998696642611305,
0.922675387296324,0.998696642611305,0.922675387296324,0.998696642611305,
0.922675387296324,0.998696642611305,0.922675387296324,0.998696642611305,
0.922675387296324,0.998696642611305,0.922675387296324,0.998696642611305,
0.922675387296324,0.998696642611305,0.922675387296324,0.998696642611305,
0.922675387296324,0.998696642611305,0.922675387296324,0.998696642611305,
0.922675387296324,0.998696642611305,0.922675387296324,0.998696642611305,
0.922675387296324,0.998696642611305,0.922675387296324,0.998696642611305,
0.922675387296324,0.998696642611305,0.922675387296324,0.998696642611305,
0.922675387296324,0.998696642611305,0.922675387296324,0.998696642611305,
0.922675387296324,0.998696642611305,0.922675387296324,0.998696642611305,
0.922675387296324,0.998696642611305,0.922675387296324,0.998696642611305,
0.922675387296324,0.998696642611305,0.922675387296324,0.998696642611305,
0.922675387296324,0.998696642611305,0.922675387296324,0.998696642611305,
0.922675387296324,0.998696642611305,0.922675387296324,0.998696642611305,
0.922675387296324,0.998696642611305,0.922675387296324,0.998696642611305,
0.922675387296324,0.998696642611305,0.922675387296324,0.998696642611305),
(1.,0.923879532511287,1.,0.923879532511287,1.,0.923879532511287,1.,0.923879532511287,
1.,0.923879532511287,1.,0.923879532511287,1.,0.923879532511287,1.,0.923879532511287,
1.,0.923879532511287,1.,0.923879532511287,1.,0.923879532511287,1.,0.923879532511287,
1.,0.923879532511287,1.,0.923879532511287,1.,0.923879532511287,1.,0.923879532511287,
1.,0.923879532511287,1.,0.923879532511287,1.,0.923879532511287,1.,0.923879532511287,
1.,0.923879532511287,1.,0.923879532511287,1.,0.923879532511287,1.,0.923879532511287,
1.,0.923879532511287,1.,0.923879532511287,1.,0.923879532511287,1.,0.923879532511287,
1.,0.923879532511287,1.,0.923879532511287,1.,0.923879532511287,1.,0.923879532511287,
1.,0.923879532511287,1.,0.923879532511287,1.,0.923879532511287,1.,0.923879532511287,
1.,0.923879532511287,1.,0.923879532511287,1.,0.923879532511287,1.,0.923879532511287,
1.,0.923879532511287,1.,0.923879532511287,1.,0.923879532511287,1.,0.923879532511287,
1.,0.923879532511287,1.,0.923879532511287,1.,0.923879532511287,1.,0.923879532511287,
1.,0.923879532511287,1.,0.923879532511287,1.,0.923879532511287,1.,0.923879532511287,
1.,0.923879532511287,1.,0.923879532511287,1.,0.923879532511287,1.,0.923879532511287,
1.,0.923879532511287,1.,0.923879532511287,1.,0.923879532511287,1.,0.923879532511287,
1.,0.923879532511287,1.,0.923879532511287,1.,0.923879532511287,1.,0.923879532511287,
1.,0.923879532511287,1.,0.923879532511287,1.,0.923879532511287,1.,0.923879532511287,
1.,0.923879532511287,1.,0.923879532511287,1.,0.923879532511287,1.,0.923879532511287,
1.,0.923879532511287,1.,0.923879532511287,1.,0.923879532511287,1.,0.923879532511287,
1.,0.923879532511287,1.,0.923879532511287,1.,0.923879532511287,1.,0.923879532511287,
1.)))
REPRESENTATION_ITEM('')
SURFACE()
);
#581=(
BOUNDED_SURFACE()
B_SPLINE_SURFACE(1,2,((#31294,#31295,#31296,#31297,#31298,#31299,#31300,
#31301,#31302,#31303,#31304,#31305,#31306,#31307,#31308,#31309,#31310,#31311,
#31312,#31313,#31314,#31315,#31316,#31317,#31318,#31319,#31320,#31321,#31322,
#31323,#31324,#31325,#31326,#31327,#31328,#31329,#31330,#31331,#31332,#31333,
#31334,#31335,#31336,#31337,#31338,#31339,#31340,#31341,#31342,#31343,#31344,
#31345,#31346,#31347,#31348,#31349,#31350,#31351,#31352,#31353,#31354,#31355,
#31356,#31357,#31358,#31359,#31360,#31361,#31362,#31363,#31364,#31365,#31366,
#31367,#31368,#31369,#31370,#31371,#31372,#31373,#31374,#31375,#31376,#31377,
#31378,#31379,#31380,#31381,#31382,#31383,#31384,#31385,#31386,#31387,#31388,
#31389,#31390,#31391,#31392,#31393,#31394,#31395,#31396,#31397,#31398,#31399,
#31400,#31401,#31402,#31403,#31404,#31405,#31406,#31407,#31408,#31409,#31410,
#31411,#31412,#31413,#31414,#31415,#31416,#31417,#31418,#31419,#31420,#31421,
#31422,#31423,#31424,#31425,#31426,#31427,#31428,#31429,#31430,#31431,#31432,
#31433,#31434,#31435,#31436,#31437,#31438,#31439,#31440,#31441,#31442,#31443,
#31444,#31445,#31446,#31447,#31448,#31449,#31450,#31451,#31452,#31453,#31454),
(#31455,#31456,#31457,#31458,#31459,#31460,#31461,#31462,#31463,#31464,
#31465,#31466,#31467,#31468,#31469,#31470,#31471,#31472,#31473,#31474,#31475,
#31476,#31477,#31478,#31479,#31480,#31481,#31482,#31483,#31484,#31485,#31486,
#31487,#31488,#31489,#31490,#31491,#31492,#31493,#31494,#31495,#31496,#31497,
#31498,#31499,#31500,#31501,#31502,#31503,#31504,#31505,#31506,#31507,#31508,
#31509,#31510,#31511,#31512,#31513,#31514,#31515,#31516,#31517,#31518,#31519,
#31520,#31521,#31522,#31523,#31524,#31525,#31526,#31527,#31528,#31529,#31530,
#31531,#31532,#31533,#31534,#31535,#31536,#31537,#31538,#31539,#31540,#31541,
#31542,#31543,#31544,#31545,#31546,#31547,#31548,#31549,#31550,#31551,#31552,
#31553,#31554,#31555,#31556,#31557,#31558,#31559,#31560,#31561,#31562,#31563,
#31564,#31565,#31566,#31567,#31568,#31569,#31570,#31571,#31572,#31573,#31574,
#31575,#31576,#31577,#31578,#31579,#31580,#31581,#31582,#31583,#31584,#31585,
#31586,#31587,#31588,#31589,#31590,#31591,#31592,#31593,#31594,#31595,#31596,
#31597,#31598,#31599,#31600,#31601,#31602,#31603,#31604,#31605,#31606,#31607,
#31608,#31609,#31610,#31611,#31612,#31613,#31614,#31615)),.UNSPECIFIED.,
 .F.,.F.,.F.)
B_SPLINE_SURFACE_WITH_KNOTS((2,2),(3,2,2,2,2,2,2,2,2,2,2,2,2,2,2,2,2,2,
2,2,2,2,2,2,2,2,2,2,2,2,2,2,2,2,2,2,2,2,2,2,2,2,2,2,2,2,2,2,2,2,2,2,2,2,
2,2,2,2,2,2,2,2,2,2,2,2,2,2,2,2,2,2,2,2,2,2,2,2,2,2,3),(0.,1.00000731743925),
(0.,0.0125,0.025,0.0375,0.05,0.0625,0.075,0.0875,0.1,0.1125,0.125,0.1375,
0.15,0.1625,0.175,0.1875,0.2,0.2125,0.225,0.2375,0.25,0.2625,0.275,0.2875,
0.3,0.3125,0.325,0.3375,0.35,0.3625,0.375,0.3875,0.4,0.4125,0.425,0.4375,
0.45,0.4625,0.475,0.4875,0.5,0.5125,0.525,0.5375,0.55,0.5625,0.575,0.5875,
0.6,0.6125,0.625,0.6375,0.65,0.6625,0.675,0.6875,0.7,0.7125,0.725,0.7375,
0.75,0.7625,0.775,0.7875,0.8,0.8125,0.825,0.8375,0.85,0.8625,0.875,0.8875,
0.9,0.9125,0.925,0.9375,0.95,0.9625,0.975,0.9875,1.),.UNSPECIFIED.)
GEOMETRIC_REPRESENTATION_ITEM()
RATIONAL_B_SPLINE_SURFACE(((1.,0.923879532511287,1.,0.923879532511287,1.,
0.923879532511287,1.,0.923879532511287,1.,0.923879532511287,1.,0.923879532511287,
1.,0.923879532511287,1.,0.923879532511287,1.,0.923879532511287,1.,0.923879532511287,
1.,0.923879532511287,1.,0.923879532511287,1.,0.923879532511287,1.,0.923879532511287,
1.,0.923879532511287,1.,0.923879532511287,1.,0.923879532511287,1.,0.923879532511287,
1.,0.923879532511287,1.,0.923879532511287,1.,0.923879532511287,1.,0.923879532511287,
1.,0.923879532511287,1.,0.923879532511287,1.,0.923879532511287,1.,0.923879532511287,
1.,0.923879532511287,1.,0.923879532511287,1.,0.923879532511287,1.,0.923879532511287,
1.,0.923879532511287,1.,0.923879532511287,1.,0.923879532511287,1.,0.923879532511287,
1.,0.923879532511287,1.,0.923879532511287,1.,0.923879532511287,1.,0.923879532511287,
1.,0.923879532511287,1.,0.923879532511287,1.,0.923879532511287,1.,0.923879532511287,
1.,0.923879532511287,1.,0.923879532511287,1.,0.923879532511287,1.,0.923879532511287,
1.,0.923879532511287,1.,0.923879532511287,1.,0.923879532511287,1.,0.923879532511287,
1.,0.923879532511287,1.,0.923879532511287,1.,0.923879532511287,1.,0.923879532511287,
1.,0.923879532511287,1.,0.923879532511287,1.,0.923879532511287,1.,0.923879532511287,
1.,0.923879532511287,1.,0.923879532511287,1.,0.923879532511287,1.,0.923879532511287,
1.,0.923879532511287,1.,0.923879532511287,1.,0.923879532511287,1.,0.923879532511287,
1.,0.923879532511287,1.,0.923879532511287,1.,0.923879532511287,1.,0.923879532511287,
1.,0.923879532511287,1.,0.923879532511287,1.,0.923879532511287,1.,0.923879532511287,
1.,0.923879532511287,1.,0.923879532511287,1.,0.923879532511287,1.,0.923879532511287,
1.,0.923879532511287,1.,0.923879532511287,1.),(1.,0.923879532511287,1.,
0.923879532511287,1.,0.923879532511287,1.,0.923879532511287,1.,0.923879532511287,
1.,0.923879532511287,1.,0.923879532511287,1.,0.923879532511287,1.,0.923879532511287,
1.,0.923879532511287,1.,0.923879532511287,1.,0.923879532511287,1.,0.923879532511287,
1.,0.923879532511287,1.,0.923879532511287,1.,0.923879532511287,1.,0.923879532511287,
1.,0.923879532511287,1.,0.923879532511287,1.,0.923879532511287,1.,0.923879532511287,
1.,0.923879532511287,1.,0.923879532511287,1.,0.923879532511287,1.,0.923879532511287,
1.,0.923879532511287,1.,0.923879532511287,1.,0.923879532511287,1.,0.923879532511287,
1.,0.923879532511287,1.,0.923879532511287,1.,0.923879532511287,1.,0.923879532511287,
1.,0.923879532511287,1.,0.923879532511287,1.,0.923879532511287,1.,0.923879532511287,
1.,0.923879532511287,1.,0.923879532511287,1.,0.923879532511287,1.,0.923879532511287,
1.,0.923879532511287,1.,0.923879532511287,1.,0.923879532511287,1.,0.923879532511287,
1.,0.923879532511287,1.,0.923879532511287,1.,0.923879532511287,1.,0.923879532511287,
1.,0.923879532511287,1.,0.923879532511287,1.,0.923879532511287,1.,0.923879532511287,
1.,0.923879532511287,1.,0.923879532511287,1.,0.923879532511287,1.,0.923879532511287,
1.,0.923879532511287,1.,0.923879532511287,1.,0.923879532511287,1.,0.923879532511287,
1.,0.923879532511287,1.,0.923879532511287,1.,0.923879532511287,1.,0.923879532511287,
1.,0.923879532511287,1.,0.923879532511287,1.,0.923879532511287,1.,0.923879532511287,
1.,0.923879532511287,1.,0.923879532511287,1.,0.923879532511287,1.,0.923879532511287,
1.,0.923879532511287,1.,0.923879532511287,1.,0.923879532511287,1.,0.923879532511287,
1.,0.923879532511287,1.,0.923879532511287,1.,0.923879532511287,1.)))
REPRESENTATION_ITEM('')
SURFACE()
);
#582=(
BOUNDED_SURFACE()
B_SPLINE_SURFACE(3,2,((#31621,#31622,#31623,#31624,#31625,#31626,#31627,
#31628,#31629,#31630,#31631,#31632,#31633,#31634,#31635,#31636,#31637,#31638,
#31639,#31640,#31641,#31642,#31643,#31644,#31645,#31646,#31647,#31648,#31649,
#31650,#31651,#31652,#31653,#31654,#31655,#31656,#31657,#31658,#31659,#31660,
#31661,#31662,#31663,#31664,#31665,#31666,#31667,#31668,#31669,#31670,#31671,
#31672,#31673,#31674,#31675,#31676,#31677,#31678,#31679,#31680,#31681,#31682,
#31683,#31684,#31685,#31686,#31687,#31688,#31689,#31690,#31691,#31692,#31693,
#31694,#31695,#31696,#31697,#31698,#31699,#31700,#31701,#31702,#31703,#31704,
#31705,#31706,#31707,#31708,#31709,#31710,#31711,#31712,#31713,#31714,#31715,
#31716,#31717,#31718,#31719,#31720,#31721,#31722,#31723,#31724,#31725,#31726,
#31727,#31728,#31729,#31730,#31731,#31732,#31733,#31734,#31735,#31736,#31737,
#31738,#31739,#31740,#31741,#31742,#31743,#31744,#31745,#31746,#31747,#31748,
#31749,#31750,#31751,#31752,#31753,#31754,#31755,#31756,#31757,#31758,#31759,
#31760,#31761,#31762,#31763,#31764,#31765,#31766,#31767,#31768,#31769,#31770,
#31771,#31772,#31773,#31774,#31775,#31776,#31777,#31778,#31779,#31780,#31781),
(#31782,#31783,#31784,#31785,#31786,#31787,#31788,#31789,#31790,#31791,
#31792,#31793,#31794,#31795,#31796,#31797,#31798,#31799,#31800,#31801,#31802,
#31803,#31804,#31805,#31806,#31807,#31808,#31809,#31810,#31811,#31812,#31813,
#31814,#31815,#31816,#31817,#31818,#31819,#31820,#31821,#31822,#31823,#31824,
#31825,#31826,#31827,#31828,#31829,#31830,#31831,#31832,#31833,#31834,#31835,
#31836,#31837,#31838,#31839,#31840,#31841,#31842,#31843,#31844,#31845,#31846,
#31847,#31848,#31849,#31850,#31851,#31852,#31853,#31854,#31855,#31856,#31857,
#31858,#31859,#31860,#31861,#31862,#31863,#31864,#31865,#31866,#31867,#31868,
#31869,#31870,#31871,#31872,#31873,#31874,#31875,#31876,#31877,#31878,#31879,
#31880,#31881,#31882,#31883,#31884,#31885,#31886,#31887,#31888,#31889,#31890,
#31891,#31892,#31893,#31894,#31895,#31896,#31897,#31898,#31899,#31900,#31901,
#31902,#31903,#31904,#31905,#31906,#31907,#31908,#31909,#31910,#31911,#31912,
#31913,#31914,#31915,#31916,#31917,#31918,#31919,#31920,#31921,#31922,#31923,
#31924,#31925,#31926,#31927,#31928,#31929,#31930,#31931,#31932,#31933,#31934,
#31935,#31936,#31937,#31938,#31939,#31940,#31941,#31942),(#31943,#31944,
#31945,#31946,#31947,#31948,#31949,#31950,#31951,#31952,#31953,#31954,#31955,
#31956,#31957,#31958,#31959,#31960,#31961,#31962,#31963,#31964,#31965,#31966,
#31967,#31968,#31969,#31970,#31971,#31972,#31973,#31974,#31975,#31976,#31977,
#31978,#31979,#31980,#31981,#31982,#31983,#31984,#31985,#31986,#31987,#31988,
#31989,#31990,#31991,#31992,#31993,#31994,#31995,#31996,#31997,#31998,#31999,
#32000,#32001,#32002,#32003,#32004,#32005,#32006,#32007,#32008,#32009,#32010,
#32011,#32012,#32013,#32014,#32015,#32016,#32017,#32018,#32019,#32020,#32021,
#32022,#32023,#32024,#32025,#32026,#32027,#32028,#32029,#32030,#32031,#32032,
#32033,#32034,#32035,#32036,#32037,#32038,#32039,#32040,#32041,#32042,#32043,
#32044,#32045,#32046,#32047,#32048,#32049,#32050,#32051,#32052,#32053,#32054,
#32055,#32056,#32057,#32058,#32059,#32060,#32061,#32062,#32063,#32064,#32065,
#32066,#32067,#32068,#32069,#32070,#32071,#32072,#32073,#32074,#32075,#32076,
#32077,#32078,#32079,#32080,#32081,#32082,#32083,#32084,#32085,#32086,#32087,
#32088,#32089,#32090,#32091,#32092,#32093,#32094,#32095,#32096,#32097,#32098,
#32099,#32100,#32101,#32102,#32103),(#32104,#32105,#32106,#32107,#32108,
#32109,#32110,#32111,#32112,#32113,#32114,#32115,#32116,#32117,#32118,#32119,
#32120,#32121,#32122,#32123,#32124,#32125,#32126,#32127,#32128,#32129,#32130,
#32131,#32132,#32133,#32134,#32135,#32136,#32137,#32138,#32139,#32140,#32141,
#32142,#32143,#32144,#32145,#32146,#32147,#32148,#32149,#32150,#32151,#32152,
#32153,#32154,#32155,#32156,#32157,#32158,#32159,#32160,#32161,#32162,#32163,
#32164,#32165,#32166,#32167,#32168,#32169,#32170,#32171,#32172,#32173,#32174,
#32175,#32176,#32177,#32178,#32179,#32180,#32181,#32182,#32183,#32184,#32185,
#32186,#32187,#32188,#32189,#32190,#32191,#32192,#32193,#32194,#32195,#32196,
#32197,#32198,#32199,#32200,#32201,#32202,#32203,#32204,#32205,#32206,#32207,
#32208,#32209,#32210,#32211,#32212,#32213,#32214,#32215,#32216,#32217,#32218,
#32219,#32220,#32221,#32222,#32223,#32224,#32225,#32226,#32227,#32228,#32229,
#32230,#32231,#32232,#32233,#32234,#32235,#32236,#32237,#32238,#32239,#32240,
#32241,#32242,#32243,#32244,#32245,#32246,#32247,#32248,#32249,#32250,#32251,
#32252,#32253,#32254,#32255,#32256,#32257,#32258,#32259,#32260,#32261,#32262,
#32263,#32264)),.UNSPECIFIED.,.F.,.F.,.F.)
B_SPLINE_SURFACE_WITH_KNOTS((4,4),(3,2,2,2,2,2,2,2,2,2,2,2,2,2,2,2,2,2,
2,2,2,2,2,2,2,2,2,2,2,2,2,2,2,2,2,2,2,2,2,2,2,2,2,2,2,2,2,2,2,2,2,2,2,2,
2,2,2,2,2,2,2,2,2,2,2,2,2,2,2,2,2,2,2,2,2,2,2,2,2,2,3),(0.,1.),(0.,0.0125,
0.025,0.0375,0.05,0.0625,0.075,0.0875,0.1,0.1125,0.125,0.1375,0.15,0.1625,
0.175,0.1875,0.2,0.2125,0.225,0.2375,0.25,0.2625,0.275,0.2875,0.3,0.3125,
0.325,0.3375,0.35,0.3625,0.375,0.3875,0.4,0.4125,0.425,0.4375,0.45,0.4625,
0.475,0.4875,0.5,0.5125,0.525,0.5375,0.55,0.5625,0.575,0.5875,0.6,0.6125,
0.625,0.6375,0.65,0.6625,0.675,0.6875,0.7,0.7125,0.725,0.7375,0.75,0.7625,
0.775,0.7875,0.8,0.8125,0.825,0.8375,0.85,0.8625,0.875,0.8875,0.9,0.9125,
0.925,0.9375,0.95,0.9625,0.975,0.9875,1.),.UNSPECIFIED.)
GEOMETRIC_REPRESENTATION_ITEM()
RATIONAL_B_SPLINE_SURFACE(((1.,0.923879532511287,1.,0.923879532511287,1.,
0.923879532511287,1.,0.923879532511287,1.,0.923879532511287,1.,0.923879532511287,
1.,0.923879532511287,1.,0.923879532511287,1.,0.923879532511287,1.,0.923879532511287,
1.,0.923879532511287,1.,0.923879532511287,1.,0.923879532511287,1.,0.923879532511287,
1.,0.923879532511287,1.,0.923879532511287,1.,0.923879532511287,1.,0.923879532511287,
1.,0.923879532511287,1.,0.923879532511287,1.,0.923879532511287,1.,0.923879532511287,
1.,0.923879532511287,1.,0.923879532511287,1.,0.923879532511287,1.,0.923879532511287,
1.,0.923879532511287,1.,0.923879532511287,1.,0.923879532511287,1.,0.923879532511287,
1.,0.923879532511287,1.,0.923879532511287,1.,0.923879532511287,1.,0.923879532511287,
1.,0.923879532511287,1.,0.923879532511287,1.,0.923879532511287,1.,0.923879532511287,
1.,0.923879532511287,1.,0.923879532511287,1.,0.923879532511287,1.,0.923879532511287,
1.,0.923879532511287,1.,0.923879532511287,1.,0.923879532511287,1.,0.923879532511287,
1.,0.923879532511287,1.,0.923879532511287,1.,0.923879532511287,1.,0.923879532511287,
1.,0.923879532511287,1.,0.923879532511287,1.,0.923879532511287,1.,0.923879532511287,
1.,0.923879532511287,1.,0.923879532511287,1.,0.923879532511287,1.,0.923879532511287,
1.,0.923879532511287,1.,0.923879532511287,1.,0.923879532511287,1.,0.923879532511287,
1.,0.923879532511287,1.,0.923879532511287,1.,0.923879532511287,1.,0.923879532511287,
1.,0.923879532511287,1.,0.923879532511287,1.,0.923879532511287,1.,0.923879532511287,
1.,0.923879532511287,1.,0.923879532511287,1.,0.923879532511287,1.,0.923879532511287,
1.,0.923879532511287,1.,0.923879532511287,1.,0.923879532511287,1.,0.923879532511287,
1.,0.923879532511287,1.,0.923879532511287,1.),(0.998696642611305,0.922675387296324,
0.998696642611305,0.922675387296324,0.998696642611305,0.922675387296324,
0.998696642611305,0.922675387296324,0.998696642611305,0.922675387296324,
0.998696642611305,0.922675387296324,0.998696642611305,0.922675387296324,
0.998696642611305,0.922675387296324,0.998696642611305,0.922675387296324,
0.998696642611305,0.922675387296324,0.998696642611305,0.922675387296324,
0.998696642611305,0.922675387296324,0.998696642611305,0.922675387296324,
0.998696642611305,0.922675387296324,0.998696642611305,0.922675387296324,
0.998696642611305,0.922675387296324,0.998696642611305,0.922675387296324,
0.998696642611305,0.922675387296324,0.998696642611305,0.922675387296324,
0.998696642611305,0.922675387296324,0.998696642611305,0.922675387296324,
0.998696642611305,0.922675387296324,0.998696642611305,0.922675387296324,
0.998696642611305,0.922675387296324,0.998696642611305,0.922675387296324,
0.998696642611305,0.922675387296324,0.998696642611305,0.922675387296324,
0.998696642611305,0.922675387296324,0.998696642611305,0.922675387296324,
0.998696642611305,0.922675387296324,0.998696642611305,0.922675387296324,
0.998696642611305,0.922675387296324,0.998696642611305,0.922675387296324,
0.998696642611305,0.922675387296324,0.998696642611305,0.922675387296324,
0.998696642611305,0.922675387296324,0.998696642611305,0.922675387296324,
0.998696642611305,0.922675387296324,0.998696642611305,0.922675387296324,
0.998696642611305,0.922675387296324,0.998696642611305,0.922675387296324,
0.998696642611305,0.922675387296324,0.998696642611305,0.922675387296324,
0.998696642611305,0.922675387296324,0.998696642611305,0.922675387296324,
0.998696642611305,0.922675387296324,0.998696642611305,0.922675387296324,
0.998696642611305,0.922675387296324,0.998696642611305,0.922675387296324,
0.998696642611305,0.922675387296324,0.998696642611305,0.922675387296324,
0.998696642611305,0.922675387296324,0.998696642611305,0.922675387296324,
0.998696642611305,0.922675387296324,0.998696642611305,0.922675387296324,
0.998696642611305,0.922675387296324,0.998696642611305,0.922675387296324,
0.998696642611305,0.922675387296324,0.998696642611305,0.922675387296324,
0.998696642611305,0.922675387296324,0.998696642611305,0.922675387296324,
0.998696642611305,0.922675387296324,0.998696642611305,0.922675387296324,
0.998696642611305,0.922675387296324,0.998696642611305,0.922675387296324,
0.998696642611305,0.922675387296324,0.998696642611305,0.922675387296324,
0.998696642611305,0.922675387296324,0.998696642611305,0.922675387296324,
0.998696642611305,0.922675387296324,0.998696642611305,0.922675387296324,
0.998696642611305,0.922675387296324,0.998696642611305,0.922675387296324,
0.998696642611305,0.922675387296324,0.998696642611305,0.922675387296324,
0.998696642611305,0.922675387296324,0.998696642611305,0.922675387296324,
0.998696642611305,0.922675387296324,0.998696642611305,0.922675387296324,
0.998696642611305,0.922675387296324,0.998696642611305),(0.998696642611305,
0.922675387296324,0.998696642611305,0.922675387296324,0.998696642611305,
0.922675387296324,0.998696642611305,0.922675387296324,0.998696642611305,
0.922675387296324,0.998696642611305,0.922675387296324,0.998696642611305,
0.922675387296324,0.998696642611305,0.922675387296324,0.998696642611305,
0.922675387296324,0.998696642611305,0.922675387296324,0.998696642611305,
0.922675387296324,0.998696642611305,0.922675387296324,0.998696642611305,
0.922675387296324,0.998696642611305,0.922675387296324,0.998696642611305,
0.922675387296324,0.998696642611305,0.922675387296324,0.998696642611305,
0.922675387296324,0.998696642611305,0.922675387296324,0.998696642611305,
0.922675387296324,0.998696642611305,0.922675387296324,0.998696642611305,
0.922675387296324,0.998696642611305,0.922675387296324,0.998696642611305,
0.922675387296324,0.998696642611305,0.922675387296324,0.998696642611305,
0.922675387296324,0.998696642611305,0.922675387296324,0.998696642611305,
0.922675387296324,0.998696642611305,0.922675387296324,0.998696642611305,
0.922675387296324,0.998696642611305,0.922675387296324,0.998696642611305,
0.922675387296324,0.998696642611305,0.922675387296324,0.998696642611305,
0.922675387296324,0.998696642611305,0.922675387296324,0.998696642611305,
0.922675387296324,0.998696642611305,0.922675387296324,0.998696642611305,
0.922675387296324,0.998696642611305,0.922675387296324,0.998696642611305,
0.922675387296324,0.998696642611305,0.922675387296324,0.998696642611305,
0.922675387296324,0.998696642611305,0.922675387296324,0.998696642611305,
0.922675387296324,0.998696642611305,0.922675387296324,0.998696642611305,
0.922675387296324,0.998696642611305,0.922675387296324,0.998696642611305,
0.922675387296324,0.998696642611305,0.922675387296324,0.998696642611305,
0.922675387296324,0.998696642611305,0.922675387296324,0.998696642611305,
0.922675387296324,0.998696642611305,0.922675387296324,0.998696642611305,
0.922675387296324,0.998696642611305,0.922675387296324,0.998696642611305,
0.922675387296324,0.998696642611305,0.922675387296324,0.998696642611305,
0.922675387296324,0.998696642611305,0.922675387296324,0.998696642611305,
0.922675387296324,0.998696642611305,0.922675387296324,0.998696642611305,
0.922675387296324,0.998696642611305,0.922675387296324,0.998696642611305,
0.922675387296324,0.998696642611305,0.922675387296324,0.998696642611305,
0.922675387296324,0.998696642611305,0.922675387296324,0.998696642611305,
0.922675387296324,0.998696642611305,0.922675387296324,0.998696642611305,
0.922675387296324,0.998696642611305,0.922675387296324,0.998696642611305,
0.922675387296324,0.998696642611305,0.922675387296324,0.998696642611305,
0.922675387296324,0.998696642611305,0.922675387296324,0.998696642611305,
0.922675387296324,0.998696642611305,0.922675387296324,0.998696642611305,
0.922675387296324,0.998696642611305,0.922675387296324,0.998696642611305,
0.922675387296324,0.998696642611305,0.922675387296324,0.998696642611305),
(1.,0.923879532511287,1.,0.923879532511287,1.,0.923879532511287,1.,0.923879532511287,
1.,0.923879532511287,1.,0.923879532511287,1.,0.923879532511287,1.,0.923879532511287,
1.,0.923879532511287,1.,0.923879532511287,1.,0.923879532511287,1.,0.923879532511287,
1.,0.923879532511287,1.,0.923879532511287,1.,0.923879532511287,1.,0.923879532511287,
1.,0.923879532511287,1.,0.923879532511287,1.,0.923879532511287,1.,0.923879532511287,
1.,0.923879532511287,1.,0.923879532511287,1.,0.923879532511287,1.,0.923879532511287,
1.,0.923879532511287,1.,0.923879532511287,1.,0.923879532511287,1.,0.923879532511287,
1.,0.923879532511287,1.,0.923879532511287,1.,0.923879532511287,1.,0.923879532511287,
1.,0.923879532511287,1.,0.923879532511287,1.,0.923879532511287,1.,0.923879532511287,
1.,0.923879532511287,1.,0.923879532511287,1.,0.923879532511287,1.,0.923879532511287,
1.,0.923879532511287,1.,0.923879532511287,1.,0.923879532511287,1.,0.923879532511287,
1.,0.923879532511287,1.,0.923879532511287,1.,0.923879532511287,1.,0.923879532511287,
1.,0.923879532511287,1.,0.923879532511287,1.,0.923879532511287,1.,0.923879532511287,
1.,0.923879532511287,1.,0.923879532511287,1.,0.923879532511287,1.,0.923879532511287,
1.,0.923879532511287,1.,0.923879532511287,1.,0.923879532511287,1.,0.923879532511287,
1.,0.923879532511287,1.,0.923879532511287,1.,0.923879532511287,1.,0.923879532511287,
1.,0.923879532511287,1.,0.923879532511287,1.,0.923879532511287,1.,0.923879532511287,
1.,0.923879532511287,1.,0.923879532511287,1.,0.923879532511287,1.,0.923879532511287,
1.,0.923879532511287,1.,0.923879532511287,1.,0.923879532511287,1.,0.923879532511287,
1.,0.923879532511287,1.,0.923879532511287,1.,0.923879532511287,1.,0.923879532511287,
1.)))
REPRESENTATION_ITEM('')
SURFACE()
);
#583=(
BOUNDED_SURFACE()
B_SPLINE_SURFACE(3,2,((#32268,#32269,#32270),(#32271,#32272,#32273),(#32274,
#32275,#32276),(#32277,#32278,#32279)),.UNSPECIFIED.,.F.,.F.,.F.)
B_SPLINE_SURFACE_WITH_KNOTS((4,4),(3,3),(-8.67361737988404E-18,0.00176076821392877),
(0.,1.),.UNSPECIFIED.)
GEOMETRIC_REPRESENTATION_ITEM()
RATIONAL_B_SPLINE_SURFACE(((1.,0.605017435075385,1.),(1.,0.607455453482648,
1.),(1.,0.609590739470685,1.),(1.,0.611227253379469,1.)))
REPRESENTATION_ITEM('')
SURFACE()
);
#584=(
BOUNDED_SURFACE()
B_SPLINE_SURFACE(3,2,((#32281,#32282,#32283),(#32284,#32285,#32286),(#32287,
#32288,#32289),(#32290,#32291,#32292),(#32293,#32294,#32295),(#32296,#32297,
#32298)),.UNSPECIFIED.,.F.,.F.,.F.)
B_SPLINE_SURFACE_WITH_KNOTS((4,2,4),(3,3),(3.35018471298021E-17,0.000541903658604953,
0.00108380731720987),(0.,1.),.UNSPECIFIED.)
GEOMETRIC_REPRESENTATION_ITEM()
RATIONAL_B_SPLINE_SURFACE(((1.,0.707106781186545,1.),(1.,0.687098191636224,
1.),(1.,0.66678877037223,1.),(1.,0.631310893346957,1.),(1.,0.615653630066085,
1.),(1.,0.605017435075385,1.)))
REPRESENTATION_ITEM('')
SURFACE()
);
#585=(
BOUNDED_SURFACE()
B_SPLINE_SURFACE(3,2,((#32311,#32312,#32313),(#32314,#32315,#32316),(#32317,
#32318,#32319),(#32320,#32321,#32322),(#32323,#32324,#32325),(#32326,#32327,
#32328)),.UNSPECIFIED.,.F.,.F.,.F.)
B_SPLINE_SURFACE_WITH_KNOTS((4,2,4),(3,3),(-2.0870891820346E-17,0.000541486237413509,
0.00108297247482704),(0.,1.),.UNSPECIFIED.)
GEOMETRIC_REPRESENTATION_ITEM()
RATIONAL_B_SPLINE_SURFACE(((1.,0.605017435075385,1.),(1.,0.615653519651203,
1.),(1.,0.631258339490859,1.),(1.,0.666776937440384,1.),(1.,0.687023379357965,
1.),(1.,0.707106781186545,1.)))
REPRESENTATION_ITEM('')
SURFACE()
);
#586=(
BOUNDED_SURFACE()
B_SPLINE_SURFACE(3,2,((#32330,#32331,#32332),(#32333,#32334,#32335),(#32336,
#32337,#32338),(#32339,#32340,#32341)),.UNSPECIFIED.,.F.,.F.,.F.)
B_SPLINE_SURFACE_WITH_KNOTS((4,4),(3,3),(1.47451495458029E-17,0.00176076821392879),
(0.,1.),.UNSPECIFIED.)
GEOMETRIC_REPRESENTATION_ITEM()
RATIONAL_B_SPLINE_SURFACE(((1.,0.605017435075385,1.),(1.,0.607455453482656,
1.),(1.,0.609590739470667,1.),(1.,0.611227253379484,1.)))
REPRESENTATION_ITEM('')
SURFACE()
);
#610=TOROIDAL_SURFACE('',#9128,39.,0.5);
#611=TOROIDAL_SURFACE('',#9132,39.,0.5);
#612=TOROIDAL_SURFACE('',#9136,6.15470053837925,0.5);
#613=TOROIDAL_SURFACE('',#9140,6.15470053837925,0.5);
#614=TOROIDAL_SURFACE('',#9282,11.1547005383793,0.5);
#615=TOROIDAL_SURFACE('',#9286,11.1547005383793,0.5);
#616=TOROIDAL_SURFACE('',#9298,15.5,0.5);
#617=TOROIDAL_SURFACE('',#9302,14.5,0.5);
#618=TOROIDAL_SURFACE('',#9305,15.5,0.5);
#619=TOROIDAL_SURFACE('',#9309,14.5,0.5);
#620=TOROIDAL_SURFACE('',#9319,14.5,0.5);
#621=TOROIDAL_SURFACE('',#9323,15.5,0.5);
#622=TOROIDAL_SURFACE('',#9333,12.2,0.5);
#623=TOROIDAL_SURFACE('',#9335,9.5,0.5);
#624=TOROIDAL_SURFACE('',#9337,4.5,0.5);
#625=TOROIDAL_SURFACE('',#9338,4.5,0.5);
#626=TOROIDAL_SURFACE('',#9340,9.5,0.5);
#627=TOROIDAL_SURFACE('',#9342,12.2,0.5);
#677=SHAPE_REPRESENTATION_RELATIONSHIP('SRR','None',#47764,#689);
#689=ADVANCED_BREP_SHAPE_REPRESENTATION('',(#713),#47708);
#701=STYLED_ITEM('',(#47830),#713);
#713=MANIFOLD_SOLID_BREP('Body1',#8928);
#726=FACE_BOUND('',#2631,.T.);
#727=FACE_BOUND('',#2665,.T.);
#728=FACE_BOUND('',#2667,.T.);
#729=FACE_BOUND('',#2673,.T.);
#765=PLANE('',#9173);
#766=PLANE('',#9193);
#767=PLANE('',#9194);
#768=PLANE('',#9198);
#769=PLANE('',#9201);
#770=PLANE('',#9202);
#771=PLANE('',#9203);
#772=PLANE('',#9214);
#773=PLANE('',#9215);
#774=PLANE('',#9216);
#775=PLANE('',#9219);
#776=PLANE('',#9225);
#777=PLANE('',#9237);
#778=PLANE('',#9238);
#779=PLANE('',#9243);
#780=PLANE('',#9244);
#781=PLANE('',#9250);
#782=PLANE('',#9252);
#783=PLANE('',#9253);
#784=PLANE('',#9254);
#785=PLANE('',#9260);
#786=PLANE('',#9261);
#787=PLANE('',#9262);
#788=PLANE('',#9263);
#789=PLANE('',#9264);
#790=PLANE('',#9265);
#791=PLANE('',#9266);
#792=PLANE('',#9267);
#793=PLANE('',#9268);
#794=PLANE('',#9269);
#795=PLANE('',#9270);
#796=PLANE('',#9271);
#797=PLANE('',#9272);
#798=PLANE('',#9273);
#799=PLANE('',#9274);
#800=PLANE('',#9275);
#801=PLANE('',#9276);
#802=PLANE('',#9277);
#803=PLANE('',#9278);
#804=PLANE('',#9291);
#805=PLANE('',#9294);
#806=PLANE('',#9295);
#807=PLANE('',#9327);
#887=LINE('',#15695,#1374);
#888=LINE('',#15699,#1375);
#889=LINE('',#15703,#1376);
#890=LINE('',#15719,#1377);
#891=LINE('',#15862,#1378);
#892=LINE('',#15868,#1379);
#893=LINE('',#15883,#1380);
#894=LINE('',#15886,#1381);
#895=LINE('',#15892,#1382);
#896=LINE('',#15905,#1383);
#897=LINE('',#15922,#1384);
#898=LINE('',#15937,#1385);
#899=LINE('',#15941,#1386);
#900=LINE('',#16174,#1387);
#901=LINE('',#16178,#1388);
#902=LINE('',#16210,#1389);
#903=LINE('',#16245,#1390);
#904=LINE('',#16277,#1391);
#905=LINE('',#16312,#1392);
#906=LINE('',#16334,#1393);
#907=LINE('',#16349,#1394);
#908=LINE('',#16361,#1395);
#909=LINE('',#16376,#1396);
#910=LINE('',#16388,#1397);
#911=LINE('',#16403,#1398);
#912=LINE('',#16415,#1399);
#913=LINE('',#16430,#1400);
#914=LINE('',#16442,#1401);
#915=LINE('',#16457,#1402);
#916=LINE('',#16469,#1403);
#917=LINE('',#16484,#1404);
#918=LINE('',#16496,#1405);
#919=LINE('',#16511,#1406);
#920=LINE('',#16523,#1407);
#921=LINE('',#17082,#1408);
#922=LINE('',#17084,#1409);
#923=LINE('',#17102,#1410);
#924=LINE('',#17120,#1411);
#925=LINE('',#17138,#1412);
#926=LINE('',#17156,#1413);
#927=LINE('',#17174,#1414);
#928=LINE('',#17192,#1415);
#929=LINE('',#17208,#1416);
#930=LINE('',#17210,#1417);
#931=LINE('',#17214,#1418);
#932=LINE('',#17217,#1419);
#933=LINE('',#17288,#1420);
#934=LINE('',#17585,#1421);
#935=LINE('',#17630,#1422);
#936=LINE('',#17677,#1423);
#937=LINE('',#17724,#1424);
#938=LINE('',#17773,#1425);
#939=LINE('',#17824,#1426);
#940=LINE('',#18047,#1427);
#941=LINE('',#18336,#1428);
#942=LINE('',#18342,#1429);
#943=LINE('',#18377,#1430);
#944=LINE('',#18379,#1431);
#945=LINE('',#18381,#1432);
#946=LINE('',#18384,#1433);
#947=LINE('',#18423,#1434);
#948=LINE('',#18426,#1435);
#949=LINE('',#18428,#1436);
#950=LINE('',#18429,#1437);
#951=LINE('',#18433,#1438);
#952=LINE('',#18435,#1439);
#953=LINE('',#18437,#1440);
#954=LINE('',#18438,#1441);
#955=LINE('',#18461,#1442);
#956=LINE('',#18465,#1443);
#957=LINE('',#18469,#1444);
#958=LINE('',#18473,#1445);
#959=LINE('',#18477,#1446);
#960=LINE('',#18502,#1447);
#961=LINE('',#18507,#1448);
#962=LINE('',#18511,#1449);
#963=LINE('',#18549,#1450);
#964=LINE('',#18579,#1451);
#965=LINE('',#18580,#1452);
#966=LINE('',#18582,#1453);
#967=LINE('',#18583,#1454);
#968=LINE('',#18672,#1455);
#969=LINE('',#18676,#1456);
#970=LINE('',#18679,#1457);
#971=LINE('',#18682,#1458);
#972=LINE('',#18686,#1459);
#973=LINE('',#18690,#1460);
#974=LINE('',#19155,#1461);
#975=LINE('',#19161,#1462);
#976=LINE('',#19162,#1463);
#977=LINE('',#19269,#1464);
#978=LINE('',#19270,#1465);
#979=LINE('',#19339,#1466);
#980=LINE('',#19343,#1467);
#981=LINE('',#19447,#1468);
#982=LINE('',#19462,#1469);
#983=LINE('',#19463,#1470);
#984=LINE('',#19467,#1471);
#985=LINE('',#19468,#1472);
#986=LINE('',#19469,#1473);
#987=LINE('',#19529,#1474);
#988=LINE('',#19589,#1475);
#989=LINE('',#19606,#1476);
#990=LINE('',#19616,#1477);
#991=LINE('',#19618,#1478);
#992=LINE('',#19620,#1479);
#993=LINE('',#19622,#1480);
#994=LINE('',#19624,#1481);
#995=LINE('',#19626,#1482);
#996=LINE('',#19628,#1483);
#997=LINE('',#19630,#1484);
#998=LINE('',#19632,#1485);
#999=LINE('',#19634,#1486);
#1000=LINE('',#19636,#1487);
#1001=LINE('',#19638,#1488);
#1002=LINE('',#19640,#1489);
#1003=LINE('',#19642,#1490);
#1004=LINE('',#19644,#1491);
#1005=LINE('',#19646,#1492);
#1006=LINE('',#19648,#1493);
#1007=LINE('',#19650,#1494);
#1008=LINE('',#19651,#1495);
#1009=LINE('',#19654,#1496);
#1010=LINE('',#19655,#1497);
#1011=LINE('',#19659,#1498);
#1012=LINE('',#19660,#1499);
#1013=LINE('',#19661,#1500);
#1014=LINE('',#19678,#1501);
#1015=LINE('',#19680,#1502);
#1016=LINE('',#19682,#1503);
#1017=LINE('',#19684,#1504);
#1018=LINE('',#19686,#1505);
#1019=LINE('',#19688,#1506);
#1020=LINE('',#19690,#1507);
#1021=LINE('',#19692,#1508);
#1022=LINE('',#19694,#1509);
#1023=LINE('',#19696,#1510);
#1024=LINE('',#19698,#1511);
#1025=LINE('',#19700,#1512);
#1026=LINE('',#19702,#1513);
#1027=LINE('',#19704,#1514);
#1028=LINE('',#19706,#1515);
#1029=LINE('',#19708,#1516);
#1030=LINE('',#19710,#1517);
#1031=LINE('',#19712,#1518);
#1032=LINE('',#19713,#1519);
#1033=LINE('',#19749,#1520);
#1034=LINE('',#19751,#1521);
#1035=LINE('',#19753,#1522);
#1036=LINE('',#19755,#1523);
#1037=LINE('',#19757,#1524);
#1038=LINE('',#19759,#1525);
#1039=LINE('',#19761,#1526);
#1040=LINE('',#19763,#1527);
#1041=LINE('',#19765,#1528);
#1042=LINE('',#19767,#1529);
#1043=LINE('',#19769,#1530);
#1044=LINE('',#19771,#1531);
#1045=LINE('',#19773,#1532);
#1046=LINE('',#19775,#1533);
#1047=LINE('',#19777,#1534);
#1048=LINE('',#19779,#1535);
#1049=LINE('',#19781,#1536);
#1050=LINE('',#19783,#1537);
#1374=VECTOR('',#10070,1000.);
#1375=VECTOR('',#10073,1000.);
#1376=VECTOR('',#10076,1000.);
#1377=VECTOR('',#10079,1000.);
#1378=VECTOR('',#10124,2.);
#1379=VECTOR('',#10131,2.);
#1380=VECTOR('',#10138,1000.);
#1381=VECTOR('',#10141,1000.);
#1382=VECTOR('',#10146,1000.);
#1383=VECTOR('',#10149,1000.);
#1384=VECTOR('',#10152,1000.);
#1385=VECTOR('',#10153,1000.);
#1386=VECTOR('',#10156,1000.);
#1387=VECTOR('',#10157,1000.);
#1388=VECTOR('',#10160,1000.);
#1389=VECTOR('',#10161,1000.);
#1390=VECTOR('',#10164,1000.);
#1391=VECTOR('',#10165,1000.);
#1392=VECTOR('',#10168,1000.);
#1393=VECTOR('',#10171,1000.);
#1394=VECTOR('',#10174,1000.);
#1395=VECTOR('',#10175,10.);
#1396=VECTOR('',#10178,1000.);
#1397=VECTOR('',#10179,10.);
#1398=VECTOR('',#10182,1000.);
#1399=VECTOR('',#10183,10.);
#1400=VECTOR('',#10186,1000.);
#1401=VECTOR('',#10187,10.);
#1402=VECTOR('',#10190,1000.);
#1403=VECTOR('',#10191,10.);
#1404=VECTOR('',#10194,1000.);
#1405=VECTOR('',#10195,10.);
#1406=VECTOR('',#10198,1000.);
#1407=VECTOR('',#10199,10.);
#1408=VECTOR('',#10204,1000.);
#1409=VECTOR('',#10205,1000.);
#1410=VECTOR('',#10208,1000.);
#1411=VECTOR('',#10211,1000.);
#1412=VECTOR('',#10214,1000.);
#1413=VECTOR('',#10217,1000.);
#1414=VECTOR('',#10220,1000.);
#1415=VECTOR('',#10223,1000.);
#1416=VECTOR('',#10224,1000.);
#1417=VECTOR('',#10225,1000.);
#1418=VECTOR('',#10228,1000.);
#1419=VECTOR('',#10231,1000.);
#1420=VECTOR('',#10232,1000.);
#1421=VECTOR('',#10237,10.);
#1422=VECTOR('',#10238,10.);
#1423=VECTOR('',#10239,10.);
#1424=VECTOR('',#10240,10.);
#1425=VECTOR('',#10241,10.);
#1426=VECTOR('',#10242,10.);
#1427=VECTOR('',#10261,1000.);
#1428=VECTOR('',#10264,1000.);
#1429=VECTOR('',#10271,1000.);
#1430=VECTOR('',#10274,1000.);
#1431=VECTOR('',#10277,1000.);
#1432=VECTOR('',#10278,1000.);
#1433=VECTOR('',#10281,1000.);
#1434=VECTOR('',#10282,1000.);
#1435=VECTOR('',#10285,1000.);
#1436=VECTOR('',#10286,1000.);
#1437=VECTOR('',#10287,1000.);
#1438=VECTOR('',#10290,1000.);
#1439=VECTOR('',#10291,1000.);
#1440=VECTOR('',#10292,1000.);
#1441=VECTOR('',#10293,1000.);
#1442=VECTOR('',#10296,1000.);
#1443=VECTOR('',#10299,1000.);
#1444=VECTOR('',#10302,1000.);
#1445=VECTOR('',#10305,1000.);
#1446=VECTOR('',#10308,1000.);
#1447=VECTOR('',#10313,1000.);
#1448=VECTOR('',#10318,1000.);
#1449=VECTOR('',#10321,1000.);
#1450=VECTOR('',#10324,1000.);
#1451=VECTOR('',#10327,1000.);
#1452=VECTOR('',#10328,1000.);
#1453=VECTOR('',#10331,1000.);
#1454=VECTOR('',#10332,1000.);
#1455=VECTOR('',#10335,1000.);
#1456=VECTOR('',#10338,1000.);
#1457=VECTOR('',#10341,1000.);
#1458=VECTOR('',#10344,1000.);
#1459=VECTOR('',#10347,1000.);
#1460=VECTOR('',#10350,1000.);
#1461=VECTOR('',#10357,10.);
#1462=VECTOR('',#10366,1000.);
#1463=VECTOR('',#10367,1000.);
#1464=VECTOR('',#10382,1000.);
#1465=VECTOR('',#10383,1000.);
#1466=VECTOR('',#10396,1000.);
#1467=VECTOR('',#10399,1000.);
#1468=VECTOR('',#10402,1000.);
#1469=VECTOR('',#10403,1000.);
#1470=VECTOR('',#10404,1000.);
#1471=VECTOR('',#10407,1000.);
#1472=VECTOR('',#10408,1000.);
#1473=VECTOR('',#10409,1000.);
#1474=VECTOR('',#10416,1000.);
#1475=VECTOR('',#10421,1000.);
#1476=VECTOR('',#10424,1000.);
#1477=VECTOR('',#10427,1000.);
#1478=VECTOR('',#10428,1000.);
#1479=VECTOR('',#10429,1000.);
#1480=VECTOR('',#10430,1000.);
#1481=VECTOR('',#10431,1000.);
#1482=VECTOR('',#10432,1000.);
#1483=VECTOR('',#10433,1000.);
#1484=VECTOR('',#10434,1000.);
#1485=VECTOR('',#10435,1000.);
#1486=VECTOR('',#10436,1000.);
#1487=VECTOR('',#10437,1000.);
#1488=VECTOR('',#10438,1000.);
#1489=VECTOR('',#10439,1000.);
#1490=VECTOR('',#10440,1000.);
#1491=VECTOR('',#10441,1000.);
#1492=VECTOR('',#10442,1000.);
#1493=VECTOR('',#10443,1000.);
#1494=VECTOR('',#10444,1000.);
#1495=VECTOR('',#10445,1000.);
#1496=VECTOR('',#10448,1000.);
#1497=VECTOR('',#10449,1000.);
#1498=VECTOR('',#10452,1000.);
#1499=VECTOR('',#10453,1000.);
#1500=VECTOR('',#10454,1000.);
#1501=VECTOR('',#10457,1000.);
#1502=VECTOR('',#10458,1000.);
#1503=VECTOR('',#10459,1000.);
#1504=VECTOR('',#10460,1000.);
#1505=VECTOR('',#10461,1000.);
#1506=VECTOR('',#10462,1000.);
#1507=VECTOR('',#10463,1000.);
#1508=VECTOR('',#10464,1000.);
#1509=VECTOR('',#10465,1000.);
#1510=VECTOR('',#10466,1000.);
#1511=VECTOR('',#10467,1000.);
#1512=VECTOR('',#10468,1000.);
#1513=VECTOR('',#10469,1000.);
#1514=VECTOR('',#10470,1000.);
#1515=VECTOR('',#10471,1000.);
#1516=VECTOR('',#10472,1000.);
#1517=VECTOR('',#10473,1000.);
#1518=VECTOR('',#10474,1000.);
#1519=VECTOR('',#10475,1000.);
#1520=VECTOR('',#10488,1000.);
#1521=VECTOR('',#10491,1000.);
#1522=VECTOR('',#10494,1000.);
#1523=VECTOR('',#10497,1000.);
#1524=VECTOR('',#10500,1000.);
#1525=VECTOR('',#10503,1000.);
#1526=VECTOR('',#10506,1000.);
#1527=VECTOR('',#10509,1000.);
#1528=VECTOR('',#10512,1000.);
#1529=VECTOR('',#10515,1000.);
#1530=VECTOR('',#10518,1000.);
#1531=VECTOR('',#10521,1000.);
#1532=VECTOR('',#10524,1000.);
#1533=VECTOR('',#10527,1000.);
#1534=VECTOR('',#10530,1000.);
#1535=VECTOR('',#10533,1000.);
#1536=VECTOR('',#10536,1000.);
#1537=VECTOR('',#10539,1000.);
#1861=CYLINDRICAL_SURFACE('',#9123,5.);
#1862=CYLINDRICAL_SURFACE('',#9148,2.);
#1863=CYLINDRICAL_SURFACE('',#9151,2.);
#1864=CYLINDRICAL_SURFACE('',#9154,15.);
#1865=CYLINDRICAL_SURFACE('',#9157,15.);
#1866=CYLINDRICAL_SURFACE('',#9160,4.);
#1867=CYLINDRICAL_SURFACE('',#9163,4.);
#1868=CYLINDRICAL_SURFACE('',#9164,4.);
#1869=CYLINDRICAL_SURFACE('',#9166,3.);
#1870=CYLINDRICAL_SURFACE('',#9167,3.);
#1871=CYLINDRICAL_SURFACE('',#9168,3.);
#1872=CYLINDRICAL_SURFACE('',#9169,3.);
#1873=CYLINDRICAL_SURFACE('',#9170,3.);
#1874=CYLINDRICAL_SURFACE('',#9171,3.);
#1875=CYLINDRICAL_SURFACE('',#9172,3.);
#1876=CYLINDRICAL_SURFACE('',#9185,3.);
#1877=CYLINDRICAL_SURFACE('',#9186,3.);
#1878=CYLINDRICAL_SURFACE('',#9187,3.);
#1879=CYLINDRICAL_SURFACE('',#9188,3.);
#1880=CYLINDRICAL_SURFACE('',#9189,3.);
#1881=CYLINDRICAL_SURFACE('',#9190,3.);
#1882=CYLINDRICAL_SURFACE('',#9191,3.);
#1883=CYLINDRICAL_SURFACE('',#9211,15.);
#1884=CYLINDRICAL_SURFACE('',#9222,15.);
#1885=CYLINDRICAL_SURFACE('',#9236,1.49999773384112);
#1886=CYLINDRICAL_SURFACE('',#9242,39.5);
#1887=CYLINDRICAL_SURFACE('',#9245,11.7);
#1888=CYLINDRICAL_SURFACE('',#9279,0.5);
#1889=CYLINDRICAL_SURFACE('',#9283,0.5);
#1890=CYLINDRICAL_SURFACE('',#9292,4.);
#1891=CYLINDRICAL_SURFACE('',#9296,0.5);
#1892=CYLINDRICAL_SURFACE('',#9300,0.500000000000003);
#1893=CYLINDRICAL_SURFACE('',#9303,0.5);
#1894=CYLINDRICAL_SURFACE('',#9307,0.500000000000003);
#1895=CYLINDRICAL_SURFACE('',#9311,0.5);
#1896=CYLINDRICAL_SURFACE('',#9314,0.500000000000001);
#1897=CYLINDRICAL_SURFACE('',#9317,0.5);
#1898=CYLINDRICAL_SURFACE('',#9321,0.500000000000003);
#1899=CYLINDRICAL_SURFACE('',#9325,0.5);
#1900=CYLINDRICAL_SURFACE('',#9328,10.);
#2087=FACE_OUTER_BOUND('',#2603,.T.);
#2088=FACE_OUTER_BOUND('',#2604,.T.);
#2089=FACE_OUTER_BOUND('',#2605,.T.);
#2090=FACE_OUTER_BOUND('',#2606,.T.);
#2091=FACE_OUTER_BOUND('',#2607,.T.);
#2092=FACE_OUTER_BOUND('',#2608,.T.);
#2093=FACE_OUTER_BOUND('',#2609,.T.);
#2094=FACE_OUTER_BOUND('',#2610,.T.);
#2095=FACE_OUTER_BOUND('',#2611,.T.);
#2096=FACE_OUTER_BOUND('',#2612,.T.);
#2097=FACE_OUTER_BOUND('',#2613,.T.);
#2098=FACE_OUTER_BOUND('',#2614,.T.);
#2099=FACE_OUTER_BOUND('',#2615,.T.);
#2100=FACE_OUTER_BOUND('',#2616,.T.);
#2101=FACE_OUTER_BOUND('',#2617,.T.);
#2102=FACE_OUTER_BOUND('',#2618,.T.);
#2103=FACE_OUTER_BOUND('',#2619,.T.);
#2104=FACE_OUTER_BOUND('',#2620,.T.);
#2105=FACE_OUTER_BOUND('',#2621,.T.);
#2106=FACE_OUTER_BOUND('',#2622,.T.);
#2107=FACE_OUTER_BOUND('',#2623,.T.);
#2108=FACE_OUTER_BOUND('',#2624,.T.);
#2109=FACE_OUTER_BOUND('',#2625,.T.);
#2110=FACE_OUTER_BOUND('',#2626,.T.);
#2111=FACE_OUTER_BOUND('',#2627,.T.);
#2112=FACE_OUTER_BOUND('',#2628,.T.);
#2113=FACE_OUTER_BOUND('',#2629,.T.);
#2114=FACE_OUTER_BOUND('',#2630,.T.);
#2115=FACE_OUTER_BOUND('',#2632,.T.);
#2116=FACE_OUTER_BOUND('',#2633,.T.);
#2117=FACE_OUTER_BOUND('',#2634,.T.);
#2118=FACE_OUTER_BOUND('',#2635,.T.);
#2119=FACE_OUTER_BOUND('',#2636,.T.);
#2120=FACE_OUTER_BOUND('',#2637,.T.);
#2121=FACE_OUTER_BOUND('',#2638,.T.);
#2122=FACE_OUTER_BOUND('',#2639,.T.);
#2123=FACE_OUTER_BOUND('',#2640,.T.);
#2124=FACE_OUTER_BOUND('',#2641,.T.);
#2125=FACE_OUTER_BOUND('',#2642,.T.);
#2126=FACE_OUTER_BOUND('',#2643,.T.);
#2127=FACE_OUTER_BOUND('',#2644,.T.);
#2128=FACE_OUTER_BOUND('',#2645,.T.);
#2129=FACE_OUTER_BOUND('',#2646,.T.);
#2130=FACE_OUTER_BOUND('',#2647,.T.);
#2131=FACE_OUTER_BOUND('',#2648,.T.);
#2132=FACE_OUTER_BOUND('',#2649,.T.);
#2133=FACE_OUTER_BOUND('',#2650,.T.);
#2134=FACE_OUTER_BOUND('',#2651,.T.);
#2135=FACE_OUTER_BOUND('',#2652,.T.);
#2136=FACE_OUTER_BOUND('',#2653,.T.);
#2137=FACE_OUTER_BOUND('',#2654,.T.);
#2138=FACE_OUTER_BOUND('',#2655,.T.);
#2139=FACE_OUTER_BOUND('',#2656,.T.);
#2140=FACE_OUTER_BOUND('',#2657,.T.);
#2141=FACE_OUTER_BOUND('',#2658,.T.);
#2142=FACE_OUTER_BOUND('',#2659,.T.);
#2143=FACE_OUTER_BOUND('',#2660,.T.);
#2144=FACE_OUTER_BOUND('',#2661,.T.);
#2145=FACE_OUTER_BOUND('',#2662,.T.);
#2146=FACE_OUTER_BOUND('',#2663,.T.);
#2147=FACE_OUTER_BOUND('',#2664,.T.);
#2148=FACE_OUTER_BOUND('',#2666,.T.);
#2149=FACE_OUTER_BOUND('',#2668,.T.);
#2150=FACE_OUTER_BOUND('',#2669,.T.);
#2151=FACE_OUTER_BOUND('',#2670,.T.);
#2152=FACE_OUTER_BOUND('',#2671,.T.);
#2153=FACE_OUTER_BOUND('',#2672,.T.);
#2154=FACE_OUTER_BOUND('',#2674,.T.);
#2155=FACE_OUTER_BOUND('',#2675,.T.);
#2156=FACE_OUTER_BOUND('',#2676,.T.);
#2157=FACE_OUTER_BOUND('',#2677,.T.);
#2158=FACE_OUTER_BOUND('',#2678,.T.);
#2159=FACE_OUTER_BOUND('',#2679,.T.);
#2160=FACE_OUTER_BOUND('',#2680,.T.);
#2161=FACE_OUTER_BOUND('',#2681,.T.);
#2162=FACE_OUTER_BOUND('',#2682,.T.);
#2163=FACE_OUTER_BOUND('',#2683,.T.);
#2164=FACE_OUTER_BOUND('',#2684,.T.);
#2165=FACE_OUTER_BOUND('',#2685,.T.);
#2166=FACE_OUTER_BOUND('',#2686,.T.);
#2167=FACE_OUTER_BOUND('',#2687,.T.);
#2168=FACE_OUTER_BOUND('',#2688,.T.);
#2169=FACE_OUTER_BOUND('',#2689,.T.);
#2170=FACE_OUTER_BOUND('',#2690,.T.);
#2171=FACE_OUTER_BOUND('',#2691,.T.);
#2172=FACE_OUTER_BOUND('',#2692,.T.);
#2173=FACE_OUTER_BOUND('',#2693,.T.);
#2174=FACE_OUTER_BOUND('',#2694,.T.);
#2175=FACE_OUTER_BOUND('',#2695,.T.);
#2176=FACE_OUTER_BOUND('',#2696,.T.);
#2177=FACE_OUTER_BOUND('',#2697,.T.);
#2178=FACE_OUTER_BOUND('',#2698,.T.);
#2179=FACE_OUTER_BOUND('',#2699,.T.);
#2180=FACE_OUTER_BOUND('',#2700,.T.);
#2181=FACE_OUTER_BOUND('',#2701,.T.);
#2182=FACE_OUTER_BOUND('',#2702,.T.);
#2183=FACE_OUTER_BOUND('',#2703,.T.);
#2184=FACE_OUTER_BOUND('',#2704,.T.);
#2185=FACE_OUTER_BOUND('',#2705,.T.);
#2186=FACE_OUTER_BOUND('',#2706,.T.);
#2187=FACE_OUTER_BOUND('',#2707,.T.);
#2188=FACE_OUTER_BOUND('',#2708,.T.);
#2189=FACE_OUTER_BOUND('',#2709,.T.);
#2190=FACE_OUTER_BOUND('',#2710,.T.);
#2191=FACE_OUTER_BOUND('',#2711,.T.);
#2192=FACE_OUTER_BOUND('',#2712,.T.);
#2193=FACE_OUTER_BOUND('',#2713,.T.);
#2194=FACE_OUTER_BOUND('',#2714,.T.);
#2195=FACE_OUTER_BOUND('',#2715,.T.);
#2196=FACE_OUTER_BOUND('',#2716,.T.);
#2197=FACE_OUTER_BOUND('',#2717,.T.);
#2198=FACE_OUTER_BOUND('',#2718,.T.);
#2199=FACE_OUTER_BOUND('',#2719,.T.);
#2200=FACE_OUTER_BOUND('',#2720,.T.);
#2201=FACE_OUTER_BOUND('',#2721,.T.);
#2202=FACE_OUTER_BOUND('',#2722,.T.);
#2203=FACE_OUTER_BOUND('',#2723,.T.);
#2204=FACE_OUTER_BOUND('',#2724,.T.);
#2205=FACE_OUTER_BOUND('',#2725,.T.);
#2206=FACE_OUTER_BOUND('',#2726,.T.);
#2207=FACE_OUTER_BOUND('',#2727,.T.);
#2208=FACE_OUTER_BOUND('',#2728,.T.);
#2209=FACE_OUTER_BOUND('',#2729,.T.);
#2210=FACE_OUTER_BOUND('',#2730,.T.);
#2211=FACE_OUTER_BOUND('',#2731,.T.);
#2212=FACE_OUTER_BOUND('',#2732,.T.);
#2213=FACE_OUTER_BOUND('',#2733,.T.);
#2214=FACE_OUTER_BOUND('',#2734,.T.);
#2215=FACE_OUTER_BOUND('',#2735,.T.);
#2216=FACE_OUTER_BOUND('',#2736,.T.);
#2217=FACE_OUTER_BOUND('',#2737,.T.);
#2218=FACE_OUTER_BOUND('',#2738,.T.);
#2219=FACE_OUTER_BOUND('',#2739,.T.);
#2220=FACE_OUTER_BOUND('',#2740,.T.);
#2221=FACE_OUTER_BOUND('',#2741,.T.);
#2222=FACE_OUTER_BOUND('',#2742,.T.);
#2223=FACE_OUTER_BOUND('',#2743,.T.);
#2224=FACE_OUTER_BOUND('',#2744,.T.);
#2225=FACE_OUTER_BOUND('',#2745,.T.);
#2226=FACE_OUTER_BOUND('',#2746,.T.);
#2227=FACE_OUTER_BOUND('',#2747,.T.);
#2228=FACE_OUTER_BOUND('',#2748,.T.);
#2229=FACE_OUTER_BOUND('',#2749,.T.);
#2230=FACE_OUTER_BOUND('',#2750,.T.);
#2231=FACE_OUTER_BOUND('',#2751,.T.);
#2232=FACE_OUTER_BOUND('',#2752,.T.);
#2233=FACE_OUTER_BOUND('',#2753,.T.);
#2234=FACE_OUTER_BOUND('',#2754,.T.);
#2235=FACE_OUTER_BOUND('',#2755,.T.);
#2236=FACE_OUTER_BOUND('',#2756,.T.);
#2237=FACE_OUTER_BOUND('',#2757,.T.);
#2238=FACE_OUTER_BOUND('',#2758,.T.);
#2239=FACE_OUTER_BOUND('',#2759,.T.);
#2240=FACE_OUTER_BOUND('',#2760,.T.);
#2241=FACE_OUTER_BOUND('',#2761,.T.);
#2242=FACE_OUTER_BOUND('',#2762,.T.);
#2243=FACE_OUTER_BOUND('',#2763,.T.);
#2244=FACE_OUTER_BOUND('',#2764,.T.);
#2245=FACE_OUTER_BOUND('',#2765,.T.);
#2246=FACE_OUTER_BOUND('',#2766,.T.);
#2247=FACE_OUTER_BOUND('',#2767,.T.);
#2248=FACE_OUTER_BOUND('',#2768,.T.);
#2249=FACE_OUTER_BOUND('',#2769,.T.);
#2250=FACE_OUTER_BOUND('',#2770,.T.);
#2251=FACE_OUTER_BOUND('',#2771,.T.);
#2252=FACE_OUTER_BOUND('',#2772,.T.);
#2253=FACE_OUTER_BOUND('',#2773,.T.);
#2254=FACE_OUTER_BOUND('',#2774,.T.);
#2255=FACE_OUTER_BOUND('',#2775,.T.);
#2603=EDGE_LOOP('',(#5807,#5808,#5809,#5810,#5811,#5812,#5813,#5814,#5815));
#2604=EDGE_LOOP('',(#5816,#5817,#5818,#5819));
#2605=EDGE_LOOP('',(#5820,#5821,#5822,#5823));
#2606=EDGE_LOOP('',(#5824,#5825,#5826,#5827));
#2607=EDGE_LOOP('',(#5828,#5829,#5830,#5831));
#2608=EDGE_LOOP('',(#5832,#5833,#5834,#5835));
#2609=EDGE_LOOP('',(#5836,#5837,#5838,#5839));
#2610=EDGE_LOOP('',(#5840,#5841,#5842,#5843));
#2611=EDGE_LOOP('',(#5844,#5845,#5846,#5847));
#2612=EDGE_LOOP('',(#5848,#5849,#5850,#5851,#5852,#5853));
#2613=EDGE_LOOP('',(#5854,#5855,#5856,#5857,#5858,#5859));
#2614=EDGE_LOOP('',(#5860,#5861,#5862,#5863,#5864,#5865,#5866,#5867,#5868,
#5869,#5870,#5871,#5872,#5873));
#2615=EDGE_LOOP('',(#5874,#5875,#5876,#5877));
#2616=EDGE_LOOP('',(#5878,#5879,#5880,#5881,#5882));
#2617=EDGE_LOOP('',(#5883,#5884,#5885,#5886));
#2618=EDGE_LOOP('',(#5887,#5888,#5889,#5890));
#2619=EDGE_LOOP('',(#5891,#5892,#5893,#5894));
#2620=EDGE_LOOP('',(#5895,#5896,#5897,#5898));
#2621=EDGE_LOOP('',(#5899,#5900,#5901,#5902));
#2622=EDGE_LOOP('',(#5903,#5904,#5905,#5906));
#2623=EDGE_LOOP('',(#5907,#5908,#5909,#5910));
#2624=EDGE_LOOP('',(#5911,#5912,#5913,#5914));
#2625=EDGE_LOOP('',(#5915,#5916,#5917,#5918));
#2626=EDGE_LOOP('',(#5919,#5920,#5921,#5922));
#2627=EDGE_LOOP('',(#5923,#5924,#5925,#5926));
#2628=EDGE_LOOP('',(#5927,#5928,#5929,#5930));
#2629=EDGE_LOOP('',(#5931,#5932,#5933,#5934));
#2630=EDGE_LOOP('',(#5935,#5936,#5937,#5938,#5939,#5940,#5941,#5942,#5943,
#5944,#5945,#5946,#5947,#5948,#5949,#5950,#5951,#5952,#5953,#5954,#5955,
#5956,#5957,#5958,#5959,#5960,#5961,#5962,#5963,#5964,#5965,#5966,#5967,
#5968,#5969,#5970,#5971,#5972,#5973,#5974,#5975,#5976,#5977,#5978,#5979));
#2631=EDGE_LOOP('',(#5980));
#2632=EDGE_LOOP('',(#5981,#5982,#5983,#5984));
#2633=EDGE_LOOP('',(#5985,#5986,#5987,#5988));
#2634=EDGE_LOOP('',(#5989,#5990,#5991,#5992));
#2635=EDGE_LOOP('',(#5993,#5994,#5995,#5996));
#2636=EDGE_LOOP('',(#5997,#5998,#5999,#6000));
#2637=EDGE_LOOP('',(#6001,#6002,#6003,#6004));
#2638=EDGE_LOOP('',(#6005,#6006,#6007,#6008));
#2639=EDGE_LOOP('',(#6009,#6010,#6011,#6012));
#2640=EDGE_LOOP('',(#6013,#6014,#6015,#6016));
#2641=EDGE_LOOP('',(#6017,#6018,#6019,#6020));
#2642=EDGE_LOOP('',(#6021,#6022,#6023,#6024));
#2643=EDGE_LOOP('',(#6025,#6026,#6027,#6028));
#2644=EDGE_LOOP('',(#6029,#6030,#6031,#6032));
#2645=EDGE_LOOP('',(#6033,#6034,#6035,#6036));
#2646=EDGE_LOOP('',(#6037,#6038,#6039,#6040));
#2647=EDGE_LOOP('',(#6041,#6042,#6043,#6044));
#2648=EDGE_LOOP('',(#6045,#6046,#6047,#6048));
#2649=EDGE_LOOP('',(#6049,#6050,#6051,#6052));
#2650=EDGE_LOOP('',(#6053,#6054,#6055));
#2651=EDGE_LOOP('',(#6056,#6057,#6058,#6059));
#2652=EDGE_LOOP('',(#6060,#6061,#6062,#6063));
#2653=EDGE_LOOP('',(#6064,#6065,#6066,#6067));
#2654=EDGE_LOOP('',(#6068,#6069,#6070,#6071));
#2655=EDGE_LOOP('',(#6072,#6073,#6074,#6075,#6076,#6077,#6078));
#2656=EDGE_LOOP('',(#6079,#6080,#6081,#6082,#6083,#6084,#6085,#6086,#6087,
#6088,#6089,#6090,#6091,#6092));
#2657=EDGE_LOOP('',(#6093,#6094,#6095,#6096));
#2658=EDGE_LOOP('',(#6097,#6098,#6099,#6100));
#2659=EDGE_LOOP('',(#6101,#6102,#6103,#6104,#6105,#6106,#6107,#6108,#6109,
#6110,#6111,#6112,#6113,#6114,#6115,#6116,#6117,#6118,#6119));
#2660=EDGE_LOOP('',(#6120,#6121,#6122,#6123));
#2661=EDGE_LOOP('',(#6124,#6125,#6126,#6127));
#2662=EDGE_LOOP('',(#6128,#6129,#6130,#6131));
#2663=EDGE_LOOP('',(#6132,#6133,#6134,#6135));
#2664=EDGE_LOOP('',(#6136,#6137,#6138,#6139,#6140,#6141,#6142));
#2665=EDGE_LOOP('',(#6143));
#2666=EDGE_LOOP('',(#6144,#6145,#6146,#6147,#6148,#6149,#6150));
#2667=EDGE_LOOP('',(#6151));
#2668=EDGE_LOOP('',(#6152,#6153,#6154,#6155));
#2669=EDGE_LOOP('',(#6156,#6157,#6158,#6159));
#2670=EDGE_LOOP('',(#6160,#6161,#6162,#6163));
#2671=EDGE_LOOP('',(#6164,#6165,#6166,#6167));
#2672=EDGE_LOOP('',(#6168,#6169,#6170,#6171,#6172,#6173,#6174,#6175,#6176,
#6177,#6178,#6179,#6180,#6181,#6182,#6183,#6184,#6185,#6186,#6187,#6188,
#6189,#6190,#6191,#6192,#6193,#6194,#6195,#6196,#6197,#6198,#6199,#6200,
#6201,#6202,#6203,#6204,#6205,#6206,#6207,#6208,#6209,#6210,#6211,#6212,
#6213));
#2673=EDGE_LOOP('',(#6214));
#2674=EDGE_LOOP('',(#6215,#6216,#6217,#6218,#6219));
#2675=EDGE_LOOP('',(#6220,#6221,#6222));
#2676=EDGE_LOOP('',(#6223,#6224,#6225,#6226,#6227,#6228));
#2677=EDGE_LOOP('',(#6229,#6230,#6231,#6232,#6233,#6234,#6235));
#2678=EDGE_LOOP('',(#6236,#6237,#6238,#6239,#6240,#6241,#6242,#6243,#6244,
#6245));
#2679=EDGE_LOOP('',(#6246,#6247,#6248,#6249,#6250,#6251));
#2680=EDGE_LOOP('',(#6252,#6253,#6254,#6255));
#2681=EDGE_LOOP('',(#6256,#6257,#6258,#6259,#6260,#6261,#6262,#6263,#6264,
#6265));
#2682=EDGE_LOOP('',(#6266,#6267,#6268,#6269,#6270,#6271,#6272,#6273,#6274,
#6275,#6276,#6277,#6278,#6279,#6280,#6281,#6282,#6283,#6284,#6285,#6286,
#6287,#6288,#6289,#6290,#6291,#6292));
#2683=EDGE_LOOP('',(#6293,#6294,#6295,#6296));
#2684=EDGE_LOOP('',(#6297,#6298,#6299,#6300));
#2685=EDGE_LOOP('',(#6301,#6302,#6303,#6304,#6305,#6306,#6307,#6308,#6309,
#6310,#6311,#6312,#6313,#6314,#6315,#6316,#6317,#6318,#6319,#6320,#6321,
#6322,#6323,#6324,#6325,#6326,#6327));
#2686=EDGE_LOOP('',(#6328,#6329,#6330,#6331));
#2687=EDGE_LOOP('',(#6332,#6333,#6334,#6335));
#2688=EDGE_LOOP('',(#6336,#6337,#6338,#6339));
#2689=EDGE_LOOP('',(#6340,#6341,#6342,#6343));
#2690=EDGE_LOOP('',(#6344,#6345,#6346,#6347));
#2691=EDGE_LOOP('',(#6348,#6349,#6350,#6351));
#2692=EDGE_LOOP('',(#6352,#6353,#6354,#6355));
#2693=EDGE_LOOP('',(#6356,#6357,#6358,#6359));
#2694=EDGE_LOOP('',(#6360,#6361,#6362,#6363));
#2695=EDGE_LOOP('',(#6364,#6365,#6366,#6367));
#2696=EDGE_LOOP('',(#6368,#6369,#6370,#6371));
#2697=EDGE_LOOP('',(#6372,#6373,#6374,#6375));
#2698=EDGE_LOOP('',(#6376,#6377,#6378,#6379));
#2699=EDGE_LOOP('',(#6380,#6381,#6382,#6383));
#2700=EDGE_LOOP('',(#6384,#6385,#6386,#6387));
#2701=EDGE_LOOP('',(#6388,#6389,#6390,#6391));
#2702=EDGE_LOOP('',(#6392,#6393,#6394,#6395));
#2703=EDGE_LOOP('',(#6396,#6397,#6398,#6399));
#2704=EDGE_LOOP('',(#6400,#6401,#6402,#6403));
#2705=EDGE_LOOP('',(#6404,#6405,#6406,#6407));
#2706=EDGE_LOOP('',(#6408,#6409,#6410,#6411));
#2707=EDGE_LOOP('',(#6412,#6413,#6414,#6415,#6416));
#2708=EDGE_LOOP('',(#6417,#6418,#6419));
#2709=EDGE_LOOP('',(#6420,#6421,#6422,#6423,#6424));
#2710=EDGE_LOOP('',(#6425,#6426,#6427));
#2711=EDGE_LOOP('',(#6428,#6429,#6430,#6431));
#2712=EDGE_LOOP('',(#6432,#6433,#6434,#6435));
#2713=EDGE_LOOP('',(#6436,#6437,#6438,#6439,#6440));
#2714=EDGE_LOOP('',(#6441,#6442,#6443,#6444));
#2715=EDGE_LOOP('',(#6445,#6446,#6447,#6448));
#2716=EDGE_LOOP('',(#6449,#6450,#6451,#6452,#6453));
#2717=EDGE_LOOP('',(#6454,#6455));
#2718=EDGE_LOOP('',(#6456,#6457,#6458));
#2719=EDGE_LOOP('',(#6459,#6460,#6461));
#2720=EDGE_LOOP('',(#6462,#6463));
#2721=EDGE_LOOP('',(#6464,#6465,#6466,#6467));
#2722=EDGE_LOOP('',(#6468,#6469,#6470,#6471));
#2723=EDGE_LOOP('',(#6472,#6473,#6474,#6475));
#2724=EDGE_LOOP('',(#6476,#6477,#6478,#6479));
#2725=EDGE_LOOP('',(#6480,#6481,#6482,#6483));
#2726=EDGE_LOOP('',(#6484,#6485,#6486,#6487));
#2727=EDGE_LOOP('',(#6488,#6489,#6490,#6491));
#2728=EDGE_LOOP('',(#6492,#6493,#6494,#6495));
#2729=EDGE_LOOP('',(#6496,#6497,#6498,#6499));
#2730=EDGE_LOOP('',(#6500,#6501,#6502,#6503));
#2731=EDGE_LOOP('',(#6504,#6505,#6506,#6507));
#2732=EDGE_LOOP('',(#6508,#6509,#6510,#6511));
#2733=EDGE_LOOP('',(#6512,#6513,#6514,#6515));
#2734=EDGE_LOOP('',(#6516,#6517,#6518,#6519));
#2735=EDGE_LOOP('',(#6520,#6521,#6522,#6523));
#2736=EDGE_LOOP('',(#6524,#6525,#6526,#6527));
#2737=EDGE_LOOP('',(#6528,#6529,#6530,#6531));
#2738=EDGE_LOOP('',(#6532,#6533,#6534,#6535,#6536,#6537,#6538,#6539,#6540));
#2739=EDGE_LOOP('',(#6541,#6542,#6543,#6544));
#2740=EDGE_LOOP('',(#6545,#6546,#6547,#6548,#6549,#6550));
#2741=EDGE_LOOP('',(#6551,#6552,#6553,#6554));
#2742=EDGE_LOOP('',(#6555,#6556));
#2743=EDGE_LOOP('',(#6557,#6558,#6559,#6560));
#2744=EDGE_LOOP('',(#6561,#6562,#6563,#6564));
#2745=EDGE_LOOP('',(#6565,#6566,#6567,#6568,#6569,#6570,#6571,#6572));
#2746=EDGE_LOOP('',(#6573,#6574,#6575,#6576,#6577,#6578,#6579));
#2747=EDGE_LOOP('',(#6580,#6581,#6582,#6583,#6584));
#2748=EDGE_LOOP('',(#6585,#6586,#6587,#6588,#6589,#6590,#6591,#6592));
#2749=EDGE_LOOP('',(#6593,#6594,#6595,#6596,#6597,#6598,#6599,#6600));
#2750=EDGE_LOOP('',(#6601,#6602,#6603,#6604));
#2751=EDGE_LOOP('',(#6605,#6606,#6607,#6608,#6609,#6610,#6611,#6612));
#2752=EDGE_LOOP('',(#6613,#6614,#6615,#6616,#6617,#6618,#6619,#6620));
#2753=EDGE_LOOP('',(#6621,#6622,#6623,#6624));
#2754=EDGE_LOOP('',(#6625,#6626,#6627,#6628,#6629,#6630,#6631,#6632));
#2755=EDGE_LOOP('',(#6633,#6634,#6635,#6636,#6637,#6638,#6639,#6640));
#2756=EDGE_LOOP('',(#6641,#6642,#6643,#6644));
#2757=EDGE_LOOP('',(#6645,#6646,#6647,#6648,#6649,#6650,#6651,#6652));
#2758=EDGE_LOOP('',(#6653,#6654,#6655,#6656,#6657,#6658,#6659,#6660));
#2759=EDGE_LOOP('',(#6661,#6662,#6663,#6664));
#2760=EDGE_LOOP('',(#6665,#6666,#6667,#6668,#6669,#6670,#6671,#6672));
#2761=EDGE_LOOP('',(#6673,#6674,#6675,#6676,#6677,#6678,#6679,#6680));
#2762=EDGE_LOOP('',(#6681,#6682,#6683,#6684));
#2763=EDGE_LOOP('',(#6685,#6686,#6687,#6688,#6689));
#2764=EDGE_LOOP('',(#6690,#6691,#6692));
#2765=EDGE_LOOP('',(#6693,#6694,#6695,#6696));
#2766=EDGE_LOOP('',(#6697,#6698,#6699,#6700));
#2767=EDGE_LOOP('',(#6701,#6702,#6703,#6704));
#2768=EDGE_LOOP('',(#6705,#6706,#6707,#6708));
#2769=EDGE_LOOP('',(#6709,#6710,#6711,#6712));
#2770=EDGE_LOOP('',(#6713,#6714,#6715,#6716,#6717));
#2771=EDGE_LOOP('',(#6718,#6719,#6720,#6721,#6722));
#2772=EDGE_LOOP('',(#6723,#6724,#6725,#6726));
#2773=EDGE_LOOP('',(#6727,#6728,#6729,#6730));
#2774=EDGE_LOOP('',(#6731,#6732,#6733,#6734));
#2775=EDGE_LOOP('',(#6735,#6736,#6737,#6738));
#3154=CIRCLE('',#9124,5.);
#3155=CIRCLE('',#9125,5.);
#3156=CIRCLE('',#9126,5.);
#3157=CIRCLE('',#9127,5.);
#3158=CIRCLE('',#9129,39.);
#3159=CIRCLE('',#9130,0.500000000000002);
#3160=CIRCLE('',#9131,39.5);
#3161=CIRCLE('',#9133,39.5);
#3162=CIRCLE('',#9134,0.499999999999999);
#3163=CIRCLE('',#9135,39.);
#3164=CIRCLE('',#9137,5.72168783648703);
#3165=CIRCLE('',#9138,6.15470053837925);
#3166=CIRCLE('',#9139,0.500126081010092);
#3167=CIRCLE('',#9141,6.15470053837925);
#3168=CIRCLE('',#9142,5.72168783648703);
#3169=CIRCLE('',#9143,0.500126081010098);
#3170=CIRCLE('',#9145,5.);
#3171=CIRCLE('',#9147,5.);
#3172=CIRCLE('',#9149,2.);
#3173=CIRCLE('',#9150,2.);
#3174=CIRCLE('',#9152,2.);
#3175=CIRCLE('',#9153,2.);
#3176=CIRCLE('',#9155,15.);
#3177=CIRCLE('',#9156,15.);
#3178=CIRCLE('',#9158,15.);
#3179=CIRCLE('',#9159,15.);
#3180=CIRCLE('',#9161,4.);
#3181=CIRCLE('',#9162,4.);
#3182=CIRCLE('',#9165,4.);
#3183=CIRCLE('',#9181,15.5);
#3184=CIRCLE('',#9182,14.5);
#3185=CIRCLE('',#9192,3.);
#3186=CIRCLE('',#9195,4.5);
#3187=CIRCLE('',#9196,9.5);
#3188=CIRCLE('',#9197,12.2);
#3189=CIRCLE('',#9199,0.5);
#3190=CIRCLE('',#9200,0.5);
#3191=CIRCLE('',#9204,0.5);
#3192=CIRCLE('',#9205,4.);
#3193=CIRCLE('',#9206,4.);
#3194=CIRCLE('',#9207,0.5);
#3195=CIRCLE('',#9208,0.5);
#3196=CIRCLE('',#9209,1.49999774798038);
#3197=CIRCLE('',#9210,1.5);
#3198=CIRCLE('',#9212,15.);
#3199=CIRCLE('',#9213,15.);
#3200=CIRCLE('',#9217,14.5);
#3201=CIRCLE('',#9218,15.5);
#3202=CIRCLE('',#9220,15.5);
#3203=CIRCLE('',#9221,14.5);
#3204=CIRCLE('',#9223,15.);
#3205=CIRCLE('',#9224,15.);
#3206=CIRCLE('',#9239,12.2);
#3207=CIRCLE('',#9240,9.5);
#3208=CIRCLE('',#9241,4.5);
#3209=CIRCLE('',#9246,11.7);
#3210=CIRCLE('',#9247,11.7);
#3211=CIRCLE('',#9248,11.7);
#3212=CIRCLE('',#9249,11.7);
#3213=CIRCLE('',#9251,10.);
#3214=CIRCLE('',#9255,10.);
#3215=CIRCLE('',#9257,10.721687836487);
#3216=CIRCLE('',#9259,10.721687836487);
#3217=CIRCLE('',#9280,0.499999999999998);
#3218=CIRCLE('',#9285,0.499999999999999);
#3219=CIRCLE('',#9287,0.500000000000002);
#3220=CIRCLE('',#9288,0.500000000000001);
#3221=CIRCLE('',#9289,0.500000000000002);
#3222=CIRCLE('',#9290,0.500000000000003);
#3223=CIRCLE('',#9293,4.);
#3224=CIRCLE('',#9297,0.5);
#3225=CIRCLE('',#9299,0.500000000000003);
#3226=CIRCLE('',#9301,0.500000000000003);
#3227=CIRCLE('',#9304,0.5);
#3228=CIRCLE('',#9306,0.500000000000003);
#3229=CIRCLE('',#9308,0.500000000000003);
#3230=CIRCLE('',#9310,0.5);
#3231=CIRCLE('',#9312,0.5);
#3232=CIRCLE('',#9313,0.500000000000001);
#3233=CIRCLE('',#9315,0.500000000000001);
#3234=CIRCLE('',#9316,0.5);
#3235=CIRCLE('',#9318,0.5);
#3236=CIRCLE('',#9320,0.500000000000003);
#3237=CIRCLE('',#9322,0.500000000000003);
#3238=CIRCLE('',#9324,0.5);
#3239=CIRCLE('',#9326,4.0000000000001);
#3240=CIRCLE('',#9329,10.);
#3241=CIRCLE('',#9330,10.);
#3242=CIRCLE('',#9331,0.500000000000003);
#3243=CIRCLE('',#9332,0.499999999999998);
#3244=CIRCLE('',#9334,0.500000000000002);
#3245=CIRCLE('',#9336,0.499999999999998);
#3246=CIRCLE('',#9339,0.499999999999998);
#3247=CIRCLE('',#9341,0.499999999999999);
#3248=CIRCLE('',#9343,0.499999999999998);
#3249=CIRCLE('',#9344,0.500000000000003);
#3558=VERTEX_POINT('',#15691);
#3559=VERTEX_POINT('',#15692);
#3560=VERTEX_POINT('',#15694);
#3561=VERTEX_POINT('',#15696);
#3562=VERTEX_POINT('',#15698);
#3563=VERTEX_POINT('',#15700);
#3564=VERTEX_POINT('',#15702);
#3565=VERTEX_POINT('',#15704);
#3566=VERTEX_POINT('',#15706);
#3567=VERTEX_POINT('',#15721);
#3568=VERTEX_POINT('',#15722);
#3569=VERTEX_POINT('',#15724);
#3570=VERTEX_POINT('',#15726);
#3571=VERTEX_POINT('',#15739);
#3572=VERTEX_POINT('',#15740);
#3573=VERTEX_POINT('',#15742);
#3574=VERTEX_POINT('',#15744);
#3575=VERTEX_POINT('',#15757);
#3576=VERTEX_POINT('',#15758);
#3577=VERTEX_POINT('',#15760);
#3578=VERTEX_POINT('',#15792);
#3579=VERTEX_POINT('',#15796);
#3580=VERTEX_POINT('',#15797);
#3581=VERTEX_POINT('',#15799);
#3582=VERTEX_POINT('',#15831);
#3583=VERTEX_POINT('',#15835);
#3584=VERTEX_POINT('',#15836);
#3585=VERTEX_POINT('',#15847);
#3586=VERTEX_POINT('',#15848);
#3587=VERTEX_POINT('',#15859);
#3588=VERTEX_POINT('',#15861);
#3589=VERTEX_POINT('',#15865);
#3590=VERTEX_POINT('',#15867);
#3591=VERTEX_POINT('',#15871);
#3592=VERTEX_POINT('',#15873);
#3593=VERTEX_POINT('',#15882);
#3594=VERTEX_POINT('',#15884);
#3595=VERTEX_POINT('',#15888);
#3596=VERTEX_POINT('',#15889);
#3597=VERTEX_POINT('',#15891);
#3598=VERTEX_POINT('',#15903);
#3599=VERTEX_POINT('',#15907);
#3600=VERTEX_POINT('',#15908);
#3601=VERTEX_POINT('',#15921);
#3602=VERTEX_POINT('',#15923);
#3603=VERTEX_POINT('',#15936);
#3604=VERTEX_POINT('',#15938);
#3605=VERTEX_POINT('',#15940);
#3606=VERTEX_POINT('',#15942);
#3607=VERTEX_POINT('',#16082);
#3608=VERTEX_POINT('',#16150);
#3609=VERTEX_POINT('',#16173);
#3610=VERTEX_POINT('',#16175);
#3611=VERTEX_POINT('',#16177);
#3612=VERTEX_POINT('',#16179);
#3613=VERTEX_POINT('',#16212);
#3614=VERTEX_POINT('',#16213);
#3615=VERTEX_POINT('',#16244);
#3616=VERTEX_POINT('',#16246);
#3617=VERTEX_POINT('',#16279);
#3618=VERTEX_POINT('',#16280);
#3619=VERTEX_POINT('',#16311);
#3620=VERTEX_POINT('',#16313);
#3621=VERTEX_POINT('',#16332);
#3622=VERTEX_POINT('',#16336);
#3623=VERTEX_POINT('',#16337);
#3624=VERTEX_POINT('',#16348);
#3625=VERTEX_POINT('',#16350);
#3626=VERTEX_POINT('',#16363);
#3627=VERTEX_POINT('',#16364);
#3628=VERTEX_POINT('',#16375);
#3629=VERTEX_POINT('',#16377);
#3630=VERTEX_POINT('',#16390);
#3631=VERTEX_POINT('',#16391);
#3632=VERTEX_POINT('',#16402);
#3633=VERTEX_POINT('',#16404);
#3634=VERTEX_POINT('',#16417);
#3635=VERTEX_POINT('',#16418);
#3636=VERTEX_POINT('',#16429);
#3637=VERTEX_POINT('',#16431);
#3638=VERTEX_POINT('',#16444);
#3639=VERTEX_POINT('',#16445);
#3640=VERTEX_POINT('',#16456);
#3641=VERTEX_POINT('',#16458);
#3642=VERTEX_POINT('',#16471);
#3643=VERTEX_POINT('',#16472);
#3644=VERTEX_POINT('',#16483);
#3645=VERTEX_POINT('',#16485);
#3646=VERTEX_POINT('',#16498);
#3647=VERTEX_POINT('',#16499);
#3648=VERTEX_POINT('',#16510);
#3649=VERTEX_POINT('',#16512);
#3650=VERTEX_POINT('',#16532);
#3651=VERTEX_POINT('',#16533);
#3652=VERTEX_POINT('',#16571);
#3653=VERTEX_POINT('',#16576);
#3654=VERTEX_POINT('',#16626);
#3655=VERTEX_POINT('',#16627);
#3656=VERTEX_POINT('',#16668);
#3657=VERTEX_POINT('',#16673);
#3658=VERTEX_POINT('',#16723);
#3659=VERTEX_POINT('',#16724);
#3660=VERTEX_POINT('',#16759);
#3661=VERTEX_POINT('',#16764);
#3662=VERTEX_POINT('',#16811);
#3663=VERTEX_POINT('',#16812);
#3664=VERTEX_POINT('',#16850);
#3665=VERTEX_POINT('',#16855);
#3666=VERTEX_POINT('',#16902);
#3667=VERTEX_POINT('',#16903);
#3668=VERTEX_POINT('',#16941);
#3669=VERTEX_POINT('',#16946);
#3670=VERTEX_POINT('',#16993);
#3671=VERTEX_POINT('',#16994);
#3672=VERTEX_POINT('',#17032);
#3673=VERTEX_POINT('',#17037);
#3674=VERTEX_POINT('',#17081);
#3675=VERTEX_POINT('',#17083);
#3676=VERTEX_POINT('',#17085);
#3677=VERTEX_POINT('',#17092);
#3678=VERTEX_POINT('',#17094);
#3679=VERTEX_POINT('',#17101);
#3680=VERTEX_POINT('',#17103);
#3681=VERTEX_POINT('',#17110);
#3682=VERTEX_POINT('',#17112);
#3683=VERTEX_POINT('',#17119);
#3684=VERTEX_POINT('',#17121);
#3685=VERTEX_POINT('',#17128);
#3686=VERTEX_POINT('',#17130);
#3687=VERTEX_POINT('',#17137);
#3688=VERTEX_POINT('',#17139);
#3689=VERTEX_POINT('',#17146);
#3690=VERTEX_POINT('',#17148);
#3691=VERTEX_POINT('',#17155);
#3692=VERTEX_POINT('',#17157);
#3693=VERTEX_POINT('',#17164);
#3694=VERTEX_POINT('',#17166);
#3695=VERTEX_POINT('',#17173);
#3696=VERTEX_POINT('',#17175);
#3697=VERTEX_POINT('',#17182);
#3698=VERTEX_POINT('',#17184);
#3699=VERTEX_POINT('',#17191);
#3700=VERTEX_POINT('',#17193);
#3701=VERTEX_POINT('',#17200);
#3702=VERTEX_POINT('',#17207);
#3703=VERTEX_POINT('',#17209);
#3704=VERTEX_POINT('',#17211);
#3705=VERTEX_POINT('',#17213);
#3706=VERTEX_POINT('',#17216);
#3707=VERTEX_POINT('',#17569);
#3708=VERTEX_POINT('',#17584);
#3709=VERTEX_POINT('',#17614);
#3710=VERTEX_POINT('',#17629);
#3711=VERTEX_POINT('',#17659);
#3712=VERTEX_POINT('',#17676);
#3713=VERTEX_POINT('',#17706);
#3714=VERTEX_POINT('',#17723);
#3715=VERTEX_POINT('',#17755);
#3716=VERTEX_POINT('',#17772);
#3717=VERTEX_POINT('',#17804);
#3718=VERTEX_POINT('',#17823);
#3719=VERTEX_POINT('',#17906);
#3720=VERTEX_POINT('',#17948);
#3721=VERTEX_POINT('',#18046);
#3722=VERTEX_POINT('',#18152);
#3723=VERTEX_POINT('',#18335);
#3724=VERTEX_POINT('',#18337);
#3725=VERTEX_POINT('',#18339);
#3726=VERTEX_POINT('',#18344);
#3727=VERTEX_POINT('',#18345);
#3728=VERTEX_POINT('',#18380);
#3729=VERTEX_POINT('',#18383);
#3730=VERTEX_POINT('',#18385);
#3731=VERTEX_POINT('',#18425);
#3732=VERTEX_POINT('',#18427);
#3733=VERTEX_POINT('',#18431);
#3734=VERTEX_POINT('',#18432);
#3735=VERTEX_POINT('',#18434);
#3736=VERTEX_POINT('',#18436);
#3737=VERTEX_POINT('',#18440);
#3738=VERTEX_POINT('',#18441);
#3739=VERTEX_POINT('',#18454);
#3740=VERTEX_POINT('',#18462);
#3741=VERTEX_POINT('',#18464);
#3742=VERTEX_POINT('',#18466);
#3743=VERTEX_POINT('',#18468);
#3744=VERTEX_POINT('',#18470);
#3745=VERTEX_POINT('',#18472);
#3746=VERTEX_POINT('',#18474);
#3747=VERTEX_POINT('',#18476);
#3748=VERTEX_POINT('',#18479);
#3749=VERTEX_POINT('',#18486);
#3750=VERTEX_POINT('',#18499);
#3751=VERTEX_POINT('',#18501);
#3752=VERTEX_POINT('',#18505);
#3753=VERTEX_POINT('',#18506);
#3754=VERTEX_POINT('',#18508);
#3755=VERTEX_POINT('',#18510);
#3756=VERTEX_POINT('',#18521);
#3757=VERTEX_POINT('',#18548);
#3758=VERTEX_POINT('',#18585);
#3759=VERTEX_POINT('',#18671);
#3760=VERTEX_POINT('',#18673);
#3761=VERTEX_POINT('',#18675);
#3762=VERTEX_POINT('',#18677);
#3763=VERTEX_POINT('',#18681);
#3764=VERTEX_POINT('',#18683);
#3765=VERTEX_POINT('',#18685);
#3766=VERTEX_POINT('',#18687);
#3767=VERTEX_POINT('',#18689);
#3768=VERTEX_POINT('',#19125);
#3769=VERTEX_POINT('',#19126);
#3770=VERTEX_POINT('',#19157);
#3771=VERTEX_POINT('',#19163);
#3772=VERTEX_POINT('',#19171);
#3773=VERTEX_POINT('',#19178);
#3774=VERTEX_POINT('',#19186);
#3775=VERTEX_POINT('',#19193);
#3776=VERTEX_POINT('',#19201);
#3777=VERTEX_POINT('',#19208);
#3778=VERTEX_POINT('',#19216);
#3779=VERTEX_POINT('',#19223);
#3780=VERTEX_POINT('',#19231);
#3781=VERTEX_POINT('',#19238);
#3782=VERTEX_POINT('',#19246);
#3783=VERTEX_POINT('',#19253);
#3784=VERTEX_POINT('',#19261);
#3785=VERTEX_POINT('',#19268);
#3786=VERTEX_POINT('',#19334);
#3787=VERTEX_POINT('',#19336);
#3788=VERTEX_POINT('',#19341);
#3789=VERTEX_POINT('',#19342);
#3790=VERTEX_POINT('',#19344);
#3791=VERTEX_POINT('',#19364);
#3792=VERTEX_POINT('',#19394);
#3793=VERTEX_POINT('',#19399);
#3794=VERTEX_POINT('',#19445);
#3795=VERTEX_POINT('',#19446);
#3796=VERTEX_POINT('',#19454);
#3797=VERTEX_POINT('',#19461);
#3798=VERTEX_POINT('',#19465);
#3799=VERTEX_POINT('',#19466);
#3800=VERTEX_POINT('',#19471);
#3801=VERTEX_POINT('',#19472);
#3802=VERTEX_POINT('',#19474);
#3803=VERTEX_POINT('',#19479);
#3804=VERTEX_POINT('',#19526);
#3805=VERTEX_POINT('',#19528);
#3806=VERTEX_POINT('',#19530);
#3807=VERTEX_POINT('',#19532);
#3808=VERTEX_POINT('',#19582);
#3809=VERTEX_POINT('',#19587);
#3810=VERTEX_POINT('',#19605);
#3811=VERTEX_POINT('',#19607);
#3812=VERTEX_POINT('',#19615);
#3813=VERTEX_POINT('',#19617);
#3814=VERTEX_POINT('',#19619);
#3815=VERTEX_POINT('',#19621);
#3816=VERTEX_POINT('',#19623);
#3817=VERTEX_POINT('',#19625);
#3818=VERTEX_POINT('',#19627);
#3819=VERTEX_POINT('',#19629);
#3820=VERTEX_POINT('',#19631);
#3821=VERTEX_POINT('',#19633);
#3822=VERTEX_POINT('',#19635);
#3823=VERTEX_POINT('',#19637);
#3824=VERTEX_POINT('',#19639);
#3825=VERTEX_POINT('',#19641);
#3826=VERTEX_POINT('',#19643);
#3827=VERTEX_POINT('',#19645);
#3828=VERTEX_POINT('',#19647);
#3829=VERTEX_POINT('',#19649);
#3830=VERTEX_POINT('',#19653);
#3831=VERTEX_POINT('',#19657);
#3832=VERTEX_POINT('',#19658);
#3833=VERTEX_POINT('',#19677);
#3834=VERTEX_POINT('',#19679);
#3835=VERTEX_POINT('',#19681);
#3836=VERTEX_POINT('',#19683);
#3837=VERTEX_POINT('',#19685);
#3838=VERTEX_POINT('',#19687);
#3839=VERTEX_POINT('',#19689);
#3840=VERTEX_POINT('',#19691);
#3841=VERTEX_POINT('',#19693);
#3842=VERTEX_POINT('',#19695);
#3843=VERTEX_POINT('',#19697);
#3844=VERTEX_POINT('',#19699);
#3845=VERTEX_POINT('',#19701);
#3846=VERTEX_POINT('',#19703);
#3847=VERTEX_POINT('',#19705);
#3848=VERTEX_POINT('',#19707);
#3849=VERTEX_POINT('',#19709);
#3850=VERTEX_POINT('',#19711);
#3851=VERTEX_POINT('',#19714);
#3852=VERTEX_POINT('',#19723);
#3853=VERTEX_POINT('',#19736);
#3854=VERTEX_POINT('',#19786);
#3855=VERTEX_POINT('',#19822);
#3856=VERTEX_POINT('',#19971);
#4429=EDGE_CURVE('',#3558,#3559,#3154,.T.);
#4430=EDGE_CURVE('',#3560,#3559,#887,.T.);
#4431=EDGE_CURVE('',#3560,#3561,#3155,.T.);
#4432=EDGE_CURVE('',#3561,#3562,#888,.T.);
#4433=EDGE_CURVE('',#3563,#3562,#3156,.T.);
#4434=EDGE_CURVE('',#3564,#3563,#889,.T.);
#4435=EDGE_CURVE('',#3565,#3564,#3157,.T.);
#4436=EDGE_CURVE('',#3566,#3565,#154,.T.);
#4437=EDGE_CURVE('',#3558,#3566,#890,.T.);
#4438=EDGE_CURVE('',#3567,#3568,#3158,.T.);
#4439=EDGE_CURVE('',#3569,#3567,#3159,.T.);
#4440=EDGE_CURVE('',#3570,#3569,#3160,.T.);
#4441=EDGE_CURVE('',#3568,#3570,#155,.T.);
#4442=EDGE_CURVE('',#3571,#3572,#3161,.T.);
#4443=EDGE_CURVE('',#3573,#3571,#3162,.T.);
#4444=EDGE_CURVE('',#3574,#3573,#3163,.T.);
#4445=EDGE_CURVE('',#3572,#3574,#156,.T.);
#4446=EDGE_CURVE('',#3575,#3576,#3164,.T.);
#4447=EDGE_CURVE('',#3575,#3577,#157,.T.);
#4448=EDGE_CURVE('',#3578,#3577,#3165,.T.);
#4449=EDGE_CURVE('',#3576,#3578,#3166,.T.);
#4450=EDGE_CURVE('',#3579,#3580,#3167,.T.);
#4451=EDGE_CURVE('',#3579,#3581,#158,.T.);
#4452=EDGE_CURVE('',#3582,#3581,#3168,.T.);
#4453=EDGE_CURVE('',#3580,#3582,#3169,.T.);
#4454=EDGE_CURVE('',#3583,#3584,#3170,.T.);
#4455=EDGE_CURVE('',#3582,#3583,#159,.T.);
#4456=EDGE_CURVE('',#3581,#3584,#160,.T.);
#4457=EDGE_CURVE('',#3585,#3586,#3171,.T.);
#4458=EDGE_CURVE('',#3586,#3575,#161,.T.);
#4459=EDGE_CURVE('',#3585,#3576,#162,.T.);
#4460=EDGE_CURVE('',#3587,#3587,#3172,.T.);
#4461=EDGE_CURVE('',#3587,#3588,#891,.T.);
#4462=EDGE_CURVE('',#3588,#3588,#3173,.T.);
#4463=EDGE_CURVE('',#3589,#3589,#3174,.T.);
#4464=EDGE_CURVE('',#3589,#3590,#892,.T.);
#4465=EDGE_CURVE('',#3590,#3590,#3175,.T.);
#4466=EDGE_CURVE('',#3591,#3562,#3176,.T.);
#4467=EDGE_CURVE('',#3561,#3592,#163,.T.);
#4468=EDGE_CURVE('',#3593,#3592,#893,.T.);
#4469=EDGE_CURVE('',#3593,#3594,#3177,.T.);
#4470=EDGE_CURVE('',#3591,#3594,#894,.T.);
#4471=EDGE_CURVE('',#3595,#3596,#3178,.T.);
#4472=EDGE_CURVE('',#3597,#3596,#895,.T.);
#4473=EDGE_CURVE('',#3597,#3558,#164,.T.);
#4474=EDGE_CURVE('',#3566,#3598,#3179,.T.);
#4475=EDGE_CURVE('',#3595,#3598,#896,.T.);
#4476=EDGE_CURVE('',#3599,#3600,#165,.T.);
#4477=EDGE_CURVE('',#3601,#3600,#897,.T.);
#4478=EDGE_CURVE('',#3602,#3601,#166,.F.);
#4479=EDGE_CURVE('',#3603,#3602,#898,.T.);
#4480=EDGE_CURVE('',#3604,#3603,#3180,.T.);
#4481=EDGE_CURVE('',#3605,#3604,#899,.T.);
#4482=EDGE_CURVE('',#3606,#3605,#167,.T.);
#4483=EDGE_CURVE('',#3606,#3607,#168,.T.);
#4484=EDGE_CURVE('',#3608,#3607,#169,.T.);
#4485=EDGE_CURVE('',#3608,#3609,#900,.T.);
#4486=EDGE_CURVE('',#3610,#3609,#3181,.T.);
#4487=EDGE_CURVE('',#3610,#3611,#901,.T.);
#4488=EDGE_CURVE('',#3612,#3611,#170,.F.);
#4489=EDGE_CURVE('',#3599,#3612,#902,.T.);
#4490=EDGE_CURVE('',#3613,#3614,#171,.T.);
#4491=EDGE_CURVE('',#3614,#3615,#903,.T.);
#4492=EDGE_CURVE('',#3616,#3615,#172,.F.);
#4493=EDGE_CURVE('',#3613,#3616,#904,.T.);
#4494=EDGE_CURVE('',#3617,#3618,#173,.T.);
#4495=EDGE_CURVE('',#3618,#3619,#905,.T.);
#4496=EDGE_CURVE('',#3620,#3619,#174,.F.);
#4497=EDGE_CURVE('',#3620,#3621,#3182,.T.);
#4498=EDGE_CURVE('',#3617,#3621,#906,.T.);
#4499=EDGE_CURVE('',#3622,#3623,#175,.F.);
#4500=EDGE_CURVE('',#3622,#3624,#907,.T.);
#4501=EDGE_CURVE('',#3625,#3624,#176,.F.);
#4502=EDGE_CURVE('',#3623,#3625,#908,.T.);
#4503=EDGE_CURVE('',#3626,#3627,#177,.F.);
#4504=EDGE_CURVE('',#3626,#3628,#909,.T.);
#4505=EDGE_CURVE('',#3629,#3628,#178,.F.);
#4506=EDGE_CURVE('',#3627,#3629,#910,.T.);
#4507=EDGE_CURVE('',#3630,#3631,#179,.F.);
#4508=EDGE_CURVE('',#3630,#3632,#911,.T.);
#4509=EDGE_CURVE('',#3633,#3632,#180,.F.);
#4510=EDGE_CURVE('',#3631,#3633,#912,.T.);
#4511=EDGE_CURVE('',#3634,#3635,#181,.F.);
#4512=EDGE_CURVE('',#3634,#3636,#913,.T.);
#4513=EDGE_CURVE('',#3637,#3636,#182,.F.);
#4514=EDGE_CURVE('',#3635,#3637,#914,.T.);
#4515=EDGE_CURVE('',#3638,#3639,#183,.F.);
#4516=EDGE_CURVE('',#3638,#3640,#915,.T.);
#4517=EDGE_CURVE('',#3641,#3640,#184,.F.);
#4518=EDGE_CURVE('',#3639,#3641,#916,.T.);
#4519=EDGE_CURVE('',#3642,#3643,#185,.F.);
#4520=EDGE_CURVE('',#3642,#3644,#917,.T.);
#4521=EDGE_CURVE('',#3645,#3644,#186,.F.);
#4522=EDGE_CURVE('',#3643,#3645,#918,.T.);
#4523=EDGE_CURVE('',#3646,#3647,#187,.F.);
#4524=EDGE_CURVE('',#3646,#3648,#919,.T.);
#4525=EDGE_CURVE('',#3649,#3648,#188,.F.);
#4526=EDGE_CURVE('',#3647,#3649,#920,.T.);
#4527=EDGE_CURVE('',#3650,#3651,#189,.T.);
#4528=EDGE_CURVE('',#3652,#3650,#190,.T.);
#4529=EDGE_CURVE('',#3653,#3652,#191,.T.);
#4530=EDGE_CURVE('',#3651,#3653,#192,.T.);
#4531=EDGE_CURVE('',#3654,#3655,#193,.T.);
#4532=EDGE_CURVE('',#3656,#3654,#194,.T.);
#4533=EDGE_CURVE('',#3657,#3656,#195,.T.);
#4534=EDGE_CURVE('',#3655,#3657,#196,.T.);
#4535=EDGE_CURVE('',#3658,#3659,#197,.T.);
#4536=EDGE_CURVE('',#3660,#3658,#198,.T.);
#4537=EDGE_CURVE('',#3661,#3660,#199,.T.);
#4538=EDGE_CURVE('',#3659,#3661,#200,.T.);
#4539=EDGE_CURVE('',#3662,#3663,#201,.T.);
#4540=EDGE_CURVE('',#3664,#3662,#202,.T.);
#4541=EDGE_CURVE('',#3665,#3664,#203,.T.);
#4542=EDGE_CURVE('',#3663,#3665,#204,.T.);
#4543=EDGE_CURVE('',#3666,#3667,#205,.T.);
#4544=EDGE_CURVE('',#3668,#3666,#206,.T.);
#4545=EDGE_CURVE('',#3669,#3668,#207,.T.);
#4546=EDGE_CURVE('',#3667,#3669,#208,.T.);
#4547=EDGE_CURVE('',#3670,#3671,#209,.T.);
#4548=EDGE_CURVE('',#3672,#3670,#210,.T.);
#4549=EDGE_CURVE('',#3673,#3672,#211,.T.);
#4550=EDGE_CURVE('',#3671,#3673,#212,.T.);
#4551=EDGE_CURVE('',#3616,#3617,#90,.T.);
#4552=EDGE_CURVE('',#3621,#3674,#921,.T.);
#4553=EDGE_CURVE('',#3674,#3675,#922,.T.);
#4554=EDGE_CURVE('',#3675,#3676,#213,.T.);
#4555=EDGE_CURVE('',#3676,#3677,#91,.T.);
#4556=EDGE_CURVE('',#3677,#3678,#214,.T.);
#4557=EDGE_CURVE('',#3678,#3679,#923,.T.);
#4558=EDGE_CURVE('',#3679,#3680,#215,.T.);
#4559=EDGE_CURVE('',#3680,#3681,#92,.T.);
#4560=EDGE_CURVE('',#3681,#3682,#216,.T.);
#4561=EDGE_CURVE('',#3682,#3683,#924,.T.);
#4562=EDGE_CURVE('',#3683,#3684,#217,.T.);
#4563=EDGE_CURVE('',#3684,#3685,#93,.T.);
#4564=EDGE_CURVE('',#3685,#3686,#218,.T.);
#4565=EDGE_CURVE('',#3686,#3687,#925,.T.);
#4566=EDGE_CURVE('',#3687,#3688,#219,.T.);
#4567=EDGE_CURVE('',#3688,#3689,#94,.T.);
#4568=EDGE_CURVE('',#3689,#3690,#220,.T.);
#4569=EDGE_CURVE('',#3690,#3691,#926,.T.);
#4570=EDGE_CURVE('',#3691,#3692,#221,.T.);
#4571=EDGE_CURVE('',#3692,#3693,#95,.T.);
#4572=EDGE_CURVE('',#3693,#3694,#222,.T.);
#4573=EDGE_CURVE('',#3694,#3695,#927,.T.);
#4574=EDGE_CURVE('',#3695,#3696,#223,.T.);
#4575=EDGE_CURVE('',#3696,#3697,#96,.T.);
#4576=EDGE_CURVE('',#3697,#3698,#224,.T.);
#4577=EDGE_CURVE('',#3698,#3699,#928,.T.);
#4578=EDGE_CURVE('',#3699,#3700,#225,.T.);
#4579=EDGE_CURVE('',#3700,#3701,#226,.T.);
#4580=EDGE_CURVE('',#3702,#3701,#929,.T.);
#4581=EDGE_CURVE('',#3702,#3703,#930,.T.);
#4582=EDGE_CURVE('',#3703,#3704,#3183,.T.);
#4583=EDGE_CURVE('',#3704,#3705,#931,.T.);
#4584=EDGE_CURVE('',#3705,#3565,#3184,.T.);
#4585=EDGE_CURVE('',#3706,#3564,#932,.T.);
#4586=EDGE_CURVE('',#3605,#3706,#227,.T.);
#4587=EDGE_CURVE('',#3603,#3604,#933,.T.);
#4588=EDGE_CURVE('',#3602,#3599,#97,.T.);
#4589=EDGE_CURVE('',#3612,#3613,#98,.T.);
#4590=EDGE_CURVE('',#3625,#3659,#228,.T.);
#4591=EDGE_CURVE('',#3661,#3623,#229,.T.);
#4592=EDGE_CURVE('',#3629,#3663,#230,.T.);
#4593=EDGE_CURVE('',#3665,#3627,#231,.T.);
#4594=EDGE_CURVE('',#3633,#3667,#232,.T.);
#4595=EDGE_CURVE('',#3669,#3631,#233,.T.);
#4596=EDGE_CURVE('',#3637,#3671,#234,.T.);
#4597=EDGE_CURVE('',#3673,#3635,#235,.T.);
#4598=EDGE_CURVE('',#3641,#3655,#236,.T.);
#4599=EDGE_CURVE('',#3657,#3639,#237,.T.);
#4600=EDGE_CURVE('',#3645,#3651,#238,.T.);
#4601=EDGE_CURVE('',#3653,#3643,#239,.T.);
#4602=EDGE_CURVE('',#3650,#3707,#240,.T.);
#4603=EDGE_CURVE('',#3707,#3708,#934,.T.);
#4604=EDGE_CURVE('',#3708,#3652,#241,.T.);
#4605=EDGE_CURVE('',#3654,#3709,#242,.T.);
#4606=EDGE_CURVE('',#3709,#3710,#935,.T.);
#4607=EDGE_CURVE('',#3710,#3656,#243,.T.);
#4608=EDGE_CURVE('',#3670,#3711,#244,.T.);
#4609=EDGE_CURVE('',#3711,#3712,#936,.T.);
#4610=EDGE_CURVE('',#3712,#3672,#245,.T.);
#4611=EDGE_CURVE('',#3666,#3713,#246,.T.);
#4612=EDGE_CURVE('',#3713,#3714,#937,.T.);
#4613=EDGE_CURVE('',#3714,#3668,#247,.T.);
#4614=EDGE_CURVE('',#3662,#3715,#248,.T.);
#4615=EDGE_CURVE('',#3715,#3716,#938,.T.);
#4616=EDGE_CURVE('',#3716,#3664,#249,.T.);
#4617=EDGE_CURVE('',#3658,#3717,#250,.T.);
#4618=EDGE_CURVE('',#3717,#3718,#939,.T.);
#4619=EDGE_CURVE('',#3718,#3660,#251,.T.);
#4620=EDGE_CURVE('',#3699,#3707,#59,.T.);
#4621=EDGE_CURVE('',#3708,#3698,#60,.T.);
#4622=EDGE_CURVE('',#3695,#3709,#61,.T.);
#4623=EDGE_CURVE('',#3710,#3694,#62,.T.);
#4624=EDGE_CURVE('',#3691,#3711,#63,.T.);
#4625=EDGE_CURVE('',#3712,#3690,#64,.T.);
#4626=EDGE_CURVE('',#3687,#3713,#65,.T.);
#4627=EDGE_CURVE('',#3714,#3686,#66,.T.);
#4628=EDGE_CURVE('',#3683,#3715,#67,.T.);
#4629=EDGE_CURVE('',#3716,#3682,#68,.T.);
#4630=EDGE_CURVE('',#3679,#3717,#69,.T.);
#4631=EDGE_CURVE('',#3718,#3678,#70,.T.);
#4632=EDGE_CURVE('',#3675,#3719,#71,.T.);
#4633=EDGE_CURVE('',#3719,#3674,#3185,.T.);
#4634=EDGE_CURVE('',#3620,#3719,#252,.T.);
#4635=EDGE_CURVE('',#3720,#3606,#253,.T.);
#4636=EDGE_CURVE('',#3720,#3721,#940,.T.);
#4637=EDGE_CURVE('',#3607,#3721,#254,.T.);
#4638=EDGE_CURVE('',#3722,#3608,#255,.T.);
#4639=EDGE_CURVE('',#3721,#3722,#256,.T.);
#4640=EDGE_CURVE('',#3706,#3720,#257,.T.);
#4641=EDGE_CURVE('',#3568,#3723,#941,.T.);
#4642=EDGE_CURVE('',#3723,#3724,#3186,.T.);
#4643=EDGE_CURVE('',#3724,#3725,#3187,.T.);
#4644=EDGE_CURVE('',#3725,#3579,#3188,.T.);
#4645=EDGE_CURVE('',#3580,#3567,#942,.T.);
#4646=EDGE_CURVE('',#3726,#3727,#258,.T.);
#4647=EDGE_CURVE('',#3727,#3593,#943,.T.);
#4648=EDGE_CURVE('',#3592,#3723,#3189,.T.);
#4649=EDGE_CURVE('',#3572,#3570,#944,.T.);
#4650=EDGE_CURVE('',#3574,#3728,#945,.T.);
#4651=EDGE_CURVE('',#3728,#3597,#3190,.T.);
#4652=EDGE_CURVE('',#3596,#3729,#946,.T.);
#4653=EDGE_CURVE('',#3729,#3730,#259,.T.);
#4654=EDGE_CURVE('',#3730,#3726,#947,.T.);
#4655=EDGE_CURVE('',#3594,#3731,#948,.T.);
#4656=EDGE_CURVE('',#3731,#3732,#949,.T.);
#4657=EDGE_CURVE('',#3591,#3732,#950,.T.);
#4658=EDGE_CURVE('',#3733,#3734,#951,.T.);
#4659=EDGE_CURVE('',#3734,#3735,#952,.T.);
#4660=EDGE_CURVE('',#3736,#3735,#953,.T.);
#4661=EDGE_CURVE('',#3733,#3736,#954,.T.);
#4662=EDGE_CURVE('',#3737,#3738,#260,.T.);
#4663=EDGE_CURVE('',#3738,#3739,#261,.T.);
#4664=EDGE_CURVE('',#3736,#3739,#955,.T.);
#4665=EDGE_CURVE('',#3735,#3740,#3191,.T.);
#4666=EDGE_CURVE('',#3740,#3741,#956,.T.);
#4667=EDGE_CURVE('',#3741,#3742,#3192,.T.);
#4668=EDGE_CURVE('',#3743,#3742,#957,.T.);
#4669=EDGE_CURVE('',#3743,#3744,#3193,.T.);
#4670=EDGE_CURVE('',#3745,#3744,#958,.T.);
#4671=EDGE_CURVE('',#3745,#3746,#3194,.T.);
#4672=EDGE_CURVE('',#3746,#3747,#959,.T.);
#4673=EDGE_CURVE('',#3747,#3702,#3195,.T.);
#4674=EDGE_CURVE('',#3701,#3748,#262,.T.);
#4675=EDGE_CURVE('',#3748,#3749,#263,.T.);
#4676=EDGE_CURVE('',#3750,#3749,#3196,.T.);
#4677=EDGE_CURVE('',#3750,#3751,#960,.T.);
#4678=EDGE_CURVE('',#3737,#3751,#3197,.T.);
#4679=EDGE_CURVE('',#3752,#3753,#961,.T.);
#4680=EDGE_CURVE('',#3752,#3754,#3198,.T.);
#4681=EDGE_CURVE('',#3755,#3754,#962,.T.);
#4682=EDGE_CURVE('',#3755,#3753,#3199,.T.);
#4683=EDGE_CURVE('',#3742,#3756,#264,.T.);
#4684=EDGE_CURVE('',#3756,#3757,#963,.T.);
#4685=EDGE_CURVE('',#3757,#3743,#265,.T.);
#4686=EDGE_CURVE('',#3598,#3752,#964,.T.);
#4687=EDGE_CURVE('',#3753,#3595,#965,.T.);
#4688=EDGE_CURVE('',#3754,#3747,#966,.T.);
#4689=EDGE_CURVE('',#3746,#3755,#967,.T.);
#4690=EDGE_CURVE('',#3744,#3758,#266,.T.);
#4691=EDGE_CURVE('',#3758,#3759,#968,.T.);
#4692=EDGE_CURVE('',#3759,#3760,#3200,.T.);
#4693=EDGE_CURVE('',#3760,#3761,#969,.T.);
#4694=EDGE_CURVE('',#3761,#3762,#3201,.T.);
#4695=EDGE_CURVE('',#3762,#3745,#970,.T.);
#4696=EDGE_CURVE('',#3740,#3763,#971,.T.);
#4697=EDGE_CURVE('',#3763,#3764,#3202,.T.);
#4698=EDGE_CURVE('',#3764,#3765,#972,.T.);
#4699=EDGE_CURVE('',#3765,#3766,#3203,.T.);
#4700=EDGE_CURVE('',#3766,#3767,#973,.T.);
#4701=EDGE_CURVE('',#3767,#3741,#267,.T.);
#4702=EDGE_CURVE('',#3731,#3734,#3204,.T.);
#4703=EDGE_CURVE('',#3733,#3732,#3205,.T.);
#4704=EDGE_CURVE('',#3767,#3756,#268,.T.);
#4705=EDGE_CURVE('',#3757,#3758,#269,.T.);
#4706=EDGE_CURVE('',#3768,#3769,#270,.T.);
#4707=EDGE_CURVE('',#3751,#3768,#271,.T.);
#4708=EDGE_CURVE('',#3769,#3750,#974,.T.);
#4709=EDGE_CURVE('',#3619,#3770,#99,.T.);
#4710=EDGE_CURVE('',#3615,#3618,#100,.T.);
#4711=EDGE_CURVE('',#3611,#3614,#101,.T.);
#4712=EDGE_CURVE('',#3610,#3609,#975,.T.);
#4713=EDGE_CURVE('',#3722,#3563,#976,.T.);
#4714=EDGE_CURVE('',#3771,#3739,#102,.T.);
#4715=EDGE_CURVE('',#3648,#3771,#272,.T.);
#4716=EDGE_CURVE('',#3772,#3646,#273,.T.);
#4717=EDGE_CURVE('',#3773,#3772,#103,.T.);
#4718=EDGE_CURVE('',#3644,#3773,#274,.T.);
#4719=EDGE_CURVE('',#3774,#3642,#275,.T.);
#4720=EDGE_CURVE('',#3775,#3774,#104,.T.);
#4721=EDGE_CURVE('',#3640,#3775,#276,.T.);
#4722=EDGE_CURVE('',#3776,#3638,#277,.T.);
#4723=EDGE_CURVE('',#3777,#3776,#105,.T.);
#4724=EDGE_CURVE('',#3636,#3777,#278,.T.);
#4725=EDGE_CURVE('',#3778,#3634,#279,.T.);
#4726=EDGE_CURVE('',#3779,#3778,#106,.T.);
#4727=EDGE_CURVE('',#3632,#3779,#280,.T.);
#4728=EDGE_CURVE('',#3780,#3630,#281,.T.);
#4729=EDGE_CURVE('',#3781,#3780,#107,.T.);
#4730=EDGE_CURVE('',#3628,#3781,#282,.T.);
#4731=EDGE_CURVE('',#3782,#3626,#283,.T.);
#4732=EDGE_CURVE('',#3783,#3782,#108,.T.);
#4733=EDGE_CURVE('',#3624,#3783,#284,.T.);
#4734=EDGE_CURVE('',#3784,#3622,#285,.T.);
#4735=EDGE_CURVE('',#3785,#3784,#977,.T.);
#4736=EDGE_CURVE('',#3770,#3785,#978,.T.);
#4737=EDGE_CURVE('',#3649,#3737,#286,.T.);
#4738=EDGE_CURVE('',#3768,#3647,#287,.T.);
#4739=EDGE_CURVE('',#3749,#3769,#288,.T.);
#4740=EDGE_CURVE('',#3577,#3786,#3206,.T.);
#4741=EDGE_CURVE('',#3786,#3787,#3207,.T.);
#4742=EDGE_CURVE('',#3787,#3728,#3208,.T.);
#4743=EDGE_CURVE('',#3573,#3578,#979,.T.);
#4744=EDGE_CURVE('',#3788,#3789,#980,.T.);
#4745=EDGE_CURVE('',#3788,#3790,#289,.T.);
#4746=EDGE_CURVE('',#3790,#3791,#290,.T.);
#4747=EDGE_CURVE('',#3791,#3571,#291,.T.);
#4748=EDGE_CURVE('',#3569,#3792,#292,.T.);
#4749=EDGE_CURVE('',#3792,#3793,#293,.T.);
#4750=EDGE_CURVE('',#3793,#3789,#294,.T.);
#4751=EDGE_CURVE('',#3794,#3795,#981,.T.);
#4752=EDGE_CURVE('',#3795,#3788,#295,.T.);
#4753=EDGE_CURVE('',#3789,#3796,#296,.T.);
#4754=EDGE_CURVE('',#3797,#3796,#982,.T.);
#4755=EDGE_CURVE('',#3794,#3797,#983,.T.);
#4756=EDGE_CURVE('',#3798,#3799,#984,.T.);
#4757=EDGE_CURVE('',#3799,#3794,#985,.T.);
#4758=EDGE_CURVE('',#3798,#3797,#986,.T.);
#4759=EDGE_CURVE('',#3800,#3801,#3209,.T.);
#4760=EDGE_CURVE('',#3800,#3802,#297,.T.);
#4761=EDGE_CURVE('',#3802,#3803,#298,.T.);
#4762=EDGE_CURVE('',#3803,#3804,#3210,.T.);
#4763=EDGE_CURVE('',#3804,#3805,#987,.T.);
#4764=EDGE_CURVE('',#3805,#3806,#3211,.T.);
#4765=EDGE_CURVE('',#3806,#3807,#299,.T.);
#4766=EDGE_CURVE('',#3807,#3808,#300,.T.);
#4767=EDGE_CURVE('',#3808,#3809,#3212,.T.);
#4768=EDGE_CURVE('',#3801,#3809,#988,.T.);
#4769=EDGE_CURVE('',#3808,#3586,#301,.T.);
#4770=EDGE_CURVE('',#3810,#3585,#989,.T.);
#4771=EDGE_CURVE('',#3810,#3811,#3213,.T.);
#4772=EDGE_CURVE('',#3811,#3795,#302,.T.);
#4773=EDGE_CURVE('',#3812,#3799,#990,.T.);
#4774=EDGE_CURVE('',#3813,#3812,#991,.T.);
#4775=EDGE_CURVE('',#3814,#3813,#992,.T.);
#4776=EDGE_CURVE('',#3815,#3814,#993,.T.);
#4777=EDGE_CURVE('',#3816,#3815,#994,.T.);
#4778=EDGE_CURVE('',#3817,#3816,#995,.T.);
#4779=EDGE_CURVE('',#3818,#3817,#996,.T.);
#4780=EDGE_CURVE('',#3819,#3818,#997,.T.);
#4781=EDGE_CURVE('',#3820,#3819,#998,.T.);
#4782=EDGE_CURVE('',#3821,#3820,#999,.T.);
#4783=EDGE_CURVE('',#3822,#3821,#1000,.T.);
#4784=EDGE_CURVE('',#3823,#3822,#1001,.T.);
#4785=EDGE_CURVE('',#3824,#3823,#1002,.T.);
#4786=EDGE_CURVE('',#3825,#3824,#1003,.T.);
#4787=EDGE_CURVE('',#3826,#3825,#1004,.T.);
#4788=EDGE_CURVE('',#3827,#3826,#1005,.T.);
#4789=EDGE_CURVE('',#3828,#3827,#1006,.T.);
#4790=EDGE_CURVE('',#3829,#3828,#1007,.T.);
#4791=EDGE_CURVE('',#3809,#3829,#1008,.T.);
#4792=EDGE_CURVE('',#3576,#3830,#1009,.T.);
#4793=EDGE_CURVE('',#3830,#3810,#1010,.T.);
#4794=EDGE_CURVE('',#3831,#3832,#1011,.T.);
#4795=EDGE_CURVE('',#3832,#3582,#1012,.T.);
#4796=EDGE_CURVE('',#3831,#3583,#1013,.T.);
#4797=EDGE_CURVE('',#3584,#3800,#303,.T.);
#4798=EDGE_CURVE('',#3801,#3833,#1014,.T.);
#4799=EDGE_CURVE('',#3833,#3834,#1015,.T.);
#4800=EDGE_CURVE('',#3834,#3835,#1016,.T.);
#4801=EDGE_CURVE('',#3835,#3836,#1017,.T.);
#4802=EDGE_CURVE('',#3836,#3837,#1018,.T.);
#4803=EDGE_CURVE('',#3837,#3838,#1019,.T.);
#4804=EDGE_CURVE('',#3838,#3839,#1020,.T.);
#4805=EDGE_CURVE('',#3839,#3840,#1021,.T.);
#4806=EDGE_CURVE('',#3840,#3841,#1022,.T.);
#4807=EDGE_CURVE('',#3841,#3842,#1023,.T.);
#4808=EDGE_CURVE('',#3842,#3843,#1024,.T.);
#4809=EDGE_CURVE('',#3843,#3844,#1025,.T.);
#4810=EDGE_CURVE('',#3844,#3845,#1026,.T.);
#4811=EDGE_CURVE('',#3845,#3846,#1027,.T.);
#4812=EDGE_CURVE('',#3846,#3847,#1028,.T.);
#4813=EDGE_CURVE('',#3847,#3848,#1029,.T.);
#4814=EDGE_CURVE('',#3848,#3849,#1030,.T.);
#4815=EDGE_CURVE('',#3849,#3850,#1031,.T.);
#4816=EDGE_CURVE('',#3850,#3798,#1032,.T.);
#4817=EDGE_CURVE('',#3796,#3851,#304,.T.);
#4818=EDGE_CURVE('',#3851,#3831,#3214,.T.);
#4819=EDGE_CURVE('',#3851,#3852,#305,.T.);
#4820=EDGE_CURVE('',#3852,#3832,#3215,.T.);
#4821=EDGE_CURVE('',#3830,#3853,#3216,.T.);
#4822=EDGE_CURVE('',#3853,#3811,#306,.T.);
#4823=EDGE_CURVE('',#3850,#3812,#1033,.T.);
#4824=EDGE_CURVE('',#3849,#3813,#1034,.T.);
#4825=EDGE_CURVE('',#3848,#3814,#1035,.T.);
#4826=EDGE_CURVE('',#3847,#3815,#1036,.T.);
#4827=EDGE_CURVE('',#3846,#3816,#1037,.T.);
#4828=EDGE_CURVE('',#3845,#3817,#1038,.T.);
#4829=EDGE_CURVE('',#3844,#3818,#1039,.T.);
#4830=EDGE_CURVE('',#3843,#3819,#1040,.T.);
#4831=EDGE_CURVE('',#3842,#3820,#1041,.T.);
#4832=EDGE_CURVE('',#3841,#3821,#1042,.T.);
#4833=EDGE_CURVE('',#3840,#3822,#1043,.T.);
#4834=EDGE_CURVE('',#3839,#3823,#1044,.T.);
#4835=EDGE_CURVE('',#3838,#3824,#1045,.T.);
#4836=EDGE_CURVE('',#3837,#3825,#1046,.T.);
#4837=EDGE_CURVE('',#3836,#3826,#1047,.T.);
#4838=EDGE_CURVE('',#3835,#3827,#1048,.T.);
#4839=EDGE_CURVE('',#3834,#3828,#1049,.T.);
#4840=EDGE_CURVE('',#3833,#3829,#1050,.T.);
#4841=EDGE_CURVE('',#3854,#3832,#3217,.T.);
#4842=EDGE_CURVE('',#3854,#3567,#109,.T.);
#4843=EDGE_CURVE('',#3852,#3854,#307,.T.);
#4844=EDGE_CURVE('',#3573,#3855,#110,.T.);
#4845=EDGE_CURVE('',#3830,#3855,#3218,.T.);
#4846=EDGE_CURVE('',#3855,#3853,#308,.T.);
#4847=EDGE_CURVE('',#3855,#3791,#3219,.T.);
#4848=EDGE_CURVE('',#3853,#3790,#3220,.T.);
#4849=EDGE_CURVE('',#3792,#3854,#3221,.T.);
#4850=EDGE_CURVE('',#3793,#3852,#3222,.T.);
#4851=EDGE_CURVE('',#3785,#3856,#3223,.T.);
#4852=EDGE_CURVE('',#3856,#3770,#72,.T.);
#4853=EDGE_CURVE('',#3784,#3856,#309,.T.);
#4854=EDGE_CURVE('',#3703,#3754,#3224,.T.);
#4855=EDGE_CURVE('',#3704,#3752,#3225,.T.);
#4856=EDGE_CURVE('',#3705,#3598,#3226,.T.);
#4857=EDGE_CURVE('',#3755,#3762,#3227,.T.);
#4858=EDGE_CURVE('',#3753,#3761,#3228,.T.);
#4859=EDGE_CURVE('',#3595,#3760,#3229,.T.);
#4860=EDGE_CURVE('',#3596,#3759,#3230,.T.);
#4861=EDGE_CURVE('',#3729,#3758,#3231,.T.);
#4862=EDGE_CURVE('',#3730,#3757,#3232,.T.);
#4863=EDGE_CURVE('',#3726,#3756,#3233,.T.);
#4864=EDGE_CURVE('',#3727,#3767,#3234,.T.);
#4865=EDGE_CURVE('',#3593,#3766,#3235,.T.);
#4866=EDGE_CURVE('',#3594,#3765,#3236,.T.);
#4867=EDGE_CURVE('',#3731,#3764,#3237,.T.);
#4868=EDGE_CURVE('',#3734,#3763,#3238,.T.);
#4869=EDGE_CURVE('',#3677,#3856,#73,.T.);
#4870=EDGE_CURVE('',#3676,#3620,#74,.T.);
#4871=EDGE_CURVE('',#3600,#3601,#3239,.T.);
#4872=EDGE_CURVE('',#3700,#3773,#75,.T.);
#4873=EDGE_CURVE('',#3748,#3772,#76,.T.);
#4874=EDGE_CURVE('',#3697,#3774,#77,.T.);
#4875=EDGE_CURVE('',#3696,#3775,#78,.T.);
#4876=EDGE_CURVE('',#3693,#3776,#79,.T.);
#4877=EDGE_CURVE('',#3692,#3777,#80,.T.);
#4878=EDGE_CURVE('',#3689,#3778,#81,.T.);
#4879=EDGE_CURVE('',#3688,#3779,#82,.T.);
#4880=EDGE_CURVE('',#3685,#3780,#83,.T.);
#4881=EDGE_CURVE('',#3684,#3781,#84,.T.);
#4882=EDGE_CURVE('',#3681,#3782,#85,.T.);
#4883=EDGE_CURVE('',#3680,#3783,#86,.T.);
#4884=EDGE_CURVE('',#3738,#3771,#87,.T.);
#4885=EDGE_CURVE('',#3804,#3560,#3240,.T.);
#4886=EDGE_CURVE('',#3559,#3805,#3241,.T.);
#4887=EDGE_CURVE('',#3802,#3581,#3242,.T.);
#4888=EDGE_CURVE('',#3803,#3579,#3243,.T.);
#4889=EDGE_CURVE('',#3804,#3725,#3244,.T.);
#4890=EDGE_CURVE('',#3560,#3724,#3245,.T.);
#4891=EDGE_CURVE('',#3559,#3787,#3246,.T.);
#4892=EDGE_CURVE('',#3805,#3786,#3247,.T.);
#4893=EDGE_CURVE('',#3806,#3577,#3248,.T.);
#4894=EDGE_CURVE('',#3807,#3575,#3249,.T.);
#5807=ORIENTED_EDGE('',*,*,#4429,.T.);
#5808=ORIENTED_EDGE('',*,*,#4430,.F.);
#5809=ORIENTED_EDGE('',*,*,#4431,.T.);
#5810=ORIENTED_EDGE('',*,*,#4432,.T.);
#5811=ORIENTED_EDGE('',*,*,#4433,.F.);
#5812=ORIENTED_EDGE('',*,*,#4434,.F.);
#5813=ORIENTED_EDGE('',*,*,#4435,.F.);
#5814=ORIENTED_EDGE('',*,*,#4436,.F.);
#5815=ORIENTED_EDGE('',*,*,#4437,.F.);
#5816=ORIENTED_EDGE('',*,*,#4438,.F.);
#5817=ORIENTED_EDGE('',*,*,#4439,.F.);
#5818=ORIENTED_EDGE('',*,*,#4440,.F.);
#5819=ORIENTED_EDGE('',*,*,#4441,.F.);
#5820=ORIENTED_EDGE('',*,*,#4442,.F.);
#5821=ORIENTED_EDGE('',*,*,#4443,.F.);
#5822=ORIENTED_EDGE('',*,*,#4444,.F.);
#5823=ORIENTED_EDGE('',*,*,#4445,.F.);
#5824=ORIENTED_EDGE('',*,*,#4446,.F.);
#5825=ORIENTED_EDGE('',*,*,#4447,.T.);
#5826=ORIENTED_EDGE('',*,*,#4448,.F.);
#5827=ORIENTED_EDGE('',*,*,#4449,.F.);
#5828=ORIENTED_EDGE('',*,*,#4450,.F.);
#5829=ORIENTED_EDGE('',*,*,#4451,.T.);
#5830=ORIENTED_EDGE('',*,*,#4452,.F.);
#5831=ORIENTED_EDGE('',*,*,#4453,.F.);
#5832=ORIENTED_EDGE('',*,*,#4454,.F.);
#5833=ORIENTED_EDGE('',*,*,#4455,.F.);
#5834=ORIENTED_EDGE('',*,*,#4452,.T.);
#5835=ORIENTED_EDGE('',*,*,#4456,.T.);
#5836=ORIENTED_EDGE('',*,*,#4457,.T.);
#5837=ORIENTED_EDGE('',*,*,#4458,.T.);
#5838=ORIENTED_EDGE('',*,*,#4446,.T.);
#5839=ORIENTED_EDGE('',*,*,#4459,.F.);
#5840=ORIENTED_EDGE('',*,*,#4460,.F.);
#5841=ORIENTED_EDGE('',*,*,#4461,.T.);
#5842=ORIENTED_EDGE('',*,*,#4462,.T.);
#5843=ORIENTED_EDGE('',*,*,#4461,.F.);
#5844=ORIENTED_EDGE('',*,*,#4463,.F.);
#5845=ORIENTED_EDGE('',*,*,#4464,.T.);
#5846=ORIENTED_EDGE('',*,*,#4465,.T.);
#5847=ORIENTED_EDGE('',*,*,#4464,.F.);
#5848=ORIENTED_EDGE('',*,*,#4466,.T.);
#5849=ORIENTED_EDGE('',*,*,#4432,.F.);
#5850=ORIENTED_EDGE('',*,*,#4467,.T.);
#5851=ORIENTED_EDGE('',*,*,#4468,.F.);
#5852=ORIENTED_EDGE('',*,*,#4469,.T.);
#5853=ORIENTED_EDGE('',*,*,#4470,.F.);
#5854=ORIENTED_EDGE('',*,*,#4471,.T.);
#5855=ORIENTED_EDGE('',*,*,#4472,.F.);
#5856=ORIENTED_EDGE('',*,*,#4473,.T.);
#5857=ORIENTED_EDGE('',*,*,#4437,.T.);
#5858=ORIENTED_EDGE('',*,*,#4474,.T.);
#5859=ORIENTED_EDGE('',*,*,#4475,.F.);
#5860=ORIENTED_EDGE('',*,*,#4476,.T.);
#5861=ORIENTED_EDGE('',*,*,#4477,.F.);
#5862=ORIENTED_EDGE('',*,*,#4478,.F.);
#5863=ORIENTED_EDGE('',*,*,#4479,.F.);
#5864=ORIENTED_EDGE('',*,*,#4480,.F.);
#5865=ORIENTED_EDGE('',*,*,#4481,.F.);
#5866=ORIENTED_EDGE('',*,*,#4482,.F.);
#5867=ORIENTED_EDGE('',*,*,#4483,.T.);
#5868=ORIENTED_EDGE('',*,*,#4484,.F.);
#5869=ORIENTED_EDGE('',*,*,#4485,.T.);
#5870=ORIENTED_EDGE('',*,*,#4486,.F.);
#5871=ORIENTED_EDGE('',*,*,#4487,.T.);
#5872=ORIENTED_EDGE('',*,*,#4488,.F.);
#5873=ORIENTED_EDGE('',*,*,#4489,.F.);
#5874=ORIENTED_EDGE('',*,*,#4490,.T.);
#5875=ORIENTED_EDGE('',*,*,#4491,.T.);
#5876=ORIENTED_EDGE('',*,*,#4492,.F.);
#5877=ORIENTED_EDGE('',*,*,#4493,.F.);
#5878=ORIENTED_EDGE('',*,*,#4494,.T.);
#5879=ORIENTED_EDGE('',*,*,#4495,.T.);
#5880=ORIENTED_EDGE('',*,*,#4496,.F.);
#5881=ORIENTED_EDGE('',*,*,#4497,.T.);
#5882=ORIENTED_EDGE('',*,*,#4498,.F.);
#5883=ORIENTED_EDGE('',*,*,#4499,.F.);
#5884=ORIENTED_EDGE('',*,*,#4500,.T.);
#5885=ORIENTED_EDGE('',*,*,#4501,.F.);
#5886=ORIENTED_EDGE('',*,*,#4502,.F.);
#5887=ORIENTED_EDGE('',*,*,#4503,.F.);
#5888=ORIENTED_EDGE('',*,*,#4504,.T.);
#5889=ORIENTED_EDGE('',*,*,#4505,.F.);
#5890=ORIENTED_EDGE('',*,*,#4506,.F.);
#5891=ORIENTED_EDGE('',*,*,#4507,.F.);
#5892=ORIENTED_EDGE('',*,*,#4508,.T.);
#5893=ORIENTED_EDGE('',*,*,#4509,.F.);
#5894=ORIENTED_EDGE('',*,*,#4510,.F.);
#5895=ORIENTED_EDGE('',*,*,#4511,.F.);
#5896=ORIENTED_EDGE('',*,*,#4512,.T.);
#5897=ORIENTED_EDGE('',*,*,#4513,.F.);
#5898=ORIENTED_EDGE('',*,*,#4514,.F.);
#5899=ORIENTED_EDGE('',*,*,#4515,.F.);
#5900=ORIENTED_EDGE('',*,*,#4516,.T.);
#5901=ORIENTED_EDGE('',*,*,#4517,.F.);
#5902=ORIENTED_EDGE('',*,*,#4518,.F.);
#5903=ORIENTED_EDGE('',*,*,#4519,.F.);
#5904=ORIENTED_EDGE('',*,*,#4520,.T.);
#5905=ORIENTED_EDGE('',*,*,#4521,.F.);
#5906=ORIENTED_EDGE('',*,*,#4522,.F.);
#5907=ORIENTED_EDGE('',*,*,#4523,.F.);
#5908=ORIENTED_EDGE('',*,*,#4524,.T.);
#5909=ORIENTED_EDGE('',*,*,#4525,.F.);
#5910=ORIENTED_EDGE('',*,*,#4526,.F.);
#5911=ORIENTED_EDGE('',*,*,#4527,.F.);
#5912=ORIENTED_EDGE('',*,*,#4528,.F.);
#5913=ORIENTED_EDGE('',*,*,#4529,.F.);
#5914=ORIENTED_EDGE('',*,*,#4530,.F.);
#5915=ORIENTED_EDGE('',*,*,#4531,.F.);
#5916=ORIENTED_EDGE('',*,*,#4532,.F.);
#5917=ORIENTED_EDGE('',*,*,#4533,.F.);
#5918=ORIENTED_EDGE('',*,*,#4534,.F.);
#5919=ORIENTED_EDGE('',*,*,#4535,.F.);
#5920=ORIENTED_EDGE('',*,*,#4536,.F.);
#5921=ORIENTED_EDGE('',*,*,#4537,.F.);
#5922=ORIENTED_EDGE('',*,*,#4538,.F.);
#5923=ORIENTED_EDGE('',*,*,#4539,.F.);
#5924=ORIENTED_EDGE('',*,*,#4540,.F.);
#5925=ORIENTED_EDGE('',*,*,#4541,.F.);
#5926=ORIENTED_EDGE('',*,*,#4542,.F.);
#5927=ORIENTED_EDGE('',*,*,#4543,.F.);
#5928=ORIENTED_EDGE('',*,*,#4544,.F.);
#5929=ORIENTED_EDGE('',*,*,#4545,.F.);
#5930=ORIENTED_EDGE('',*,*,#4546,.F.);
#5931=ORIENTED_EDGE('',*,*,#4547,.F.);
#5932=ORIENTED_EDGE('',*,*,#4548,.F.);
#5933=ORIENTED_EDGE('',*,*,#4549,.F.);
#5934=ORIENTED_EDGE('',*,*,#4550,.F.);
#5935=ORIENTED_EDGE('',*,*,#4493,.T.);
#5936=ORIENTED_EDGE('',*,*,#4551,.T.);
#5937=ORIENTED_EDGE('',*,*,#4498,.T.);
#5938=ORIENTED_EDGE('',*,*,#4552,.T.);
#5939=ORIENTED_EDGE('',*,*,#4553,.T.);
#5940=ORIENTED_EDGE('',*,*,#4554,.T.);
#5941=ORIENTED_EDGE('',*,*,#4555,.T.);
#5942=ORIENTED_EDGE('',*,*,#4556,.T.);
#5943=ORIENTED_EDGE('',*,*,#4557,.T.);
#5944=ORIENTED_EDGE('',*,*,#4558,.T.);
#5945=ORIENTED_EDGE('',*,*,#4559,.T.);
#5946=ORIENTED_EDGE('',*,*,#4560,.T.);
#5947=ORIENTED_EDGE('',*,*,#4561,.T.);
#5948=ORIENTED_EDGE('',*,*,#4562,.T.);
#5949=ORIENTED_EDGE('',*,*,#4563,.T.);
#5950=ORIENTED_EDGE('',*,*,#4564,.T.);
#5951=ORIENTED_EDGE('',*,*,#4565,.T.);
#5952=ORIENTED_EDGE('',*,*,#4566,.T.);
#5953=ORIENTED_EDGE('',*,*,#4567,.T.);
#5954=ORIENTED_EDGE('',*,*,#4568,.T.);
#5955=ORIENTED_EDGE('',*,*,#4569,.T.);
#5956=ORIENTED_EDGE('',*,*,#4570,.T.);
#5957=ORIENTED_EDGE('',*,*,#4571,.T.);
#5958=ORIENTED_EDGE('',*,*,#4572,.T.);
#5959=ORIENTED_EDGE('',*,*,#4573,.T.);
#5960=ORIENTED_EDGE('',*,*,#4574,.T.);
#5961=ORIENTED_EDGE('',*,*,#4575,.T.);
#5962=ORIENTED_EDGE('',*,*,#4576,.T.);
#5963=ORIENTED_EDGE('',*,*,#4577,.T.);
#5964=ORIENTED_EDGE('',*,*,#4578,.T.);
#5965=ORIENTED_EDGE('',*,*,#4579,.T.);
#5966=ORIENTED_EDGE('',*,*,#4580,.F.);
#5967=ORIENTED_EDGE('',*,*,#4581,.T.);
#5968=ORIENTED_EDGE('',*,*,#4582,.T.);
#5969=ORIENTED_EDGE('',*,*,#4583,.T.);
#5970=ORIENTED_EDGE('',*,*,#4584,.T.);
#5971=ORIENTED_EDGE('',*,*,#4435,.T.);
#5972=ORIENTED_EDGE('',*,*,#4585,.F.);
#5973=ORIENTED_EDGE('',*,*,#4586,.F.);
#5974=ORIENTED_EDGE('',*,*,#4481,.T.);
#5975=ORIENTED_EDGE('',*,*,#4587,.F.);
#5976=ORIENTED_EDGE('',*,*,#4479,.T.);
#5977=ORIENTED_EDGE('',*,*,#4588,.T.);
#5978=ORIENTED_EDGE('',*,*,#4489,.T.);
#5979=ORIENTED_EDGE('',*,*,#4589,.T.);
#5980=ORIENTED_EDGE('',*,*,#4460,.T.);
#5981=ORIENTED_EDGE('',*,*,#4502,.T.);
#5982=ORIENTED_EDGE('',*,*,#4590,.T.);
#5983=ORIENTED_EDGE('',*,*,#4538,.T.);
#5984=ORIENTED_EDGE('',*,*,#4591,.T.);
#5985=ORIENTED_EDGE('',*,*,#4506,.T.);
#5986=ORIENTED_EDGE('',*,*,#4592,.T.);
#5987=ORIENTED_EDGE('',*,*,#4542,.T.);
#5988=ORIENTED_EDGE('',*,*,#4593,.T.);
#5989=ORIENTED_EDGE('',*,*,#4510,.T.);
#5990=ORIENTED_EDGE('',*,*,#4594,.T.);
#5991=ORIENTED_EDGE('',*,*,#4546,.T.);
#5992=ORIENTED_EDGE('',*,*,#4595,.T.);
#5993=ORIENTED_EDGE('',*,*,#4514,.T.);
#5994=ORIENTED_EDGE('',*,*,#4596,.T.);
#5995=ORIENTED_EDGE('',*,*,#4550,.T.);
#5996=ORIENTED_EDGE('',*,*,#4597,.T.);
#5997=ORIENTED_EDGE('',*,*,#4518,.T.);
#5998=ORIENTED_EDGE('',*,*,#4598,.T.);
#5999=ORIENTED_EDGE('',*,*,#4534,.T.);
#6000=ORIENTED_EDGE('',*,*,#4599,.T.);
#6001=ORIENTED_EDGE('',*,*,#4522,.T.);
#6002=ORIENTED_EDGE('',*,*,#4600,.T.);
#6003=ORIENTED_EDGE('',*,*,#4530,.T.);
#6004=ORIENTED_EDGE('',*,*,#4601,.T.);
#6005=ORIENTED_EDGE('',*,*,#4528,.T.);
#6006=ORIENTED_EDGE('',*,*,#4602,.T.);
#6007=ORIENTED_EDGE('',*,*,#4603,.T.);
#6008=ORIENTED_EDGE('',*,*,#4604,.T.);
#6009=ORIENTED_EDGE('',*,*,#4532,.T.);
#6010=ORIENTED_EDGE('',*,*,#4605,.T.);
#6011=ORIENTED_EDGE('',*,*,#4606,.T.);
#6012=ORIENTED_EDGE('',*,*,#4607,.T.);
#6013=ORIENTED_EDGE('',*,*,#4548,.T.);
#6014=ORIENTED_EDGE('',*,*,#4608,.T.);
#6015=ORIENTED_EDGE('',*,*,#4609,.T.);
#6016=ORIENTED_EDGE('',*,*,#4610,.T.);
#6017=ORIENTED_EDGE('',*,*,#4544,.T.);
#6018=ORIENTED_EDGE('',*,*,#4611,.T.);
#6019=ORIENTED_EDGE('',*,*,#4612,.T.);
#6020=ORIENTED_EDGE('',*,*,#4613,.T.);
#6021=ORIENTED_EDGE('',*,*,#4540,.T.);
#6022=ORIENTED_EDGE('',*,*,#4614,.T.);
#6023=ORIENTED_EDGE('',*,*,#4615,.T.);
#6024=ORIENTED_EDGE('',*,*,#4616,.T.);
#6025=ORIENTED_EDGE('',*,*,#4536,.T.);
#6026=ORIENTED_EDGE('',*,*,#4617,.T.);
#6027=ORIENTED_EDGE('',*,*,#4618,.T.);
#6028=ORIENTED_EDGE('',*,*,#4619,.T.);
#6029=ORIENTED_EDGE('',*,*,#4620,.F.);
#6030=ORIENTED_EDGE('',*,*,#4577,.F.);
#6031=ORIENTED_EDGE('',*,*,#4621,.F.);
#6032=ORIENTED_EDGE('',*,*,#4603,.F.);
#6033=ORIENTED_EDGE('',*,*,#4622,.F.);
#6034=ORIENTED_EDGE('',*,*,#4573,.F.);
#6035=ORIENTED_EDGE('',*,*,#4623,.F.);
#6036=ORIENTED_EDGE('',*,*,#4606,.F.);
#6037=ORIENTED_EDGE('',*,*,#4624,.F.);
#6038=ORIENTED_EDGE('',*,*,#4569,.F.);
#6039=ORIENTED_EDGE('',*,*,#4625,.F.);
#6040=ORIENTED_EDGE('',*,*,#4609,.F.);
#6041=ORIENTED_EDGE('',*,*,#4626,.F.);
#6042=ORIENTED_EDGE('',*,*,#4565,.F.);
#6043=ORIENTED_EDGE('',*,*,#4627,.F.);
#6044=ORIENTED_EDGE('',*,*,#4612,.F.);
#6045=ORIENTED_EDGE('',*,*,#4628,.F.);
#6046=ORIENTED_EDGE('',*,*,#4561,.F.);
#6047=ORIENTED_EDGE('',*,*,#4629,.F.);
#6048=ORIENTED_EDGE('',*,*,#4615,.F.);
#6049=ORIENTED_EDGE('',*,*,#4630,.F.);
#6050=ORIENTED_EDGE('',*,*,#4557,.F.);
#6051=ORIENTED_EDGE('',*,*,#4631,.F.);
#6052=ORIENTED_EDGE('',*,*,#4618,.F.);
#6053=ORIENTED_EDGE('',*,*,#4632,.F.);
#6054=ORIENTED_EDGE('',*,*,#4553,.F.);
#6055=ORIENTED_EDGE('',*,*,#4633,.F.);
#6056=ORIENTED_EDGE('',*,*,#4497,.F.);
#6057=ORIENTED_EDGE('',*,*,#4634,.T.);
#6058=ORIENTED_EDGE('',*,*,#4633,.T.);
#6059=ORIENTED_EDGE('',*,*,#4552,.F.);
#6060=ORIENTED_EDGE('',*,*,#4483,.F.);
#6061=ORIENTED_EDGE('',*,*,#4635,.F.);
#6062=ORIENTED_EDGE('',*,*,#4636,.T.);
#6063=ORIENTED_EDGE('',*,*,#4637,.F.);
#6064=ORIENTED_EDGE('',*,*,#4638,.T.);
#6065=ORIENTED_EDGE('',*,*,#4484,.T.);
#6066=ORIENTED_EDGE('',*,*,#4637,.T.);
#6067=ORIENTED_EDGE('',*,*,#4639,.T.);
#6068=ORIENTED_EDGE('',*,*,#4635,.T.);
#6069=ORIENTED_EDGE('',*,*,#4482,.T.);
#6070=ORIENTED_EDGE('',*,*,#4586,.T.);
#6071=ORIENTED_EDGE('',*,*,#4640,.T.);
#6072=ORIENTED_EDGE('',*,*,#4641,.T.);
#6073=ORIENTED_EDGE('',*,*,#4642,.T.);
#6074=ORIENTED_EDGE('',*,*,#4643,.T.);
#6075=ORIENTED_EDGE('',*,*,#4644,.T.);
#6076=ORIENTED_EDGE('',*,*,#4450,.T.);
#6077=ORIENTED_EDGE('',*,*,#4645,.T.);
#6078=ORIENTED_EDGE('',*,*,#4438,.T.);
#6079=ORIENTED_EDGE('',*,*,#4646,.T.);
#6080=ORIENTED_EDGE('',*,*,#4647,.T.);
#6081=ORIENTED_EDGE('',*,*,#4468,.T.);
#6082=ORIENTED_EDGE('',*,*,#4648,.T.);
#6083=ORIENTED_EDGE('',*,*,#4641,.F.);
#6084=ORIENTED_EDGE('',*,*,#4441,.T.);
#6085=ORIENTED_EDGE('',*,*,#4649,.F.);
#6086=ORIENTED_EDGE('',*,*,#4445,.T.);
#6087=ORIENTED_EDGE('',*,*,#4650,.T.);
#6088=ORIENTED_EDGE('',*,*,#4651,.T.);
#6089=ORIENTED_EDGE('',*,*,#4472,.T.);
#6090=ORIENTED_EDGE('',*,*,#4652,.T.);
#6091=ORIENTED_EDGE('',*,*,#4653,.T.);
#6092=ORIENTED_EDGE('',*,*,#4654,.T.);
#6093=ORIENTED_EDGE('',*,*,#4470,.T.);
#6094=ORIENTED_EDGE('',*,*,#4655,.T.);
#6095=ORIENTED_EDGE('',*,*,#4656,.T.);
#6096=ORIENTED_EDGE('',*,*,#4657,.F.);
#6097=ORIENTED_EDGE('',*,*,#4658,.T.);
#6098=ORIENTED_EDGE('',*,*,#4659,.T.);
#6099=ORIENTED_EDGE('',*,*,#4660,.F.);
#6100=ORIENTED_EDGE('',*,*,#4661,.F.);
#6101=ORIENTED_EDGE('',*,*,#4662,.T.);
#6102=ORIENTED_EDGE('',*,*,#4663,.T.);
#6103=ORIENTED_EDGE('',*,*,#4664,.F.);
#6104=ORIENTED_EDGE('',*,*,#4660,.T.);
#6105=ORIENTED_EDGE('',*,*,#4665,.T.);
#6106=ORIENTED_EDGE('',*,*,#4666,.T.);
#6107=ORIENTED_EDGE('',*,*,#4667,.T.);
#6108=ORIENTED_EDGE('',*,*,#4668,.F.);
#6109=ORIENTED_EDGE('',*,*,#4669,.T.);
#6110=ORIENTED_EDGE('',*,*,#4670,.F.);
#6111=ORIENTED_EDGE('',*,*,#4671,.T.);
#6112=ORIENTED_EDGE('',*,*,#4672,.T.);
#6113=ORIENTED_EDGE('',*,*,#4673,.T.);
#6114=ORIENTED_EDGE('',*,*,#4580,.T.);
#6115=ORIENTED_EDGE('',*,*,#4674,.T.);
#6116=ORIENTED_EDGE('',*,*,#4675,.T.);
#6117=ORIENTED_EDGE('',*,*,#4676,.F.);
#6118=ORIENTED_EDGE('',*,*,#4677,.T.);
#6119=ORIENTED_EDGE('',*,*,#4678,.F.);
#6120=ORIENTED_EDGE('',*,*,#4679,.F.);
#6121=ORIENTED_EDGE('',*,*,#4680,.T.);
#6122=ORIENTED_EDGE('',*,*,#4681,.F.);
#6123=ORIENTED_EDGE('',*,*,#4682,.T.);
#6124=ORIENTED_EDGE('',*,*,#4683,.T.);
#6125=ORIENTED_EDGE('',*,*,#4684,.T.);
#6126=ORIENTED_EDGE('',*,*,#4685,.T.);
#6127=ORIENTED_EDGE('',*,*,#4668,.T.);
#6128=ORIENTED_EDGE('',*,*,#4475,.T.);
#6129=ORIENTED_EDGE('',*,*,#4686,.T.);
#6130=ORIENTED_EDGE('',*,*,#4679,.T.);
#6131=ORIENTED_EDGE('',*,*,#4687,.T.);
#6132=ORIENTED_EDGE('',*,*,#4681,.T.);
#6133=ORIENTED_EDGE('',*,*,#4688,.T.);
#6134=ORIENTED_EDGE('',*,*,#4672,.F.);
#6135=ORIENTED_EDGE('',*,*,#4689,.T.);
#6136=ORIENTED_EDGE('',*,*,#4690,.T.);
#6137=ORIENTED_EDGE('',*,*,#4691,.T.);
#6138=ORIENTED_EDGE('',*,*,#4692,.T.);
#6139=ORIENTED_EDGE('',*,*,#4693,.T.);
#6140=ORIENTED_EDGE('',*,*,#4694,.T.);
#6141=ORIENTED_EDGE('',*,*,#4695,.T.);
#6142=ORIENTED_EDGE('',*,*,#4670,.T.);
#6143=ORIENTED_EDGE('',*,*,#4462,.F.);
#6144=ORIENTED_EDGE('',*,*,#4666,.F.);
#6145=ORIENTED_EDGE('',*,*,#4696,.T.);
#6146=ORIENTED_EDGE('',*,*,#4697,.T.);
#6147=ORIENTED_EDGE('',*,*,#4698,.T.);
#6148=ORIENTED_EDGE('',*,*,#4699,.T.);
#6149=ORIENTED_EDGE('',*,*,#4700,.T.);
#6150=ORIENTED_EDGE('',*,*,#4701,.T.);
#6151=ORIENTED_EDGE('',*,*,#4463,.T.);
#6152=ORIENTED_EDGE('',*,*,#4656,.F.);
#6153=ORIENTED_EDGE('',*,*,#4702,.T.);
#6154=ORIENTED_EDGE('',*,*,#4658,.F.);
#6155=ORIENTED_EDGE('',*,*,#4703,.T.);
#6156=ORIENTED_EDGE('',*,*,#4701,.F.);
#6157=ORIENTED_EDGE('',*,*,#4704,.T.);
#6158=ORIENTED_EDGE('',*,*,#4683,.F.);
#6159=ORIENTED_EDGE('',*,*,#4667,.F.);
#6160=ORIENTED_EDGE('',*,*,#4685,.F.);
#6161=ORIENTED_EDGE('',*,*,#4705,.T.);
#6162=ORIENTED_EDGE('',*,*,#4690,.F.);
#6163=ORIENTED_EDGE('',*,*,#4669,.F.);
#6164=ORIENTED_EDGE('',*,*,#4706,.F.);
#6165=ORIENTED_EDGE('',*,*,#4707,.F.);
#6166=ORIENTED_EDGE('',*,*,#4677,.F.);
#6167=ORIENTED_EDGE('',*,*,#4708,.F.);
#6168=ORIENTED_EDGE('',*,*,#4709,.F.);
#6169=ORIENTED_EDGE('',*,*,#4495,.F.);
#6170=ORIENTED_EDGE('',*,*,#4710,.F.);
#6171=ORIENTED_EDGE('',*,*,#4491,.F.);
#6172=ORIENTED_EDGE('',*,*,#4711,.F.);
#6173=ORIENTED_EDGE('',*,*,#4487,.F.);
#6174=ORIENTED_EDGE('',*,*,#4712,.T.);
#6175=ORIENTED_EDGE('',*,*,#4485,.F.);
#6176=ORIENTED_EDGE('',*,*,#4638,.F.);
#6177=ORIENTED_EDGE('',*,*,#4713,.T.);
#6178=ORIENTED_EDGE('',*,*,#4433,.T.);
#6179=ORIENTED_EDGE('',*,*,#4466,.F.);
#6180=ORIENTED_EDGE('',*,*,#4657,.T.);
#6181=ORIENTED_EDGE('',*,*,#4703,.F.);
#6182=ORIENTED_EDGE('',*,*,#4661,.T.);
#6183=ORIENTED_EDGE('',*,*,#4664,.T.);
#6184=ORIENTED_EDGE('',*,*,#4714,.F.);
#6185=ORIENTED_EDGE('',*,*,#4715,.F.);
#6186=ORIENTED_EDGE('',*,*,#4524,.F.);
#6187=ORIENTED_EDGE('',*,*,#4716,.F.);
#6188=ORIENTED_EDGE('',*,*,#4717,.F.);
#6189=ORIENTED_EDGE('',*,*,#4718,.F.);
#6190=ORIENTED_EDGE('',*,*,#4520,.F.);
#6191=ORIENTED_EDGE('',*,*,#4719,.F.);
#6192=ORIENTED_EDGE('',*,*,#4720,.F.);
#6193=ORIENTED_EDGE('',*,*,#4721,.F.);
#6194=ORIENTED_EDGE('',*,*,#4516,.F.);
#6195=ORIENTED_EDGE('',*,*,#4722,.F.);
#6196=ORIENTED_EDGE('',*,*,#4723,.F.);
#6197=ORIENTED_EDGE('',*,*,#4724,.F.);
#6198=ORIENTED_EDGE('',*,*,#4512,.F.);
#6199=ORIENTED_EDGE('',*,*,#4725,.F.);
#6200=ORIENTED_EDGE('',*,*,#4726,.F.);
#6201=ORIENTED_EDGE('',*,*,#4727,.F.);
#6202=ORIENTED_EDGE('',*,*,#4508,.F.);
#6203=ORIENTED_EDGE('',*,*,#4728,.F.);
#6204=ORIENTED_EDGE('',*,*,#4729,.F.);
#6205=ORIENTED_EDGE('',*,*,#4730,.F.);
#6206=ORIENTED_EDGE('',*,*,#4504,.F.);
#6207=ORIENTED_EDGE('',*,*,#4731,.F.);
#6208=ORIENTED_EDGE('',*,*,#4732,.F.);
#6209=ORIENTED_EDGE('',*,*,#4733,.F.);
#6210=ORIENTED_EDGE('',*,*,#4500,.F.);
#6211=ORIENTED_EDGE('',*,*,#4734,.F.);
#6212=ORIENTED_EDGE('',*,*,#4735,.F.);
#6213=ORIENTED_EDGE('',*,*,#4736,.F.);
#6214=ORIENTED_EDGE('',*,*,#4465,.F.);
#6215=ORIENTED_EDGE('',*,*,#4526,.T.);
#6216=ORIENTED_EDGE('',*,*,#4737,.T.);
#6217=ORIENTED_EDGE('',*,*,#4678,.T.);
#6218=ORIENTED_EDGE('',*,*,#4707,.T.);
#6219=ORIENTED_EDGE('',*,*,#4738,.T.);
#6220=ORIENTED_EDGE('',*,*,#4676,.T.);
#6221=ORIENTED_EDGE('',*,*,#4739,.T.);
#6222=ORIENTED_EDGE('',*,*,#4708,.T.);
#6223=ORIENTED_EDGE('',*,*,#4585,.T.);
#6224=ORIENTED_EDGE('',*,*,#4434,.T.);
#6225=ORIENTED_EDGE('',*,*,#4713,.F.);
#6226=ORIENTED_EDGE('',*,*,#4639,.F.);
#6227=ORIENTED_EDGE('',*,*,#4636,.F.);
#6228=ORIENTED_EDGE('',*,*,#4640,.F.);
#6229=ORIENTED_EDGE('',*,*,#4448,.T.);
#6230=ORIENTED_EDGE('',*,*,#4740,.T.);
#6231=ORIENTED_EDGE('',*,*,#4741,.T.);
#6232=ORIENTED_EDGE('',*,*,#4742,.T.);
#6233=ORIENTED_EDGE('',*,*,#4650,.F.);
#6234=ORIENTED_EDGE('',*,*,#4444,.T.);
#6235=ORIENTED_EDGE('',*,*,#4743,.T.);
#6236=ORIENTED_EDGE('',*,*,#4744,.F.);
#6237=ORIENTED_EDGE('',*,*,#4745,.T.);
#6238=ORIENTED_EDGE('',*,*,#4746,.T.);
#6239=ORIENTED_EDGE('',*,*,#4747,.T.);
#6240=ORIENTED_EDGE('',*,*,#4442,.T.);
#6241=ORIENTED_EDGE('',*,*,#4649,.T.);
#6242=ORIENTED_EDGE('',*,*,#4440,.T.);
#6243=ORIENTED_EDGE('',*,*,#4748,.T.);
#6244=ORIENTED_EDGE('',*,*,#4749,.T.);
#6245=ORIENTED_EDGE('',*,*,#4750,.T.);
#6246=ORIENTED_EDGE('',*,*,#4751,.T.);
#6247=ORIENTED_EDGE('',*,*,#4752,.T.);
#6248=ORIENTED_EDGE('',*,*,#4744,.T.);
#6249=ORIENTED_EDGE('',*,*,#4753,.T.);
#6250=ORIENTED_EDGE('',*,*,#4754,.F.);
#6251=ORIENTED_EDGE('',*,*,#4755,.F.);
#6252=ORIENTED_EDGE('',*,*,#4756,.T.);
#6253=ORIENTED_EDGE('',*,*,#4757,.T.);
#6254=ORIENTED_EDGE('',*,*,#4755,.T.);
#6255=ORIENTED_EDGE('',*,*,#4758,.F.);
#6256=ORIENTED_EDGE('',*,*,#4759,.F.);
#6257=ORIENTED_EDGE('',*,*,#4760,.T.);
#6258=ORIENTED_EDGE('',*,*,#4761,.T.);
#6259=ORIENTED_EDGE('',*,*,#4762,.T.);
#6260=ORIENTED_EDGE('',*,*,#4763,.T.);
#6261=ORIENTED_EDGE('',*,*,#4764,.T.);
#6262=ORIENTED_EDGE('',*,*,#4765,.T.);
#6263=ORIENTED_EDGE('',*,*,#4766,.T.);
#6264=ORIENTED_EDGE('',*,*,#4767,.T.);
#6265=ORIENTED_EDGE('',*,*,#4768,.F.);
#6266=ORIENTED_EDGE('',*,*,#4767,.F.);
#6267=ORIENTED_EDGE('',*,*,#4769,.T.);
#6268=ORIENTED_EDGE('',*,*,#4457,.F.);
#6269=ORIENTED_EDGE('',*,*,#4770,.F.);
#6270=ORIENTED_EDGE('',*,*,#4771,.T.);
#6271=ORIENTED_EDGE('',*,*,#4772,.T.);
#6272=ORIENTED_EDGE('',*,*,#4751,.F.);
#6273=ORIENTED_EDGE('',*,*,#4757,.F.);
#6274=ORIENTED_EDGE('',*,*,#4773,.F.);
#6275=ORIENTED_EDGE('',*,*,#4774,.F.);
#6276=ORIENTED_EDGE('',*,*,#4775,.F.);
#6277=ORIENTED_EDGE('',*,*,#4776,.F.);
#6278=ORIENTED_EDGE('',*,*,#4777,.F.);
#6279=ORIENTED_EDGE('',*,*,#4778,.F.);
#6280=ORIENTED_EDGE('',*,*,#4779,.F.);
#6281=ORIENTED_EDGE('',*,*,#4780,.F.);
#6282=ORIENTED_EDGE('',*,*,#4781,.F.);
#6283=ORIENTED_EDGE('',*,*,#4782,.F.);
#6284=ORIENTED_EDGE('',*,*,#4783,.F.);
#6285=ORIENTED_EDGE('',*,*,#4784,.F.);
#6286=ORIENTED_EDGE('',*,*,#4785,.F.);
#6287=ORIENTED_EDGE('',*,*,#4786,.F.);
#6288=ORIENTED_EDGE('',*,*,#4787,.F.);
#6289=ORIENTED_EDGE('',*,*,#4788,.F.);
#6290=ORIENTED_EDGE('',*,*,#4789,.F.);
#6291=ORIENTED_EDGE('',*,*,#4790,.F.);
#6292=ORIENTED_EDGE('',*,*,#4791,.F.);
#6293=ORIENTED_EDGE('',*,*,#4459,.T.);
#6294=ORIENTED_EDGE('',*,*,#4792,.T.);
#6295=ORIENTED_EDGE('',*,*,#4793,.T.);
#6296=ORIENTED_EDGE('',*,*,#4770,.T.);
#6297=ORIENTED_EDGE('',*,*,#4794,.T.);
#6298=ORIENTED_EDGE('',*,*,#4795,.T.);
#6299=ORIENTED_EDGE('',*,*,#4455,.T.);
#6300=ORIENTED_EDGE('',*,*,#4796,.F.);
#6301=ORIENTED_EDGE('',*,*,#4454,.T.);
#6302=ORIENTED_EDGE('',*,*,#4797,.T.);
#6303=ORIENTED_EDGE('',*,*,#4759,.T.);
#6304=ORIENTED_EDGE('',*,*,#4798,.T.);
#6305=ORIENTED_EDGE('',*,*,#4799,.T.);
#6306=ORIENTED_EDGE('',*,*,#4800,.T.);
#6307=ORIENTED_EDGE('',*,*,#4801,.T.);
#6308=ORIENTED_EDGE('',*,*,#4802,.T.);
#6309=ORIENTED_EDGE('',*,*,#4803,.T.);
#6310=ORIENTED_EDGE('',*,*,#4804,.T.);
#6311=ORIENTED_EDGE('',*,*,#4805,.T.);
#6312=ORIENTED_EDGE('',*,*,#4806,.T.);
#6313=ORIENTED_EDGE('',*,*,#4807,.T.);
#6314=ORIENTED_EDGE('',*,*,#4808,.T.);
#6315=ORIENTED_EDGE('',*,*,#4809,.T.);
#6316=ORIENTED_EDGE('',*,*,#4810,.T.);
#6317=ORIENTED_EDGE('',*,*,#4811,.T.);
#6318=ORIENTED_EDGE('',*,*,#4812,.T.);
#6319=ORIENTED_EDGE('',*,*,#4813,.T.);
#6320=ORIENTED_EDGE('',*,*,#4814,.T.);
#6321=ORIENTED_EDGE('',*,*,#4815,.T.);
#6322=ORIENTED_EDGE('',*,*,#4816,.T.);
#6323=ORIENTED_EDGE('',*,*,#4758,.T.);
#6324=ORIENTED_EDGE('',*,*,#4754,.T.);
#6325=ORIENTED_EDGE('',*,*,#4817,.T.);
#6326=ORIENTED_EDGE('',*,*,#4818,.T.);
#6327=ORIENTED_EDGE('',*,*,#4796,.T.);
#6328=ORIENTED_EDGE('',*,*,#4818,.F.);
#6329=ORIENTED_EDGE('',*,*,#4819,.T.);
#6330=ORIENTED_EDGE('',*,*,#4820,.T.);
#6331=ORIENTED_EDGE('',*,*,#4794,.F.);
#6332=ORIENTED_EDGE('',*,*,#4821,.T.);
#6333=ORIENTED_EDGE('',*,*,#4822,.T.);
#6334=ORIENTED_EDGE('',*,*,#4771,.F.);
#6335=ORIENTED_EDGE('',*,*,#4793,.F.);
#6336=ORIENTED_EDGE('',*,*,#4773,.T.);
#6337=ORIENTED_EDGE('',*,*,#4756,.F.);
#6338=ORIENTED_EDGE('',*,*,#4816,.F.);
#6339=ORIENTED_EDGE('',*,*,#4823,.T.);
#6340=ORIENTED_EDGE('',*,*,#4774,.T.);
#6341=ORIENTED_EDGE('',*,*,#4823,.F.);
#6342=ORIENTED_EDGE('',*,*,#4815,.F.);
#6343=ORIENTED_EDGE('',*,*,#4824,.T.);
#6344=ORIENTED_EDGE('',*,*,#4775,.T.);
#6345=ORIENTED_EDGE('',*,*,#4824,.F.);
#6346=ORIENTED_EDGE('',*,*,#4814,.F.);
#6347=ORIENTED_EDGE('',*,*,#4825,.T.);
#6348=ORIENTED_EDGE('',*,*,#4776,.T.);
#6349=ORIENTED_EDGE('',*,*,#4825,.F.);
#6350=ORIENTED_EDGE('',*,*,#4813,.F.);
#6351=ORIENTED_EDGE('',*,*,#4826,.T.);
#6352=ORIENTED_EDGE('',*,*,#4777,.T.);
#6353=ORIENTED_EDGE('',*,*,#4826,.F.);
#6354=ORIENTED_EDGE('',*,*,#4812,.F.);
#6355=ORIENTED_EDGE('',*,*,#4827,.T.);
#6356=ORIENTED_EDGE('',*,*,#4778,.T.);
#6357=ORIENTED_EDGE('',*,*,#4827,.F.);
#6358=ORIENTED_EDGE('',*,*,#4811,.F.);
#6359=ORIENTED_EDGE('',*,*,#4828,.T.);
#6360=ORIENTED_EDGE('',*,*,#4779,.T.);
#6361=ORIENTED_EDGE('',*,*,#4828,.F.);
#6362=ORIENTED_EDGE('',*,*,#4810,.F.);
#6363=ORIENTED_EDGE('',*,*,#4829,.T.);
#6364=ORIENTED_EDGE('',*,*,#4780,.T.);
#6365=ORIENTED_EDGE('',*,*,#4829,.F.);
#6366=ORIENTED_EDGE('',*,*,#4809,.F.);
#6367=ORIENTED_EDGE('',*,*,#4830,.T.);
#6368=ORIENTED_EDGE('',*,*,#4781,.T.);
#6369=ORIENTED_EDGE('',*,*,#4830,.F.);
#6370=ORIENTED_EDGE('',*,*,#4808,.F.);
#6371=ORIENTED_EDGE('',*,*,#4831,.T.);
#6372=ORIENTED_EDGE('',*,*,#4782,.T.);
#6373=ORIENTED_EDGE('',*,*,#4831,.F.);
#6374=ORIENTED_EDGE('',*,*,#4807,.F.);
#6375=ORIENTED_EDGE('',*,*,#4832,.T.);
#6376=ORIENTED_EDGE('',*,*,#4783,.T.);
#6377=ORIENTED_EDGE('',*,*,#4832,.F.);
#6378=ORIENTED_EDGE('',*,*,#4806,.F.);
#6379=ORIENTED_EDGE('',*,*,#4833,.T.);
#6380=ORIENTED_EDGE('',*,*,#4784,.T.);
#6381=ORIENTED_EDGE('',*,*,#4833,.F.);
#6382=ORIENTED_EDGE('',*,*,#4805,.F.);
#6383=ORIENTED_EDGE('',*,*,#4834,.T.);
#6384=ORIENTED_EDGE('',*,*,#4785,.T.);
#6385=ORIENTED_EDGE('',*,*,#4834,.F.);
#6386=ORIENTED_EDGE('',*,*,#4804,.F.);
#6387=ORIENTED_EDGE('',*,*,#4835,.T.);
#6388=ORIENTED_EDGE('',*,*,#4786,.T.);
#6389=ORIENTED_EDGE('',*,*,#4835,.F.);
#6390=ORIENTED_EDGE('',*,*,#4803,.F.);
#6391=ORIENTED_EDGE('',*,*,#4836,.T.);
#6392=ORIENTED_EDGE('',*,*,#4787,.T.);
#6393=ORIENTED_EDGE('',*,*,#4836,.F.);
#6394=ORIENTED_EDGE('',*,*,#4802,.F.);
#6395=ORIENTED_EDGE('',*,*,#4837,.T.);
#6396=ORIENTED_EDGE('',*,*,#4788,.T.);
#6397=ORIENTED_EDGE('',*,*,#4837,.F.);
#6398=ORIENTED_EDGE('',*,*,#4801,.F.);
#6399=ORIENTED_EDGE('',*,*,#4838,.T.);
#6400=ORIENTED_EDGE('',*,*,#4789,.T.);
#6401=ORIENTED_EDGE('',*,*,#4838,.F.);
#6402=ORIENTED_EDGE('',*,*,#4800,.F.);
#6403=ORIENTED_EDGE('',*,*,#4839,.T.);
#6404=ORIENTED_EDGE('',*,*,#4790,.T.);
#6405=ORIENTED_EDGE('',*,*,#4839,.F.);
#6406=ORIENTED_EDGE('',*,*,#4799,.F.);
#6407=ORIENTED_EDGE('',*,*,#4840,.T.);
#6408=ORIENTED_EDGE('',*,*,#4791,.T.);
#6409=ORIENTED_EDGE('',*,*,#4840,.F.);
#6410=ORIENTED_EDGE('',*,*,#4798,.F.);
#6411=ORIENTED_EDGE('',*,*,#4768,.T.);
#6412=ORIENTED_EDGE('',*,*,#4841,.F.);
#6413=ORIENTED_EDGE('',*,*,#4842,.T.);
#6414=ORIENTED_EDGE('',*,*,#4645,.F.);
#6415=ORIENTED_EDGE('',*,*,#4453,.T.);
#6416=ORIENTED_EDGE('',*,*,#4795,.F.);
#6417=ORIENTED_EDGE('',*,*,#4820,.F.);
#6418=ORIENTED_EDGE('',*,*,#4843,.T.);
#6419=ORIENTED_EDGE('',*,*,#4841,.T.);
#6420=ORIENTED_EDGE('',*,*,#4743,.F.);
#6421=ORIENTED_EDGE('',*,*,#4844,.T.);
#6422=ORIENTED_EDGE('',*,*,#4845,.F.);
#6423=ORIENTED_EDGE('',*,*,#4792,.F.);
#6424=ORIENTED_EDGE('',*,*,#4449,.T.);
#6425=ORIENTED_EDGE('',*,*,#4845,.T.);
#6426=ORIENTED_EDGE('',*,*,#4846,.T.);
#6427=ORIENTED_EDGE('',*,*,#4821,.F.);
#6428=ORIENTED_EDGE('',*,*,#4443,.T.);
#6429=ORIENTED_EDGE('',*,*,#4747,.F.);
#6430=ORIENTED_EDGE('',*,*,#4847,.F.);
#6431=ORIENTED_EDGE('',*,*,#4844,.F.);
#6432=ORIENTED_EDGE('',*,*,#4847,.T.);
#6433=ORIENTED_EDGE('',*,*,#4746,.F.);
#6434=ORIENTED_EDGE('',*,*,#4848,.F.);
#6435=ORIENTED_EDGE('',*,*,#4846,.F.);
#6436=ORIENTED_EDGE('',*,*,#4848,.T.);
#6437=ORIENTED_EDGE('',*,*,#4745,.F.);
#6438=ORIENTED_EDGE('',*,*,#4752,.F.);
#6439=ORIENTED_EDGE('',*,*,#4772,.F.);
#6440=ORIENTED_EDGE('',*,*,#4822,.F.);
#6441=ORIENTED_EDGE('',*,*,#4439,.T.);
#6442=ORIENTED_EDGE('',*,*,#4842,.F.);
#6443=ORIENTED_EDGE('',*,*,#4849,.F.);
#6444=ORIENTED_EDGE('',*,*,#4748,.F.);
#6445=ORIENTED_EDGE('',*,*,#4849,.T.);
#6446=ORIENTED_EDGE('',*,*,#4843,.F.);
#6447=ORIENTED_EDGE('',*,*,#4850,.F.);
#6448=ORIENTED_EDGE('',*,*,#4749,.F.);
#6449=ORIENTED_EDGE('',*,*,#4850,.T.);
#6450=ORIENTED_EDGE('',*,*,#4819,.F.);
#6451=ORIENTED_EDGE('',*,*,#4817,.F.);
#6452=ORIENTED_EDGE('',*,*,#4753,.F.);
#6453=ORIENTED_EDGE('',*,*,#4750,.F.);
#6454=ORIENTED_EDGE('',*,*,#4587,.T.);
#6455=ORIENTED_EDGE('',*,*,#4480,.T.);
#6456=ORIENTED_EDGE('',*,*,#4851,.T.);
#6457=ORIENTED_EDGE('',*,*,#4852,.T.);
#6458=ORIENTED_EDGE('',*,*,#4736,.T.);
#6459=ORIENTED_EDGE('',*,*,#4735,.T.);
#6460=ORIENTED_EDGE('',*,*,#4853,.T.);
#6461=ORIENTED_EDGE('',*,*,#4851,.F.);
#6462=ORIENTED_EDGE('',*,*,#4486,.T.);
#6463=ORIENTED_EDGE('',*,*,#4712,.F.);
#6464=ORIENTED_EDGE('',*,*,#4673,.F.);
#6465=ORIENTED_EDGE('',*,*,#4688,.F.);
#6466=ORIENTED_EDGE('',*,*,#4854,.F.);
#6467=ORIENTED_EDGE('',*,*,#4581,.F.);
#6468=ORIENTED_EDGE('',*,*,#4854,.T.);
#6469=ORIENTED_EDGE('',*,*,#4680,.F.);
#6470=ORIENTED_EDGE('',*,*,#4855,.F.);
#6471=ORIENTED_EDGE('',*,*,#4582,.F.);
#6472=ORIENTED_EDGE('',*,*,#4855,.T.);
#6473=ORIENTED_EDGE('',*,*,#4686,.F.);
#6474=ORIENTED_EDGE('',*,*,#4856,.F.);
#6475=ORIENTED_EDGE('',*,*,#4583,.F.);
#6476=ORIENTED_EDGE('',*,*,#4474,.F.);
#6477=ORIENTED_EDGE('',*,*,#4436,.T.);
#6478=ORIENTED_EDGE('',*,*,#4584,.F.);
#6479=ORIENTED_EDGE('',*,*,#4856,.T.);
#6480=ORIENTED_EDGE('',*,*,#4671,.F.);
#6481=ORIENTED_EDGE('',*,*,#4695,.F.);
#6482=ORIENTED_EDGE('',*,*,#4857,.F.);
#6483=ORIENTED_EDGE('',*,*,#4689,.F.);
#6484=ORIENTED_EDGE('',*,*,#4857,.T.);
#6485=ORIENTED_EDGE('',*,*,#4694,.F.);
#6486=ORIENTED_EDGE('',*,*,#4858,.F.);
#6487=ORIENTED_EDGE('',*,*,#4682,.F.);
#6488=ORIENTED_EDGE('',*,*,#4858,.T.);
#6489=ORIENTED_EDGE('',*,*,#4693,.F.);
#6490=ORIENTED_EDGE('',*,*,#4859,.F.);
#6491=ORIENTED_EDGE('',*,*,#4687,.F.);
#6492=ORIENTED_EDGE('',*,*,#4859,.T.);
#6493=ORIENTED_EDGE('',*,*,#4692,.F.);
#6494=ORIENTED_EDGE('',*,*,#4860,.F.);
#6495=ORIENTED_EDGE('',*,*,#4471,.F.);
#6496=ORIENTED_EDGE('',*,*,#4860,.T.);
#6497=ORIENTED_EDGE('',*,*,#4691,.F.);
#6498=ORIENTED_EDGE('',*,*,#4861,.F.);
#6499=ORIENTED_EDGE('',*,*,#4652,.F.);
#6500=ORIENTED_EDGE('',*,*,#4861,.T.);
#6501=ORIENTED_EDGE('',*,*,#4705,.F.);
#6502=ORIENTED_EDGE('',*,*,#4862,.F.);
#6503=ORIENTED_EDGE('',*,*,#4653,.F.);
#6504=ORIENTED_EDGE('',*,*,#4862,.T.);
#6505=ORIENTED_EDGE('',*,*,#4684,.F.);
#6506=ORIENTED_EDGE('',*,*,#4863,.F.);
#6507=ORIENTED_EDGE('',*,*,#4654,.F.);
#6508=ORIENTED_EDGE('',*,*,#4863,.T.);
#6509=ORIENTED_EDGE('',*,*,#4704,.F.);
#6510=ORIENTED_EDGE('',*,*,#4864,.F.);
#6511=ORIENTED_EDGE('',*,*,#4646,.F.);
#6512=ORIENTED_EDGE('',*,*,#4864,.T.);
#6513=ORIENTED_EDGE('',*,*,#4700,.F.);
#6514=ORIENTED_EDGE('',*,*,#4865,.F.);
#6515=ORIENTED_EDGE('',*,*,#4647,.F.);
#6516=ORIENTED_EDGE('',*,*,#4865,.T.);
#6517=ORIENTED_EDGE('',*,*,#4699,.F.);
#6518=ORIENTED_EDGE('',*,*,#4866,.F.);
#6519=ORIENTED_EDGE('',*,*,#4469,.F.);
#6520=ORIENTED_EDGE('',*,*,#4866,.T.);
#6521=ORIENTED_EDGE('',*,*,#4698,.F.);
#6522=ORIENTED_EDGE('',*,*,#4867,.F.);
#6523=ORIENTED_EDGE('',*,*,#4655,.F.);
#6524=ORIENTED_EDGE('',*,*,#4867,.T.);
#6525=ORIENTED_EDGE('',*,*,#4697,.F.);
#6526=ORIENTED_EDGE('',*,*,#4868,.F.);
#6527=ORIENTED_EDGE('',*,*,#4702,.F.);
#6528=ORIENTED_EDGE('',*,*,#4868,.T.);
#6529=ORIENTED_EDGE('',*,*,#4696,.F.);
#6530=ORIENTED_EDGE('',*,*,#4665,.F.);
#6531=ORIENTED_EDGE('',*,*,#4659,.F.);
#6532=ORIENTED_EDGE('',*,*,#4869,.T.);
#6533=ORIENTED_EDGE('',*,*,#4853,.F.);
#6534=ORIENTED_EDGE('',*,*,#4734,.T.);
#6535=ORIENTED_EDGE('',*,*,#4499,.T.);
#6536=ORIENTED_EDGE('',*,*,#4591,.F.);
#6537=ORIENTED_EDGE('',*,*,#4537,.T.);
#6538=ORIENTED_EDGE('',*,*,#4619,.F.);
#6539=ORIENTED_EDGE('',*,*,#4631,.T.);
#6540=ORIENTED_EDGE('',*,*,#4556,.F.);
#6541=ORIENTED_EDGE('',*,*,#4632,.T.);
#6542=ORIENTED_EDGE('',*,*,#4634,.F.);
#6543=ORIENTED_EDGE('',*,*,#4870,.F.);
#6544=ORIENTED_EDGE('',*,*,#4554,.F.);
#6545=ORIENTED_EDGE('',*,*,#4870,.T.);
#6546=ORIENTED_EDGE('',*,*,#4496,.T.);
#6547=ORIENTED_EDGE('',*,*,#4709,.T.);
#6548=ORIENTED_EDGE('',*,*,#4852,.F.);
#6549=ORIENTED_EDGE('',*,*,#4869,.F.);
#6550=ORIENTED_EDGE('',*,*,#4555,.F.);
#6551=ORIENTED_EDGE('',*,*,#4478,.T.);
#6552=ORIENTED_EDGE('',*,*,#4871,.F.);
#6553=ORIENTED_EDGE('',*,*,#4476,.F.);
#6554=ORIENTED_EDGE('',*,*,#4588,.F.);
#6555=ORIENTED_EDGE('',*,*,#4477,.T.);
#6556=ORIENTED_EDGE('',*,*,#4871,.T.);
#6557=ORIENTED_EDGE('',*,*,#4488,.T.);
#6558=ORIENTED_EDGE('',*,*,#4711,.T.);
#6559=ORIENTED_EDGE('',*,*,#4490,.F.);
#6560=ORIENTED_EDGE('',*,*,#4589,.F.);
#6561=ORIENTED_EDGE('',*,*,#4492,.T.);
#6562=ORIENTED_EDGE('',*,*,#4710,.T.);
#6563=ORIENTED_EDGE('',*,*,#4494,.F.);
#6564=ORIENTED_EDGE('',*,*,#4551,.F.);
#6565=ORIENTED_EDGE('',*,*,#4620,.T.);
#6566=ORIENTED_EDGE('',*,*,#4602,.F.);
#6567=ORIENTED_EDGE('',*,*,#4527,.T.);
#6568=ORIENTED_EDGE('',*,*,#4600,.F.);
#6569=ORIENTED_EDGE('',*,*,#4521,.T.);
#6570=ORIENTED_EDGE('',*,*,#4718,.T.);
#6571=ORIENTED_EDGE('',*,*,#4872,.F.);
#6572=ORIENTED_EDGE('',*,*,#4578,.F.);
#6573=ORIENTED_EDGE('',*,*,#4873,.T.);
#6574=ORIENTED_EDGE('',*,*,#4716,.T.);
#6575=ORIENTED_EDGE('',*,*,#4523,.T.);
#6576=ORIENTED_EDGE('',*,*,#4738,.F.);
#6577=ORIENTED_EDGE('',*,*,#4706,.T.);
#6578=ORIENTED_EDGE('',*,*,#4739,.F.);
#6579=ORIENTED_EDGE('',*,*,#4675,.F.);
#6580=ORIENTED_EDGE('',*,*,#4579,.F.);
#6581=ORIENTED_EDGE('',*,*,#4872,.T.);
#6582=ORIENTED_EDGE('',*,*,#4717,.T.);
#6583=ORIENTED_EDGE('',*,*,#4873,.F.);
#6584=ORIENTED_EDGE('',*,*,#4674,.F.);
#6585=ORIENTED_EDGE('',*,*,#4874,.T.);
#6586=ORIENTED_EDGE('',*,*,#4719,.T.);
#6587=ORIENTED_EDGE('',*,*,#4519,.T.);
#6588=ORIENTED_EDGE('',*,*,#4601,.F.);
#6589=ORIENTED_EDGE('',*,*,#4529,.T.);
#6590=ORIENTED_EDGE('',*,*,#4604,.F.);
#6591=ORIENTED_EDGE('',*,*,#4621,.T.);
#6592=ORIENTED_EDGE('',*,*,#4576,.F.);
#6593=ORIENTED_EDGE('',*,*,#4622,.T.);
#6594=ORIENTED_EDGE('',*,*,#4605,.F.);
#6595=ORIENTED_EDGE('',*,*,#4531,.T.);
#6596=ORIENTED_EDGE('',*,*,#4598,.F.);
#6597=ORIENTED_EDGE('',*,*,#4517,.T.);
#6598=ORIENTED_EDGE('',*,*,#4721,.T.);
#6599=ORIENTED_EDGE('',*,*,#4875,.F.);
#6600=ORIENTED_EDGE('',*,*,#4574,.F.);
#6601=ORIENTED_EDGE('',*,*,#4875,.T.);
#6602=ORIENTED_EDGE('',*,*,#4720,.T.);
#6603=ORIENTED_EDGE('',*,*,#4874,.F.);
#6604=ORIENTED_EDGE('',*,*,#4575,.F.);
#6605=ORIENTED_EDGE('',*,*,#4876,.T.);
#6606=ORIENTED_EDGE('',*,*,#4722,.T.);
#6607=ORIENTED_EDGE('',*,*,#4515,.T.);
#6608=ORIENTED_EDGE('',*,*,#4599,.F.);
#6609=ORIENTED_EDGE('',*,*,#4533,.T.);
#6610=ORIENTED_EDGE('',*,*,#4607,.F.);
#6611=ORIENTED_EDGE('',*,*,#4623,.T.);
#6612=ORIENTED_EDGE('',*,*,#4572,.F.);
#6613=ORIENTED_EDGE('',*,*,#4624,.T.);
#6614=ORIENTED_EDGE('',*,*,#4608,.F.);
#6615=ORIENTED_EDGE('',*,*,#4547,.T.);
#6616=ORIENTED_EDGE('',*,*,#4596,.F.);
#6617=ORIENTED_EDGE('',*,*,#4513,.T.);
#6618=ORIENTED_EDGE('',*,*,#4724,.T.);
#6619=ORIENTED_EDGE('',*,*,#4877,.F.);
#6620=ORIENTED_EDGE('',*,*,#4570,.F.);
#6621=ORIENTED_EDGE('',*,*,#4877,.T.);
#6622=ORIENTED_EDGE('',*,*,#4723,.T.);
#6623=ORIENTED_EDGE('',*,*,#4876,.F.);
#6624=ORIENTED_EDGE('',*,*,#4571,.F.);
#6625=ORIENTED_EDGE('',*,*,#4878,.T.);
#6626=ORIENTED_EDGE('',*,*,#4725,.T.);
#6627=ORIENTED_EDGE('',*,*,#4511,.T.);
#6628=ORIENTED_EDGE('',*,*,#4597,.F.);
#6629=ORIENTED_EDGE('',*,*,#4549,.T.);
#6630=ORIENTED_EDGE('',*,*,#4610,.F.);
#6631=ORIENTED_EDGE('',*,*,#4625,.T.);
#6632=ORIENTED_EDGE('',*,*,#4568,.F.);
#6633=ORIENTED_EDGE('',*,*,#4626,.T.);
#6634=ORIENTED_EDGE('',*,*,#4611,.F.);
#6635=ORIENTED_EDGE('',*,*,#4543,.T.);
#6636=ORIENTED_EDGE('',*,*,#4594,.F.);
#6637=ORIENTED_EDGE('',*,*,#4509,.T.);
#6638=ORIENTED_EDGE('',*,*,#4727,.T.);
#6639=ORIENTED_EDGE('',*,*,#4879,.F.);
#6640=ORIENTED_EDGE('',*,*,#4566,.F.);
#6641=ORIENTED_EDGE('',*,*,#4879,.T.);
#6642=ORIENTED_EDGE('',*,*,#4726,.T.);
#6643=ORIENTED_EDGE('',*,*,#4878,.F.);
#6644=ORIENTED_EDGE('',*,*,#4567,.F.);
#6645=ORIENTED_EDGE('',*,*,#4880,.T.);
#6646=ORIENTED_EDGE('',*,*,#4728,.T.);
#6647=ORIENTED_EDGE('',*,*,#4507,.T.);
#6648=ORIENTED_EDGE('',*,*,#4595,.F.);
#6649=ORIENTED_EDGE('',*,*,#4545,.T.);
#6650=ORIENTED_EDGE('',*,*,#4613,.F.);
#6651=ORIENTED_EDGE('',*,*,#4627,.T.);
#6652=ORIENTED_EDGE('',*,*,#4564,.F.);
#6653=ORIENTED_EDGE('',*,*,#4628,.T.);
#6654=ORIENTED_EDGE('',*,*,#4614,.F.);
#6655=ORIENTED_EDGE('',*,*,#4539,.T.);
#6656=ORIENTED_EDGE('',*,*,#4592,.F.);
#6657=ORIENTED_EDGE('',*,*,#4505,.T.);
#6658=ORIENTED_EDGE('',*,*,#4730,.T.);
#6659=ORIENTED_EDGE('',*,*,#4881,.F.);
#6660=ORIENTED_EDGE('',*,*,#4562,.F.);
#6661=ORIENTED_EDGE('',*,*,#4881,.T.);
#6662=ORIENTED_EDGE('',*,*,#4729,.T.);
#6663=ORIENTED_EDGE('',*,*,#4880,.F.);
#6664=ORIENTED_EDGE('',*,*,#4563,.F.);
#6665=ORIENTED_EDGE('',*,*,#4882,.T.);
#6666=ORIENTED_EDGE('',*,*,#4731,.T.);
#6667=ORIENTED_EDGE('',*,*,#4503,.T.);
#6668=ORIENTED_EDGE('',*,*,#4593,.F.);
#6669=ORIENTED_EDGE('',*,*,#4541,.T.);
#6670=ORIENTED_EDGE('',*,*,#4616,.F.);
#6671=ORIENTED_EDGE('',*,*,#4629,.T.);
#6672=ORIENTED_EDGE('',*,*,#4560,.F.);
#6673=ORIENTED_EDGE('',*,*,#4630,.T.);
#6674=ORIENTED_EDGE('',*,*,#4617,.F.);
#6675=ORIENTED_EDGE('',*,*,#4535,.T.);
#6676=ORIENTED_EDGE('',*,*,#4590,.F.);
#6677=ORIENTED_EDGE('',*,*,#4501,.T.);
#6678=ORIENTED_EDGE('',*,*,#4733,.T.);
#6679=ORIENTED_EDGE('',*,*,#4883,.F.);
#6680=ORIENTED_EDGE('',*,*,#4558,.F.);
#6681=ORIENTED_EDGE('',*,*,#4883,.T.);
#6682=ORIENTED_EDGE('',*,*,#4732,.T.);
#6683=ORIENTED_EDGE('',*,*,#4882,.F.);
#6684=ORIENTED_EDGE('',*,*,#4559,.F.);
#6685=ORIENTED_EDGE('',*,*,#4737,.F.);
#6686=ORIENTED_EDGE('',*,*,#4525,.T.);
#6687=ORIENTED_EDGE('',*,*,#4715,.T.);
#6688=ORIENTED_EDGE('',*,*,#4884,.F.);
#6689=ORIENTED_EDGE('',*,*,#4662,.F.);
#6690=ORIENTED_EDGE('',*,*,#4884,.T.);
#6691=ORIENTED_EDGE('',*,*,#4714,.T.);
#6692=ORIENTED_EDGE('',*,*,#4663,.F.);
#6693=ORIENTED_EDGE('',*,*,#4763,.F.);
#6694=ORIENTED_EDGE('',*,*,#4885,.T.);
#6695=ORIENTED_EDGE('',*,*,#4430,.T.);
#6696=ORIENTED_EDGE('',*,*,#4886,.T.);
#6697=ORIENTED_EDGE('',*,*,#4797,.F.);
#6698=ORIENTED_EDGE('',*,*,#4456,.F.);
#6699=ORIENTED_EDGE('',*,*,#4887,.F.);
#6700=ORIENTED_EDGE('',*,*,#4760,.F.);
#6701=ORIENTED_EDGE('',*,*,#4887,.T.);
#6702=ORIENTED_EDGE('',*,*,#4451,.F.);
#6703=ORIENTED_EDGE('',*,*,#4888,.F.);
#6704=ORIENTED_EDGE('',*,*,#4761,.F.);
#6705=ORIENTED_EDGE('',*,*,#4888,.T.);
#6706=ORIENTED_EDGE('',*,*,#4644,.F.);
#6707=ORIENTED_EDGE('',*,*,#4889,.F.);
#6708=ORIENTED_EDGE('',*,*,#4762,.F.);
#6709=ORIENTED_EDGE('',*,*,#4889,.T.);
#6710=ORIENTED_EDGE('',*,*,#4643,.F.);
#6711=ORIENTED_EDGE('',*,*,#4890,.F.);
#6712=ORIENTED_EDGE('',*,*,#4885,.F.);
#6713=ORIENTED_EDGE('',*,*,#4467,.F.);
#6714=ORIENTED_EDGE('',*,*,#4431,.F.);
#6715=ORIENTED_EDGE('',*,*,#4890,.T.);
#6716=ORIENTED_EDGE('',*,*,#4642,.F.);
#6717=ORIENTED_EDGE('',*,*,#4648,.F.);
#6718=ORIENTED_EDGE('',*,*,#4651,.F.);
#6719=ORIENTED_EDGE('',*,*,#4742,.F.);
#6720=ORIENTED_EDGE('',*,*,#4891,.F.);
#6721=ORIENTED_EDGE('',*,*,#4429,.F.);
#6722=ORIENTED_EDGE('',*,*,#4473,.F.);
#6723=ORIENTED_EDGE('',*,*,#4891,.T.);
#6724=ORIENTED_EDGE('',*,*,#4741,.F.);
#6725=ORIENTED_EDGE('',*,*,#4892,.F.);
#6726=ORIENTED_EDGE('',*,*,#4886,.F.);
#6727=ORIENTED_EDGE('',*,*,#4892,.T.);
#6728=ORIENTED_EDGE('',*,*,#4740,.F.);
#6729=ORIENTED_EDGE('',*,*,#4893,.F.);
#6730=ORIENTED_EDGE('',*,*,#4764,.F.);
#6731=ORIENTED_EDGE('',*,*,#4893,.T.);
#6732=ORIENTED_EDGE('',*,*,#4447,.F.);
#6733=ORIENTED_EDGE('',*,*,#4894,.F.);
#6734=ORIENTED_EDGE('',*,*,#4765,.F.);
#6735=ORIENTED_EDGE('',*,*,#4769,.F.);
#6736=ORIENTED_EDGE('',*,*,#4766,.F.);
#6737=ORIENTED_EDGE('',*,*,#4894,.T.);
#6738=ORIENTED_EDGE('',*,*,#4458,.F.);
#8437=ADVANCED_FACE('',(#2087),#1861,.T.);
#8438=ADVANCED_FACE('',(#2088),#610,.T.);
#8439=ADVANCED_FACE('',(#2089),#611,.T.);
#8440=ADVANCED_FACE('',(#2090),#612,.F.);
#8441=ADVANCED_FACE('',(#2091),#613,.F.);
#8442=ADVANCED_FACE('',(#2092),#137,.T.);
#8443=ADVANCED_FACE('',(#2093),#138,.T.);
#8444=ADVANCED_FACE('',(#2094),#1862,.F.);
#8445=ADVANCED_FACE('',(#2095),#1863,.F.);
#8446=ADVANCED_FACE('',(#2096),#1864,.T.);
#8447=ADVANCED_FACE('',(#2097),#1865,.T.);
#8448=ADVANCED_FACE('',(#2098),#1866,.F.);
#8449=ADVANCED_FACE('',(#2099),#1867,.F.);
#8450=ADVANCED_FACE('',(#2100),#1868,.F.);
#8451=ADVANCED_FACE('',(#2101),#1869,.F.);
#8452=ADVANCED_FACE('',(#2102),#1870,.F.);
#8453=ADVANCED_FACE('',(#2103),#1871,.F.);
#8454=ADVANCED_FACE('',(#2104),#1872,.F.);
#8455=ADVANCED_FACE('',(#2105),#1873,.F.);
#8456=ADVANCED_FACE('',(#2106),#1874,.F.);
#8457=ADVANCED_FACE('',(#2107),#1875,.F.);
#8458=ADVANCED_FACE('',(#2108),#124,.T.);
#8459=ADVANCED_FACE('',(#2109),#125,.T.);
#8460=ADVANCED_FACE('',(#2110),#126,.T.);
#8461=ADVANCED_FACE('',(#2111),#127,.T.);
#8462=ADVANCED_FACE('',(#2112),#128,.T.);
#8463=ADVANCED_FACE('',(#2113),#129,.T.);
#8464=ADVANCED_FACE('',(#2114,#726),#765,.F.);
#8465=ADVANCED_FACE('',(#2115),#532,.F.);
#8466=ADVANCED_FACE('',(#2116),#533,.F.);
#8467=ADVANCED_FACE('',(#2117),#534,.F.);
#8468=ADVANCED_FACE('',(#2118),#535,.F.);
#8469=ADVANCED_FACE('',(#2119),#536,.F.);
#8470=ADVANCED_FACE('',(#2120),#537,.F.);
#8471=ADVANCED_FACE('',(#2121),#538,.F.);
#8472=ADVANCED_FACE('',(#2122),#539,.F.);
#8473=ADVANCED_FACE('',(#2123),#540,.F.);
#8474=ADVANCED_FACE('',(#2124),#541,.F.);
#8475=ADVANCED_FACE('',(#2125),#542,.F.);
#8476=ADVANCED_FACE('',(#2126),#543,.F.);
#8477=ADVANCED_FACE('',(#2127),#1876,.F.);
#8478=ADVANCED_FACE('',(#2128),#1877,.F.);
#8479=ADVANCED_FACE('',(#2129),#1878,.F.);
#8480=ADVANCED_FACE('',(#2130),#1879,.F.);
#8481=ADVANCED_FACE('',(#2131),#1880,.F.);
#8482=ADVANCED_FACE('',(#2132),#1881,.F.);
#8483=ADVANCED_FACE('',(#2133),#1882,.F.);
#8484=ADVANCED_FACE('',(#2134),#766,.F.);
#8485=ADVANCED_FACE('',(#2135),#130,.T.);
#8486=ADVANCED_FACE('',(#2136),#544,.F.);
#8487=ADVANCED_FACE('',(#2137),#545,.F.);
#8488=ADVANCED_FACE('',(#2138),#767,.F.);
#8489=ADVANCED_FACE('',(#2139),#768,.F.);
#8490=ADVANCED_FACE('',(#2140),#769,.F.);
#8491=ADVANCED_FACE('',(#2141),#770,.F.);
#8492=ADVANCED_FACE('',(#2142),#771,.F.);
#8493=ADVANCED_FACE('',(#2143),#1883,.F.);
#8494=ADVANCED_FACE('',(#2144),#131,.F.);
#8495=ADVANCED_FACE('',(#2145),#772,.F.);
#8496=ADVANCED_FACE('',(#2146),#773,.F.);
#8497=ADVANCED_FACE('',(#2147,#727),#774,.T.);
#8498=ADVANCED_FACE('',(#2148,#728),#775,.F.);
#8499=ADVANCED_FACE('',(#2149),#1884,.F.);
#8500=ADVANCED_FACE('',(#2150),#546,.T.);
#8501=ADVANCED_FACE('',(#2151),#547,.T.);
#8502=ADVANCED_FACE('',(#2152),#132,.T.);
#8503=ADVANCED_FACE('',(#2153,#729),#776,.T.);
#8504=ADVANCED_FACE('',(#2154),#548,.F.);
#8505=ADVANCED_FACE('',(#2155),#1885,.F.);
#8506=ADVANCED_FACE('',(#2156),#777,.T.);
#8507=ADVANCED_FACE('',(#2157),#778,.T.);
#8508=ADVANCED_FACE('',(#2158),#1886,.T.);
#8509=ADVANCED_FACE('',(#2159),#779,.T.);
#8510=ADVANCED_FACE('',(#2160),#780,.T.);
#8511=ADVANCED_FACE('',(#2161),#1887,.F.);
#8512=ADVANCED_FACE('',(#2162),#781,.T.);
#8513=ADVANCED_FACE('',(#2163),#782,.T.);
#8514=ADVANCED_FACE('',(#2164),#783,.T.);
#8515=ADVANCED_FACE('',(#2165),#784,.F.);
#8516=ADVANCED_FACE('',(#2166),#139,.T.);
#8517=ADVANCED_FACE('',(#2167),#140,.T.);
#8518=ADVANCED_FACE('',(#2168),#785,.F.);
#8519=ADVANCED_FACE('',(#2169),#786,.F.);
#8520=ADVANCED_FACE('',(#2170),#787,.F.);
#8521=ADVANCED_FACE('',(#2171),#788,.F.);
#8522=ADVANCED_FACE('',(#2172),#789,.F.);
#8523=ADVANCED_FACE('',(#2173),#790,.F.);
#8524=ADVANCED_FACE('',(#2174),#791,.F.);
#8525=ADVANCED_FACE('',(#2175),#792,.F.);
#8526=ADVANCED_FACE('',(#2176),#793,.F.);
#8527=ADVANCED_FACE('',(#2177),#794,.F.);
#8528=ADVANCED_FACE('',(#2178),#795,.F.);
#8529=ADVANCED_FACE('',(#2179),#796,.F.);
#8530=ADVANCED_FACE('',(#2180),#797,.F.);
#8531=ADVANCED_FACE('',(#2181),#798,.F.);
#8532=ADVANCED_FACE('',(#2182),#799,.F.);
#8533=ADVANCED_FACE('',(#2183),#800,.F.);
#8534=ADVANCED_FACE('',(#2184),#801,.F.);
#8535=ADVANCED_FACE('',(#2185),#802,.F.);
#8536=ADVANCED_FACE('',(#2186),#803,.F.);
#8537=ADVANCED_FACE('',(#2187),#1888,.F.);
#8538=ADVANCED_FACE('',(#2188),#614,.F.);
#8539=ADVANCED_FACE('',(#2189),#1889,.F.);
#8540=ADVANCED_FACE('',(#2190),#615,.F.);
#8541=ADVANCED_FACE('',(#2191),#549,.T.);
#8542=ADVANCED_FACE('',(#2192),#550,.T.);
#8543=ADVANCED_FACE('',(#2193),#551,.T.);
#8544=ADVANCED_FACE('',(#2194),#552,.T.);
#8545=ADVANCED_FACE('',(#2195),#553,.T.);
#8546=ADVANCED_FACE('',(#2196),#554,.T.);
#8547=ADVANCED_FACE('',(#2197),#804,.T.);
#8548=ADVANCED_FACE('',(#2198),#1890,.F.);
#8549=ADVANCED_FACE('',(#2199),#805,.F.);
#8550=ADVANCED_FACE('',(#2200),#806,.T.);
#8551=ADVANCED_FACE('',(#2201),#1891,.T.);
#8552=ADVANCED_FACE('',(#2202),#616,.T.);
#8553=ADVANCED_FACE('',(#2203),#1892,.T.);
#8554=ADVANCED_FACE('',(#2204),#617,.T.);
#8555=ADVANCED_FACE('',(#2205),#1893,.T.);
#8556=ADVANCED_FACE('',(#2206),#618,.T.);
#8557=ADVANCED_FACE('',(#2207),#1894,.T.);
#8558=ADVANCED_FACE('',(#2208),#619,.T.);
#8559=ADVANCED_FACE('',(#2209),#1895,.T.);
#8560=ADVANCED_FACE('',(#2210),#555,.T.);
#8561=ADVANCED_FACE('',(#2211),#1896,.T.);
#8562=ADVANCED_FACE('',(#2212),#556,.T.);
#8563=ADVANCED_FACE('',(#2213),#1897,.T.);
#8564=ADVANCED_FACE('',(#2214),#620,.T.);
#8565=ADVANCED_FACE('',(#2215),#1898,.T.);
#8566=ADVANCED_FACE('',(#2216),#621,.T.);
#8567=ADVANCED_FACE('',(#2217),#1899,.T.);
#8568=ADVANCED_FACE('',(#2218),#557,.F.);
#8569=ADVANCED_FACE('',(#2219),#558,.F.);
#8570=ADVANCED_FACE('',(#2220),#559,.F.);
#8571=ADVANCED_FACE('',(#2221),#560,.F.);
#8572=ADVANCED_FACE('',(#2222),#807,.T.);
#8573=ADVANCED_FACE('',(#2223),#561,.F.);
#8574=ADVANCED_FACE('',(#2224),#562,.F.);
#8575=ADVANCED_FACE('',(#2225),#563,.F.);
#8576=ADVANCED_FACE('',(#2226),#564,.F.);
#8577=ADVANCED_FACE('',(#2227),#565,.F.);
#8578=ADVANCED_FACE('',(#2228),#566,.F.);
#8579=ADVANCED_FACE('',(#2229),#567,.F.);
#8580=ADVANCED_FACE('',(#2230),#568,.F.);
#8581=ADVANCED_FACE('',(#2231),#569,.F.);
#8582=ADVANCED_FACE('',(#2232),#570,.F.);
#8583=ADVANCED_FACE('',(#2233),#571,.F.);
#8584=ADVANCED_FACE('',(#2234),#572,.F.);
#8585=ADVANCED_FACE('',(#2235),#573,.F.);
#8586=ADVANCED_FACE('',(#2236),#574,.F.);
#8587=ADVANCED_FACE('',(#2237),#575,.F.);
#8588=ADVANCED_FACE('',(#2238),#576,.F.);
#8589=ADVANCED_FACE('',(#2239),#577,.F.);
#8590=ADVANCED_FACE('',(#2240),#578,.F.);
#8591=ADVANCED_FACE('',(#2241),#579,.F.);
#8592=ADVANCED_FACE('',(#2242),#580,.F.);
#8593=ADVANCED_FACE('',(#2243),#581,.F.);
#8594=ADVANCED_FACE('',(#2244),#582,.F.);
#8595=ADVANCED_FACE('',(#2245),#1900,.T.);
#8596=ADVANCED_FACE('',(#2246),#583,.T.);
#8597=ADVANCED_FACE('',(#2247),#584,.T.);
#8598=ADVANCED_FACE('',(#2248),#622,.T.);
#8599=ADVANCED_FACE('',(#2249),#623,.T.);
#8600=ADVANCED_FACE('',(#2250),#624,.T.);
#8601=ADVANCED_FACE('',(#2251),#625,.T.);
#8602=ADVANCED_FACE('',(#2252),#626,.T.);
#8603=ADVANCED_FACE('',(#2253),#627,.T.);
#8604=ADVANCED_FACE('',(#2254),#585,.T.);
#8605=ADVANCED_FACE('',(#2255),#586,.T.);
#8928=CLOSED_SHELL('',(#8437,#8438,#8439,#8440,#8441,#8442,#8443,#8444,
#8445,#8446,#8447,#8448,#8449,#8450,#8451,#8452,#8453,#8454,#8455,#8456,
#8457,#8458,#8459,#8460,#8461,#8462,#8463,#8464,#8465,#8466,#8467,#8468,
#8469,#8470,#8471,#8472,#8473,#8474,#8475,#8476,#8477,#8478,#8479,#8480,
#8481,#8482,#8483,#8484,#8485,#8486,#8487,#8488,#8489,#8490,#8491,#8492,
#8493,#8494,#8495,#8496,#8497,#8498,#8499,#8500,#8501,#8502,#8503,#8504,
#8505,#8506,#8507,#8508,#8509,#8510,#8511,#8512,#8513,#8514,#8515,#8516,
#8517,#8518,#8519,#8520,#8521,#8522,#8523,#8524,#8525,#8526,#8527,#8528,
#8529,#8530,#8531,#8532,#8533,#8534,#8535,#8536,#8537,#8538,#8539,#8540,
#8541,#8542,#8543,#8544,#8545,#8546,#8547,#8548,#8549,#8550,#8551,#8552,
#8553,#8554,#8555,#8556,#8557,#8558,#8559,#8560,#8561,#8562,#8563,#8564,
#8565,#8566,#8567,#8568,#8569,#8570,#8571,#8572,#8573,#8574,#8575,#8576,
#8577,#8578,#8579,#8580,#8581,#8582,#8583,#8584,#8585,#8586,#8587,#8588,
#8589,#8590,#8591,#8592,#8593,#8594,#8595,#8596,#8597,#8598,#8599,#8600,
#8601,#8602,#8603,#8604,#8605));
#9122=AXIS2_PLACEMENT_3D('',#15689,#10064,#10065);
#9123=AXIS2_PLACEMENT_3D('',#15690,#10066,#10067);
#9124=AXIS2_PLACEMENT_3D('',#15693,#10068,#10069);
#9125=AXIS2_PLACEMENT_3D('',#15697,#10071,#10072);
#9126=AXIS2_PLACEMENT_3D('',#15701,#10074,#10075);
#9127=AXIS2_PLACEMENT_3D('',#15705,#10077,#10078);
#9128=AXIS2_PLACEMENT_3D('',#15720,#10080,#10081);
#9129=AXIS2_PLACEMENT_3D('',#15723,#10082,#10083);
#9130=AXIS2_PLACEMENT_3D('',#15725,#10084,#10085);
#9131=AXIS2_PLACEMENT_3D('',#15727,#10086,#10087);
#9132=AXIS2_PLACEMENT_3D('',#15738,#10088,#10089);
#9133=AXIS2_PLACEMENT_3D('',#15741,#10090,#10091);
#9134=AXIS2_PLACEMENT_3D('',#15743,#10092,#10093);
#9135=AXIS2_PLACEMENT_3D('',#15745,#10094,#10095);
#9136=AXIS2_PLACEMENT_3D('',#15756,#10096,#10097);
#9137=AXIS2_PLACEMENT_3D('',#15759,#10098,#10099);
#9138=AXIS2_PLACEMENT_3D('',#15793,#10100,#10101);
#9139=AXIS2_PLACEMENT_3D('',#15794,#10102,#10103);
#9140=AXIS2_PLACEMENT_3D('',#15795,#10104,#10105);
#9141=AXIS2_PLACEMENT_3D('',#15798,#10106,#10107);
#9142=AXIS2_PLACEMENT_3D('',#15832,#10108,#10109);
#9143=AXIS2_PLACEMENT_3D('',#15833,#10110,#10111);
#9144=AXIS2_PLACEMENT_3D('',#15834,#10112,#10113);
#9145=AXIS2_PLACEMENT_3D('',#15837,#10114,#10115);
#9146=AXIS2_PLACEMENT_3D('',#15846,#10116,#10117);
#9147=AXIS2_PLACEMENT_3D('',#15849,#10118,#10119);
#9148=AXIS2_PLACEMENT_3D('',#15858,#10120,#10121);
#9149=AXIS2_PLACEMENT_3D('',#15860,#10122,#10123);
#9150=AXIS2_PLACEMENT_3D('',#15863,#10125,#10126);
#9151=AXIS2_PLACEMENT_3D('',#15864,#10127,#10128);
#9152=AXIS2_PLACEMENT_3D('',#15866,#10129,#10130);
#9153=AXIS2_PLACEMENT_3D('',#15869,#10132,#10133);
#9154=AXIS2_PLACEMENT_3D('',#15870,#10134,#10135);
#9155=AXIS2_PLACEMENT_3D('',#15872,#10136,#10137);
#9156=AXIS2_PLACEMENT_3D('',#15885,#10139,#10140);
#9157=AXIS2_PLACEMENT_3D('',#15887,#10142,#10143);
#9158=AXIS2_PLACEMENT_3D('',#15890,#10144,#10145);
#9159=AXIS2_PLACEMENT_3D('',#15904,#10147,#10148);
#9160=AXIS2_PLACEMENT_3D('',#15906,#10150,#10151);
#9161=AXIS2_PLACEMENT_3D('',#15939,#10154,#10155);
#9162=AXIS2_PLACEMENT_3D('',#16176,#10158,#10159);
#9163=AXIS2_PLACEMENT_3D('',#16211,#10162,#10163);
#9164=AXIS2_PLACEMENT_3D('',#16278,#10166,#10167);
#9165=AXIS2_PLACEMENT_3D('',#16333,#10169,#10170);
#9166=AXIS2_PLACEMENT_3D('',#16335,#10172,#10173);
#9167=AXIS2_PLACEMENT_3D('',#16362,#10176,#10177);
#9168=AXIS2_PLACEMENT_3D('',#16389,#10180,#10181);
#9169=AXIS2_PLACEMENT_3D('',#16416,#10184,#10185);
#9170=AXIS2_PLACEMENT_3D('',#16443,#10188,#10189);
#9171=AXIS2_PLACEMENT_3D('',#16470,#10192,#10193);
#9172=AXIS2_PLACEMENT_3D('',#16497,#10196,#10197);
#9173=AXIS2_PLACEMENT_3D('',#17079,#10200,#10201);
#9174=AXIS2_PLACEMENT_3D('',#17080,#10202,#10203);
#9175=AXIS2_PLACEMENT_3D('',#17093,#10206,#10207);
#9176=AXIS2_PLACEMENT_3D('',#17111,#10209,#10210);
#9177=AXIS2_PLACEMENT_3D('',#17129,#10212,#10213);
#9178=AXIS2_PLACEMENT_3D('',#17147,#10215,#10216);
#9179=AXIS2_PLACEMENT_3D('',#17165,#10218,#10219);
#9180=AXIS2_PLACEMENT_3D('',#17183,#10221,#10222);
#9181=AXIS2_PLACEMENT_3D('',#17212,#10226,#10227);
#9182=AXIS2_PLACEMENT_3D('',#17215,#10229,#10230);
#9183=AXIS2_PLACEMENT_3D('',#17289,#10233,#10234);
#9184=AXIS2_PLACEMENT_3D('',#17290,#10235,#10236);
#9185=AXIS2_PLACEMENT_3D('',#17839,#10243,#10244);
#9186=AXIS2_PLACEMENT_3D('',#17850,#10245,#10246);
#9187=AXIS2_PLACEMENT_3D('',#17861,#10247,#10248);
#9188=AXIS2_PLACEMENT_3D('',#17872,#10249,#10250);
#9189=AXIS2_PLACEMENT_3D('',#17883,#10251,#10252);
#9190=AXIS2_PLACEMENT_3D('',#17894,#10253,#10254);
#9191=AXIS2_PLACEMENT_3D('',#17905,#10255,#10256);
#9192=AXIS2_PLACEMENT_3D('',#17912,#10257,#10258);
#9193=AXIS2_PLACEMENT_3D('',#17913,#10259,#10260);
#9194=AXIS2_PLACEMENT_3D('',#18334,#10262,#10263);
#9195=AXIS2_PLACEMENT_3D('',#18338,#10265,#10266);
#9196=AXIS2_PLACEMENT_3D('',#18340,#10267,#10268);
#9197=AXIS2_PLACEMENT_3D('',#18341,#10269,#10270);
#9198=AXIS2_PLACEMENT_3D('',#18343,#10272,#10273);
#9199=AXIS2_PLACEMENT_3D('',#18378,#10275,#10276);
#9200=AXIS2_PLACEMENT_3D('',#18382,#10279,#10280);
#9201=AXIS2_PLACEMENT_3D('',#18424,#10283,#10284);
#9202=AXIS2_PLACEMENT_3D('',#18430,#10288,#10289);
#9203=AXIS2_PLACEMENT_3D('',#18439,#10294,#10295);
#9204=AXIS2_PLACEMENT_3D('',#18463,#10297,#10298);
#9205=AXIS2_PLACEMENT_3D('',#18467,#10300,#10301);
#9206=AXIS2_PLACEMENT_3D('',#18471,#10303,#10304);
#9207=AXIS2_PLACEMENT_3D('',#18475,#10306,#10307);
#9208=AXIS2_PLACEMENT_3D('',#18478,#10309,#10310);
#9209=AXIS2_PLACEMENT_3D('',#18500,#10311,#10312);
#9210=AXIS2_PLACEMENT_3D('',#18503,#10314,#10315);
#9211=AXIS2_PLACEMENT_3D('',#18504,#10316,#10317);
#9212=AXIS2_PLACEMENT_3D('',#18509,#10319,#10320);
#9213=AXIS2_PLACEMENT_3D('',#18512,#10322,#10323);
#9214=AXIS2_PLACEMENT_3D('',#18578,#10325,#10326);
#9215=AXIS2_PLACEMENT_3D('',#18581,#10329,#10330);
#9216=AXIS2_PLACEMENT_3D('',#18584,#10333,#10334);
#9217=AXIS2_PLACEMENT_3D('',#18674,#10336,#10337);
#9218=AXIS2_PLACEMENT_3D('',#18678,#10339,#10340);
#9219=AXIS2_PLACEMENT_3D('',#18680,#10342,#10343);
#9220=AXIS2_PLACEMENT_3D('',#18684,#10345,#10346);
#9221=AXIS2_PLACEMENT_3D('',#18688,#10348,#10349);
#9222=AXIS2_PLACEMENT_3D('',#18773,#10351,#10352);
#9223=AXIS2_PLACEMENT_3D('',#18774,#10353,#10354);
#9224=AXIS2_PLACEMENT_3D('',#18775,#10355,#10356);
#9225=AXIS2_PLACEMENT_3D('',#19156,#10358,#10359);
#9226=AXIS2_PLACEMENT_3D('',#19158,#10360,#10361);
#9227=AXIS2_PLACEMENT_3D('',#19159,#10362,#10363);
#9228=AXIS2_PLACEMENT_3D('',#19160,#10364,#10365);
#9229=AXIS2_PLACEMENT_3D('',#19164,#10368,#10369);
#9230=AXIS2_PLACEMENT_3D('',#19179,#10370,#10371);
#9231=AXIS2_PLACEMENT_3D('',#19194,#10372,#10373);
#9232=AXIS2_PLACEMENT_3D('',#19209,#10374,#10375);
#9233=AXIS2_PLACEMENT_3D('',#19224,#10376,#10377);
#9234=AXIS2_PLACEMENT_3D('',#19239,#10378,#10379);
#9235=AXIS2_PLACEMENT_3D('',#19254,#10380,#10381);
#9236=AXIS2_PLACEMENT_3D('',#19303,#10384,#10385);
#9237=AXIS2_PLACEMENT_3D('',#19332,#10386,#10387);
#9238=AXIS2_PLACEMENT_3D('',#19333,#10388,#10389);
#9239=AXIS2_PLACEMENT_3D('',#19335,#10390,#10391);
#9240=AXIS2_PLACEMENT_3D('',#19337,#10392,#10393);
#9241=AXIS2_PLACEMENT_3D('',#19338,#10394,#10395);
#9242=AXIS2_PLACEMENT_3D('',#19340,#10397,#10398);
#9243=AXIS2_PLACEMENT_3D('',#19444,#10400,#10401);
#9244=AXIS2_PLACEMENT_3D('',#19464,#10405,#10406);
#9245=AXIS2_PLACEMENT_3D('',#19470,#10410,#10411);
#9246=AXIS2_PLACEMENT_3D('',#19473,#10412,#10413);
#9247=AXIS2_PLACEMENT_3D('',#19527,#10414,#10415);
#9248=AXIS2_PLACEMENT_3D('',#19531,#10417,#10418);
#9249=AXIS2_PLACEMENT_3D('',#19588,#10419,#10420);
#9250=AXIS2_PLACEMENT_3D('',#19590,#10422,#10423);
#9251=AXIS2_PLACEMENT_3D('',#19608,#10425,#10426);
#9252=AXIS2_PLACEMENT_3D('',#19652,#10446,#10447);
#9253=AXIS2_PLACEMENT_3D('',#19656,#10450,#10451);
#9254=AXIS2_PLACEMENT_3D('',#19662,#10455,#10456);
#9255=AXIS2_PLACEMENT_3D('',#19721,#10476,#10477);
#9256=AXIS2_PLACEMENT_3D('',#19722,#10478,#10479);
#9257=AXIS2_PLACEMENT_3D('',#19734,#10480,#10481);
#9258=AXIS2_PLACEMENT_3D('',#19735,#10482,#10483);
#9259=AXIS2_PLACEMENT_3D('',#19737,#10484,#10485);
#9260=AXIS2_PLACEMENT_3D('',#19748,#10486,#10487);
#9261=AXIS2_PLACEMENT_3D('',#19750,#10489,#10490);
#9262=AXIS2_PLACEMENT_3D('',#19752,#10492,#10493);
#9263=AXIS2_PLACEMENT_3D('',#19754,#10495,#10496);
#9264=AXIS2_PLACEMENT_3D('',#19756,#10498,#10499);
#9265=AXIS2_PLACEMENT_3D('',#19758,#10501,#10502);
#9266=AXIS2_PLACEMENT_3D('',#19760,#10504,#10505);
#9267=AXIS2_PLACEMENT_3D('',#19762,#10507,#10508);
#9268=AXIS2_PLACEMENT_3D('',#19764,#10510,#10511);
#9269=AXIS2_PLACEMENT_3D('',#19766,#10513,#10514);
#9270=AXIS2_PLACEMENT_3D('',#19768,#10516,#10517);
#9271=AXIS2_PLACEMENT_3D('',#19770,#10519,#10520);
#9272=AXIS2_PLACEMENT_3D('',#19772,#10522,#10523);
#9273=AXIS2_PLACEMENT_3D('',#19774,#10525,#10526);
#9274=AXIS2_PLACEMENT_3D('',#19776,#10528,#10529);
#9275=AXIS2_PLACEMENT_3D('',#19778,#10531,#10532);
#9276=AXIS2_PLACEMENT_3D('',#19780,#10534,#10535);
#9277=AXIS2_PLACEMENT_3D('',#19782,#10537,#10538);
#9278=AXIS2_PLACEMENT_3D('',#19784,#10540,#10541);
#9279=AXIS2_PLACEMENT_3D('',#19785,#10542,#10543);
#9280=AXIS2_PLACEMENT_3D('',#19787,#10544,#10545);
#9281=AXIS2_PLACEMENT_3D('',#19788,#10546,#10547);
#9282=AXIS2_PLACEMENT_3D('',#19789,#10548,#10549);
#9283=AXIS2_PLACEMENT_3D('',#19821,#10550,#10551);
#9284=AXIS2_PLACEMENT_3D('',#19823,#10552,#10553);
#9285=AXIS2_PLACEMENT_3D('',#19824,#10554,#10555);
#9286=AXIS2_PLACEMENT_3D('',#19825,#10556,#10557);
#9287=AXIS2_PLACEMENT_3D('',#19869,#10558,#10559);
#9288=AXIS2_PLACEMENT_3D('',#19894,#10560,#10561);
#9289=AXIS2_PLACEMENT_3D('',#19925,#10562,#10563);
#9290=AXIS2_PLACEMENT_3D('',#19950,#10564,#10565);
#9291=AXIS2_PLACEMENT_3D('',#19969,#10566,#10567);
#9292=AXIS2_PLACEMENT_3D('',#19970,#10568,#10569);
#9293=AXIS2_PLACEMENT_3D('',#19972,#10570,#10571);
#9294=AXIS2_PLACEMENT_3D('',#19978,#10572,#10573);
#9295=AXIS2_PLACEMENT_3D('',#19985,#10574,#10575);
#9296=AXIS2_PLACEMENT_3D('',#19986,#10576,#10577);
#9297=AXIS2_PLACEMENT_3D('',#19987,#10578,#10579);
#9298=AXIS2_PLACEMENT_3D('',#19988,#10580,#10581);
#9299=AXIS2_PLACEMENT_3D('',#19989,#10582,#10583);
#9300=AXIS2_PLACEMENT_3D('',#19990,#10584,#10585);
#9301=AXIS2_PLACEMENT_3D('',#19991,#10586,#10587);
#9302=AXIS2_PLACEMENT_3D('',#19992,#10588,#10589);
#9303=AXIS2_PLACEMENT_3D('',#19993,#10590,#10591);
#9304=AXIS2_PLACEMENT_3D('',#19994,#10592,#10593);
#9305=AXIS2_PLACEMENT_3D('',#19995,#10594,#10595);
#9306=AXIS2_PLACEMENT_3D('',#19996,#10596,#10597);
#9307=AXIS2_PLACEMENT_3D('',#19997,#10598,#10599);
#9308=AXIS2_PLACEMENT_3D('',#19998,#10600,#10601);
#9309=AXIS2_PLACEMENT_3D('',#19999,#10602,#10603);
#9310=AXIS2_PLACEMENT_3D('',#20000,#10604,#10605);
#9311=AXIS2_PLACEMENT_3D('',#20001,#10606,#10607);
#9312=AXIS2_PLACEMENT_3D('',#20002,#10608,#10609);
#9313=AXIS2_PLACEMENT_3D('',#20051,#10610,#10611);
#9314=AXIS2_PLACEMENT_3D('',#20052,#10612,#10613);
#9315=AXIS2_PLACEMENT_3D('',#20053,#10614,#10615);
#9316=AXIS2_PLACEMENT_3D('',#20108,#10616,#10617);
#9317=AXIS2_PLACEMENT_3D('',#20109,#10618,#10619);
#9318=AXIS2_PLACEMENT_3D('',#20110,#10620,#10621);
#9319=AXIS2_PLACEMENT_3D('',#20111,#10622,#10623);
#9320=AXIS2_PLACEMENT_3D('',#20112,#10624,#10625);
#9321=AXIS2_PLACEMENT_3D('',#20113,#10626,#10627);
#9322=AXIS2_PLACEMENT_3D('',#20114,#10628,#10629);
#9323=AXIS2_PLACEMENT_3D('',#20115,#10630,#10631);
#9324=AXIS2_PLACEMENT_3D('',#20116,#10632,#10633);
#9325=AXIS2_PLACEMENT_3D('',#20117,#10634,#10635);
#9326=AXIS2_PLACEMENT_3D('',#22074,#10636,#10637);
#9327=AXIS2_PLACEMENT_3D('',#22075,#10638,#10639);
#9328=AXIS2_PLACEMENT_3D('',#32265,#10640,#10641);
#9329=AXIS2_PLACEMENT_3D('',#32266,#10642,#10643);
#9330=AXIS2_PLACEMENT_3D('',#32267,#10644,#10645);
#9331=AXIS2_PLACEMENT_3D('',#32280,#10646,#10647);
#9332=AXIS2_PLACEMENT_3D('',#32299,#10648,#10649);
#9333=AXIS2_PLACEMENT_3D('',#32300,#10650,#10651);
#9334=AXIS2_PLACEMENT_3D('',#32301,#10652,#10653);
#9335=AXIS2_PLACEMENT_3D('',#32302,#10654,#10655);
#9336=AXIS2_PLACEMENT_3D('',#32303,#10656,#10657);
#9337=AXIS2_PLACEMENT_3D('',#32304,#10658,#10659);
#9338=AXIS2_PLACEMENT_3D('',#32305,#10660,#10661);
#9339=AXIS2_PLACEMENT_3D('',#32306,#10662,#10663);
#9340=AXIS2_PLACEMENT_3D('',#32307,#10664,#10665);
#9341=AXIS2_PLACEMENT_3D('',#32308,#10666,#10667);
#9342=AXIS2_PLACEMENT_3D('',#32309,#10668,#10669);
#9343=AXIS2_PLACEMENT_3D('',#32310,#10670,#10671);
#9344=AXIS2_PLACEMENT_3D('',#32329,#10672,#10673);
#10064=DIRECTION('axis',(0.,0.,1.));
#10065=DIRECTION('refdir',(1.,0.,0.));
#10066=DIRECTION('center_axis',(0.,0.,-1.));
#10067=DIRECTION('ref_axis',(-0.994365489657067,0.106006004448152,0.));
#10068=DIRECTION('center_axis',(0.,0.,-1.));
#10069=DIRECTION('ref_axis',(0.994365489657067,-0.106006004448146,0.));
#10070=DIRECTION('',(0.,0.,1.));
#10071=DIRECTION('center_axis',(0.,0.,1.));
#10072=DIRECTION('ref_axis',(0.994365489657067,-0.106006004448152,0.));
#10073=DIRECTION('',(0.,0.,-1.));
#10074=DIRECTION('center_axis',(0.,0.,-1.));
#10075=DIRECTION('ref_axis',(0.994365489657067,-0.106006004448153,0.));
#10076=DIRECTION('',(0.,0.,-1.));
#10077=DIRECTION('center_axis',(0.,0.,1.));
#10078=DIRECTION('ref_axis',(0.994365489657067,-0.106006004448152,0.));
#10079=DIRECTION('',(0.,0.,1.));
#10080=DIRECTION('center_axis',(0.,0.,1.));
#10081=DIRECTION('ref_axis',(0.994365489657067,-0.106006004448152,0.));
#10082=DIRECTION('center_axis',(0.,0.,-1.));
#10083=DIRECTION('ref_axis',(0.994365489657067,-0.106006004448152,0.));
#10084=DIRECTION('center_axis',(-0.568143764888917,0.822929317996295,-6.78809094260901E-15));
#10085=DIRECTION('ref_axis',(-0.822929317996295,-0.568143764888917,-2.73194523340008E-29));
#10086=DIRECTION('center_axis',(0.,0.,1.));
#10087=DIRECTION('ref_axis',(0.994365489657067,-0.106006004448152,0.));
#10088=DIRECTION('center_axis',(0.,0.,1.));
#10089=DIRECTION('ref_axis',(0.994365489657067,-0.106006004448152,0.));
#10090=DIRECTION('center_axis',(0.,0.,-1.));
#10091=DIRECTION('ref_axis',(0.994365489657067,-0.106006004448152,0.));
#10092=DIRECTION('center_axis',(-0.568143764888923,0.822929317996291,0.));
#10093=DIRECTION('ref_axis',(-0.822929317996291,-0.568143764888923,0.));
#10094=DIRECTION('center_axis',(0.,0.,1.));
#10095=DIRECTION('ref_axis',(0.994365489657067,-0.106006004448152,0.));
#10096=DIRECTION('center_axis',(0.,0.,1.));
#10097=DIRECTION('ref_axis',(0.994365489657067,-0.106006004448151,0.));
#10098=DIRECTION('center_axis',(0.,0.,1.));
#10099=DIRECTION('ref_axis',(-0.994365489657068,0.106006004448146,0.));
#10100=DIRECTION('center_axis',(0.,0.,-1.));
#10101=DIRECTION('ref_axis',(0.99436548965707,-0.106006004448119,0.));
#10102=DIRECTION('center_axis',(0.125069777171418,-0.992147948055995,-2.56328127499069E-6));
#10103=DIRECTION('ref_axis',(-0.000144711787631079,-1.5658743047867E-5,
-0.999999989406651));
#10104=DIRECTION('center_axis',(0.,0.,1.));
#10105=DIRECTION('ref_axis',(0.994365489657067,-0.106006004448151,0.));
#10106=DIRECTION('center_axis',(0.,0.,1.));
#10107=DIRECTION('ref_axis',(0.994365489657067,-0.106006004448152,0.));
#10108=DIRECTION('center_axis',(0.,0.,-1.));
#10109=DIRECTION('ref_axis',(-0.994365489657067,0.106006004448152,0.));
#10110=DIRECTION('center_axis',(0.125069777171398,-0.992147948055998,2.56328132497629E-6));
#10111=DIRECTION('ref_axis',(-0.85915326949364,-0.108303228584418,0.500126054306892));
#10112=DIRECTION('center_axis',(0.,0.,1.));
#10113=DIRECTION('ref_axis',(0.994365489657067,-0.106006004448152,0.));
#10114=DIRECTION('center_axis',(0.,0.,-1.));
#10115=DIRECTION('ref_axis',(0.994365489657067,-0.106006004448152,0.));
#10116=DIRECTION('center_axis',(0.,0.,-1.));
#10117=DIRECTION('ref_axis',(0.994365489657067,-0.106006004448152,0.));
#10118=DIRECTION('center_axis',(0.,0.,-1.));
#10119=DIRECTION('ref_axis',(0.994365489657068,-0.106006004448145,0.));
#10120=DIRECTION('center_axis',(0.,0.,1.));
#10121=DIRECTION('ref_axis',(0.994365489657067,-0.106006004448151,0.));
#10122=DIRECTION('center_axis',(0.,0.,1.));
#10123=DIRECTION('ref_axis',(0.994365489657067,-0.106006004448151,0.));
#10124=DIRECTION('',(0.,0.,1.));
#10125=DIRECTION('center_axis',(0.,0.,1.));
#10126=DIRECTION('ref_axis',(0.994365489657067,-0.106006004448151,0.));
#10127=DIRECTION('center_axis',(0.,0.,1.));
#10128=DIRECTION('ref_axis',(0.994365489657067,-0.106006004448151,0.));
#10129=DIRECTION('center_axis',(0.,0.,1.));
#10130=DIRECTION('ref_axis',(0.994365489657067,-0.106006004448151,0.));
#10131=DIRECTION('',(0.,0.,1.));
#10132=DIRECTION('center_axis',(0.,0.,1.));
#10133=DIRECTION('ref_axis',(0.994365489657067,-0.106006004448151,0.));
#10134=DIRECTION('center_axis',(0.,0.,-1.));
#10135=DIRECTION('ref_axis',(-0.994365489657067,0.106006004448152,0.));
#10136=DIRECTION('center_axis',(0.,0.,-1.));
#10137=DIRECTION('ref_axis',(0.994365489657067,-0.106006004448152,0.));
#10138=DIRECTION('',(0.,0.,1.));
#10139=DIRECTION('center_axis',(0.,0.,1.));
#10140=DIRECTION('ref_axis',(0.994365489657067,-0.106006004448152,0.));
#10141=DIRECTION('',(0.,0.,-1.));
#10142=DIRECTION('center_axis',(0.,0.,-1.));
#10143=DIRECTION('ref_axis',(-0.994365489657067,0.106006004448152,0.));
#10144=DIRECTION('center_axis',(0.,0.,-1.));
#10145=DIRECTION('ref_axis',(0.994365489657067,-0.106006004448152,0.));
#10146=DIRECTION('',(0.,0.,1.));
#10147=DIRECTION('center_axis',(0.,0.,1.));
#10148=DIRECTION('ref_axis',(0.994365489657067,-0.106006004448152,0.));
#10149=DIRECTION('',(0.,0.,-1.));
#10150=DIRECTION('center_axis',(-0.106006004448152,-0.994365489657067,0.));
#10151=DIRECTION('ref_axis',(0.994365489657067,-0.106006004448152,1.08418380562736E-14));
#10152=DIRECTION('',(-0.106006004448152,-0.994365489657067,0.));
#10153=DIRECTION('',(-0.106006004448152,-0.994365489657067,0.));
#10154=DIRECTION('center_axis',(-0.106006004448152,-0.994365489657067,0.));
#10155=DIRECTION('ref_axis',(0.,0.,-1.));
#10156=DIRECTION('',(0.106006004448152,0.994365489657067,0.));
#10157=DIRECTION('',(0.106006004448152,0.994365489657067,0.));
#10158=DIRECTION('center_axis',(-0.106006004448152,-0.994365489657067,0.));
#10159=DIRECTION('ref_axis',(0.,0.,-1.));
#10160=DIRECTION('',(-0.106006004448152,-0.994365489657067,0.));
#10161=DIRECTION('',(-0.106006004448152,-0.994365489657067,0.));
#10162=DIRECTION('center_axis',(-0.106006004448152,-0.994365489657067,0.));
#10163=DIRECTION('ref_axis',(0.994365489657067,-0.106006004448152,-4.06725102863337E-14));
#10164=DIRECTION('',(-0.106006004448152,-0.994365489657067,0.));
#10165=DIRECTION('',(-0.106006004448152,-0.994365489657067,0.));
#10166=DIRECTION('center_axis',(-0.106006004448152,-0.994365489657067,0.));
#10167=DIRECTION('ref_axis',(0.994365489657067,-0.106006004448152,5.51276753807285E-15));
#10168=DIRECTION('',(-0.106006004448152,-0.994365489657067,0.));
#10169=DIRECTION('center_axis',(-0.106006004448152,-0.994365489657067,0.));
#10170=DIRECTION('ref_axis',(0.,0.,-1.));
#10171=DIRECTION('',(-0.106006004448152,-0.994365489657067,0.));
#10172=DIRECTION('center_axis',(-0.106006004448152,-0.994365489657067,0.));
#10173=DIRECTION('ref_axis',(0.,0.,-1.));
#10174=DIRECTION('',(-0.106006004448152,-0.994365489657067,0.));
#10175=DIRECTION('',(-0.104595521960225,-0.994514394606886,0.000946417226730482));
#10176=DIRECTION('center_axis',(-0.106006004448152,-0.994365489657067,0.));
#10177=DIRECTION('ref_axis',(0.,0.,-1.));
#10178=DIRECTION('',(-0.106006004448152,-0.994365489657067,0.));
#10179=DIRECTION('',(-0.104644914852541,-0.994509228045758,0.000914946629410067));
#10180=DIRECTION('center_axis',(-0.106006004448152,-0.994365489657067,0.));
#10181=DIRECTION('ref_axis',(0.,0.,-1.));
#10182=DIRECTION('',(-0.106006004448152,-0.994365489657067,0.));
#10183=DIRECTION('',(-0.104789157575189,-0.994494123194127,0.000819382100487921));
#10184=DIRECTION('center_axis',(-0.106006004448152,-0.994365489657067,0.));
#10185=DIRECTION('ref_axis',(0.,0.,-1.));
#10186=DIRECTION('',(-0.106006004448152,-0.994365489657067,0.));
#10187=DIRECTION('',(-0.105011768308297,-0.994470753208597,0.000670469604745426));
#10188=DIRECTION('center_axis',(-0.106006004448152,-0.994365489657067,0.));
#10189=DIRECTION('ref_axis',(0.,0.,-1.));
#10190=DIRECTION('',(-0.106006004448152,-0.994365489657067,0.));
#10191=DIRECTION('',(-0.105293840413202,-0.994441036965239,0.000480801975987768));
#10192=DIRECTION('center_axis',(-0.106006004448152,-0.994365489657067,0.));
#10193=DIRECTION('ref_axis',(0.,0.,-1.));
#10194=DIRECTION('',(-0.106006004448152,-0.994365489657067,0.));
#10195=DIRECTION('',(-0.10561478582907,-0.994407083215312,0.000264320818382655));
#10196=DIRECTION('center_axis',(-0.106006004448152,-0.994365489657067,0.));
#10197=DIRECTION('ref_axis',(0.,0.,-1.));
#10198=DIRECTION('',(-0.106006004448152,-0.994365489657067,0.));
#10199=DIRECTION('',(-0.105953253909959,-0.994371111162663,3.56514048180235E-5));
#10200=DIRECTION('center_axis',(0.,0.,1.));
#10201=DIRECTION('ref_axis',(0.994365489657067,-0.106006004448152,0.));
#10202=DIRECTION('center_axis',(-5.29294451150809E-11,5.6426324652942E-12,
1.));
#10203=DIRECTION('ref_axis',(0.775613864659347,0.6312076781442,3.74911385429433E-11));
#10204=DIRECTION('',(0.994365489657067,-0.106006004448152,0.));
#10205=DIRECTION('',(-0.106006004448152,-0.994365489657067,0.));
#10206=DIRECTION('center_axis',(-5.29294451147456E-11,5.64263246525919E-12,
1.));
#10207=DIRECTION('ref_axis',(0.775613853926467,0.631207691332523,3.7491137900203E-11));
#10208=DIRECTION('',(-0.106006004448152,-0.994365489657067,0.));
#10209=DIRECTION('center_axis',(-4.940081544063E-11,5.26645696759596E-12,
1.));
#10210=DIRECTION('ref_axis',(0.775613813195398,0.631207741381943,3.49917264312677E-11));
#10211=DIRECTION('',(-0.106006004448152,-0.994365489657067,0.));
#10212=DIRECTION('center_axis',(-5.1157602968305E-11,5.52519915316751E-12,
1.));
#10213=DIRECTION('ref_axis',(0.775613834257577,0.631207715501212,3.61909962545137E-11));
#10214=DIRECTION('',(-0.106006004448152,-0.994365489657067,0.));
#10215=DIRECTION('center_axis',(-5.4686232642848E-11,5.90137465087394E-12,
1.));
#10216=DIRECTION('ref_axis',(0.7756138251515,0.631207726690555,3.86904048055168E-11));
#10217=DIRECTION('',(-0.106006004448152,-0.994365489657067,0.));
#10218=DIRECTION('center_axis',(-5.64580747891702E-11,6.01880796295792E-12,
1.));
#10219=DIRECTION('ref_axis',(0.775613814734935,0.631207739490195,3.99905445910943E-11));
#10220=DIRECTION('',(-0.106006004448152,-0.994365489657067,0.));
#10221=DIRECTION('center_axis',(-5.46862326427878E-11,5.90137465086926E-12,
1.));
#10222=DIRECTION('ref_axis',(0.775613821569081,0.631207731092551,3.86904045835862E-11));
#10223=DIRECTION('',(-0.106006004448152,-0.994365489657067,0.));
#10224=DIRECTION('',(0.994365489657067,-0.106006004448152,0.));
#10225=DIRECTION('',(0.106006004448152,0.994365489657067,0.));
#10226=DIRECTION('center_axis',(0.,0.,1.));
#10227=DIRECTION('ref_axis',(0.994365489657067,-0.106006004448152,0.));
#10228=DIRECTION('',(-0.0682742201674492,0.997666593036234,0.));
#10229=DIRECTION('center_axis',(0.,0.,-1.));
#10230=DIRECTION('ref_axis',(0.994365489657067,-0.106006004448152,0.));
#10231=DIRECTION('',(-0.992147762966023,-0.125071245462399,0.));
#10232=DIRECTION('',(0.994365489657067,-0.106006004448152,0.));
#10233=DIRECTION('center_axis',(-4.94008154407823E-11,5.26645696761484E-12,
1.));
#10234=DIRECTION('ref_axis',(0.775613862100156,0.631207681288877,3.49917291637863E-11));
#10235=DIRECTION('center_axis',(-4.94008154408169E-11,5.266456967615E-12,
1.));
#10236=DIRECTION('ref_axis',(0.775613846609227,0.631207700323783,3.49917282983021E-11));
#10237=DIRECTION('',(0.105718986639004,0.994396026866766,0.000193947443827362));
#10238=DIRECTION('',(0.105390335156554,0.99443084444827,0.000415770959693973));
#10239=DIRECTION('',(0.105093973279893,0.994462104966823,0.000615276524171631));
#10240=DIRECTION('',(0.104850811522338,0.994487657870431,0.000778245777930233));
#10241=DIRECTION('',(0.104680345174056,0.994505520521614,0.000891620028430924));
#10242=DIRECTION('',(0.104599853734027,0.994513941261197,0.000944052933083771));
#10243=DIRECTION('center_axis',(-0.106006004448152,-0.994365489657067,0.));
#10244=DIRECTION('ref_axis',(0.00297357138932237,-0.00031700257621784,0.999995528681283));
#10245=DIRECTION('center_axis',(-0.106006004448152,-0.994365489657067,0.));
#10246=DIRECTION('ref_axis',(0.0028493267959079,-0.000303757272494865,0.999995894525737));
#10247=DIRECTION('center_axis',(-0.106006004448152,-0.994365489657067,0.));
#10248=DIRECTION('ref_axis',(0.00262933317937824,-0.000280304483218709,
0.999996504012103));
#10249=DIRECTION('center_axis',(-0.106006004448152,-0.994365489657067,0.));
#10250=DIRECTION('ref_axis',(0.00232579287797141,-0.000247945059168078,
0.999997264601627));
#10251=DIRECTION('center_axis',(-0.106006004448152,-0.994365489657067,0.));
#10252=DIRECTION('ref_axis',(0.00195706334323466,-0.000208636027322103,
0.999998063185164));
#10253=DIRECTION('center_axis',(-0.106006004448152,-0.994365489657067,0.));
#10254=DIRECTION('ref_axis',(0.00154710569925948,-0.000164931803590671,
0.999998789629995));
#10255=DIRECTION('center_axis',(-0.106006004448152,-0.994365489657067,0.));
#10256=DIRECTION('ref_axis',(-0.164515306403286,0.0175384307719592,0.986218595142624));
#10257=DIRECTION('center_axis',(-0.106006004448152,-0.994365489657067,0.));
#10258=DIRECTION('ref_axis',(0.,0.,-1.));
#10259=DIRECTION('center_axis',(-0.106006004448152,-0.994365489657067,0.));
#10260=DIRECTION('ref_axis',(0.,0.,-1.));
#10261=DIRECTION('',(0.,0.,-1.));
#10262=DIRECTION('center_axis',(0.,0.,1.));
#10263=DIRECTION('ref_axis',(0.994365489657067,-0.106006004448152,0.));
#10264=DIRECTION('',(-0.992147762966023,-0.125071245462401,0.));
#10265=DIRECTION('center_axis',(0.,0.,-1.));
#10266=DIRECTION('ref_axis',(0.994365489657067,-0.106006004448152,0.));
#10267=DIRECTION('center_axis',(0.,0.,-1.));
#10268=DIRECTION('ref_axis',(0.994365489657067,-0.10600600444815,0.));
#10269=DIRECTION('center_axis',(0.,0.,1.));
#10270=DIRECTION('ref_axis',(0.994365489657067,-0.106006004448152,0.));
#10271=DIRECTION('',(-0.125071245462401,0.992147762966023,0.));
#10272=DIRECTION('center_axis',(0.125071245462402,-0.992147762966023,0.));
#10273=DIRECTION('ref_axis',(0.992147762966023,0.125071245462402,0.));
#10274=DIRECTION('',(-0.992147762966023,-0.125071245462401,0.));
#10275=DIRECTION('center_axis',(0.125071245462402,-0.992147762966023,0.));
#10276=DIRECTION('ref_axis',(0.992147762966023,0.125071245462401,0.));
#10277=DIRECTION('',(0.,0.,-1.));
#10278=DIRECTION('',(-0.992147762966023,-0.125071245462401,0.));
#10279=DIRECTION('center_axis',(0.125071245462402,-0.992147762966023,0.));
#10280=DIRECTION('ref_axis',(0.992147762966023,0.125071245462401,0.));
#10281=DIRECTION('',(0.992147762966023,0.125071245462401,0.));
#10282=DIRECTION('',(0.,0.,-1.));
#10283=DIRECTION('center_axis',(0.997666593036234,0.0682742201674492,0.));
#10284=DIRECTION('ref_axis',(-0.0682742201674492,0.997666593036234,0.));
#10285=DIRECTION('',(0.0682742201674492,-0.997666593036234,0.));
#10286=DIRECTION('',(0.,0.,1.));
#10287=DIRECTION('',(0.0682742201674492,-0.997666593036234,0.));
#10288=DIRECTION('center_axis',(0.994365489657067,-0.106006004448152,0.));
#10289=DIRECTION('ref_axis',(0.,0.,-1.));
#10290=DIRECTION('',(0.,0.,-1.));
#10291=DIRECTION('',(-0.106006004448152,-0.994365489657067,0.));
#10292=DIRECTION('',(0.,0.,-1.));
#10293=DIRECTION('',(-0.106006004448152,-0.994365489657067,0.));
#10294=DIRECTION('center_axis',(0.106006004448152,0.994365489657067,0.));
#10295=DIRECTION('ref_axis',(0.,0.,1.));
#10296=DIRECTION('',(0.994365489657067,-0.106006004448152,0.));
#10297=DIRECTION('center_axis',(-0.106006004448152,-0.994365489657067,0.));
#10298=DIRECTION('ref_axis',(0.,0.,1.));
#10299=DIRECTION('',(0.994365489657067,-0.106006004448152,0.));
#10300=DIRECTION('center_axis',(-0.106006004448152,-0.994365489657067,0.));
#10301=DIRECTION('ref_axis',(0.,0.,1.));
#10302=DIRECTION('',(0.,0.,-1.));
#10303=DIRECTION('center_axis',(-0.106006004448152,-0.994365489657067,0.));
#10304=DIRECTION('ref_axis',(0.,0.,1.));
#10305=DIRECTION('',(0.994365489657067,-0.106006004448152,0.));
#10306=DIRECTION('center_axis',(-0.106006004448152,-0.994365489657067,0.));
#10307=DIRECTION('ref_axis',(0.,0.,1.));
#10308=DIRECTION('',(0.,0.,-1.));
#10309=DIRECTION('center_axis',(-0.106006004448152,-0.994365489657067,0.));
#10310=DIRECTION('ref_axis',(0.,0.,1.));
#10311=DIRECTION('center_axis',(-0.106006004448152,-0.994365489657067,0.));
#10312=DIRECTION('ref_axis',(0.990000482593489,-0.105540665533024,-0.093596006236942));
#10313=DIRECTION('',(0.,0.,-1.));
#10314=DIRECTION('center_axis',(-0.106006004448152,-0.994365489657067,0.));
#10315=DIRECTION('ref_axis',(0.,0.,1.));
#10316=DIRECTION('center_axis',(0.,0.,1.));
#10317=DIRECTION('ref_axis',(0.994365489657067,-0.106006004448152,0.));
#10318=DIRECTION('',(0.,0.,1.));
#10319=DIRECTION('center_axis',(0.,0.,-1.));
#10320=DIRECTION('ref_axis',(0.994365489657065,-0.106006004448171,0.));
#10321=DIRECTION('',(0.,0.,-1.));
#10322=DIRECTION('center_axis',(0.,0.,1.));
#10323=DIRECTION('ref_axis',(0.994365489657067,-0.106006004448152,0.));
#10324=DIRECTION('',(0.,0.,1.));
#10325=DIRECTION('center_axis',(0.997666593036234,0.0682742201674492,0.));
#10326=DIRECTION('ref_axis',(-0.0682742201674492,0.997666593036234,0.));
#10327=DIRECTION('',(0.0682742201674492,-0.997666593036234,0.));
#10328=DIRECTION('',(-0.0682742201674492,0.997666593036234,0.));
#10329=DIRECTION('center_axis',(0.994365489657067,-0.106006004448152,0.));
#10330=DIRECTION('ref_axis',(0.,0.,-1.));
#10331=DIRECTION('',(-0.106006004448152,-0.994365489657067,0.));
#10332=DIRECTION('',(0.106006004448152,0.994365489657067,0.));
#10333=DIRECTION('center_axis',(0.,0.,1.));
#10334=DIRECTION('ref_axis',(0.994365489657067,-0.106006004448152,0.));
#10335=DIRECTION('',(-0.992147762966023,-0.125071245462401,0.));
#10336=DIRECTION('center_axis',(0.,0.,1.));
#10337=DIRECTION('ref_axis',(0.994365489657067,-0.106006004448152,0.));
#10338=DIRECTION('',(0.0682742201674492,-0.997666593036234,0.));
#10339=DIRECTION('center_axis',(0.,0.,-1.));
#10340=DIRECTION('ref_axis',(0.994365489657065,-0.106006004448169,0.));
#10341=DIRECTION('',(-0.106006004448152,-0.994365489657067,0.));
#10342=DIRECTION('center_axis',(0.,0.,1.));
#10343=DIRECTION('ref_axis',(0.994365489657067,-0.106006004448152,0.));
#10344=DIRECTION('',(0.106006004448152,0.994365489657067,0.));
#10345=DIRECTION('center_axis',(0.,0.,1.));
#10346=DIRECTION('ref_axis',(0.994365489657067,-0.106006004448152,0.));
#10347=DIRECTION('',(-0.0682742201674492,0.997666593036234,0.));
#10348=DIRECTION('center_axis',(0.,0.,-1.));
#10349=DIRECTION('ref_axis',(0.994365489657067,-0.106006004448152,0.));
#10350=DIRECTION('',(0.992147762966023,0.125071245462401,0.));
#10351=DIRECTION('center_axis',(0.,0.,1.));
#10352=DIRECTION('ref_axis',(0.994365489657067,-0.106006004448152,0.));
#10353=DIRECTION('center_axis',(0.,0.,-1.));
#10354=DIRECTION('ref_axis',(0.994365489657065,-0.106006004448171,0.));
#10355=DIRECTION('center_axis',(0.,0.,1.));
#10356=DIRECTION('ref_axis',(0.994365489657067,-0.106006004448152,0.));
#10357=DIRECTION('',(-0.106092348033695,-0.994356281062627,0.));
#10358=DIRECTION('center_axis',(0.,0.,1.));
#10359=DIRECTION('ref_axis',(0.994365489657067,-0.106006004448152,0.));
#10360=DIRECTION('center_axis',(4.31480997391025E-8,-4.59987570007986E-9,
0.999999999999999));
#10361=DIRECTION('ref_axis',(0.551662933371381,-0.834067148342435,-2.76398124793695E-8));
#10362=DIRECTION('center_axis',(4.31463281213693E-8,-4.59975829069094E-9,
0.999999999999999));
#10363=DIRECTION('ref_axis',(0.551662908720544,-0.834067164646822,-2.76387362276229E-8));
#10364=DIRECTION('center_axis',(4.31480997391815E-8,-4.59987570008751E-9,
0.999999999999999));
#10365=DIRECTION('ref_axis',(0.551662934443112,-0.834067147633579,-2.7639812522402E-8));
#10366=DIRECTION('',(0.994365489657067,-0.106006004448152,0.));
#10367=DIRECTION('',(-0.992147762966023,-0.125071245462399,0.));
#10368=DIRECTION('center_axis',(7.37052354886326E-6,-1.28250520570221E-6,
0.999999999972015));
#10369=DIRECTION('ref_axis',(0.8981791063997,-0.43962972235215,-7.18387766251503E-6));
#10370=DIRECTION('center_axis',(4.31480997391323E-8,-4.59987570008457E-9,
0.999999999999999));
#10371=DIRECTION('ref_axis',(0.55166291981908,-0.834067157306105,-2.76398119358656E-8));
#10372=DIRECTION('center_axis',(4.31445711081758E-8,-4.59949952444789E-9,
0.999999999999999));
#10373=DIRECTION('ref_axis',(0.551662901360848,-0.83406716951462,-2.76375508250458E-8));
#10374=DIRECTION('center_axis',(4.3144571108166E-8,-4.59949952444854E-9,
0.999999999999999));
#10375=DIRECTION('ref_axis',(0.551662893412369,-0.834067174771848,-2.76375505062878E-8));
#10376=DIRECTION('center_axis',(4.31480851344174E-8,-4.60001705691756E-9,
0.999999999999999));
#10377=DIRECTION('ref_axis',(0.55166290335284,-0.834067168197091,-2.76399211196898E-8));
#10378=DIRECTION('center_axis',(4.31480997391094E-8,-4.59987570007966E-9,
0.999999999999999));
#10379=DIRECTION('ref_axis',(0.551662947457436,-0.834067139025734,-2.7639813044304E-8));
#10380=DIRECTION('center_axis',(4.31498421474835E-8,-4.60027582314505E-9,
0.999999999999999));
#10381=DIRECTION('ref_axis',(0.551662900079072,-0.834067170362404,-2.76411060957321E-8));
#10382=DIRECTION('',(0.994365489657067,-0.106006004448152,0.));
#10383=DIRECTION('',(-0.106006004448152,-0.994365489657067,0.));
#10384=DIRECTION('center_axis',(0.10614193441841,0.994350989134504,-1.28511006137957E-5));
#10385=DIRECTION('ref_axis',(0.261552703869028,-0.0279069580928212,0.964785667798193));
#10386=DIRECTION('center_axis',(0.125071245462399,-0.992147762966023,0.));
#10387=DIRECTION('ref_axis',(0.992147762966023,0.125071245462399,0.));
#10388=DIRECTION('center_axis',(0.,0.,1.));
#10389=DIRECTION('ref_axis',(0.994365489657067,-0.106006004448152,0.));
#10390=DIRECTION('center_axis',(0.,0.,-1.));
#10391=DIRECTION('ref_axis',(0.994365489657067,-0.106006004448151,0.));
#10392=DIRECTION('center_axis',(0.,0.,1.));
#10393=DIRECTION('ref_axis',(0.994365489657067,-0.106006004448152,0.));
#10394=DIRECTION('center_axis',(0.,0.,1.));
#10395=DIRECTION('ref_axis',(0.994365489657067,-0.106006004448152,0.));
#10396=DIRECTION('',(0.125071245462401,-0.992147762966023,0.));
#10397=DIRECTION('center_axis',(0.,0.,-1.));
#10398=DIRECTION('ref_axis',(0.961056660210967,0.276351399244047,0.));
#10399=DIRECTION('',(0.,0.,-1.));
#10400=DIRECTION('center_axis',(0.232004772421175,0.972714647557956,0.));
#10401=DIRECTION('ref_axis',(-0.972714647557956,0.232004772421175,0.));
#10402=DIRECTION('',(0.972714647557956,-0.232004772421175,0.));
#10403=DIRECTION('',(0.972714647557956,-0.232004772421175,0.));
#10404=DIRECTION('',(0.,0.,-1.));
#10405=DIRECTION('center_axis',(-0.992147762966023,-0.125071245462401,0.));
#10406=DIRECTION('ref_axis',(0.125071245462401,-0.992147762966023,0.));
#10407=DIRECTION('',(0.,0.,1.));
#10408=DIRECTION('',(-0.125071245462401,0.992147762966023,0.));
#10409=DIRECTION('',(-0.125071245462401,0.992147762966023,0.));
#10410=DIRECTION('center_axis',(0.,0.,-1.));
#10411=DIRECTION('ref_axis',(0.884759974153376,-0.466046980610451,0.));
#10412=DIRECTION('center_axis',(0.,0.,1.));
#10413=DIRECTION('ref_axis',(0.994365489657067,-0.106006004448152,0.));
#10414=DIRECTION('center_axis',(0.,0.,-1.));
#10415=DIRECTION('ref_axis',(0.994365489657067,-0.106006004448152,0.));
#10416=DIRECTION('',(0.,0.,1.));
#10417=DIRECTION('center_axis',(0.,0.,1.));
#10418=DIRECTION('ref_axis',(0.994365489657067,-0.106006004448152,0.));
#10419=DIRECTION('center_axis',(0.,0.,1.));
#10420=DIRECTION('ref_axis',(0.994365489657067,-0.106006004448152,0.));
#10421=DIRECTION('',(0.,0.,1.));
#10422=DIRECTION('center_axis',(0.,0.,1.));
#10423=DIRECTION('ref_axis',(0.994365489657067,-0.106006004448152,0.));
#10424=DIRECTION('',(0.125071245462401,-0.992147762966023,0.));
#10425=DIRECTION('center_axis',(0.,0.,1.));
#10426=DIRECTION('ref_axis',(0.994365489657067,-0.106006004448152,0.));
#10427=DIRECTION('',(-0.789993136930247,0.61311568533443,0.));
#10428=DIRECTION('',(0.613115685334428,0.789993136930249,0.));
#10429=DIRECTION('',(-0.789993136930257,0.613115685334417,0.));
#10430=DIRECTION('',(0.613115685334426,0.78999313693025,0.));
#10431=DIRECTION('',(-0.789993136930246,0.613115685334431,0.));
#10432=DIRECTION('',(0.613115685334426,0.78999313693025,0.));
#10433=DIRECTION('',(-0.789993136930246,0.613115685334431,0.));
#10434=DIRECTION('',(0.613115685334426,0.78999313693025,0.));
#10435=DIRECTION('',(-0.789993136930246,0.613115685334431,0.));
#10436=DIRECTION('',(0.613115685334426,0.78999313693025,0.));
#10437=DIRECTION('',(-0.789993136930246,0.613115685334431,0.));
#10438=DIRECTION('',(0.613115685334426,0.78999313693025,0.));
#10439=DIRECTION('',(-0.789993136930246,0.613115685334431,0.));
#10440=DIRECTION('',(0.613115685334426,0.78999313693025,0.));
#10441=DIRECTION('',(-0.789993136930246,0.613115685334431,0.));
#10442=DIRECTION('',(0.613115685334426,0.78999313693025,0.));
#10443=DIRECTION('',(-0.789993136930246,0.613115685334431,0.));
#10444=DIRECTION('',(0.613115685334426,0.78999313693025,0.));
#10445=DIRECTION('',(0.992014908988184,0.126120657884284,0.));
#10446=DIRECTION('center_axis',(0.859225167036477,0.108314875853399,0.500000000000001));
#10447=DIRECTION('ref_axis',(0.50730728131349,-0.05408234545433,-0.860066521983314));
#10448=DIRECTION('',(-0.125071245462401,0.992147762966023,-1.16159728063882E-17));
#10449=DIRECTION('',(-0.496073881483013,-0.0625356227312008,0.866025403784438));
#10450=DIRECTION('center_axis',(0.859225167036477,0.108314875853399,-0.500000000000001));
#10451=DIRECTION('ref_axis',(-0.50730728131349,0.05408234545433,-0.860066521983314));
#10452=DIRECTION('',(0.496073881483013,0.0625356227312008,0.866025403784438));
#10453=DIRECTION('',(0.125071245462401,-0.992147762966023,-1.46206020038625E-17));
#10454=DIRECTION('',(0.125071245462401,-0.992147762966023,0.));
#10455=DIRECTION('center_axis',(0.,0.,1.));
#10456=DIRECTION('ref_axis',(0.994365489657067,-0.106006004448152,0.));
#10457=DIRECTION('',(0.992014908988184,0.126120657884284,0.));
#10458=DIRECTION('',(0.613115685334426,0.78999313693025,0.));
#10459=DIRECTION('',(-0.789993136930246,0.613115685334431,0.));
#10460=DIRECTION('',(0.613115685334426,0.78999313693025,0.));
#10461=DIRECTION('',(-0.789993136930246,0.613115685334431,0.));
#10462=DIRECTION('',(0.613115685334426,0.78999313693025,0.));
#10463=DIRECTION('',(-0.789993136930246,0.613115685334431,0.));
#10464=DIRECTION('',(0.613115685334426,0.78999313693025,0.));
#10465=DIRECTION('',(-0.789993136930246,0.613115685334431,0.));
#10466=DIRECTION('',(0.613115685334426,0.78999313693025,0.));
#10467=DIRECTION('',(-0.789993136930246,0.613115685334431,0.));
#10468=DIRECTION('',(0.613115685334426,0.78999313693025,0.));
#10469=DIRECTION('',(-0.789993136930246,0.613115685334431,0.));
#10470=DIRECTION('',(0.613115685334426,0.78999313693025,0.));
#10471=DIRECTION('',(-0.789993136930246,0.613115685334431,0.));
#10472=DIRECTION('',(0.613115685334426,0.78999313693025,0.));
#10473=DIRECTION('',(-0.789993136930257,0.613115685334417,0.));
#10474=DIRECTION('',(0.613115685334428,0.789993136930249,0.));
#10475=DIRECTION('',(-0.789993136930247,0.61311568533443,0.));
#10476=DIRECTION('center_axis',(0.,0.,-1.));
#10477=DIRECTION('ref_axis',(0.994365489657067,-0.106006004448149,0.));
#10478=DIRECTION('center_axis',(0.,0.,1.));
#10479=DIRECTION('ref_axis',(0.994365489657067,-0.106006004448152,0.));
#10480=DIRECTION('center_axis',(0.,0.,-1.));
#10481=DIRECTION('ref_axis',(-0.994365489657067,0.106006004448152,0.));
#10482=DIRECTION('center_axis',(0.,0.,-1.));
#10483=DIRECTION('ref_axis',(0.994365489657067,-0.106006004448152,0.));
#10484=DIRECTION('center_axis',(0.,0.,1.));
#10485=DIRECTION('ref_axis',(-0.994365489657067,0.106006004448152,0.));
#10486=DIRECTION('center_axis',(0.61311568533443,0.789993136930247,0.));
#10487=DIRECTION('ref_axis',(-0.789993136930247,0.61311568533443,0.));
#10488=DIRECTION('',(0.,0.,1.));
#10489=DIRECTION('center_axis',(0.789993136930249,-0.613115685334428,0.));
#10490=DIRECTION('ref_axis',(0.613115685334428,0.789993136930249,0.));
#10491=DIRECTION('',(0.,0.,1.));
#10492=DIRECTION('center_axis',(0.613115685334417,0.789993136930257,0.));
#10493=DIRECTION('ref_axis',(-0.789993136930257,0.613115685334417,0.));
#10494=DIRECTION('',(0.,0.,1.));
#10495=DIRECTION('center_axis',(0.78999313693025,-0.613115685334426,0.));
#10496=DIRECTION('ref_axis',(0.613115685334426,0.78999313693025,0.));
#10497=DIRECTION('',(0.,0.,1.));
#10498=DIRECTION('center_axis',(0.613115685334431,0.789993136930246,0.));
#10499=DIRECTION('ref_axis',(-0.789993136930246,0.613115685334431,0.));
#10500=DIRECTION('',(0.,0.,1.));
#10501=DIRECTION('center_axis',(0.78999313693025,-0.613115685334426,0.));
#10502=DIRECTION('ref_axis',(0.613115685334426,0.78999313693025,0.));
#10503=DIRECTION('',(0.,0.,1.));
#10504=DIRECTION('center_axis',(0.613115685334431,0.789993136930246,0.));
#10505=DIRECTION('ref_axis',(-0.789993136930246,0.613115685334431,0.));
#10506=DIRECTION('',(0.,0.,1.));
#10507=DIRECTION('center_axis',(0.78999313693025,-0.613115685334426,0.));
#10508=DIRECTION('ref_axis',(0.613115685334426,0.78999313693025,0.));
#10509=DIRECTION('',(0.,0.,1.));
#10510=DIRECTION('center_axis',(0.613115685334431,0.789993136930246,0.));
#10511=DIRECTION('ref_axis',(-0.789993136930246,0.613115685334431,0.));
#10512=DIRECTION('',(0.,0.,1.));
#10513=DIRECTION('center_axis',(0.78999313693025,-0.613115685334426,0.));
#10514=DIRECTION('ref_axis',(0.613115685334426,0.78999313693025,0.));
#10515=DIRECTION('',(0.,0.,1.));
#10516=DIRECTION('center_axis',(0.613115685334431,0.789993136930246,0.));
#10517=DIRECTION('ref_axis',(-0.789993136930246,0.613115685334431,0.));
#10518=DIRECTION('',(0.,0.,1.));
#10519=DIRECTION('center_axis',(0.78999313693025,-0.613115685334426,0.));
#10520=DIRECTION('ref_axis',(0.613115685334426,0.78999313693025,0.));
#10521=DIRECTION('',(0.,0.,1.));
#10522=DIRECTION('center_axis',(0.613115685334431,0.789993136930246,0.));
#10523=DIRECTION('ref_axis',(-0.789993136930246,0.613115685334431,0.));
#10524=DIRECTION('',(0.,0.,1.));
#10525=DIRECTION('center_axis',(0.78999313693025,-0.613115685334426,0.));
#10526=DIRECTION('ref_axis',(0.613115685334426,0.78999313693025,0.));
#10527=DIRECTION('',(0.,0.,1.));
#10528=DIRECTION('center_axis',(0.613115685334431,0.789993136930246,0.));
#10529=DIRECTION('ref_axis',(-0.789993136930246,0.613115685334431,0.));
#10530=DIRECTION('',(0.,0.,1.));
#10531=DIRECTION('center_axis',(0.78999313693025,-0.613115685334426,0.));
#10532=DIRECTION('ref_axis',(0.613115685334426,0.78999313693025,0.));
#10533=DIRECTION('',(0.,0.,1.));
#10534=DIRECTION('center_axis',(0.613115685334431,0.789993136930246,0.));
#10535=DIRECTION('ref_axis',(-0.789993136930246,0.613115685334431,0.));
#10536=DIRECTION('',(0.,0.,1.));
#10537=DIRECTION('center_axis',(0.78999313693025,-0.613115685334426,0.));
#10538=DIRECTION('ref_axis',(0.613115685334426,0.78999313693025,0.));
#10539=DIRECTION('',(0.,0.,1.));
#10540=DIRECTION('center_axis',(0.126120657884284,-0.992014908988184,0.));
#10541=DIRECTION('ref_axis',(0.992014908988184,0.126120657884283,0.));
#10542=DIRECTION('center_axis',(-0.125071245462401,0.992147762966023,0.));
#10543=DIRECTION('ref_axis',(-0.992147762966023,-0.125071245462401,0.));
#10544=DIRECTION('center_axis',(0.125071245462382,-0.992147762966025,0.));
#10545=DIRECTION('ref_axis',(0.992147762966025,0.125071245462382,0.));
#10546=DIRECTION('center_axis',(0.921021641733725,0.367194793699938,-0.129950448009129));
#10547=DIRECTION('ref_axis',(-0.148531324297176,0.639504090265382,0.754302965814382));
#10548=DIRECTION('center_axis',(0.,0.,1.));
#10549=DIRECTION('ref_axis',(0.994365489657067,-0.106006004448151,0.));
#10550=DIRECTION('center_axis',(0.125071245462401,-0.992147762966023,0.));
#10551=DIRECTION('ref_axis',(0.992147762966023,0.125071245462401,0.));
#10552=DIRECTION('center_axis',(0.921021641736802,0.367194793701463,0.129950447983017));
#10553=DIRECTION('ref_axis',(0.148622468696408,-0.639675044703561,0.754140039370727));
#10554=DIRECTION('center_axis',(0.125071245462387,-0.992147762966025,-1.19456606278864E-15));
#10555=DIRECTION('ref_axis',(0.992147762966025,0.125071245462387,-5.27799728148075E-30));
#10556=DIRECTION('center_axis',(0.,0.,1.));
#10557=DIRECTION('ref_axis',(0.994365489657067,-0.106006004448151,0.));
#10558=DIRECTION('center_axis',(-0.569403560671587,0.821951347323845,0.0132501972451484));
#10559=DIRECTION('ref_axis',(-0.82202351089107,-0.569453551698748,5.99549716779258E-17));
#10560=DIRECTION('center_axis',(-0.523075905343007,0.67621202355281,0.518776345309043));
#10561=DIRECTION('ref_axis',(-0.79097451855598,-0.61184909168449,-8.0247329727962E-16));
#10562=DIRECTION('center_axis',(-0.569403560671589,0.821951347323843,-0.01325019724517));
#10563=DIRECTION('ref_axis',(-0.822023510891069,-0.56945355169875,-3.009874593151E-17));
#10564=DIRECTION('center_axis',(-0.523075905342989,0.676212023552819,-0.51877634530905));
#10565=DIRECTION('ref_axis',(-0.790974518555994,-0.611849091684473,-1.07459757475795E-15));
#10566=DIRECTION('center_axis',(-0.106006004448152,-0.994365489657067,0.));
#10567=DIRECTION('ref_axis',(0.,0.,-1.));
#10568=DIRECTION('center_axis',(-0.106006004448152,-0.994365489657067,0.));
#10569=DIRECTION('ref_axis',(0.,0.,-1.));
#10570=DIRECTION('center_axis',(-0.106006004448152,-0.994365489657067,0.));
#10571=DIRECTION('ref_axis',(0.,0.,-1.));
#10572=DIRECTION('center_axis',(-0.106006004448152,-0.994365489657067,0.));
#10573=DIRECTION('ref_axis',(0.,0.,-1.));
#10574=DIRECTION('center_axis',(-0.106006004448152,-0.994365489657067,0.));
#10575=DIRECTION('ref_axis',(0.,0.,-1.));
#10576=DIRECTION('center_axis',(-0.106006004448152,-0.994365489657067,0.));
#10577=DIRECTION('ref_axis',(0.,0.,-1.));
#10578=DIRECTION('center_axis',(0.106006004448152,0.994365489657067,0.));
#10579=DIRECTION('ref_axis',(0.,0.,1.));
#10580=DIRECTION('center_axis',(0.,0.,1.));
#10581=DIRECTION('ref_axis',(0.994365489657067,-0.106006004448152,0.));
#10582=DIRECTION('center_axis',(-0.0682742201674528,0.997666593036234,0.));
#10583=DIRECTION('ref_axis',(-0.997666593036234,-0.0682742201674528,0.));
#10584=DIRECTION('center_axis',(0.0682742201674492,-0.997666593036234,0.));
#10585=DIRECTION('ref_axis',(0.997666593036234,0.0682742201674492,0.));
#10586=DIRECTION('center_axis',(-0.0682742201674521,0.997666593036234,0.));
#10587=DIRECTION('ref_axis',(-0.997666593036234,-0.0682742201674521,0.));
#10588=DIRECTION('center_axis',(0.,0.,1.));
#10589=DIRECTION('ref_axis',(-0.778213103173909,0.628000291439769,0.));
#10590=DIRECTION('center_axis',(0.106006004448152,0.994365489657067,0.));
#10591=DIRECTION('ref_axis',(0.,0.,1.));
#10592=DIRECTION('center_axis',(0.106006004448152,0.994365489657067,0.));
#10593=DIRECTION('ref_axis',(0.,0.,1.));
#10594=DIRECTION('center_axis',(0.,0.,1.));
#10595=DIRECTION('ref_axis',(0.994365489657067,-0.106006004448152,0.));
#10596=DIRECTION('center_axis',(-0.0682742201674527,0.997666593036234,0.));
#10597=DIRECTION('ref_axis',(-0.997666593036234,-0.0682742201674527,0.));
#10598=DIRECTION('center_axis',(-0.0682742201674492,0.997666593036234,0.));
#10599=DIRECTION('ref_axis',(-0.997666593036234,-0.0682742201674492,0.));
#10600=DIRECTION('center_axis',(-0.0682742201674527,0.997666593036234,-1.2049262814377E-15));
#10601=DIRECTION('ref_axis',(-0.997666593036234,-0.0682742201674527,-8.5942731427727E-31));
#10602=DIRECTION('center_axis',(0.,0.,1.));
#10603=DIRECTION('ref_axis',(-0.77217793226518,0.635406358893795,0.));
#10604=DIRECTION('center_axis',(0.992147762966023,0.125071245462401,-8.44202479736859E-16));
#10605=DIRECTION('ref_axis',(-0.125071245462401,0.992147762966023,-3.17912585643067E-30));
#10606=DIRECTION('center_axis',(0.992147762966023,0.125071245462402,0.));
#10607=DIRECTION('ref_axis',(-0.125071245462401,0.992147762966023,0.));
#10608=DIRECTION('center_axis',(0.992147762966023,0.125071245462403,1.6155123493858E-12));
#10609=DIRECTION('ref_axis',(-0.125071245462403,0.992147762966023,3.33856974702238E-27));
#10610=DIRECTION('center_axis',(0.,0.,-1.));
#10611=DIRECTION('ref_axis',(-0.994365489657067,0.106006004448149,0.));
#10612=DIRECTION('center_axis',(0.,0.,-1.));
#10613=DIRECTION('ref_axis',(0.712495620570301,0.701676557017649,0.));
#10614=DIRECTION('center_axis',(0.,0.,-1.));
#10615=DIRECTION('ref_axis',(-0.994365489657067,0.106006004448149,0.));
#10616=DIRECTION('center_axis',(-0.992147762966023,-0.125071245462403,3.37680991894744E-15));
#10617=DIRECTION('ref_axis',(0.125071245462403,-0.992147762966023,6.989343426552E-30));
#10618=DIRECTION('center_axis',(-0.992147762966023,-0.125071245462402,0.));
#10619=DIRECTION('ref_axis',(0.125071245462401,-0.992147762966023,0.));
#10620=DIRECTION('center_axis',(-0.992147762966023,-0.125071245462401,0.));
#10621=DIRECTION('ref_axis',(0.125071245462401,-0.992147762966023,0.));
#10622=DIRECTION('center_axis',(0.,0.,1.));
#10623=DIRECTION('ref_axis',(-0.77217793226518,0.635406358893796,0.));
#10624=DIRECTION('center_axis',(0.0682742201674527,-0.997666593036234,0.));
#10625=DIRECTION('ref_axis',(0.997666593036234,0.0682742201674527,0.));
#10626=DIRECTION('center_axis',(0.0682742201674492,-0.997666593036234,0.));
#10627=DIRECTION('ref_axis',(0.997666593036234,0.0682742201674492,0.));
#10628=DIRECTION('center_axis',(0.0682742201674527,-0.997666593036234,0.));
#10629=DIRECTION('ref_axis',(0.997666593036234,0.0682742201674527,0.));
#10630=DIRECTION('center_axis',(0.,0.,1.));
#10631=DIRECTION('ref_axis',(0.994365489657067,-0.106006004448152,0.));
#10632=DIRECTION('center_axis',(-0.106006004448152,-0.994365489657067,0.));
#10633=DIRECTION('ref_axis',(0.,0.,-1.));
#10634=DIRECTION('center_axis',(-0.106006004448152,-0.994365489657067,0.));
#10635=DIRECTION('ref_axis',(0.,0.,-1.));
#10636=DIRECTION('center_axis',(-0.703122551293604,0.0749575614553266,0.707106810774047));
#10637=DIRECTION('ref_axis',(0.708373355339574,-0.012663179875062,0.705724332385107));
#10638=DIRECTION('center_axis',(-0.703122551293603,0.0749575614553284,0.707106810774048));
#10639=DIRECTION('ref_axis',(0.703122610135183,-0.074957567728232,0.707106751599046));
#10640=DIRECTION('center_axis',(0.,0.,-1.));
#10641=DIRECTION('ref_axis',(-0.994365489657067,0.106006004448152,0.));
#10642=DIRECTION('center_axis',(0.,0.,1.));
#10643=DIRECTION('ref_axis',(0.994365489657067,-0.106006004448152,0.));
#10644=DIRECTION('center_axis',(0.,0.,-1.));
#10645=DIRECTION('ref_axis',(0.994365489657067,-0.106006004448153,0.));
#10646=DIRECTION('center_axis',(-0.238110783115727,-0.461122963333811,0.854791710096828));
#10647=DIRECTION('ref_axis',(-0.0922560805895924,-0.865387420522683,-0.492537742711504));
#10648=DIRECTION('center_axis',(-0.524045111191337,-0.851690508011249,-5.23133005782331E-15));
#10649=DIRECTION('ref_axis',(0.851690508011249,-0.524045111191337,-3.3077968467653E-30));
#10650=DIRECTION('center_axis',(0.,0.,1.));
#10651=DIRECTION('ref_axis',(0.994365489657067,-0.106006004448151,0.));
#10652=DIRECTION('center_axis',(-0.822883401708071,-0.56821026670886,-1.64367902233808E-15));
#10653=DIRECTION('ref_axis',(0.56821026670886,-0.822883401708071,-1.45228749875528E-30));
#10654=DIRECTION('center_axis',(0.,0.,1.));
#10655=DIRECTION('ref_axis',(0.994365489657067,-0.106006004448152,0.));
#10656=DIRECTION('center_axis',(-0.190413144371284,-0.981704046263761,0.));
#10657=DIRECTION('ref_axis',(0.981704046263761,-0.190413144371284,0.));
#10658=DIRECTION('center_axis',(0.,0.,1.));
#10659=DIRECTION('ref_axis',(-0.999462558498673,0.0327810030244038,0.));
#10660=DIRECTION('center_axis',(0.,0.,1.));
#10661=DIRECTION('ref_axis',(-0.999462558498673,0.0327810030244038,0.));
#10662=DIRECTION('center_axis',(0.190413144371284,0.981704046263761,0.));
#10663=DIRECTION('ref_axis',(-0.981704046263761,0.190413144371284,0.));
#10664=DIRECTION('center_axis',(0.,0.,1.));
#10665=DIRECTION('ref_axis',(0.994365489657067,-0.106006004448152,0.));
#10666=DIRECTION('center_axis',(0.822883401708071,0.56821026670886,1.64367902233808E-16));
#10667=DIRECTION('ref_axis',(-0.56821026670886,0.822883401708071,7.80923877284138E-31));
#10668=DIRECTION('center_axis',(0.,0.,1.));
#10669=DIRECTION('ref_axis',(0.994365489657067,-0.106006004448151,0.));
#10670=DIRECTION('center_axis',(0.524045111191337,0.851690508011249,-6.72599578862997E-15));
#10671=DIRECTION('ref_axis',(-0.851690508011249,0.524045111191337,-4.14233781763102E-30));
#10672=DIRECTION('center_axis',(0.238110783115725,0.461122963333806,0.854791710096832));
#10673=DIRECTION('ref_axis',(-0.0922560805895938,-0.865387420522686,0.492537742711499));
#15689=CARTESIAN_POINT('',(0.,0.,0.));
#15690=CARTESIAN_POINT('Origin',(-36.6843857876575,24.5637629925993,178.485485069079));
#15691=CARTESIAN_POINT('',(-41.6447424765058,23.9353829170101,177.985485069079));
#15692=CARTESIAN_POINT('',(-41.5929060189763,25.5158287144556,177.985485069079));
#15693=CARTESIAN_POINT('Origin',(-36.6843857876575,24.5637629925993,177.985485069079));
#15694=CARTESIAN_POINT('',(-41.5929060189763,25.5158287144556,173.985485069079));
#15695=CARTESIAN_POINT('',(-41.5929060189763,25.5158287144556,178.485485069079));
#15696=CARTESIAN_POINT('',(-41.6447424765058,23.9353829170101,173.985485069079));
#15697=CARTESIAN_POINT('Origin',(-36.6843857876575,24.5637629925993,173.985485069079));
#15698=CARTESIAN_POINT('',(-41.6447424765058,23.9353829170101,173.485485069079));
#15699=CARTESIAN_POINT('',(-41.6447424765058,23.9353829170101,173.985485069079));
#15700=CARTESIAN_POINT('',(-36.0590295603455,19.6030241777692,173.485485069079));
#15701=CARTESIAN_POINT('Origin',(-36.6843857876575,24.5637629925993,173.485485069079));
#15702=CARTESIAN_POINT('',(-36.0590295603455,19.6030241777692,178.485485069079));
#15703=CARTESIAN_POINT('',(-36.0590295603455,19.6030241777692,178.485485069079));
#15704=CARTESIAN_POINT('',(-41.5571272820614,23.4428748051719,178.485485069079));
#15705=CARTESIAN_POINT('Origin',(-36.6843857876575,24.5637629925993,178.485485069079));
#15706=CARTESIAN_POINT('',(-41.6447424765058,23.9353829170101,178.985485069079));
#15707=CARTESIAN_POINT('Ctrl Pts',(-41.6447424765058,23.9353829170101,178.985485069079));
#15708=CARTESIAN_POINT('Ctrl Pts',(-41.6447424765058,23.9353829170101,178.947628514448));
#15709=CARTESIAN_POINT('Ctrl Pts',(-41.6442074037926,23.931116111951,178.909894818394));
#15710=CARTESIAN_POINT('Ctrl Pts',(-41.6420233045055,23.9142225446529,178.836122709058));
#15711=CARTESIAN_POINT('Ctrl Pts',(-41.6403803832545,23.9016504746563,178.800323230855));
#15712=CARTESIAN_POINT('Ctrl Pts',(-41.6342624737586,23.8569870933521,178.707899216115));
#15713=CARTESIAN_POINT('Ctrl Pts',(-41.628662774516,23.817789652519,178.655609780093));
#15714=CARTESIAN_POINT('Ctrl Pts',(-41.61328097085,23.722137104376,178.569197903206));
#15715=CARTESIAN_POINT('Ctrl Pts',(-41.6036260582216,23.6666496809067,178.535876943855));
#15716=CARTESIAN_POINT('Ctrl Pts',(-41.5816188124318,23.5538091064277,178.495162061707));
#15717=CARTESIAN_POINT('Ctrl Pts',(-41.5699032941903,23.4984148716403,178.485485069079));
#15718=CARTESIAN_POINT('Ctrl Pts',(-41.5571272820614,23.4428748051719,178.485485069079));
#15719=CARTESIAN_POINT('',(-41.6447424765058,23.9353829170101,178.485485069079));
#15720=CARTESIAN_POINT('Origin',(-60.1632027754914,33.6789365837495,173.985485069079));
#15721=CARTESIAN_POINT('',(-28.0689593736356,55.8365434144167,173.485485069079));
#15722=CARTESIAN_POINT('',(-21.8418923193128,26.4348241521828,173.485485069079));
#15723=CARTESIAN_POINT('Origin',(-60.1632027754914,33.6789365837495,173.485485069079));
#15724=CARTESIAN_POINT('',(-27.6574947146374,56.1206152968612,173.985485069079));
#15725=CARTESIAN_POINT('Origin',(-28.0689593736356,55.8365434144167,173.985485069079));
#15726=CARTESIAN_POINT('',(-21.3209582807514,26.5004936738394,173.985485069079));
#15727=CARTESIAN_POINT('Origin',(-60.1632027754914,33.6789365837495,173.985485069079));
#15728=CARTESIAN_POINT('Ctrl Pts',(-21.8418923193129,26.4348241521828,173.485485069079));
#15729=CARTESIAN_POINT('Ctrl Pts',(-21.7765607092714,26.443059927277,173.485485069079));
#15730=CARTESIAN_POINT('Ctrl Pts',(-21.6995647127339,26.4527661278471,173.500361703275));
#15731=CARTESIAN_POINT('Ctrl Pts',(-21.5798826947022,26.4678533755469,173.548919514567));
#15732=CARTESIAN_POINT('Ctrl Pts',(-21.5156359974204,26.4759523853374,173.590627108911));
#15733=CARTESIAN_POINT('Ctrl Pts',(-21.4256203189965,26.487299861421,173.678725059264));
#15734=CARTESIAN_POINT('Ctrl Pts',(-21.3833926501498,26.4926231281084,173.740151465957));
#15735=CARTESIAN_POINT('Ctrl Pts',(-21.3355571377766,26.4986533257596,173.853335868708));
#15736=CARTESIAN_POINT('Ctrl Pts',(-21.3209582807514,26.5004936738394,173.924735228568));
#15737=CARTESIAN_POINT('Ctrl Pts',(-21.3209582807514,26.5004936738394,173.985485069079));
#15738=CARTESIAN_POINT('Origin',(-60.1632027754914,33.6789365837495,177.985485069079));
#15739=CARTESIAN_POINT('',(-27.6574947146374,56.1206152968612,177.985485069079));
#15740=CARTESIAN_POINT('',(-21.3209582807514,26.5004936738394,177.985485069079));
#15741=CARTESIAN_POINT('Origin',(-60.1632027754914,33.6789365837495,177.985485069079));
#15742=CARTESIAN_POINT('',(-28.0689593736356,55.8365434144167,178.485485069079));
#15743=CARTESIAN_POINT('Origin',(-28.0689593736356,55.8365434144167,177.985485069079));
#15744=CARTESIAN_POINT('',(-21.8418923193128,26.4348241521828,178.485485069079));
#15745=CARTESIAN_POINT('Origin',(-60.1632027754914,33.6789365837495,178.485485069079));
#15746=CARTESIAN_POINT('Ctrl Pts',(-21.3209582807514,26.5004936738394,177.985485069079));
#15747=CARTESIAN_POINT('Ctrl Pts',(-21.3209582807514,26.5004936738394,178.046234909591));
#15748=CARTESIAN_POINT('Ctrl Pts',(-21.3355571377766,26.4986533257596,178.117634269451));
#15749=CARTESIAN_POINT('Ctrl Pts',(-21.3833926501498,26.4926231281084,178.230818672202));
#15750=CARTESIAN_POINT('Ctrl Pts',(-21.4256203189965,26.487299861421,178.292245078894));
#15751=CARTESIAN_POINT('Ctrl Pts',(-21.5156359974204,26.4759523853374,178.380343029248));
#15752=CARTESIAN_POINT('Ctrl Pts',(-21.5798826947022,26.4678533755469,178.422050623592));
#15753=CARTESIAN_POINT('Ctrl Pts',(-21.6995647127339,26.4527661278471,178.470608434884));
#15754=CARTESIAN_POINT('Ctrl Pts',(-21.7765607092714,26.443059927277,178.485485069079));
#15755=CARTESIAN_POINT('Ctrl Pts',(-21.8418923193129,26.4348241521828,178.485485069079));
#15756=CARTESIAN_POINT('Origin',(-32.4121430547972,41.0900517459514,178.985485069079));
#15757=CARTESIAN_POINT('',(-33.3358320373305,35.4434146616551,178.735485069079));
#15758=CARTESIAN_POINT('',(-26.7516402862307,41.9245696338691,178.735485069079));
#15759=CARTESIAN_POINT('Origin',(-32.4121430547972,41.0900517459514,178.735485069079));
#15760=CARTESIAN_POINT('',(-33.7154041461839,35.0749167312736,178.485485069079));
#15761=CARTESIAN_POINT('Ctrl Pts',(-33.3358320373305,35.4434146616551,178.735485069079));
#15762=CARTESIAN_POINT('Ctrl Pts',(-33.3446356128532,35.4344346820991,178.717673683699));
#15763=CARTESIAN_POINT('Ctrl Pts',(-33.3542668467474,35.4246420637755,178.700821574011));
#15764=CARTESIAN_POINT('Ctrl Pts',(-33.3645777815926,35.4142026008384,178.684920753159));
#15765=CARTESIAN_POINT('Ctrl Pts',(-33.3756414866745,35.4030009842163,178.667859061362));
#15766=CARTESIAN_POINT('Ctrl Pts',(-33.3874878790304,35.3910544439032,178.65189219269));
#15767=CARTESIAN_POINT('Ctrl Pts',(-33.3999755348309,35.3785236283123,178.637015071129));
#15768=CARTESIAN_POINT('Ctrl Pts',(-33.4130084572907,35.3654456615133,178.621488348193));
#15769=CARTESIAN_POINT('Ctrl Pts',(-33.4267402497532,35.351730797418,178.607148080583));
#15770=CARTESIAN_POINT('Ctrl Pts',(-33.4410493968144,35.3375207872263,178.594001236326));
#15771=CARTESIAN_POINT('Ctrl Pts',(-33.4561591001456,35.3225157671918,178.58011886335));
#15772=CARTESIAN_POINT('Ctrl Pts',(-33.4719129905256,35.3069580905995,178.567566428292));
#15773=CARTESIAN_POINT('Ctrl Pts',(-33.4882045709165,35.2909781638283,178.55637629334));
#15774=CARTESIAN_POINT('Ctrl Pts',(-33.4908937363219,35.2883404414452,178.554529196676));
#15775=CARTESIAN_POINT('Ctrl Pts',(-33.4935976198782,35.2856911491175,178.552719283668));
#15776=CARTESIAN_POINT('Ctrl Pts',(-33.496315818567,35.2830308017146,178.550946781807));
#15777=CARTESIAN_POINT('Ctrl Pts',(-33.4979816419081,35.2814004320077,178.549860520165));
#15778=CARTESIAN_POINT('Ctrl Pts',(-33.4996535237804,35.2797653173119,178.548787729124));
#15779=CARTESIAN_POINT('Ctrl Pts',(-33.5013313549608,35.2781255722169,178.547728373383));
#15780=CARTESIAN_POINT('Ctrl Pts',(-33.5188939634074,35.2609616278402,178.536639623625));
#15781=CARTESIAN_POINT('Ctrl Pts',(-33.5370160952805,35.2433826910993,178.527077684688));
#15782=CARTESIAN_POINT('Ctrl Pts',(-33.555555321407,35.2255349949421,178.51898718902));
#15783=CARTESIAN_POINT('Ctrl Pts',(-33.5747845425526,35.2070230412065,178.510595580367));
#15784=CARTESIAN_POINT('Ctrl Pts',(-33.5944632801671,35.1882210900316,178.503786595037));
#15785=CARTESIAN_POINT('Ctrl Pts',(-33.6144624549482,35.1692666992868,178.498541410487));
#15786=CARTESIAN_POINT('Ctrl Pts',(-33.6347878405447,35.1500031394223,178.49321067061));
#15787=CARTESIAN_POINT('Ctrl Pts',(-33.6554451836208,35.1305810847787,178.48949483668));
#15788=CARTESIAN_POINT('Ctrl Pts',(-33.6763154303043,35.111133705737,178.487422973537));
#15789=CARTESIAN_POINT('Ctrl Pts',(-33.6892719921304,35.0990604814608,178.486136729856));
#15790=CARTESIAN_POINT('Ctrl Pts',(-33.7023108775159,35.0869773346724,178.485485069079));
#15791=CARTESIAN_POINT('Ctrl Pts',(-33.7154041461839,35.0749167312735,178.485485069079));
#15792=CARTESIAN_POINT('',(-26.3219838963068,41.9787334640029,178.485485070198));
#15793=CARTESIAN_POINT('Origin',(-32.4121430547972,41.0900517459514,178.485485069079));
#15794=CARTESIAN_POINT('Origin',(-26.3219553285719,41.9787349031418,178.985611152631));
#15795=CARTESIAN_POINT('Origin',(-32.4121430547972,41.0900517459514,172.985485069079));
#15796=CARTESIAN_POINT('',(-33.7154041461839,35.0749167312736,173.485485069079));
#15797=CARTESIAN_POINT('',(-26.3219838963069,41.978733464003,173.485485067961));
#15798=CARTESIAN_POINT('Origin',(-32.4121430547972,41.0900517459514,173.485485069079));
#15799=CARTESIAN_POINT('',(-33.3358320373305,35.4434146616551,173.235485069079));
#15800=CARTESIAN_POINT('Ctrl Pts',(-33.7154041461839,35.0749167312736,173.485485069079));
#15801=CARTESIAN_POINT('Ctrl Pts',(-33.6954888490377,35.0932613104929,173.485485069079));
#15802=CARTESIAN_POINT('Ctrl Pts',(-33.6757087151231,35.1116502887521,173.483968922187));
#15803=CARTESIAN_POINT('Ctrl Pts',(-33.6561598265164,35.1299705828502,173.481006046776));
#15804=CARTESIAN_POINT('Ctrl Pts',(-33.636566911742,35.1483321361909,173.478036498656));
#15805=CARTESIAN_POINT('Ctrl Pts',(-33.6172052208955,35.1666258031105,173.473613456166));
#15806=CARTESIAN_POINT('Ctrl Pts',(-33.5981739866564,35.1847410363725,173.467754726979));
#15807=CARTESIAN_POINT('Ctrl Pts',(-33.580095426628,35.2019494490188,173.462189276732));
#15808=CARTESIAN_POINT('Ctrl Pts',(-33.5623142955273,35.2189976863789,173.455327760286));
#15809=CARTESIAN_POINT('Ctrl Pts',(-33.5449309637082,35.2357800196407,173.447144659799));
#15810=CARTESIAN_POINT('Ctrl Pts',(-33.530114973709,35.2500837724746,173.440170120267));
#15811=CARTESIAN_POINT('Ctrl Pts',(-33.5155878973462,35.2641945027656,173.43223485025));
#15812=CARTESIAN_POINT('Ctrl Pts',(-33.5014276378414,35.2780331864915,173.423301327231));
#15813=CARTESIAN_POINT('Ctrl Pts',(-33.4997577343866,35.2796651668769,173.422247806923));
#15814=CARTESIAN_POINT('Ctrl Pts',(-33.4980939376313,35.2812923576261,173.421181015993));
#15815=CARTESIAN_POINT('Ctrl Pts',(-33.4964363677189,35.2829146343261,173.420100920878));
#15816=CARTESIAN_POINT('Ctrl Pts',(-33.4803968946902,35.2986125926318,173.409649381951));
#15817=CARTESIAN_POINT('Ctrl Pts',(-33.4648415796479,35.3139396402464,173.397884146828));
#15818=CARTESIAN_POINT('Ctrl Pts',(-33.4498680795511,35.3287758944578,173.384843020246));
#15819=CARTESIAN_POINT('Ctrl Pts',(-33.4355338630463,35.3429787246988,173.372358675859));
#15820=CARTESIAN_POINT('Ctrl Pts',(-33.4217324124934,35.3567323181604,173.358704431557));
#15821=CARTESIAN_POINT('Ctrl Pts',(-33.4085774472733,35.3699038956445,173.343892300498));
#15822=CARTESIAN_POINT('Ctrl Pts',(-33.3960026091048,35.3824946134848,173.329733376633));
#15823=CARTESIAN_POINT('Ctrl Pts',(-33.3840181614552,35.3945539366785,173.314515951653));
#15824=CARTESIAN_POINT('Ctrl Pts',(-33.3727549753283,35.4059333420876,173.298238618397));
#15825=CARTESIAN_POINT('Ctrl Pts',(-33.3621571222363,35.4166405492172,173.282922811249));
#15826=CARTESIAN_POINT('Ctrl Pts',(-33.352197670638,35.4267460178717,173.266668241163));
#15827=CARTESIAN_POINT('Ctrl Pts',(-33.3430175110135,35.4360922327446,173.249468987379));
#15828=CARTESIAN_POINT('Ctrl Pts',(-33.3405655228213,35.4385885737068,173.244875127476));
#15829=CARTESIAN_POINT('Ctrl Pts',(-33.3381693226984,35.4410305423009,173.240213862542));
#15830=CARTESIAN_POINT('Ctrl Pts',(-33.3358320373305,35.4434146616551,173.235485069079));
#15831=CARTESIAN_POINT('',(-26.7516402862308,41.9245696338692,173.235485069079));
#15832=CARTESIAN_POINT('Origin',(-32.4121430547972,41.0900517459514,173.235485069079));
#15833=CARTESIAN_POINT('Origin',(-26.3219553285719,41.9787349031418,172.985358985528));
#15834=CARTESIAN_POINT('Origin',(-32.4121430547972,41.0900517459514,171.985485069079));
#15835=CARTESIAN_POINT('',(-27.4666827350209,41.8265449404332,171.985485069079));
#15836=CARTESIAN_POINT('',(-32.9897423165504,36.1235254330303,171.985485177731));
#15837=CARTESIAN_POINT('Origin',(-32.4121430547972,41.0900517459514,171.985485069079));
#15838=CARTESIAN_POINT('Ctrl Pts',(-26.7516402862308,41.9245696338692,173.235485069079));
#15839=CARTESIAN_POINT('Ctrl Pts',(-26.9899986267538,41.8919790534973,172.818818009845));
#15840=CARTESIAN_POINT('Ctrl Pts',(-27.2283468751689,41.8593100351519,172.402151301397));
#15841=CARTESIAN_POINT('Ctrl Pts',(-27.4666827350209,41.8265449404332,171.985485069079));
#15842=CARTESIAN_POINT('Ctrl Pts',(-33.3358320373305,35.4434146616551,173.235485069079));
#15843=CARTESIAN_POINT('Ctrl Pts',(-33.2135131757875,35.6670237814666,172.81906058758));
#15844=CARTESIAN_POINT('Ctrl Pts',(-33.0981931871628,35.893798298462,172.402420570166));
#15845=CARTESIAN_POINT('Ctrl Pts',(-32.9897418511957,36.1235256358927,171.985485410552));
#15846=CARTESIAN_POINT('Origin',(-32.4121430547972,41.0900517459514,179.985485069079));
#15847=CARTESIAN_POINT('',(-27.4666827350209,41.8265449404332,179.985485069079));
#15848=CARTESIAN_POINT('',(-32.9897423165518,36.1235254330304,179.985484960428));
#15849=CARTESIAN_POINT('Origin',(-32.4121430547972,41.0900517459514,179.985485069079));
#15850=CARTESIAN_POINT('Ctrl Pts',(-32.9897418511957,36.1235256358926,179.985484727606));
#15851=CARTESIAN_POINT('Ctrl Pts',(-33.0981931871628,35.893798298462,179.568549567993));
#15852=CARTESIAN_POINT('Ctrl Pts',(-33.2135131757875,35.6670237814665,179.151909550578));
#15853=CARTESIAN_POINT('Ctrl Pts',(-33.3358320373305,35.4434146616551,178.735485069079));
#15854=CARTESIAN_POINT('Ctrl Pts',(-27.4666827350209,41.8265449404332,179.985485069079));
#15855=CARTESIAN_POINT('Ctrl Pts',(-27.2283468751687,41.8593100351504,179.568818836762));
#15856=CARTESIAN_POINT('Ctrl Pts',(-26.9899986267537,41.8919790534971,179.152152128314));
#15857=CARTESIAN_POINT('Ctrl Pts',(-26.7516402862307,41.9245696338691,178.735485069079));
#15858=CARTESIAN_POINT('Origin',(-38.9776940652676,8.40516957928876,165.645237852233));
#15859=CARTESIAN_POINT('',(-40.9664250445818,8.61718158818506,178.485485069079));
#15860=CARTESIAN_POINT('Origin',(-38.9776940652676,8.40516957928876,178.485485069079));
#15861=CARTESIAN_POINT('',(-40.9664250445818,8.61718158818506,180.985485069079));
#15862=CARTESIAN_POINT('',(-40.9664250445818,8.61718158818506,165.645237852233));
#15863=CARTESIAN_POINT('Origin',(-38.9776940652676,8.40516957928876,180.985485069079));
#15864=CARTESIAN_POINT('Origin',(-38.9776940652676,8.40516957928876,165.645237852233));
#15865=CARTESIAN_POINT('',(-40.9664250445818,8.61718158818506,170.985485069079));
#15866=CARTESIAN_POINT('Origin',(-38.9776940652676,8.40516957928876,170.985485069079));
#15867=CARTESIAN_POINT('',(-40.9664250445818,8.61718158818506,173.485485069079));
#15868=CARTESIAN_POINT('',(-40.9664250445818,8.61718158818506,165.645237852233));
#15869=CARTESIAN_POINT('Origin',(-38.9776940652676,8.40516957928876,173.485485069079));
#15870=CARTESIAN_POINT('Origin',(-39.4690592605811,9.0940082318961,180.985485069079));
#15871=CARTESIAN_POINT('',(-54.4340581561246,8.06989492938437,173.485485069079));
#15872=CARTESIAN_POINT('Origin',(-39.4690592605811,9.0940082318961,173.485485069079));
#15873=CARTESIAN_POINT('',(-41.3451279425171,23.9762246763865,173.526200018228));
#15874=CARTESIAN_POINT('Ctrl Pts',(-41.6447424765058,23.9353829170101,173.985485069079));
#15875=CARTESIAN_POINT('Ctrl Pts',(-41.6447424765058,23.9353829170101,173.920389070876));
#15876=CARTESIAN_POINT('Ctrl Pts',(-41.6321641038074,23.9372419809971,173.855916759188));
#15877=CARTESIAN_POINT('Ctrl Pts',(-41.5832406087156,23.944289310737,173.735462005052));
#15878=CARTESIAN_POINT('Ctrl Pts',(-41.547358159805,23.9494033791653,173.680632537013));
#15879=CARTESIAN_POINT('Ctrl Pts',(-41.4571701130823,23.9617406441373,173.588390147553));
#15880=CARTESIAN_POINT('Ctrl Pts',(-41.4038900740746,23.9688170570234,173.551685312956));
#15881=CARTESIAN_POINT('Ctrl Pts',(-41.3451279425169,23.9762246763865,173.526200018228));
#15882=CARTESIAN_POINT('',(-41.3451279425171,23.9762246763865,171.485485069079));
#15883=CARTESIAN_POINT('',(-41.3451279425171,23.9762246763865,180.985485069079));
#15884=CARTESIAN_POINT('',(-54.4340581561246,8.06989492938437,171.485485069079));
#15885=CARTESIAN_POINT('Origin',(-39.4690592605811,9.0940082318961,171.485485069079));
#15886=CARTESIAN_POINT('',(-54.4340581561246,8.06989492938437,180.985485069079));
#15887=CARTESIAN_POINT('Origin',(-39.4690592605811,9.0940082318961,180.985485069079));
#15888=CARTESIAN_POINT('',(-54.4340581561246,8.06989492938437,180.485485069079));
#15889=CARTESIAN_POINT('',(-41.3451279425171,23.9762246763865,180.485485069079));
#15890=CARTESIAN_POINT('Origin',(-39.4690592605811,9.0940082318961,180.485485069079));
#15891=CARTESIAN_POINT('',(-41.3451279425171,23.9762246763865,178.444770119931));
#15892=CARTESIAN_POINT('',(-41.3451279425171,23.9762246763865,180.985485069079));
#15893=CARTESIAN_POINT('Ctrl Pts',(-41.3451279425169,23.9762246763865,178.444770119931));
#15894=CARTESIAN_POINT('Ctrl Pts',(-41.3955883597458,23.969863580323,178.422885301067));
#15895=CARTESIAN_POINT('Ctrl Pts',(-41.4421229365782,23.9637326784515,178.392675835198));
#15896=CARTESIAN_POINT('Ctrl Pts',(-41.5305271634123,23.9517560192715,178.311515809307));
#15897=CARTESIAN_POINT('Ctrl Pts',(-41.5692848349094,23.9462751370746,178.258717426295));
#15898=CARTESIAN_POINT('Ctrl Pts',(-41.6126217111684,23.9400646596951,178.166504459593));
#15899=CARTESIAN_POINT('Ctrl Pts',(-41.6245994664793,23.9383240624959,178.131449443898));
#15900=CARTESIAN_POINT('Ctrl Pts',(-41.6406845749615,23.9359794470033,178.059314374365));
#15901=CARTESIAN_POINT('Ctrl Pts',(-41.6447424765058,23.9353829170101,178.022456793883));
#15902=CARTESIAN_POINT('Ctrl Pts',(-41.6447424765058,23.9353829170101,177.985485069079));
#15903=CARTESIAN_POINT('',(-54.4340581561246,8.06989492938437,178.985485069079));
#15904=CARTESIAN_POINT('Origin',(-39.4690592605811,9.0940082318961,178.985485069079));
#15905=CARTESIAN_POINT('',(-54.4340581561246,8.06989492938437,180.985485069079));
#15906=CARTESIAN_POINT('Origin',(-51.4899841053611,-42.5281564925371,175.985485069079));
#15907=CARTESIAN_POINT('',(-60.5935545601082,-98.4662830593508,178.485485069079));
#15908=CARTESIAN_POINT('',(-54.633706038692,-98.6988977036234,178.813912075476));
#15909=CARTESIAN_POINT('Ctrl Pts',(-60.5935545601082,-98.4662830593508,
178.485485069079));
#15910=CARTESIAN_POINT('Ctrl Pts',(-60.3880207695053,-98.4688260755358,
178.741086946021));
#15911=CARTESIAN_POINT('Ctrl Pts',(-60.152209790567,-98.4757252435905,178.970557766682));
#15912=CARTESIAN_POINT('Ctrl Pts',(-59.6240017814705,-98.4925949995657,
179.371542094559));
#15913=CARTESIAN_POINT('Ctrl Pts',(-59.3326632292186,-98.503134685847,179.539996656388));
#15914=CARTESIAN_POINT('Ctrl Pts',(-58.5298830462485,-98.5351183946245,
179.878612357701));
#15915=CARTESIAN_POINT('Ctrl Pts',(-57.9994202067562,-98.5589973863814,
179.98575755042));
#15916=CARTESIAN_POINT('Ctrl Pts',(-56.948798132757,-98.6112255589572,179.985221824441));
#15917=CARTESIAN_POINT('Ctrl Pts',(-56.4382579068318,-98.6342747561005,
179.885486106302));
#15918=CARTESIAN_POINT('Ctrl Pts',(-55.4642502766152,-98.673456639198,179.49070605567));
#15919=CARTESIAN_POINT('Ctrl Pts',(-55.0130604929058,-98.6888974774772,
179.192189168768));
#15920=CARTESIAN_POINT('Ctrl Pts',(-54.6337060386916,-98.6988977036235,
178.813912075475));
#15921=CARTESIAN_POINT('',(-54.580703036468,-98.2017149587949,178.813912075476));
#15922=CARTESIAN_POINT('',(-48.6774936648204,-42.82798676345,178.813912075476));
#15923=CARTESIAN_POINT('',(-60.5405515578841,-97.9691003145223,178.485485069079));
#15924=CARTESIAN_POINT('Ctrl Pts',(-54.580703036468,-98.2017149587947,178.813912075476));
#15925=CARTESIAN_POINT('Ctrl Pts',(-54.9600551075263,-98.1917147954715,
179.19218679238));
#15926=CARTESIAN_POINT('Ctrl Pts',(-55.4112503915159,-98.1762737685919,
179.490707319102));
#15927=CARTESIAN_POINT('Ctrl Pts',(-56.3852549043046,-98.1370920116987,
179.88548610616));
#15928=CARTESIAN_POINT('Ctrl Pts',(-56.8957951303142,-98.1140428141397,
179.985221824425));
#15929=CARTESIAN_POINT('Ctrl Pts',(-57.946417204408,-98.0618146415591,179.985757550436));
#15930=CARTESIAN_POINT('Ctrl Pts',(-58.4768800438985,-98.0379356498009,
179.878612357734));
#15931=CARTESIAN_POINT('Ctrl Pts',(-59.279658681122,-98.005952002607,179.539997308455));
#15932=CARTESIAN_POINT('Ctrl Pts',(-59.5709958684452,-97.9954123600177,
179.371543778558));
#15933=CARTESIAN_POINT('Ctrl Pts',(-60.099201714192,-97.9785426487718,178.970562132848));
#15934=CARTESIAN_POINT('Ctrl Pts',(-60.335018812839,-97.9716433177709,178.741085645765));
#15935=CARTESIAN_POINT('Ctrl Pts',(-60.5405515578841,-97.9691003145223,
178.485485069079));
#15936=CARTESIAN_POINT('',(-54.5948893516535,-42.1971528497386,178.485485069079));
#15937=CARTESIAN_POINT('',(-54.5948893516535,-42.1971528497386,178.485485069079));
#15938=CARTESIAN_POINT('',(-48.3850788590687,-42.8591601353355,178.485485069079));
#15939=CARTESIAN_POINT('Origin',(-51.4899841053611,-42.5281564925371,175.985485069079));
#15940=CARTESIAN_POINT('',(-50.7024802268255,-64.597022606232,178.485485069079));
#15941=CARTESIAN_POINT('',(-48.3850788590687,-42.8591601353355,178.485485069079));
#15942=CARTESIAN_POINT('',(-51.1888180761633,-76.238457947575,176.985485069122));
#15943=CARTESIAN_POINT('Ctrl Pts',(-51.1888180761633,-76.238457947575,176.985485069122));
#15944=CARTESIAN_POINT('Ctrl Pts',(-51.2021305879066,-76.3214937428782,
177.002667010649));
#15945=CARTESIAN_POINT('Ctrl Pts',(-51.2156898705536,-76.4043562432359,
177.020272310541));
#15946=CARTESIAN_POINT('Ctrl Pts',(-51.2295466744237,-76.4869415706103,
177.038591562764));
#15947=CARTESIAN_POINT('Ctrl Pts',(-51.2428693654739,-76.5663436327459,
177.056204696349));
#15948=CARTESIAN_POINT('Ctrl Pts',(-51.2564667204762,-76.6454895294908,
177.074478125875));
#15949=CARTESIAN_POINT('Ctrl Pts',(-51.2704287680282,-76.7242798841604,
177.093677810158));
#15950=CARTESIAN_POINT('Ctrl Pts',(-51.2834506181271,-76.7977645348837,
177.111584597091));
#15951=CARTESIAN_POINT('Ctrl Pts',(-51.2967895433251,-76.8709399358143,
177.130297444209));
#15952=CARTESIAN_POINT('Ctrl Pts',(-51.3105617329162,-76.9437187503107,
177.15003421173));
#15953=CARTESIAN_POINT('Ctrl Pts',(-51.3223585263326,-77.0060586298211,
177.166940061566));
#15954=CARTESIAN_POINT('Ctrl Pts',(-51.3344736028237,-77.0681074686509,
177.184597395297));
#15955=CARTESIAN_POINT('Ctrl Pts',(-51.3470101229251,-77.1298057199427,
177.20314103713));
#15956=CARTESIAN_POINT('Ctrl Pts',(-51.3557988119162,-77.1730590898982,
177.216141000399));
#15957=CARTESIAN_POINT('Ctrl Pts',(-51.364781415635,-77.2161774090964,177.229465123715));
#15958=CARTESIAN_POINT('Ctrl Pts',(-51.3740444012484,-77.2590260001929,
177.243492025122));
#15959=CARTESIAN_POINT('Ctrl Pts',(-51.3828789589595,-77.2998927754084,
177.256870159901));
#15960=CARTESIAN_POINT('Ctrl Pts',(-51.3919681872068,-77.3405142529802,
177.270887849947));
#15961=CARTESIAN_POINT('Ctrl Pts',(-51.401432215628,-77.3807665395897,177.285874813254));
#15962=CARTESIAN_POINT('Ctrl Pts',(-51.4101714388937,-77.4179360940314,
177.299713995956));
#15963=CARTESIAN_POINT('Ctrl Pts',(-51.4192300650648,-77.4547908693569,
177.314379973633));
#15964=CARTESIAN_POINT('Ctrl Pts',(-51.4287456836206,-77.4912266116723,
177.330129441093));
#15965=CARTESIAN_POINT('Ctrl Pts',(-51.4345017021272,-77.5132666720046,
177.339656328456));
#15966=CARTESIAN_POINT('Ctrl Pts',(-51.4404257743927,-77.5351532749502,
177.349579610017));
#15967=CARTESIAN_POINT('Ctrl Pts',(-51.4465575779221,-77.5568619102505,
177.359954660612));
#15968=CARTESIAN_POINT('Ctrl Pts',(-51.4526736736208,-77.5785149345768,
177.370303133458));
#15969=CARTESIAN_POINT('Ctrl Pts',(-51.4590189397432,-77.6002653389843,
177.38103395459));
#15970=CARTESIAN_POINT('Ctrl Pts',(-51.4656713009053,-77.6215697467313,
177.392576424021));
#15971=CARTESIAN_POINT('Ctrl Pts',(-51.4719423749727,-77.6416530698833,
177.403457324646));
#15972=CARTESIAN_POINT('Ctrl Pts',(-51.4784859081488,-77.6613401262172,
177.415059786582));
#15973=CARTESIAN_POINT('Ctrl Pts',(-51.485411326381,-77.6801687747737,177.427738660107));
#15974=CARTESIAN_POINT('Ctrl Pts',(-51.491747978897,-77.6973967022792,177.439339636846));
#15975=CARTESIAN_POINT('Ctrl Pts',(-51.4984041162443,-77.7139060095734,
177.4518420813));
#15976=CARTESIAN_POINT('Ctrl Pts',(-51.5055059785157,-77.7293360108029,
177.465509726159));
#15977=CARTESIAN_POINT('Ctrl Pts',(-51.5084960109055,-77.7358323636871,
177.471264090192));
#15978=CARTESIAN_POINT('Ctrl Pts',(-51.5115656173302,-77.7421373112703,
177.47722486705));
#15979=CARTESIAN_POINT('Ctrl Pts',(-51.5147269509126,-77.7482235053492,
177.483411011986));
#15980=CARTESIAN_POINT('Ctrl Pts',(-51.5232794127367,-77.7646886904234,
177.500146597468));
#15981=CARTESIAN_POINT('Ctrl Pts',(-51.5327381680121,-77.7794241002675,
177.519242344142));
#15982=CARTESIAN_POINT('Ctrl Pts',(-51.5425320619611,-77.7882308246434,
177.540116101265));
#15983=CARTESIAN_POINT('Ctrl Pts',(-51.5485309012701,-77.7936250145994,
177.552901446441));
#15984=CARTESIAN_POINT('Ctrl Pts',(-51.5546552639884,-77.7967949768587,
177.566353184388));
#15985=CARTESIAN_POINT('Ctrl Pts',(-51.5607652634837,-77.7967769698663,
177.580332016632));
#15986=CARTESIAN_POINT('Ctrl Pts',(-51.5673406412735,-77.7967575913413,
177.595375569931));
#15987=CARTESIAN_POINT('Ctrl Pts',(-51.5734029435428,-77.7927425070794,
177.609994002081));
#15988=CARTESIAN_POINT('Ctrl Pts',(-51.5789129584608,-77.786000814162,177.623796257218));
#15989=CARTESIAN_POINT('Ctrl Pts',(-51.5850074273648,-77.7785440216746,
177.639062534351));
#15990=CARTESIAN_POINT('Ctrl Pts',(-51.5904257027035,-77.7677515886449,
177.653329863453));
#15991=CARTESIAN_POINT('Ctrl Pts',(-51.5950548021663,-77.7553505852216,
177.666095526557));
#15992=CARTESIAN_POINT('Ctrl Pts',(-51.5964787378413,-77.7515359704523,
177.670022312588));
#15993=CARTESIAN_POINT('Ctrl Pts',(-51.5978276539958,-77.7475692084199,
177.673807202938));
#15994=CARTESIAN_POINT('Ctrl Pts',(-51.5990975017122,-77.7435006940469,
177.677436042246));
#15995=CARTESIAN_POINT('Ctrl Pts',(-51.6038775271175,-77.7281857851694,
177.691095903863));
#15996=CARTESIAN_POINT('Ctrl Pts',(-51.6079935240033,-77.7117519853323,
177.703326388188));
#15997=CARTESIAN_POINT('Ctrl Pts',(-51.6115435129349,-77.6945144134463,
177.714453362138));
#15998=CARTESIAN_POINT('Ctrl Pts',(-51.6153029287069,-77.6762599341032,
177.726236757007));
#15999=CARTESIAN_POINT('Ctrl Pts',(-51.618428308146,-77.6571039402551,177.736782793592));
#16000=CARTESIAN_POINT('Ctrl Pts',(-51.6210961780892,-77.6374112528145,
177.746464371838));
#16001=CARTESIAN_POINT('Ctrl Pts',(-51.6240034009094,-77.6159517995671,
177.757014550748));
#16002=CARTESIAN_POINT('Ctrl Pts',(-51.6263678480769,-77.5938549565873,
177.766538360512));
#16003=CARTESIAN_POINT('Ctrl Pts',(-51.6284773090603,-77.5715834420731,
177.775499096543));
#16004=CARTESIAN_POINT('Ctrl Pts',(-51.62958722901,-77.5598649990846,177.780213902724));
#16005=CARTESIAN_POINT('Ctrl Pts',(-51.6306274481688,-77.5480980575388,
177.784772501055));
#16006=CARTESIAN_POINT('Ctrl Pts',(-51.6316450558895,-77.5363491979955,
177.789240317579));
#16007=CARTESIAN_POINT('Ctrl Pts',(-51.6345785013937,-77.5024809022792,
177.802119638392));
#16008=CARTESIAN_POINT('Ctrl Pts',(-51.6369806567888,-77.4682654516565,
177.8138359583));
#16009=CARTESIAN_POINT('Ctrl Pts',(-51.6389709535977,-77.4337999799066,
177.824711738984));
#16010=CARTESIAN_POINT('Ctrl Pts',(-51.6411016541027,-77.3969031724893,
177.836354741822));
#16011=CARTESIAN_POINT('Ctrl Pts',(-51.642760815162,-77.3597197547319,177.847034606129));
#16012=CARTESIAN_POINT('Ctrl Pts',(-51.6441487479128,-77.3223603097426,
177.857125713464));
#16013=CARTESIAN_POINT('Ctrl Pts',(-51.6442939346125,-77.318452271319,177.858181308247));
#16014=CARTESIAN_POINT('Ctrl Pts',(-51.6444361951343,-77.314542299998,177.859230441347));
#16015=CARTESIAN_POINT('Ctrl Pts',(-51.6445757869095,-77.3106305178212,
177.860273527955));
#16016=CARTESIAN_POINT('Ctrl Pts',(-51.646532188841,-77.2558062404107,177.874892560132));
#16017=CARTESIAN_POINT('Ctrl Pts',(-51.6479312585446,-77.2005791231423,
177.888296102344));
#16018=CARTESIAN_POINT('Ctrl Pts',(-51.6488633782082,-77.1450897561686,
177.900765991515));
#16019=CARTESIAN_POINT('Ctrl Pts',(-51.6498609622602,-77.085703274256,177.914111662732));
#16020=CARTESIAN_POINT('Ctrl Pts',(-51.6503241286654,-77.0260163532741,
177.926388205594));
#16021=CARTESIAN_POINT('Ctrl Pts',(-51.6504193884841,-76.966192392791,177.937917077868));
#16022=CARTESIAN_POINT('Ctrl Pts',(-51.6504826689159,-76.9264517539148,
177.945575627153));
#16023=CARTESIAN_POINT('Ctrl Pts',(-51.6503847250362,-76.8866504601454,
177.95290372211));
#16024=CARTESIAN_POINT('Ctrl Pts',(-51.6501852172071,-76.8468346421424,
177.959989646563));
#16025=CARTESIAN_POINT('Ctrl Pts',(-51.6497395509928,-76.7578929451445,
177.975818384418));
#16026=CARTESIAN_POINT('Ctrl Pts',(-51.6487423505584,-76.6688263647255,
177.990398012595));
#16027=CARTESIAN_POINT('Ctrl Pts',(-51.6472480837277,-76.5796659014834,
178.0039885827));
#16028=CARTESIAN_POINT('Ctrl Pts',(-51.6456937152051,-76.4869192683657,
178.018125786271));
#16029=CARTESIAN_POINT('Ctrl Pts',(-51.6436020909363,-76.3940709627132,
178.03119298766));
#16030=CARTESIAN_POINT('Ctrl Pts',(-51.6410857399421,-76.3011475515338,
178.043456674307));
#16031=CARTESIAN_POINT('Ctrl Pts',(-51.6384292049469,-76.2030474477577,
178.056403561614));
#16032=CARTESIAN_POINT('Ctrl Pts',(-51.6352997717696,-76.1048635740488,
178.068455130834));
#16033=CARTESIAN_POINT('Ctrl Pts',(-51.6318773801508,-76.0066192617694,
178.079892775063));
#16034=CARTESIAN_POINT('Ctrl Pts',(-51.6307428227353,-75.9740502791856,
178.083684469738));
#16035=CARTESIAN_POINT('Ctrl Pts',(-51.6295764095476,-75.9414745967699,
178.087408430568));
#16036=CARTESIAN_POINT('Ctrl Pts',(-51.6283856383612,-75.9088929032812,
178.091074131322));
#16037=CARTESIAN_POINT('Ctrl Pts',(-51.6230479302402,-75.762843375106,178.107505869769));
#16038=CARTESIAN_POINT('Ctrl Pts',(-51.617133671971,-75.6166509425742,178.122695645834));
#16039=CARTESIAN_POINT('Ctrl Pts',(-51.6106720679446,-75.4703596661805,
178.13686703474));
#16040=CARTESIAN_POINT('Ctrl Pts',(-51.603825778809,-75.3153590854994,178.151882103059));
#16041=CARTESIAN_POINT('Ctrl Pts',(-51.5963654529363,-75.1602474897245,
178.165754310024));
#16042=CARTESIAN_POINT('Ctrl Pts',(-51.5883753887386,-75.005069113572,178.178719571855));
#16043=CARTESIAN_POINT('Ctrl Pts',(-51.5799333134435,-74.8411120409846,
178.192418299912));
#16044=CARTESIAN_POINT('Ctrl Pts',(-51.5709003709617,-74.6770803555337,
178.205104877183));
#16045=CARTESIAN_POINT('Ctrl Pts',(-51.5614222526274,-74.5130183020776,
178.217019375693));
#16046=CARTESIAN_POINT('Ctrl Pts',(-51.5519949464334,-74.3498357843876,
178.228870000643));
#16047=CARTESIAN_POINT('Ctrl Pts',(-51.5421279869841,-74.1866231105131,
178.239956676937));
#16048=CARTESIAN_POINT('Ctrl Pts',(-51.5319988666506,-74.0234176542754,
178.250478142846));
#16049=CARTESIAN_POINT('Ctrl Pts',(-51.5178618990269,-73.7956357566507,
178.265162697675));
#16050=CARTESIAN_POINT('Ctrl Pts',(-51.5030623270387,-73.5678777386058,
178.278645978382));
#16051=CARTESIAN_POINT('Ctrl Pts',(-51.487657634943,-73.3401462751523,178.291141952504));
#16052=CARTESIAN_POINT('Ctrl Pts',(-51.4714916117283,-73.1011598610119,
178.304255503004));
#16053=CARTESIAN_POINT('Ctrl Pts',(-51.4546597605595,-72.8622026182683,
178.316282066724));
#16054=CARTESIAN_POINT('Ctrl Pts',(-51.4372695238474,-72.6232703614539,
178.327427903459));
#16055=CARTESIAN_POINT('Ctrl Pts',(-51.4254590327489,-72.461000730569,178.334997541971));
#16056=CARTESIAN_POINT('Ctrl Pts',(-51.4133918338923,-72.2987424737129,
178.342160074865));
#16057=CARTESIAN_POINT('Ctrl Pts',(-51.4011095455939,-72.1364927659349,
178.348969236345));
#16058=CARTESIAN_POINT('Ctrl Pts',(-51.3768673720191,-71.8162523121323,
178.362408822721));
#16059=CARTESIAN_POINT('Ctrl Pts',(-51.3517889968695,-71.4960451991844,
178.374473831145));
#16060=CARTESIAN_POINT('Ctrl Pts',(-51.325910214073,-71.175876660519,178.385374291189));
#16061=CARTESIAN_POINT('Ctrl Pts',(-51.299237757716,-70.8458889079437,178.396609056251));
#16062=CARTESIAN_POINT('Ctrl Pts',(-51.2717158347394,-70.5159420263348,
178.406606963097));
#16063=CARTESIAN_POINT('Ctrl Pts',(-51.2434204705399,-70.1860349960978,
178.415554089733));
#16064=CARTESIAN_POINT('Ctrl Pts',(-51.2138284065372,-69.8410092213846,
178.424911238918));
#16065=CARTESIAN_POINT('Ctrl Pts',(-51.1833911427243,-69.4960269329799,
178.433119311743));
#16066=CARTESIAN_POINT('Ctrl Pts',(-51.1522232776757,-69.1510812999414,
178.440340314044));
#16067=CARTESIAN_POINT('Ctrl Pts',(-51.1285558932623,-68.8891461020658,
178.445823597453));
#16068=CARTESIAN_POINT('Ctrl Pts',(-51.1044678762701,-68.6272319106942,
178.45073662802));
#16069=CARTESIAN_POINT('Ctrl Pts',(-51.0800153847959,-68.3653342504166,
178.455131374877));
#16070=CARTESIAN_POINT('Ctrl Pts',(-51.0392670697878,-67.9289006717707,
178.462454903829));
#16071=CARTESIAN_POINT('Ctrl Pts',(-50.9974328843074,-67.4925218290922,
178.468324733422));
#16072=CARTESIAN_POINT('Ctrl Pts',(-50.9545694977588,-67.0561972253282,
178.472891592671));
#16073=CARTESIAN_POINT('Ctrl Pts',(-50.909938769321,-66.601882098378,178.477646752527));
#16074=CARTESIAN_POINT('Ctrl Pts',(-50.8641932062194,-66.1476256195205,
178.480989278531));
#16075=CARTESIAN_POINT('Ctrl Pts',(-50.8174078822645,-65.6934241972506,
178.483034538648));
#16076=CARTESIAN_POINT('Ctrl Pts',(-50.8061241485162,-65.5838794194492,
178.483527816639));
#16077=CARTESIAN_POINT('Ctrl Pts',(-50.7947799440958,-65.4743378370309,
178.483945395322));
#16078=CARTESIAN_POINT('Ctrl Pts',(-50.7833763168631,-65.36479939044,178.484288448851));
#16079=CARTESIAN_POINT('Ctrl Pts',(-50.7567311311835,-65.1088569443284,
178.485090011792));
#16080=CARTESIAN_POINT('Ctrl Pts',(-50.7297618268952,-64.852931521511,178.485485016653));
#16081=CARTESIAN_POINT('Ctrl Pts',(-50.7024802268255,-64.597022606232,178.485485069074));
#16082=CARTESIAN_POINT('',(-51.1887931847522,-76.2384284136363,174.985485069079));
#16083=CARTESIAN_POINT('Ctrl Pts',(-51.1887978133155,-76.2384598819686,
176.985483211559));
#16084=CARTESIAN_POINT('Ctrl Pts',(-51.168723086379,-76.1132573740385,176.959575232915));
#16085=CARTESIAN_POINT('Ctrl Pts',(-51.1477303137464,-75.982626364191,176.931299532441));
#16086=CARTESIAN_POINT('Ctrl Pts',(-51.1263778064616,-75.8500958709827,
176.900742946067));
#16087=CARTESIAN_POINT('Ctrl Pts',(-51.1052284580587,-75.7188263419536,
176.870477090979));
#16088=CARTESIAN_POINT('Ctrl Pts',(-51.0837261817287,-75.5856934803233,
176.837973546585));
#16089=CARTESIAN_POINT('Ctrl Pts',(-51.0624157913829,-75.4540754929927,
176.803316693716));
#16090=CARTESIAN_POINT('Ctrl Pts',(-51.0406184711992,-75.3194501123587,
176.76786795222));
#16091=CARTESIAN_POINT('Ctrl Pts',(-51.0190219083614,-75.1864096200007,
176.730166374361));
#16092=CARTESIAN_POINT('Ctrl Pts',(-50.9982115787268,-75.0585136716332,
176.690302258296));
#16093=CARTESIAN_POINT('Ctrl Pts',(-50.9897004353455,-75.0062059584184,
176.673998373949));
#16094=CARTESIAN_POINT('Ctrl Pts',(-50.9813208328539,-74.9547581431755,
176.657332761972));
#16095=CARTESIAN_POINT('Ctrl Pts',(-50.9731129323308,-74.9044112818398,
176.640311599764));
#16096=CARTESIAN_POINT('Ctrl Pts',(-50.9581672362543,-74.8127351113248,
176.609317910633));
#16097=CARTESIAN_POINT('Ctrl Pts',(-50.9428274715336,-74.7188051428769,
176.575173825758));
#16098=CARTESIAN_POINT('Ctrl Pts',(-50.927879342889,-74.6274317515189,176.538057900926));
#16099=CARTESIAN_POINT('Ctrl Pts',(-50.9119396002641,-74.5299969236798,
176.498479817063));
#16100=CARTESIAN_POINT('Ctrl Pts',(-50.8964451777353,-74.4354691361771,
176.45552252949));
#16101=CARTESIAN_POINT('Ctrl Pts',(-50.8823514823103,-74.3496185699138,
176.409402537941));
#16102=CARTESIAN_POINT('Ctrl Pts',(-50.8756807371488,-74.3089842839974,
176.387573294354));
#16103=CARTESIAN_POINT('Ctrl Pts',(-50.869323829929,-74.2702930463482,176.365035522011));
#16104=CARTESIAN_POINT('Ctrl Pts',(-50.8633822358648,-74.2341528138115,
176.341812177418));
#16105=CARTESIAN_POINT('Ctrl Pts',(-50.8548047188014,-74.1819793637386,
176.308286050866));
#16106=CARTESIAN_POINT('Ctrl Pts',(-50.8459342959469,-74.1280817181684,
176.268790272864));
#16107=CARTESIAN_POINT('Ctrl Pts',(-50.8383519847354,-74.0820498566621,
176.224327986109));
#16108=CARTESIAN_POINT('Ctrl Pts',(-50.8362284960464,-74.069158254812,176.211875956592));
#16109=CARTESIAN_POINT('Ctrl Pts',(-50.8342060519672,-74.05688325133,176.199034390808));
#16110=CARTESIAN_POINT('Ctrl Pts',(-50.8323194103639,-74.0454348151833,
176.185825323489));
#16111=CARTESIAN_POINT('Ctrl Pts',(-50.827864840102,-74.018403786549,176.154637249209));
#16112=CARTESIAN_POINT('Ctrl Pts',(-50.8239090771887,-73.9944144112031,
176.119612333733));
#16113=CARTESIAN_POINT('Ctrl Pts',(-50.821298479485,-73.9785862257575,176.081298694509));
#16114=CARTESIAN_POINT('Ctrl Pts',(-50.8193532731165,-73.9667923415113,
176.052750467827));
#16115=CARTESIAN_POINT('Ctrl Pts',(-50.8181944769487,-73.9597687273717,
176.022964685054));
#16116=CARTESIAN_POINT('Ctrl Pts',(-50.8180506457443,-73.9588968877778,
175.992027399553));
#16117=CARTESIAN_POINT('Ctrl Pts',(-50.817908130518,-73.9580330250466,175.961373173548));
#16118=CARTESIAN_POINT('Ctrl Pts',(-50.818771419997,-73.9632653488002,175.931596917882));
#16119=CARTESIAN_POINT('Ctrl Pts',(-50.8204678882598,-73.9735504690026,
175.902755935248));
#16120=CARTESIAN_POINT('Ctrl Pts',(-50.8226211501266,-73.9866049761884,
175.866149186116));
#16121=CARTESIAN_POINT('Ctrl Pts',(-50.8260344374881,-74.0073021325509,
175.832457982263));
#16122=CARTESIAN_POINT('Ctrl Pts',(-50.8299972977936,-74.0313451228971,
175.80212682161));
#16123=CARTESIAN_POINT('Ctrl Pts',(-50.8362737302612,-74.0694247405445,
175.754087913644));
#16124=CARTESIAN_POINT('Ctrl Pts',(-50.8443796156014,-74.1186360495895,
175.711069473412));
#16125=CARTESIAN_POINT('Ctrl Pts',(-50.8526027993114,-74.1686130255098,
175.674187743685));
#16126=CARTESIAN_POINT('Ctrl Pts',(-50.8539198545757,-74.1766175212803,
175.668280630576));
#16127=CARTESIAN_POINT('Ctrl Pts',(-50.8552399236702,-74.1846415471193,
175.662530938822));
#16128=CARTESIAN_POINT('Ctrl Pts',(-50.8565559779939,-74.1926423775393,
175.6569432546));
#16129=CARTESIAN_POINT('Ctrl Pts',(-50.868899714928,-74.2676849834404,175.604534396648));
#16130=CARTESIAN_POINT('Ctrl Pts',(-50.8833664041038,-74.3557461756237,
175.555830160403));
#16131=CARTESIAN_POINT('Ctrl Pts',(-50.898709234606,-74.449322863261,175.511142903759));
#16132=CARTESIAN_POINT('Ctrl Pts',(-50.9122347199158,-74.5318154720261,
175.471748814567));
#16133=CARTESIAN_POINT('Ctrl Pts',(-50.9264410802539,-74.6185943708312,
175.435476448387));
#16134=CARTESIAN_POINT('Ctrl Pts',(-50.9404762908346,-74.7044702872778,
175.40253979577));
#16135=CARTESIAN_POINT('Ctrl Pts',(-50.9423621250129,-74.7160089626255,
175.398114278613));
#16136=CARTESIAN_POINT('Ctrl Pts',(-50.9442448726816,-74.727531258289,175.393748983833));
#16137=CARTESIAN_POINT('Ctrl Pts',(-50.9461224701891,-74.7390245137205,
175.389444430525));
#16138=CARTESIAN_POINT('Ctrl Pts',(-50.9649625531635,-74.8543494889124,
175.346251924598));
#16139=CARTESIAN_POINT('Ctrl Pts',(-50.9850447742112,-74.977532800152,175.305189767046));
#16140=CARTESIAN_POINT('Ctrl Pts',(-51.0057593748162,-75.1049143140581,
175.266364772338));
#16141=CARTESIAN_POINT('Ctrl Pts',(-51.0260059583032,-75.2294178227266,
175.228416973502));
#16142=CARTESIAN_POINT('Ctrl Pts',(-51.0468566504168,-75.3579323481973,
175.192606388452));
#16143=CARTESIAN_POINT('Ctrl Pts',(-51.0677442194091,-75.4869918763851,
175.159032754036));
#16144=CARTESIAN_POINT('Ctrl Pts',(-51.0888832841532,-75.6176053395035,
175.125054877919));
#16145=CARTESIAN_POINT('Ctrl Pts',(-51.1100601094042,-75.7487771848276,
175.093368144521));
#16146=CARTESIAN_POINT('Ctrl Pts',(-51.1306891566218,-75.876859965402,175.064075936874));
#16147=CARTESIAN_POINT('Ctrl Pts',(-51.1507544538042,-76.0014425032698,
175.035584225871));
#16148=CARTESIAN_POINT('Ctrl Pts',(-51.1703015295575,-76.1231018808035,
175.009357953825));
#16149=CARTESIAN_POINT('Ctrl Pts',(-51.1887936826668,-76.2384341198503,
174.985492257536));
#16150=CARTESIAN_POINT('',(-50.7024802268295,-64.5970226062537,173.485485069079));
#16151=CARTESIAN_POINT('Ctrl Pts',(-50.7024802268248,-64.5970226062542,
173.485485069085));
#16152=CARTESIAN_POINT('Ctrl Pts',(-50.9643032922535,-67.0529990415413,
173.485485603988));
#16153=CARTESIAN_POINT('Ctrl Pts',(-51.218469484852,-69.7245979498243,173.520841304362));
#16154=CARTESIAN_POINT('Ctrl Pts',(-51.4912169004962,-73.3272878136435,
173.671974926571));
#16155=CARTESIAN_POINT('Ctrl Pts',(-51.7170878156646,-76.636174896363,173.822575916535));
#16156=CARTESIAN_POINT('Ctrl Pts',(-51.6237538197336,-77.6203204977443,
174.215041830701));
#16157=CARTESIAN_POINT('Ctrl Pts',(-51.6154076427636,-77.6830014132838,
174.245424370326));
#16158=CARTESIAN_POINT('Ctrl Pts',(-51.5981975764625,-77.7480985755699,
174.296408211552));
#16159=CARTESIAN_POINT('Ctrl Pts',(-51.5917351323593,-77.7667510220376,
174.314500312631));
#16160=CARTESIAN_POINT('Ctrl Pts',(-51.5786277845437,-77.7877830295759,
174.348195468307));
#16161=CARTESIAN_POINT('Ctrl Pts',(-51.5729256033243,-77.7935256381876,
174.362246416503));
#16162=CARTESIAN_POINT('Ctrl Pts',(-51.5609350615783,-77.7976939764001,
174.390403091874));
#16163=CARTESIAN_POINT('Ctrl Pts',(-51.5551546562069,-77.796735277411,174.403455794326));
#16164=CARTESIAN_POINT('Ctrl Pts',(-51.5420841811777,-77.7889989352672,
174.432006923496));
#16165=CARTESIAN_POINT('Ctrl Pts',(-51.5350614462774,-77.7811412466012,
174.446707746341));
#16166=CARTESIAN_POINT('Ctrl Pts',(-51.5167709889332,-77.7544514481327,
174.4839390495));
#16167=CARTESIAN_POINT('Ctrl Pts',(-51.5056242119341,-77.7306696787344,
174.505354751846));
#16168=CARTESIAN_POINT('Ctrl Pts',(-51.4723854079891,-77.6487073114297,
174.567396292195));
#16169=CARTESIAN_POINT('Ctrl Pts',(-51.449199025989,-77.5696294940345,174.607070508007));
#16170=CARTESIAN_POINT('Ctrl Pts',(-51.3451043426313,-77.1694577561508,
174.778180690935));
#16171=CARTESIAN_POINT('Ctrl Pts',(-51.255403237339,-76.6537518959946,174.899487153725));
#16172=CARTESIAN_POINT('Ctrl Pts',(-51.1888118575074,-76.2384181515047,
174.985415709881));
#16173=CARTESIAN_POINT('',(-48.3850788590687,-42.8591601353355,173.485485069079));
#16174=CARTESIAN_POINT('',(-48.3850788590687,-42.8591601353355,173.485485069079));
#16175=CARTESIAN_POINT('',(-54.5948893516535,-42.1971528497386,173.485485069079));
#16176=CARTESIAN_POINT('Origin',(-51.4899841053611,-42.5281564925371,175.985485069079));
#16177=CARTESIAN_POINT('',(-60.5749026458094,-98.2913229710871,173.485485069079));
#16178=CARTESIAN_POINT('',(-54.5948893516535,-42.1971528497386,173.485485069079));
#16179=CARTESIAN_POINT('',(-60.6995605645563,-99.4606485490079,178.485485069079));
#16180=CARTESIAN_POINT('Ctrl Pts',(-60.5749026458094,-98.2913229710871,
173.485485069079));
#16181=CARTESIAN_POINT('Ctrl Pts',(-60.3843342578436,-98.3299608318209,
173.243690644989));
#16182=CARTESIAN_POINT('Ctrl Pts',(-60.1664113055595,-98.3704554623929,
173.025230159753));
#16183=CARTESIAN_POINT('Ctrl Pts',(-59.6797951404782,-98.4594953210885,
172.639492409097));
#16184=CARTESIAN_POINT('Ctrl Pts',(-59.4118189594528,-98.507396166173,172.474839570992));
#16185=CARTESIAN_POINT('Ctrl Pts',(-58.6475696307461,-98.6412135625171,
172.12302034014));
#16186=CARTESIAN_POINT('Ctrl Pts',(-58.1285326590571,-98.7293077079875,
172.001630150343));
#16187=CARTESIAN_POINT('Ctrl Pts',(-57.0934944411569,-98.8999216213785,
171.972905197423));
#16188=CARTESIAN_POINT('Ctrl Pts',(-56.5880866935318,-98.9843175007548,
172.057860325957));
#16189=CARTESIAN_POINT('Ctrl Pts',(-55.6187428548676,-99.1521396670418,
172.423693545831));
#16190=CARTESIAN_POINT('Ctrl Pts',(-55.1668789617469,-99.2330770981518,
172.708357719645));
#16191=CARTESIAN_POINT('Ctrl Pts',(-54.4152301073058,-99.3735193085268,
173.42678745864));
#16192=CARTESIAN_POINT('Ctrl Pts',(-54.117636559382,-99.4356985494873,173.847812184324));
#16193=CARTESIAN_POINT('Ctrl Pts',(-53.6961108373074,-99.5440869286819,
174.784491901195));
#16194=CARTESIAN_POINT('Ctrl Pts',(-53.5772634151522,-99.5885264630858,
175.29189396112));
#16195=CARTESIAN_POINT('Ctrl Pts',(-53.5376636121844,-99.6533071133646,
176.336975547334));
#16196=CARTESIAN_POINT('Ctrl Pts',(-53.6220957342369,-99.6753461866961,
176.86477871382));
#16197=CARTESIAN_POINT('Ctrl Pts',(-53.9867706921353,-99.7008570794232,
177.847215661255));
#16198=CARTESIAN_POINT('Ctrl Pts',(-54.2591330424856,-99.7036171849942,
178.293920024946));
#16199=CARTESIAN_POINT('Ctrl Pts',(-54.9652132353756,-99.688957954165,179.067651982994));
#16200=CARTESIAN_POINT('Ctrl Pts',(-55.3955739876124,-99.6740155440745,
179.384324188019));
#16201=CARTESIAN_POINT('Ctrl Pts',(-56.3444317593121,-99.6372231709392,
179.82771784559));
#16202=CARTESIAN_POINT('Ctrl Pts',(-56.8518377636485,-99.6149533982737,
179.954069319539));
#16203=CARTESIAN_POINT('Ctrl Pts',(-57.8965798954297,-99.5642480107107,
180.007121753964));
#16204=CARTESIAN_POINT('Ctrl Pts',(-58.4243189790396,-99.5388174118719,
179.929254775814));
#16205=CARTESIAN_POINT('Ctrl Pts',(-59.2732803979538,-99.5037201258886,
179.625522348307));
#16206=CARTESIAN_POINT('Ctrl Pts',(-59.6053345182171,-99.4912868821982,
179.451477802644));
#16207=CARTESIAN_POINT('Ctrl Pts',(-60.2050026582842,-99.4715409050409,
179.021596162725));
#16208=CARTESIAN_POINT('Ctrl Pts',(-60.4709693041988,-99.4634768492749,
178.769761221572));
#16209=CARTESIAN_POINT('Ctrl Pts',(-60.6995605645563,-99.4606485490079,
178.485485069079));
#16210=CARTESIAN_POINT('',(-54.5948893516535,-42.1971528497386,178.485485069079));
#16211=CARTESIAN_POINT('Origin',(-51.4899841053611,-42.5281564925371,175.985485069079));
#16212=CARTESIAN_POINT('',(-60.7525635667804,-99.9578312938364,178.485485069079));
#16213=CARTESIAN_POINT('',(-60.6279056480334,-98.7885057159157,173.485485069079));
#16214=CARTESIAN_POINT('Ctrl Pts',(-60.7525635667804,-99.9578312938363,
178.485485069079));
#16215=CARTESIAN_POINT('Ctrl Pts',(-60.5471423783721,-99.9603729168234,
178.740946913902));
#16216=CARTESIAN_POINT('Ctrl Pts',(-60.3114768367406,-99.9672665268891,
178.970306818076));
#16217=CARTESIAN_POINT('Ctrl Pts',(-59.7836134097214,-99.984122670903,179.371140823409));
#16218=CARTESIAN_POINT('Ctrl Pts',(-59.4924716081514,-99.9946533930933,
179.539560425843));
#16219=CARTESIAN_POINT('Ctrl Pts',(-58.689917777404,-100.026622058121,179.878337837155));
#16220=CARTESIAN_POINT('Ctrl Pts',(-58.1594421477247,-100.050492208668,
179.985627564123));
#16221=CARTESIAN_POINT('Ctrl Pts',(-57.1087945616306,-100.102727643745,
179.98534767287));
#16222=CARTESIAN_POINT('Ctrl Pts',(-56.598242490745,-100.125780453932,179.885741010665));
#16223=CARTESIAN_POINT('Ctrl Pts',(-55.6234756153487,-100.164999588288,
179.490939604252));
#16224=CARTESIAN_POINT('Ctrl Pts',(-55.1718628664936,-100.180456631909,
179.192079540234));
#16225=CARTESIAN_POINT('Ctrl Pts',(-54.4271820616128,-100.200076542985,
178.449324335202));
#16226=CARTESIAN_POINT('Ctrl Pts',(-54.1351780528778,-100.199832004087,
178.01823003711));
#16227=CARTESIAN_POINT('Ctrl Pts',(-53.7214511213677,-100.179252959187,
177.050986426422));
#16228=CARTESIAN_POINT('Ctrl Pts',(-53.6110793820867,-100.158325421843,
176.520980040015));
#16229=CARTESIAN_POINT('Ctrl Pts',(-53.6046567482091,-100.098079340991,
175.450211066692));
#16230=CARTESIAN_POINT('Ctrl Pts',(-53.7080530455439,-100.05436333493,174.920181160456));
#16231=CARTESIAN_POINT('Ctrl Pts',(-54.1082249007172,-99.9470040374134,
173.952740103037));
#16232=CARTESIAN_POINT('Ctrl Pts',(-54.3936147011503,-99.8852054601572,
173.521645801326));
#16233=CARTESIAN_POINT('Ctrl Pts',(-55.1256953569007,-99.7473927319089,
172.778890603587));
#16234=CARTESIAN_POINT('Ctrl Pts',(-55.5704169165303,-99.6672945533789,
172.480030545584));
#16235=CARTESIAN_POINT('Ctrl Pts',(-56.5315444145501,-99.5001344145226,
172.085229134352));
#16236=CARTESIAN_POINT('Ctrl Pts',(-57.035481997341,-99.4150358490739,171.985622467862));
#16237=CARTESIAN_POINT('Ctrl Pts',(-58.0735288862887,-99.2446024971114,
171.985342571377));
#16238=CARTESIAN_POINT('Ctrl Pts',(-58.5971145479235,-99.156102675648,172.092632290086));
#16239=CARTESIAN_POINT('Ctrl Pts',(-59.3883708997698,-99.0181605272865,
172.431409687741));
#16240=CARTESIAN_POINT('Ctrl Pts',(-59.6751894929103,-98.9670768091508,
172.599829292627));
#16241=CARTESIAN_POINT('Ctrl Pts',(-60.1947430170222,-98.8722713063087,
173.000663306832));
#16242=CARTESIAN_POINT('Ctrl Pts',(-60.4265653832759,-98.8293275814563,
173.230023216865));
#16243=CARTESIAN_POINT('Ctrl Pts',(-60.6279056480337,-98.7885057159156,
173.48548506908));
#16244=CARTESIAN_POINT('',(-60.7339116524816,-99.7828712055727,173.485485069079));
#16245=CARTESIAN_POINT('',(-54.5948893516535,-42.1971528497386,173.485485069079));
#16246=CARTESIAN_POINT('',(-60.8585695712285,-100.952196783494,178.485485069079));
#16247=CARTESIAN_POINT('Ctrl Pts',(-60.7339116524819,-99.7828712055727,
173.48548506908));
#16248=CARTESIAN_POINT('Ctrl Pts',(-60.5433422383796,-99.8215092743563,
173.243689343021));
#16249=CARTESIAN_POINT('Ctrl Pts',(-60.3254252550916,-99.8620027807692,
173.025234570342));
#16250=CARTESIAN_POINT('Ctrl Pts',(-59.8388069738715,-99.9510430502776,
172.639494146729));
#16251=CARTESIAN_POINT('Ctrl Pts',(-59.5708294688831,-99.9989441375308,
172.474840262781));
#16252=CARTESIAN_POINT('Ctrl Pts',(-58.8065786374188,-100.132761797002,
172.123020340141));
#16253=CARTESIAN_POINT('Ctrl Pts',(-58.2875416657299,-100.220855942473,
172.001630150343));
#16254=CARTESIAN_POINT('Ctrl Pts',(-57.2525034478298,-100.391469855864,
171.972905197423));
#16255=CARTESIAN_POINT('Ctrl Pts',(-56.7470957002047,-100.47586573524,172.057860325957));
#16256=CARTESIAN_POINT('Ctrl Pts',(-55.7777518615402,-100.643687901527,
172.423693545831));
#16257=CARTESIAN_POINT('Ctrl Pts',(-55.3258879684196,-100.724625332637,
172.708357719645));
#16258=CARTESIAN_POINT('Ctrl Pts',(-54.5742391139785,-100.865067543012,
173.42678745864));
#16259=CARTESIAN_POINT('Ctrl Pts',(-54.2766455660546,-100.927246783973,
173.847812184324));
#16260=CARTESIAN_POINT('Ctrl Pts',(-53.8551198439798,-101.035635163167,
174.784491901194));
#16261=CARTESIAN_POINT('Ctrl Pts',(-53.7362724218245,-101.080074697571,
175.291893961119));
#16262=CARTESIAN_POINT('Ctrl Pts',(-53.6966726188566,-101.14485534785,176.336975547333));
#16263=CARTESIAN_POINT('Ctrl Pts',(-53.781104740909,-101.166894421182,176.864778713819));
#16264=CARTESIAN_POINT('Ctrl Pts',(-54.1457796988072,-101.192405313909,
177.847215661254));
#16265=CARTESIAN_POINT('Ctrl Pts',(-54.4181420491574,-101.195165419479,
178.293920024946));
#16266=CARTESIAN_POINT('Ctrl Pts',(-55.124222242047,-101.18050618865,179.067651982994));
#16267=CARTESIAN_POINT('Ctrl Pts',(-55.5545829942836,-101.16556377856,179.384324188018));
#16268=CARTESIAN_POINT('Ctrl Pts',(-56.5034407659834,-101.128771405425,
179.827717845589));
#16269=CARTESIAN_POINT('Ctrl Pts',(-57.0108467703198,-101.106501632759,
179.954069319539));
#16270=CARTESIAN_POINT('Ctrl Pts',(-58.0555889021011,-101.055796245196,
180.007121753964));
#16271=CARTESIAN_POINT('Ctrl Pts',(-58.583327985711,-101.030365646357,179.929254775814));
#16272=CARTESIAN_POINT('Ctrl Pts',(-59.4322909909086,-100.995268294794,
179.625521780784));
#16273=CARTESIAN_POINT('Ctrl Pts',(-59.7643465168892,-100.982835004683,
179.451476233125));
#16274=CARTESIAN_POINT('Ctrl Pts',(-60.3640168394565,-100.963088982314,
179.021591890977));
#16275=CARTESIAN_POINT('Ctrl Pts',(-60.629977267773,-100.955025096667,178.769762518769));
#16276=CARTESIAN_POINT('Ctrl Pts',(-60.8585695712285,-100.952196783494,
178.485485069079));
#16277=CARTESIAN_POINT('',(-54.5948893516535,-42.1971528497386,178.485485069079));
#16278=CARTESIAN_POINT('Origin',(-51.4899841053611,-42.5281564925371,175.985485069079));
#16279=CARTESIAN_POINT('',(-60.9115725734526,-101.449379528322,178.485485069079));
#16280=CARTESIAN_POINT('',(-60.7869146547057,-100.280053950401,173.485485069079));
#16281=CARTESIAN_POINT('Ctrl Pts',(-60.9115725734526,-101.449379528322,
178.485485069079));
#16282=CARTESIAN_POINT('Ctrl Pts',(-60.7061513850443,-101.451921151309,
178.740946913902));
#16283=CARTESIAN_POINT('Ctrl Pts',(-60.4704858434129,-101.458814761375,
178.970306818076));
#16284=CARTESIAN_POINT('Ctrl Pts',(-59.9426224163936,-101.475670905389,
179.371140823409));
#16285=CARTESIAN_POINT('Ctrl Pts',(-59.6514806148234,-101.48620162758,179.539560425843));
#16286=CARTESIAN_POINT('Ctrl Pts',(-58.8489267840763,-101.518170292608,
179.878337837155));
#16287=CARTESIAN_POINT('Ctrl Pts',(-58.318451154397,-101.542040443154,179.985627564123));
#16288=CARTESIAN_POINT('Ctrl Pts',(-57.2678035683027,-101.594275878231,
179.98534767287));
#16289=CARTESIAN_POINT('Ctrl Pts',(-56.757251497417,-101.617328688418,179.885741010665));
#16290=CARTESIAN_POINT('Ctrl Pts',(-55.782484622021,-101.656547822774,179.490939604252));
#16291=CARTESIAN_POINT('Ctrl Pts',(-55.3308718731657,-101.672004866394,
179.192079540234));
#16292=CARTESIAN_POINT('Ctrl Pts',(-54.5861910682848,-101.69162477747,178.449324335202));
#16293=CARTESIAN_POINT('Ctrl Pts',(-54.2941870595498,-101.691380238572,
178.01823003711));
#16294=CARTESIAN_POINT('Ctrl Pts',(-53.8804601280398,-101.670801193672,
177.050986426422));
#16295=CARTESIAN_POINT('Ctrl Pts',(-53.7700883887589,-101.649873656328,
176.520980040015));
#16296=CARTESIAN_POINT('Ctrl Pts',(-53.7636657548814,-101.589627575476,
175.450211066692));
#16297=CARTESIAN_POINT('Ctrl Pts',(-53.8670620522162,-101.545911569416,
174.920181160456));
#16298=CARTESIAN_POINT('Ctrl Pts',(-54.2672339073893,-101.438552271899,
173.952740103038));
#16299=CARTESIAN_POINT('Ctrl Pts',(-54.5526237078223,-101.376753694642,
173.521645801326));
#16300=CARTESIAN_POINT('Ctrl Pts',(-55.2847043635729,-101.238940966394,
172.778890603587));
#16301=CARTESIAN_POINT('Ctrl Pts',(-55.7294259232024,-101.158842787864,
172.480030545584));
#16302=CARTESIAN_POINT('Ctrl Pts',(-56.6905534212225,-100.991682649007,
172.085229134352));
#16303=CARTESIAN_POINT('Ctrl Pts',(-57.1944910040133,-100.906584083559,
171.985622467862));
#16304=CARTESIAN_POINT('Ctrl Pts',(-58.2325378929607,-100.736150731597,
171.985342571377));
#16305=CARTESIAN_POINT('Ctrl Pts',(-58.7561235545955,-100.647650910134,
172.092632290086));
#16306=CARTESIAN_POINT('Ctrl Pts',(-59.547378382634,-100.509709027422,172.431409035321));
#16307=CARTESIAN_POINT('Ctrl Pts',(-59.8341956324852,-100.458625554302,
172.599827608127));
#16308=CARTESIAN_POINT('Ctrl Pts',(-60.353747032482,-100.363820463799,173.000658940243));
#16309=CARTESIAN_POINT('Ctrl Pts',(-60.5855754147608,-100.320875608161,
173.230024517154));
#16310=CARTESIAN_POINT('Ctrl Pts',(-60.7869146547057,-100.280053950401,
173.485485069079));
#16311=CARTESIAN_POINT('',(-60.8929206591539,-101.274419440058,173.485485069079));
#16312=CARTESIAN_POINT('',(-54.5948893516535,-42.1971528497386,173.485485069079));
#16313=CARTESIAN_POINT('',(-53.8728824136219,-102.614109889754,175.985485078249));
#16314=CARTESIAN_POINT('Ctrl Pts',(-60.8929206591538,-101.274419440058,
173.485485069079));
#16315=CARTESIAN_POINT('Ctrl Pts',(-60.7102269210105,-101.311460710579,
173.253682052479));
#16316=CARTESIAN_POINT('Ctrl Pts',(-60.502365296309,-101.350178825903,173.043294821439));
#16317=CARTESIAN_POINT('Ctrl Pts',(-60.0395467045387,-101.435037463867,
172.669117273279));
#16318=CARTESIAN_POINT('Ctrl Pts',(-59.7851929521217,-101.480626055513,
172.507657607619));
#16319=CARTESIAN_POINT('Ctrl Pts',(-59.0406892261035,-101.611411060069,
172.147006028652));
#16320=CARTESIAN_POINT('Ctrl Pts',(-58.5252323432285,-101.699158257146,
172.015459906787));
#16321=CARTESIAN_POINT('Ctrl Pts',(-57.4926845327902,-101.869865342548,
171.965563441252));
#16322=CARTESIAN_POINT('Ctrl Pts',(-56.9862231691556,-101.953834724284,
172.039921277568));
#16323=CARTESIAN_POINT('Ctrl Pts',(-56.0247569440159,-102.11975084989,172.379917992812));
#16324=CARTESIAN_POINT('Ctrl Pts',(-55.5793041661649,-102.199151236466,
172.644151600608));
#16325=CARTESIAN_POINT('Ctrl Pts',(-54.8070206720663,-102.342342925632,
173.335663171704));
#16326=CARTESIAN_POINT('Ctrl Pts',(-54.4900108722134,-102.406626608065,
173.758726921452));
#16327=CARTESIAN_POINT('Ctrl Pts',(-54.1325977439973,-102.495899358773,
174.506835663783));
#16328=CARTESIAN_POINT('Ctrl Pts',(-54.033087296471,-102.525372948297,174.796081818852));
#16329=CARTESIAN_POINT('Ctrl Pts',(-53.9027346997917,-102.576055283617,
175.386624643971));
#16330=CARTESIAN_POINT('Ctrl Pts',(-53.8710837883173,-102.597238295983,
175.685621934182));
#16331=CARTESIAN_POINT('Ctrl Pts',(-53.8728824136219,-102.614109889754,
175.985485078249));
#16332=CARTESIAN_POINT('',(-60.9552496185426,-101.859082229163,178.485485069079));
#16333=CARTESIAN_POINT('Origin',(-57.8503443722502,-102.190085871961,175.985485069079));
#16334=CARTESIAN_POINT('',(-54.5948893516535,-42.1971528497386,178.485485069079));
#16335=CARTESIAN_POINT('Origin',(-57.8503443722502,-102.190085871961,175.985485069079));
#16336=CARTESIAN_POINT('',(-59.5310685485181,-102.312170685956,173.485485069079));
#16337=CARTESIAN_POINT('',(-56.2564866337797,-102.944965370977,173.489866571436));
#16338=CARTESIAN_POINT('Ctrl Pts',(-56.2564866337792,-102.944965370977,
173.489866571436));
#16339=CARTESIAN_POINT('Ctrl Pts',(-56.4989794446454,-102.895253602946,
173.325488559424));
#16340=CARTESIAN_POINT('Ctrl Pts',(-56.7642531084334,-102.842545984514,
173.198515194001));
#16341=CARTESIAN_POINT('Ctrl Pts',(-57.3189939774646,-102.735361409915,
173.028869909839));
#16342=CARTESIAN_POINT('Ctrl Pts',(-57.6051560932325,-102.681480718025,
172.985872610607));
#16343=CARTESIAN_POINT('Ctrl Pts',(-58.1808148055288,-102.575807458543,
172.985103094898));
#16344=CARTESIAN_POINT('Ctrl Pts',(-58.4670480699436,-102.521964579041,
173.02725873048));
#16345=CARTESIAN_POINT('Ctrl Pts',(-59.0224385185242,-102.414706992302,
173.195445680148));
#16346=CARTESIAN_POINT('Ctrl Pts',(-59.2880999534127,-102.361950173258,
173.32172571804));
#16347=CARTESIAN_POINT('Ctrl Pts',(-59.5310685485181,-102.312170685956,
173.485485069079));
#16348=CARTESIAN_POINT('',(-59.5702274233335,-102.679491706429,173.485485069079));
#16349=CARTESIAN_POINT('',(-59.4993129890855,-102.014294800821,173.485485069079));
#16350=CARTESIAN_POINT('',(-56.2951298069876,-103.312392114382,173.490216228516));
#16351=CARTESIAN_POINT('Ctrl Pts',(-59.570227423334,-102.679491706429,173.48548506908));
#16352=CARTESIAN_POINT('Ctrl Pts',(-59.3272139607109,-102.729280386204,
173.321695477607));
#16353=CARTESIAN_POINT('Ctrl Pts',(-59.0614995139417,-102.782047448757,
173.195399203235));
#16354=CARTESIAN_POINT('Ctrl Pts',(-58.5060004700764,-102.889324948104,
173.027212807591));
#16355=CARTESIAN_POINT('Ctrl Pts',(-58.2197132838581,-102.943175309962,
172.985072830814));
#16356=CARTESIAN_POINT('Ctrl Pts',(-57.6439497370216,-103.048869755498,
172.98590377254));
#16357=CARTESIAN_POINT('Ctrl Pts',(-57.3577384239598,-103.102760957316,
173.028947814549));
#16358=CARTESIAN_POINT('Ctrl Pts',(-56.8029251208583,-103.209962647076,
173.198713721519));
#16359=CARTESIAN_POINT('Ctrl Pts',(-56.5376294470979,-103.262676571874,
173.325758640231));
#16360=CARTESIAN_POINT('Ctrl Pts',(-56.2951298069871,-103.312392114382,
173.490216228516));
#16361=CARTESIAN_POINT('',(-56.2564866337797,-102.944965370977,173.489866571436));
#16362=CARTESIAN_POINT('Origin',(-57.8503443722502,-102.190085871961,175.985485069079));
#16363=CARTESIAN_POINT('',(-59.6900775551904,-103.803718920442,173.485485069079));
#16364=CARTESIAN_POINT('',(-56.4134173387405,-104.436939704691,173.491276679515));
#16365=CARTESIAN_POINT('Ctrl Pts',(-56.41341733874,-104.436939704691,173.491276679516));
#16366=CARTESIAN_POINT('Ctrl Pts',(-56.6559375281166,-104.387212747836,
173.326577849171));
#16367=CARTESIAN_POINT('Ctrl Pts',(-56.9212997932767,-104.334479728502,
173.199315985643));
#16368=CARTESIAN_POINT('Ctrl Pts',(-57.4763324841321,-104.227226186699,
173.029184302443));
#16369=CARTESIAN_POINT('Ctrl Pts',(-57.7626928792531,-104.173303132952,
172.985998496287));
#16370=CARTESIAN_POINT('Ctrl Pts',(-58.3387741518067,-104.067544473328,
172.984981238005));
#16371=CARTESIAN_POINT('Ctrl Pts',(-58.6252247782338,-104.013671424672,
173.02707370444));
#16372=CARTESIAN_POINT('Ctrl Pts',(-59.1810529817342,-103.906333570922,
173.195258356014));
#16373=CARTESIAN_POINT('Ctrl Pts',(-59.4469281068036,-103.853535461025,
173.321603824031));
#16374=CARTESIAN_POINT('Ctrl Pts',(-59.6900775551904,-103.803718920442,
173.485485069079));
#16375=CARTESIAN_POINT('',(-59.7292364300057,-104.171039940915,173.485485069079));
#16376=CARTESIAN_POINT('',(-59.4993129890855,-102.014294800821,173.485485069079));
#16377=CARTESIAN_POINT('',(-56.4520785736129,-104.80436276488,173.491614708043));
#16378=CARTESIAN_POINT('Ctrl Pts',(-59.7292364300062,-104.171039940915,
173.48548506908));
#16379=CARTESIAN_POINT('Ctrl Pts',(-59.4860436647418,-104.220865356275,
173.32157462872));
#16380=CARTESIAN_POINT('Ctrl Pts',(-59.2201173545953,-104.273673356308,
173.195213495731));
#16381=CARTESIAN_POINT('Ctrl Pts',(-58.6641842924699,-104.381030436189,
173.027029420215));
#16382=CARTESIAN_POINT('Ctrl Pts',(-58.3776815999021,-104.434910714353,
172.984952103883));
#16383=CARTESIAN_POINT('Ctrl Pts',(-57.8014991187094,-104.540689830233,
172.986028757149));
#16384=CARTESIAN_POINT('Ctrl Pts',(-57.5150912399971,-104.594623030155,
173.029259751801));
#16385=CARTESIAN_POINT('Ctrl Pts',(-56.9599887060397,-104.70189308346,173.199508012997));
#16386=CARTESIAN_POINT('Ctrl Pts',(-56.6946052633784,-104.754632179713,
173.326839009941));
#16387=CARTESIAN_POINT('Ctrl Pts',(-56.452078573613,-104.80436276488,173.491614708043));
#16388=CARTESIAN_POINT('',(-56.4134173387405,-104.436939704691,173.491276679515));
#16389=CARTESIAN_POINT('Origin',(-57.8503443722502,-102.190085871961,175.985485069079));
#16390=CARTESIAN_POINT('',(-59.8490865618626,-105.295267154927,173.485485069079));
#16391=CARTESIAN_POINT('',(-56.5704762085008,-105.92888783639,173.492602186485));
#16392=CARTESIAN_POINT('Ctrl Pts',(-56.5704762085003,-105.92888783639,173.492602186486));
#16393=CARTESIAN_POINT('Ctrl Pts',(-56.8130217456382,-105.879146680719,
173.327602022451));
#16394=CARTESIAN_POINT('Ctrl Pts',(-57.07846691305,-105.826389859661,173.200069123079));
#16395=CARTESIAN_POINT('Ctrl Pts',(-57.633773223064,-105.719071619894,173.029480349745));
#16396=CARTESIAN_POINT('Ctrl Pts',(-57.9203197057099,-105.6651088001,172.986117345367));
#16397=CARTESIAN_POINT('Ctrl Pts',(-58.4967976547893,-105.559269960174,
172.984867162949));
#16398=CARTESIAN_POINT('Ctrl Pts',(-58.7834523644571,-105.505368567675,
173.026900204104));
#16399=CARTESIAN_POINT('Ctrl Pts',(-59.339691582227,-105.397955355066,173.195082541135));
#16400=CARTESIAN_POINT('Ctrl Pts',(-59.6057673336779,-105.345118480053,
173.321489393483));
#16401=CARTESIAN_POINT('Ctrl Pts',(-59.8490865618626,-105.295267154927,
173.485485069079));
#16402=CARTESIAN_POINT('',(-59.8882454366779,-105.662588175401,173.485485069079));
#16403=CARTESIAN_POINT('',(-59.4993129890855,-102.014294800821,173.485485069079));
#16404=CARTESIAN_POINT('',(-56.6091901843099,-106.296300098484,173.492904904243));
#16405=CARTESIAN_POINT('Ctrl Pts',(-59.8882454366779,-105.662588175401,
173.485485069079));
#16406=CARTESIAN_POINT('Ctrl Pts',(-59.6448874651583,-105.712447438273,
173.321463280712));
#16407=CARTESIAN_POINT('Ctrl Pts',(-59.3787659285087,-105.765293159726,
173.195042425979));
#16408=CARTESIAN_POINT('Ctrl Pts',(-58.8224329097879,-105.872723569926,
173.026860638454));
#16409=CARTESIAN_POINT('Ctrl Pts',(-58.5357316247444,-105.926631433394,
172.984841174824));
#16410=CARTESIAN_POINT('Ctrl Pts',(-57.959163155205,-106.03248857175,172.986144557556));
#16411=CARTESIAN_POINT('Ctrl Pts',(-57.6725742135264,-106.086460466031,
173.029548030212));
#16412=CARTESIAN_POINT('Ctrl Pts',(-57.1172055074798,-106.19379346387,173.200241176083));
#16413=CARTESIAN_POINT('Ctrl Pts',(-56.8517414582687,-106.246555710665,
173.327835953701));
#16414=CARTESIAN_POINT('Ctrl Pts',(-56.60919018431,-106.296300098484,173.492904904243));
#16415=CARTESIAN_POINT('',(-56.5704762085008,-105.92888783639,173.492602186485));
#16416=CARTESIAN_POINT('Origin',(-57.8503443722502,-102.190085871961,175.985485069079));
#16417=CARTESIAN_POINT('',(-60.0080955685348,-106.786815389413,173.485485069079));
#16418=CARTESIAN_POINT('',(-56.7277951555015,-107.420782694947,173.49375276819));
#16419=CARTESIAN_POINT('Ctrl Pts',(-56.727795155501,-107.420782694947,173.49375276819));
#16420=CARTESIAN_POINT('Ctrl Pts',(-56.9703623912548,-107.371029275934,
173.328491222585));
#16421=CARTESIAN_POINT('Ctrl Pts',(-57.2358792201269,-107.318251853156,
173.200723175827));
#16422=CARTESIAN_POINT('Ctrl Pts',(-57.7914224962462,-107.210877556492,
173.02973773311));
#16423=CARTESIAN_POINT('Ctrl Pts',(-58.0781302770999,-107.156880260998,
172.986220914227));
#16424=CARTESIAN_POINT('Ctrl Pts',(-58.6549521376339,-107.050971897315,
172.984768510842));
#16425=CARTESIAN_POINT('Ctrl Pts',(-58.9417838117716,-106.997045913428,
173.026749932901));
#16426=CARTESIAN_POINT('Ctrl Pts',(-59.4983794295013,-106.889567359307,
173.194930140002));
#16427=CARTESIAN_POINT('Ctrl Pts',(-59.7646291406404,-106.836696872864,
173.321390181777));
#16428=CARTESIAN_POINT('Ctrl Pts',(-60.0080955685353,-106.786815389413,
173.48548506908));
#16429=CARTESIAN_POINT('',(-60.0472544433502,-107.154136409886,173.485485069079));
#16430=CARTESIAN_POINT('',(-59.4993129890855,-102.014294800821,173.485485069079));
#16431=CARTESIAN_POINT('',(-56.766590524313,-107.788178276076,173.494000465338));
#16432=CARTESIAN_POINT('Ctrl Pts',(-60.0472544433507,-107.154136409886,
173.48548506908));
#16433=CARTESIAN_POINT('Ctrl Pts',(-59.803756348025,-107.204024381371,173.321368838121));
#16434=CARTESIAN_POINT('Ctrl Pts',(-59.5374692105895,-107.256902098957,
173.194897357342));
#16435=CARTESIAN_POINT('Ctrl Pts',(-58.9807969137183,-107.364394710774,
173.026717623417));
#16436=CARTESIAN_POINT('Ctrl Pts',(-58.6939271659299,-107.41832598715,172.984747318098));
#16437=CARTESIAN_POINT('Ctrl Pts',(-58.1170313186328,-107.524249308753,
172.98624325915));
#16438=CARTESIAN_POINT('Ctrl Pts',(-57.83028884093,-107.578254021139,173.029793191131));
#16439=CARTESIAN_POINT('Ctrl Pts',(-57.2746946153895,-107.685640373486,
173.200864016778));
#16440=CARTESIAN_POINT('Ctrl Pts',(-57.0091623950157,-107.73842222438,173.328682671664));
#16441=CARTESIAN_POINT('Ctrl Pts',(-56.766590524313,-107.788178276076,173.494000465338));
#16442=CARTESIAN_POINT('',(-56.7277951555015,-107.420782694947,173.49375276819));
#16443=CARTESIAN_POINT('Origin',(-57.8503443722502,-102.190085871961,175.985485069079));
#16444=CARTESIAN_POINT('',(-60.167104575207,-108.278363623899,173.485485069079));
#16445=CARTESIAN_POINT('',(-56.8854801878217,-108.912602509009,173.494655322398));
#16446=CARTESIAN_POINT('Ctrl Pts',(-56.8854801878217,-108.912602509009,
173.494655322398));
#16447=CARTESIAN_POINT('Ctrl Pts',(-57.1280642474478,-108.86283951024,173.329188860889));
#16448=CARTESIAN_POINT('Ctrl Pts',(-57.3936370951202,-108.810045965017,
173.20123643479));
#16449=CARTESIAN_POINT('Ctrl Pts',(-57.9493659024473,-108.702627762264,
173.029939895836));
#16450=CARTESIAN_POINT('Ctrl Pts',(-58.2362000607429,-108.648603450439,
172.986302419157));
#16451=CARTESIAN_POINT('Ctrl Pts',(-58.8132914268818,-108.542640598827,
172.984691363898));
#16452=CARTESIAN_POINT('Ctrl Pts',(-59.1002617970616,-108.488695332397,
173.026632270813));
#16453=CARTESIAN_POINT('Ctrl Pts',(-59.657136744632,-108.381165569144,173.194810728768));
#16454=CARTESIAN_POINT('Ctrl Pts',(-59.9235227921166,-108.328268741361,
173.321312433078));
#16455=CARTESIAN_POINT('Ctrl Pts',(-60.1671045752075,-108.278363623899,
173.48548506908));
#16456=CARTESIAN_POINT('',(-60.2062634500224,-108.645684644372,173.485485069079));
#16457=CARTESIAN_POINT('',(-59.4993129890855,-102.014294800821,173.485485069079));
#16458=CARTESIAN_POINT('',(-56.9243786881305,-109.279976942609,173.494832944144));
#16459=CARTESIAN_POINT('Ctrl Pts',(-60.2062634500224,-108.645684644372,
173.485485069079));
#16460=CARTESIAN_POINT('Ctrl Pts',(-59.9626589773804,-108.695594410477,
173.321297140459));
#16461=CARTESIAN_POINT('Ctrl Pts',(-59.6962461124362,-108.748496419544,
173.194787243505));
#16462=CARTESIAN_POINT('Ctrl Pts',(-59.1393162193742,-108.856036255613,
173.026609137869));
#16463=CARTESIAN_POINT('Ctrl Pts',(-58.8523185670886,-108.909985315935,
172.984676206522));
#16464=CARTESIAN_POINT('Ctrl Pts',(-58.2751741904042,-109.01595888565,172.986318485945));
#16465=CARTESIAN_POINT('Ctrl Pts',(-57.988315176016,-109.069988511531,173.029979707834));
#16466=CARTESIAN_POINT('Ctrl Pts',(-57.4325498914681,-109.1774153483,173.201337463568));
#16467=CARTESIAN_POINT('Ctrl Pts',(-57.1669660388386,-109.230212062577,
173.32932616747));
#16468=CARTESIAN_POINT('Ctrl Pts',(-56.92437868813,-109.279976942609,173.494832944145));
#16469=CARTESIAN_POINT('',(-56.8854801878217,-108.912602509009,173.494655322398));
#16470=CARTESIAN_POINT('Origin',(-57.8503443722502,-102.190085871961,175.985485069079));
#16471=CARTESIAN_POINT('',(-60.3261135818793,-109.769911858384,173.485485069079));
#16472=CARTESIAN_POINT('',(-57.043608201862,-110.404331475209,173.49525648095));
#16473=CARTESIAN_POINT('Ctrl Pts',(-57.043608201862,-110.404331475209,173.49525648095));
#16474=CARTESIAN_POINT('Ctrl Pts',(-57.2862033712323,-110.354562115194,
173.329653591047));
#16475=CARTESIAN_POINT('Ctrl Pts',(-57.5518134361477,-110.301757850008,
173.201578394561));
#16476=CARTESIAN_POINT('Ctrl Pts',(-58.1076656473085,-110.194310435517,
173.030074676988));
#16477=CARTESIAN_POINT('Ctrl Pts',(-58.3945839079253,-110.140268142502,
172.986356834207));
#16478=CARTESIAN_POINT('Ctrl Pts',(-58.9718546506282,-110.034269022205,
172.984640095432));
#16479=CARTESIAN_POINT('Ctrl Pts',(-59.258917342467,-109.980310916145,173.026554005271));
#16480=CARTESIAN_POINT('Ctrl Pts',(-59.8159782237473,-109.872747067167,
173.194731260047));
#16481=CARTESIAN_POINT('Ctrl Pts',(-60.0824550199058,-109.81983270633,173.321260684579));
#16482=CARTESIAN_POINT('Ctrl Pts',(-60.3261135818792,-109.769911858384,
173.485485069079));
#16483=CARTESIAN_POINT('',(-60.3652724566946,-110.137232878857,173.485485069079));
#16484=CARTESIAN_POINT('',(-59.4993129890855,-102.014294800821,173.485485069079));
#16485=CARTESIAN_POINT('',(-57.0826240442751,-110.771681839542,173.495354125416));
#16486=CARTESIAN_POINT('Ctrl Pts',(-60.3652724566951,-110.137232878857,
173.48548506908));
#16487=CARTESIAN_POINT('Ctrl Pts',(-60.1216014284393,-110.187156280899,
173.321252282381));
#16488=CARTESIAN_POINT('Ctrl Pts',(-59.8551098973998,-110.240073488555,
173.194718357766));
#16489=CARTESIAN_POINT('Ctrl Pts',(-59.2980188256342,-110.347642872018,
173.026541301285));
#16490=CARTESIAN_POINT('Ctrl Pts',(-59.0109411433348,-110.401603063207,
172.984631777171));
#16491=CARTESIAN_POINT('Ctrl Pts',(-58.4336412749047,-110.507608072709,
172.986365681921));
#16492=CARTESIAN_POINT('Ctrl Pts',(-58.1467093586421,-110.561653285463,
173.030096578176));
#16493=CARTESIAN_POINT('Ctrl Pts',(-57.5908371149738,-110.669105442524,
173.201633944823));
#16494=CARTESIAN_POINT('Ctrl Pts',(-57.3252210114735,-110.721911447645,
173.32972907989));
#16495=CARTESIAN_POINT('Ctrl Pts',(-57.0826240442746,-110.771681839542,
173.495354125417));
#16496=CARTESIAN_POINT('',(-57.043608201862,-110.404331475209,173.49525648095));
#16497=CARTESIAN_POINT('Origin',(-57.8503443722502,-102.190085871961,175.985485069079));
#16498=CARTESIAN_POINT('',(-60.4851225885515,-111.26146009287,173.485485069079));
#16499=CARTESIAN_POINT('',(-57.2022249863543,-111.895960177099,173.495524270213));
#16500=CARTESIAN_POINT('Ctrl Pts',(-57.2022168441609,-111.895961847564,
173.49552983027));
#16501=CARTESIAN_POINT('Ctrl Pts',(-57.4448169377341,-111.846189658907,
173.329866182698));
#16502=CARTESIAN_POINT('Ctrl Pts',(-57.7104516990721,-111.793378952777,
173.201730747205));
#16503=CARTESIAN_POINT('Ctrl Pts',(-58.2663588369567,-111.685918534124,
173.030134748854));
#16504=CARTESIAN_POINT('Ctrl Pts',(-58.5533145426031,-111.631868234738,
172.986381106475));
#16505=CARTESIAN_POINT('Ctrl Pts',(-59.1306651557994,-111.525852964465,
172.984617287507));
#16506=CARTESIAN_POINT('Ctrl Pts',(-59.417768957726,-111.471889139892,173.026519168419));
#16507=CARTESIAN_POINT('Ctrl Pts',(-59.9749126339239,-111.364310113107,
173.194695877431));
#16508=CARTESIAN_POINT('Ctrl Pts',(-60.2414298391488,-111.311387945147,
173.321237642461));
#16509=CARTESIAN_POINT('Ctrl Pts',(-60.4851225885515,-111.26146009287,173.485485069079));
#16510=CARTESIAN_POINT('',(-60.5242814633668,-111.628781113343,173.485485069079));
#16511=CARTESIAN_POINT('',(-59.4993129890855,-102.014294800821,173.485485069079));
#16512=CARTESIAN_POINT('',(-57.2413645753253,-112.263285154287,173.495537439996));
#16513=CARTESIAN_POINT('Ctrl Pts',(-60.5242814633673,-111.628781113343,
173.48548506908));
#16514=CARTESIAN_POINT('Ctrl Pts',(-60.2805870334125,-111.678709309933,
173.321236509779));
#16515=CARTESIAN_POINT('Ctrl Pts',(-60.014067841777,-111.73163186167,173.194694138168));
#16516=CARTESIAN_POINT('Ctrl Pts',(-59.4569200955657,-111.839211634557,
173.026517456143));
#16517=CARTESIAN_POINT('Ctrl Pts',(-59.1698142727596,-111.893175740257,
172.984616166662));
#16518=CARTESIAN_POINT('Ctrl Pts',(-58.5924597320949,-111.999191804659,
172.986382300312));
#16519=CARTESIAN_POINT('Ctrl Pts',(-58.3055021845535,-112.053242497856,
173.030137703114));
#16520=CARTESIAN_POINT('Ctrl Pts',(-57.7495923447614,-112.160703556161,
173.201738239673));
#16521=CARTESIAN_POINT('Ctrl Pts',(-57.4839649112239,-112.213512826487,
173.329870804249));
#16522=CARTESIAN_POINT('Ctrl Pts',(-57.2413645753249,-112.263285154288,
173.495537439996));
#16523=CARTESIAN_POINT('',(-57.2022249863543,-111.895960177099,173.495524270213));
#16524=CARTESIAN_POINT('Ctrl Pts',(-55.8010581637105,-111.27473179072,176.985485069079));
#16525=CARTESIAN_POINT('Ctrl Pts',(-55.8010581637105,-111.27473179072,174.585485069079));
#16526=CARTESIAN_POINT('Ctrl Pts',(-55.7783810390096,-111.064602968901,
176.985485069079));
#16527=CARTESIAN_POINT('Ctrl Pts',(-55.7783810390096,-111.064602968901,
174.585485069079));
#16528=CARTESIAN_POINT('Ctrl Pts',(-55.7556780473044,-110.854924957015,
176.985485069079));
#16529=CARTESIAN_POINT('Ctrl Pts',(-55.7556780473044,-110.854924957015,
174.585485069079));
#16530=CARTESIAN_POINT('Ctrl Pts',(-55.7329493398378,-110.645696396341,
176.985485069079));
#16531=CARTESIAN_POINT('Ctrl Pts',(-55.7329493398378,-110.645696396341,
174.585485069079));
#16532=CARTESIAN_POINT('',(-55.8006548129149,-111.270994369097,176.985485069079));
#16533=CARTESIAN_POINT('',(-55.7842612734031,-111.119216054728,174.985485069079));
#16534=CARTESIAN_POINT('Ctrl Pts',(-55.8006548129149,-111.270994369097,
176.985485069079));
#16535=CARTESIAN_POINT('Ctrl Pts',(-55.7959899850579,-111.227771226778,
176.734066274092));
#16536=CARTESIAN_POINT('Ctrl Pts',(-55.7920778567201,-111.19155181727,176.481361799263));
#16537=CARTESIAN_POINT('Ctrl Pts',(-55.7892777370619,-111.165635089573,
176.226833564659));
#16538=CARTESIAN_POINT('Ctrl Pts',(-55.7887660302618,-111.160898947044,
176.180319899403));
#16539=CARTESIAN_POINT('Ctrl Pts',(-55.788291815303,-111.156510162777,176.133790055636));
#16540=CARTESIAN_POINT('Ctrl Pts',(-55.7878564822688,-111.152481456388,
176.087208558517));
#16541=CARTESIAN_POINT('Ctrl Pts',(-55.787624519141,-111.150334797942,176.062388044287));
#16542=CARTESIAN_POINT('Ctrl Pts',(-55.7874036801174,-111.148291157356,
176.037561954759));
#16543=CARTESIAN_POINT('Ctrl Pts',(-55.7871941426494,-111.146352156858,
176.012724127882));
#16544=CARTESIAN_POINT('Ctrl Pts',(-55.7871517350105,-111.145959728556,
176.00769727706));
#16545=CARTESIAN_POINT('Ctrl Pts',(-55.7871097917316,-111.145571599719,
176.002670116688));
#16546=CARTESIAN_POINT('Ctrl Pts',(-55.7870683141655,-111.145187782708,
175.997642593218));
#16547=CARTESIAN_POINT('Ctrl Pts',(-55.787045553112,-111.144977160911,175.994883710735));
#16548=CARTESIAN_POINT('Ctrl Pts',(-55.7870229324165,-111.144767838626,
175.99212473304));
#16549=CARTESIAN_POINT('Ctrl Pts',(-55.7870004522962,-111.144559817836,
175.989365651051));
#16550=CARTESIAN_POINT('Ctrl Pts',(-55.7869897994373,-111.144461241134,
175.988058179796));
#16551=CARTESIAN_POINT('Ctrl Pts',(-55.7869792403406,-111.144363532218,
175.986758281555));
#16552=CARTESIAN_POINT('Ctrl Pts',(-55.7869689268157,-111.144268095849,
175.985484943511));
#16553=CARTESIAN_POINT('Ctrl Pts',(-55.7869624231925,-111.144207914466,
175.98468198711));
#16554=CARTESIAN_POINT('Ctrl Pts',(-55.7869560149882,-111.144148616101,
175.983889593831));
#16555=CARTESIAN_POINT('Ctrl Pts',(-55.7869497397808,-111.144090548475,
175.983112525094));
#16556=CARTESIAN_POINT('Ctrl Pts',(-55.7869283414167,-111.143892538734,
175.980462732245));
#16557=CARTESIAN_POINT('Ctrl Pts',(-55.7869070495478,-111.143695515059,
175.977812867795));
#16558=CARTESIAN_POINT('Ctrl Pts',(-55.7868858643761,-111.143499479302,
175.975162926479));
#16559=CARTESIAN_POINT('Ctrl Pts',(-55.7868496261866,-111.143164151318,
175.970630082616));
#16560=CARTESIAN_POINT('Ctrl Pts',(-55.7868137003751,-111.142831715664,
175.966097037108));
#16561=CARTESIAN_POINT('Ctrl Pts',(-55.7867780879403,-111.142502181493,
175.961563763315));
#16562=CARTESIAN_POINT('Ctrl Pts',(-55.7866367441066,-111.141194278134,
175.94357144406));
#16563=CARTESIAN_POINT('Ctrl Pts',(-55.786500346155,-111.13993216747,175.925576725693));
#16564=CARTESIAN_POINT('Ctrl Pts',(-55.7863689538889,-111.138716397416,
175.90757786131));
#16565=CARTESIAN_POINT('Ctrl Pts',(-55.7859262399947,-111.134619974459,
175.84693237906));
#16566=CARTESIAN_POINT('Ctrl Pts',(-55.785540741415,-111.131053222404,175.786292696376));
#16567=CARTESIAN_POINT('Ctrl Pts',(-55.7852143761284,-111.128033707311,
175.725582395189));
#16568=CARTESIAN_POINT('Ctrl Pts',(-55.7838829914684,-111.115715803902,
175.477918911893));
#16569=CARTESIAN_POINT('Ctrl Pts',(-55.7835587254065,-111.112716714097,
175.233343306962));
#16570=CARTESIAN_POINT('Ctrl Pts',(-55.7842612734033,-111.119216054728,
174.985485069079));
#16571=CARTESIAN_POINT('',(-55.7498389523163,-110.801299724063,176.985485069079));
#16572=CARTESIAN_POINT('Ctrl Pts',(-55.7498389523163,-110.801299724063,
176.985485069079));
#16573=CARTESIAN_POINT('Ctrl Pts',(-55.7668185587566,-110.957859362734,
176.98548506908));
#16574=CARTESIAN_POINT('Ctrl Pts',(-55.7837570912844,-111.114424255627,
176.985485069079));
#16575=CARTESIAN_POINT('Ctrl Pts',(-55.8006548129149,-111.270994369097,
176.985485069079));
#16576=CARTESIAN_POINT('',(-55.7333536026738,-110.64941790035,174.985485069079));
#16577=CARTESIAN_POINT('Ctrl Pts',(-55.7333536026738,-110.64941790035,174.985485069079));
#16578=CARTESIAN_POINT('Ctrl Pts',(-55.7372834331241,-110.685595265291,
175.195807752872));
#16579=CARTESIAN_POINT('Ctrl Pts',(-55.7406814496559,-110.716897508472,
175.407178770022));
#16580=CARTESIAN_POINT('Ctrl Pts',(-55.7433327290313,-110.741328193525,
175.619578568996));
#16581=CARTESIAN_POINT('Ctrl Pts',(-55.7442914854839,-110.750162825271,
175.696386648785));
#16582=CARTESIAN_POINT('Ctrl Pts',(-55.7451515103665,-110.758088892097,
175.773224689473));
#16583=CARTESIAN_POINT('Ctrl Pts',(-55.7459059204445,-110.765042260031,
175.850232063412));
#16584=CARTESIAN_POINT('Ctrl Pts',(-55.7462523324549,-110.768235125867,
175.885592512583));
#16585=CARTESIAN_POINT('Ctrl Pts',(-55.7465762177677,-110.771220523207,
175.920962194947));
#16586=CARTESIAN_POINT('Ctrl Pts',(-55.7468770555128,-110.773993592097,
175.956358578691));
#16587=CARTESIAN_POINT('Ctrl Pts',(-55.7469241848152,-110.774428021633,
175.961903783369));
#16588=CARTESIAN_POINT('Ctrl Pts',(-55.746970746089,-110.77485721814,175.967449362544));
#16589=CARTESIAN_POINT('Ctrl Pts',(-55.7470167375474,-110.775281164934,
175.972995388113));
#16590=CARTESIAN_POINT('Ctrl Pts',(-55.7470405191156,-110.775500382153,
175.975863163782));
#16591=CARTESIAN_POINT('Ctrl Pts',(-55.7470641481921,-110.775718194464,
175.978731042493));
#16592=CARTESIAN_POINT('Ctrl Pts',(-55.7470876245358,-110.775934599617,
175.981599034278));
#16593=CARTESIAN_POINT('Ctrl Pts',(-55.7470982974718,-110.776032982839,
175.982902895442));
#16594=CARTESIAN_POINT('Ctrl Pts',(-55.7471089431013,-110.776131114505,
175.984207354532));
#16595=CARTESIAN_POINT('Ctrl Pts',(-55.7471193391274,-110.776226945462,
175.985484943485));
#16596=CARTESIAN_POINT('Ctrl Pts',(-55.7471278543292,-110.77630543891,175.986531394086));
#16597=CARTESIAN_POINT('Ctrl Pts',(-55.747136205884,-110.776382423951,175.987559814951));
#16598=CARTESIAN_POINT('Ctrl Pts',(-55.7471442735878,-110.776456792525,
175.988555110492));
#16599=CARTESIAN_POINT('Ctrl Pts',(-55.7471656873326,-110.776654185699,
175.991196878856));
#16600=CARTESIAN_POINT('Ctrl Pts',(-55.7471869945963,-110.776850597934,
175.993838718488));
#16601=CARTESIAN_POINT('Ctrl Pts',(-55.7472081951813,-110.777046027391,
175.996480634583));
#16602=CARTESIAN_POINT('Ctrl Pts',(-55.7472443395524,-110.777379210404,
176.000984774238));
#16603=CARTESIAN_POINT('Ctrl Pts',(-55.7472801736672,-110.777709535178,
176.005489113248));
#16604=CARTESIAN_POINT('Ctrl Pts',(-55.7473156965597,-110.77803699272,176.009993677794));
#16605=CARTESIAN_POINT('Ctrl Pts',(-55.7474552321236,-110.779323261079,
176.027687815538));
#16606=CARTESIAN_POINT('Ctrl Pts',(-55.7475899566659,-110.780565206319,
176.045384291183));
#16607=CARTESIAN_POINT('Ctrl Pts',(-55.7477198140849,-110.781762306068,
176.063084767689));
#16608=CARTESIAN_POINT('Ctrl Pts',(-55.7481667684031,-110.785882585879,
176.124007774403));
#16609=CARTESIAN_POINT('Ctrl Pts',(-55.7485556725842,-110.789467988468,
176.184924768193));
#16610=CARTESIAN_POINT('Ctrl Pts',(-55.7488846099061,-110.792500660407,
176.245913294751));
#16611=CARTESIAN_POINT('Ctrl Pts',(-55.7502194176992,-110.804807060041,
176.493401053396));
#16612=CARTESIAN_POINT('Ctrl Pts',(-55.7505439219598,-110.807799862509,
176.737802780905));
#16613=CARTESIAN_POINT('Ctrl Pts',(-55.7498389523165,-110.801299724063,
176.985485069079));
#16614=CARTESIAN_POINT('Ctrl Pts',(-55.7842612734031,-111.119216054728,
174.985485069079));
#16615=CARTESIAN_POINT('Ctrl Pts',(-55.7673330881313,-110.962611747484,
174.985485069079));
#16616=CARTESIAN_POINT('Ctrl Pts',(-55.750363952816,-110.806012352105,174.985485069079));
#16617=CARTESIAN_POINT('Ctrl Pts',(-55.7333536026738,-110.64941790035,174.985485069079));
#16618=CARTESIAN_POINT('Ctrl Pts',(-55.6389642047373,-109.784410209239,
176.985485069079));
#16619=CARTESIAN_POINT('Ctrl Pts',(-55.6389642047373,-109.784410209239,
174.585485069079));
#16620=CARTESIAN_POINT('Ctrl Pts',(-55.6158587430936,-109.573622204912,
176.985485069079));
#16621=CARTESIAN_POINT('Ctrl Pts',(-55.6158587430936,-109.573622204912,
174.585485069079));
#16622=CARTESIAN_POINT('Ctrl Pts',(-55.5927270839073,-109.363293887315,
176.98548506908));
#16623=CARTESIAN_POINT('Ctrl Pts',(-55.5927270839073,-109.363293887315,
174.58548506908));
#16624=CARTESIAN_POINT('Ctrl Pts',(-55.5695693845384,-109.153423842286,
176.98548506908));
#16625=CARTESIAN_POINT('Ctrl Pts',(-55.5695693845384,-109.153423842286,
174.58548506908));
#16626=CARTESIAN_POINT('',(-55.6385532352656,-109.780661063962,176.985485069079));
#16627=CARTESIAN_POINT('',(-55.6219312570818,-109.629147380551,174.985485069079));
#16628=CARTESIAN_POINT('Ctrl Pts',(-55.6385532352656,-109.780661063962,
176.985485069079));
#16629=CARTESIAN_POINT('Ctrl Pts',(-55.6364090528804,-109.761100746612,
176.871529272123));
#16630=CARTESIAN_POINT('Ctrl Pts',(-55.6344206303383,-109.742967391913,
176.757244549389));
#16631=CARTESIAN_POINT('Ctrl Pts',(-55.632624701929,-109.726593308319,176.64274596629));
#16632=CARTESIAN_POINT('Ctrl Pts',(-55.6302616254732,-109.705048345154,
176.492089122433));
#16633=CARTESIAN_POINT('Ctrl Pts',(-55.6282354868976,-109.686582603912,
176.34130394811));
#16634=CARTESIAN_POINT('Ctrl Pts',(-55.6266116662059,-109.671786190867,
176.189750722006));
#16635=CARTESIAN_POINT('Ctrl Pts',(-55.626204109179,-109.668072491355,176.151712912431));
#16636=CARTESIAN_POINT('Ctrl Pts',(-55.6258222679447,-109.664593332989,
176.113663047176));
#16637=CARTESIAN_POINT('Ctrl Pts',(-55.6254668827296,-109.661355382375,
176.07558107738));
#16638=CARTESIAN_POINT('Ctrl Pts',(-55.625268687235,-109.659549603192,176.054343067137));
#16639=CARTESIAN_POINT('Ctrl Pts',(-55.6250787727883,-109.657819324701,
176.033100724868));
#16640=CARTESIAN_POINT('Ctrl Pts',(-55.624897250403,-109.656165545924,176.011850174535));
#16641=CARTESIAN_POINT('Ctrl Pts',(-55.6248563305293,-109.655792741112,
176.007059746982));
#16642=CARTESIAN_POINT('Ctrl Pts',(-55.6248158382756,-109.655423834363,
176.002269038379));
#16643=CARTESIAN_POINT('Ctrl Pts',(-55.6247757748228,-109.655058836301,
175.997478002448));
#16644=CARTESIAN_POINT('Ctrl Pts',(-55.6247531302752,-109.654852533164,
175.994770027129));
#16645=CARTESIAN_POINT('Ctrl Pts',(-55.6247306228264,-109.654647479735,
175.992061960349));
#16646=CARTESIAN_POINT('Ctrl Pts',(-55.6247082526837,-109.654443677878,
175.989353793512));
#16647=CARTESIAN_POINT('Ctrl Pts',(-55.6246975274837,-109.654345966581,
175.988055382898));
#16648=CARTESIAN_POINT('Ctrl Pts',(-55.6246868325191,-109.654248530892,
175.986756735708));
#16649=CARTESIAN_POINT('Ctrl Pts',(-55.6246763889997,-109.654153386119,
175.985484943368));
#16650=CARTESIAN_POINT('Ctrl Pts',(-55.6246679437789,-109.654076446671,
175.984456500102));
#16651=CARTESIAN_POINT('Ctrl Pts',(-55.624659659271,-109.654000971477,175.983445620473));
#16652=CARTESIAN_POINT('Ctrl Pts',(-55.6246516506085,-109.653928009428,
175.98246663173));
#16653=CARTESIAN_POINT('Ctrl Pts',(-55.6246288764581,-109.653720528006,
175.97968269159));
#16654=CARTESIAN_POINT('Ctrl Pts',(-55.6246062215329,-109.653514133448,
175.976898672936));
#16655=CARTESIAN_POINT('Ctrl Pts',(-55.6245836860687,-109.653308827883,
175.974114569615));
#16656=CARTESIAN_POINT('Ctrl Pts',(-55.6245420900418,-109.652929874262,
175.968975663425));
#16657=CARTESIAN_POINT('Ctrl Pts',(-55.624500901285,-109.652554633264,175.963836501813));
#16658=CARTESIAN_POINT('Ctrl Pts',(-55.6244601212647,-109.65218311812,175.958697045889));
#16659=CARTESIAN_POINT('Ctrl Pts',(-55.6242482374254,-109.650252808753,
175.931993585618));
#16660=CARTESIAN_POINT('Ctrl Pts',(-55.6240474178744,-109.64842335603,175.90528595974));
#16661=CARTESIAN_POINT('Ctrl Pts',(-55.623857856037,-109.646696504493,175.878568359176));
#16662=CARTESIAN_POINT('Ctrl Pts',(-55.6234970668234,-109.643409822864,
175.827717290019));
#16663=CARTESIAN_POINT('Ctrl Pts',(-55.6231773197003,-109.640497190402,
175.776866909026));
#16664=CARTESIAN_POINT('Ctrl Pts',(-55.6228997282151,-109.637968646638,
175.725971544764));
#16665=CARTESIAN_POINT('Ctrl Pts',(-55.6215482370463,-109.62565809408,175.478180675772));
#16666=CARTESIAN_POINT('Ctrl Pts',(-55.6212187388722,-109.622657747841,
175.233470911589));
#16667=CARTESIAN_POINT('Ctrl Pts',(-55.6219312570821,-109.629147380551,
174.985485069079));
#16668=CARTESIAN_POINT('',(-55.586709713872,-109.308887482778,176.985485069079));
#16669=CARTESIAN_POINT('Ctrl Pts',(-55.586709713872,-109.308887482778,176.985485069079));
#16670=CARTESIAN_POINT('Ctrl Pts',(-55.6040331133308,-109.466139941617,
176.985485069079));
#16671=CARTESIAN_POINT('Ctrl Pts',(-55.6213141953808,-109.623397813748,
176.985485069079));
#16672=CARTESIAN_POINT('Ctrl Pts',(-55.6385532352656,-109.780661063962,
176.985485069079));
#16673=CARTESIAN_POINT('',(-55.5699812776309,-109.157156757027,174.985485069079));
#16674=CARTESIAN_POINT('Ctrl Pts',(-55.5699812776309,-109.157156757027,
174.98548506908));
#16675=CARTESIAN_POINT('Ctrl Pts',(-55.5732866004807,-109.187112904902,
175.159804470874));
#16676=CARTESIAN_POINT('Ctrl Pts',(-55.5762218608553,-109.213729419147,
175.334889205444));
#16677=CARTESIAN_POINT('Ctrl Pts',(-55.578660281489,-109.235847109079,175.510572458271));
#16678=CARTESIAN_POINT('Ctrl Pts',(-55.5801069603974,-109.248969207492,
175.614802734586));
#16679=CARTESIAN_POINT('Ctrl Pts',(-55.5813766993776,-109.260489063237,
175.71907795542));
#16680=CARTESIAN_POINT('Ctrl Pts',(-55.5824505396604,-109.270232848391,
175.82369743394));
#16681=CARTESIAN_POINT('Ctrl Pts',(-55.5829005685282,-109.274316309098,
175.867541743207));
#16682=CARTESIAN_POINT('Ctrl Pts',(-55.5833156970086,-109.278083353021,
175.911397741191));
#16683=CARTESIAN_POINT('Ctrl Pts',(-55.5836948941706,-109.281524510865,
175.955298099187));
#16684=CARTESIAN_POINT('Ctrl Pts',(-55.5837453433951,-109.281982330074,
175.961138699377));
#16685=CARTESIAN_POINT('Ctrl Pts',(-55.5837951534157,-109.282434351904,
175.966979712571));
#16686=CARTESIAN_POINT('Ctrl Pts',(-55.5838443221141,-109.282880556884,
175.972821222537));
#16687=CARTESIAN_POINT('Ctrl Pts',(-55.583868966911,-109.283104207936,175.975749159043));
#16688=CARTESIAN_POINT('Ctrl Pts',(-55.5838934504385,-109.283326396259,
175.978677202591));
#16689=CARTESIAN_POINT('Ctrl Pts',(-55.5839177724371,-109.283547119468,
175.981605363915));
#16690=CARTESIAN_POINT('Ctrl Pts',(-55.5839285834645,-109.283645230017,
175.982906919464));
#16691=CARTESIAN_POINT('Ctrl Pts',(-55.5839393686461,-109.283743106169,
175.984209282882));
#16692=CARTESIAN_POINT('Ctrl Pts',(-55.5839499020231,-109.283838697322,
175.985484943316));
#16693=CARTESIAN_POINT('Ctrl Pts',(-55.5839585992817,-109.283917625569,
175.986538237873));
#16694=CARTESIAN_POINT('Ctrl Pts',(-55.5839671287816,-109.283995031492,
175.987573324793));
#16695=CARTESIAN_POINT('Ctrl Pts',(-55.583975365368,-109.284069779287,175.988574716349));
#16696=CARTESIAN_POINT('Ctrl Pts',(-55.5839967509971,-109.284263855878,
175.991174748357));
#16697=CARTESIAN_POINT('Ctrl Pts',(-55.5840180319528,-109.284456983142,
175.993774849365));
#16698=CARTESIAN_POINT('Ctrl Pts',(-55.584039208044,-109.284649159328,175.996375024287));
#16699=CARTESIAN_POINT('Ctrl Pts',(-55.5840744020402,-109.28496855009,176.000696433042));
#16700=CARTESIAN_POINT('Ctrl Pts',(-55.5841093062199,-109.285285312331,
176.005018025533));
#16701=CARTESIAN_POINT('Ctrl Pts',(-55.584143919719,-109.285599438132,176.009339824886));
#16702=CARTESIAN_POINT('Ctrl Pts',(-55.5842698791708,-109.286742550346,
176.02506696862));
#16703=CARTESIAN_POINT('Ctrl Pts',(-55.5843919827929,-109.287850690552,
176.040796041382));
#16704=CARTESIAN_POINT('Ctrl Pts',(-55.5845101904938,-109.288923491222,
176.0565282034));
#16705=CARTESIAN_POINT('Ctrl Pts',(-55.584960025238,-109.293005991866,176.116396325553));
#16706=CARTESIAN_POINT('Ctrl Pts',(-55.5853530717745,-109.296573366859,
176.176259980973));
#16707=CARTESIAN_POINT('Ctrl Pts',(-55.5856874617408,-109.299608482482,
176.236191992831));
#16708=CARTESIAN_POINT('Ctrl Pts',(-55.5870865691322,-109.312307585713,
176.486951074261));
#16709=CARTESIAN_POINT('Ctrl Pts',(-55.5874344793557,-109.315466512178,
176.73451470052));
#16710=CARTESIAN_POINT('Ctrl Pts',(-55.5867097138723,-109.308887482778,
176.985485069079));
#16711=CARTESIAN_POINT('Ctrl Pts',(-55.6219312570818,-109.629147380551,
174.985485069079));
#16712=CARTESIAN_POINT('Ctrl Pts',(-55.6046568968532,-109.47181209897,174.985485069079));
#16713=CARTESIAN_POINT('Ctrl Pts',(-55.5873403294727,-109.314481880041,
174.985485069079));
#16714=CARTESIAN_POINT('Ctrl Pts',(-55.5699812776309,-109.157156757027,
174.985485069079));
#16715=CARTESIAN_POINT('Ctrl Pts',(-54.9656605004213,-103.833027927217,
176.985485069079));
#16716=CARTESIAN_POINT('Ctrl Pts',(-54.9656605004213,-103.833027927217,
174.585485069079));
#16717=CARTESIAN_POINT('Ctrl Pts',(-54.9401779838911,-103.614774580036,
176.985485069079));
#16718=CARTESIAN_POINT('Ctrl Pts',(-54.9401779838911,-103.614774580036,
174.585485069079));
#16719=CARTESIAN_POINT('Ctrl Pts',(-54.914666672271,-103.39704157916,176.985485069079));
#16720=CARTESIAN_POINT('Ctrl Pts',(-54.914666672271,-103.39704157916,174.585485069079));
#16721=CARTESIAN_POINT('Ctrl Pts',(-54.8891267634922,-103.179827143433,
176.985485069079));
#16722=CARTESIAN_POINT('Ctrl Pts',(-54.8891267634922,-103.179827143433,
174.585485069079));
#16723=CARTESIAN_POINT('',(-54.9652072510433,-103.829146005559,176.985485069079));
#16724=CARTESIAN_POINT('',(-54.9477711935236,-103.67993499333,174.985485069079));
#16725=CARTESIAN_POINT('Ctrl Pts',(-54.9652072510433,-103.829146005559,
176.985485069079));
#16726=CARTESIAN_POINT('Ctrl Pts',(-54.9603446400948,-103.787500319099,
176.739490147077));
#16727=CARTESIAN_POINT('Ctrl Pts',(-54.9562599984868,-103.752545584536,
176.492377432739));
#16728=CARTESIAN_POINT('Ctrl Pts',(-54.9532994998274,-103.727218214377,
176.24352953951));
#16729=CARTESIAN_POINT('Ctrl Pts',(-54.9525165046112,-103.720519609866,
176.177714035987));
#16730=CARTESIAN_POINT('Ctrl Pts',(-54.951813145893,-103.714503021022,176.111882747266));
#16731=CARTESIAN_POINT('Ctrl Pts',(-54.9511933972497,-103.709202033452,
176.045936596505));
#16732=CARTESIAN_POINT('Ctrl Pts',(-54.9510769059183,-103.708205630948,
176.033540998729));
#16733=CARTESIAN_POINT('Ctrl Pts',(-54.9509633911318,-103.70723470415,176.02114375147));
#16734=CARTESIAN_POINT('Ctrl Pts',(-54.9508528746203,-103.706289436525,
176.008744093197));
#16735=CARTESIAN_POINT('Ctrl Pts',(-54.9508174843107,-103.705986736833,
176.004773394702));
#16736=CARTESIAN_POINT('Ctrl Pts',(-54.950782401975,-103.705686672774,176.000802506865));
#16737=CARTESIAN_POINT('Ctrl Pts',(-54.9507476282943,-103.705389250096,
175.996831404116));
#16738=CARTESIAN_POINT('Ctrl Pts',(-54.9507254845137,-103.705199852184,
175.99430261723));
#16739=CARTESIAN_POINT('Ctrl Pts',(-54.9507034659822,-103.705011526117,
175.991773753038));
#16740=CARTESIAN_POINT('Ctrl Pts',(-54.9506815728693,-103.704824273326,
175.989244804546));
#16741=CARTESIAN_POINT('Ctrl Pts',(-54.9506706715899,-103.704731034188,
175.987985560415));
#16742=CARTESIAN_POINT('Ctrl Pts',(-54.9506597749779,-103.704637835112,
175.986723190717));
#16743=CARTESIAN_POINT('Ctrl Pts',(-54.9506491166976,-103.704546674627,
175.985484941713));
#16744=CARTESIAN_POINT('Ctrl Pts',(-54.9506394019653,-103.704463584327,
175.984356311458));
#16745=CARTESIAN_POINT('Ctrl Pts',(-54.9506298806488,-103.70438214843,175.983247723187));
#16746=CARTESIAN_POINT('Ctrl Pts',(-54.9506207267441,-103.704303855104,
175.982179810625));
#16747=CARTESIAN_POINT('Ctrl Pts',(-54.9505941095538,-103.704076198336,
175.97907459676));
#16748=CARTESIAN_POINT('Ctrl Pts',(-54.9505676481464,-103.703849874815,
175.975969288503));
#16749=CARTESIAN_POINT('Ctrl Pts',(-54.9505413428546,-103.703624887355,
175.972863877515));
#16750=CARTESIAN_POINT('Ctrl Pts',(-54.9504845796731,-103.703139395535,
175.966162830107));
#16751=CARTESIAN_POINT('Ctrl Pts',(-54.9504285440011,-103.702660129853,
175.959461372579));
#16752=CARTESIAN_POINT('Ctrl Pts',(-54.9503732391284,-103.702187118158,
175.952759420293));
#16753=CARTESIAN_POINT('Ctrl Pts',(-54.9497915780554,-103.697212285439,
175.88227259756));
#16754=CARTESIAN_POINT('Ctrl Pts',(-54.9492913032303,-103.692933925243,
175.811797486704));
#16755=CARTESIAN_POINT('Ctrl Pts',(-54.9488756720445,-103.689379602438,
175.741221887012));
#16756=CARTESIAN_POINT('Ctrl Pts',(-54.9473863602973,-103.676643564123,
175.488331648524));
#16757=CARTESIAN_POINT('Ctrl Pts',(-54.9470101313529,-103.673427333826,
175.238593067858));
#16758=CARTESIAN_POINT('Ctrl Pts',(-54.9477711935239,-103.67993499333,174.985485069079));
#16759=CARTESIAN_POINT('',(-54.9071900358701,-103.333580645004,176.985485069079));
#16760=CARTESIAN_POINT('Ctrl Pts',(-54.9071900358701,-103.333580645004,
176.985485069079));
#16761=CARTESIAN_POINT('Ctrl Pts',(-54.9265798996307,-103.498762601146,
176.985485069079));
#16762=CARTESIAN_POINT('Ctrl Pts',(-54.9459188500188,-103.663951070186,
176.985485069079));
#16763=CARTESIAN_POINT('Ctrl Pts',(-54.9652072510433,-103.829146005559,
176.985485069079));
#16764=CARTESIAN_POINT('',(-54.8895810276286,-103.183690695987,174.985485069079));
#16765=CARTESIAN_POINT('Ctrl Pts',(-54.8895810276286,-103.183690695987,
174.985485069079));
#16766=CARTESIAN_POINT('Ctrl Pts',(-54.894579533373,-103.226204268245,175.235671327022));
#16767=CARTESIAN_POINT('Ctrl Pts',(-54.8987611854365,-103.261799603572,
175.487040663794));
#16768=CARTESIAN_POINT('Ctrl Pts',(-54.9017619269949,-103.287350165154,
175.740218794686));
#16769=CARTESIAN_POINT('Ctrl Pts',(-54.9025899334085,-103.294400432046,
175.810079231545));
#16770=CARTESIAN_POINT('Ctrl Pts',(-54.9033268465538,-103.300675857414,
175.87995195485));
#16771=CARTESIAN_POINT('Ctrl Pts',(-54.9039680529975,-103.306136673011,
175.949958567431));
#16772=CARTESIAN_POINT('Ctrl Pts',(-54.9040354843144,-103.306710949815,
175.957320686338));
#16773=CARTESIAN_POINT('Ctrl Pts',(-54.9041018493881,-103.307276151311,
175.964683431554));
#16774=CARTESIAN_POINT('Ctrl Pts',(-54.904167143829,-103.307832239617,175.972046966102));
#16775=CARTESIAN_POINT('Ctrl Pts',(-54.9041956515931,-103.30807502957,175.975261909108));
#16776=CARTESIAN_POINT('Ctrl Pts',(-54.9042239550488,-103.308316080457,
175.978476977567));
#16777=CARTESIAN_POINT('Ctrl Pts',(-54.9042520538418,-103.308555389218,
175.981692185214));
#16778=CARTESIAN_POINT('Ctrl Pts',(-54.9042631575422,-103.308649956013,
175.982962727421));
#16779=CARTESIAN_POINT('Ctrl Pts',(-54.9042742534349,-103.308744456458,
175.984236107471));
#16780=CARTESIAN_POINT('Ctrl Pts',(-54.904285104508,-103.308836871984,175.98548494154));
#16781=CARTESIAN_POINT('Ctrl Pts',(-54.9042948652852,-103.308920001767,
175.986608295046));
#16782=CARTESIAN_POINT('Ctrl Pts',(-54.9043044325544,-103.30900148361,175.987711784495));
#16783=CARTESIAN_POINT('Ctrl Pts',(-54.9043136366808,-103.30907987276,175.988775477043));
#16784=CARTESIAN_POINT('Ctrl Pts',(-54.9043349662627,-103.309261531262,
175.991240471174));
#16785=CARTESIAN_POINT('Ctrl Pts',(-54.9043561967022,-103.309442345925,
175.993705526031));
#16786=CARTESIAN_POINT('Ctrl Pts',(-54.9043773278324,-103.309622315315,
175.99617064576));
#16787=CARTESIAN_POINT('Ctrl Pts',(-54.9044093023417,-103.309894635484,
175.999900734628));
#16788=CARTESIAN_POINT('Ctrl Pts',(-54.904441049357,-103.31016501933,176.003630958694));
#16789=CARTESIAN_POINT('Ctrl Pts',(-54.9044725683072,-103.31043346194,176.0073613325));
#16790=CARTESIAN_POINT('Ctrl Pts',(-54.9045625504215,-103.311199827362,
176.018011018467));
#16791=CARTESIAN_POINT('Ctrl Pts',(-54.9046506715745,-103.311950352705,
176.028661666441));
#16792=CARTESIAN_POINT('Ctrl Pts',(-54.9047369188309,-103.312684926642,
176.039313624502));
#16793=CARTESIAN_POINT('Ctrl Pts',(-54.9052649957913,-103.317182595187,
176.104533712293));
#16794=CARTESIAN_POINT('Ctrl Pts',(-54.9057223621618,-103.321078338012,
176.169746019421));
#16795=CARTESIAN_POINT('Ctrl Pts',(-54.9061064975074,-103.324350456313,
176.235041316554));
#16796=CARTESIAN_POINT('Ctrl Pts',(-54.9075838256808,-103.336934543165,
176.486157448245));
#16797=CARTESIAN_POINT('Ctrl Pts',(-54.9079526518267,-103.340077358802,
176.73415655439));
#16798=CARTESIAN_POINT('Ctrl Pts',(-54.9071900358704,-103.333580645004,
176.985485069079));
#16799=CARTESIAN_POINT('Ctrl Pts',(-54.9477711935236,-103.67993499333,174.985485069079));
#16800=CARTESIAN_POINT('Ctrl Pts',(-54.928425440487,-103.514514113942,174.985485069079));
#16801=CARTESIAN_POINT('Ctrl Pts',(-54.9090288411297,-103.349099333454,
174.985485069079));
#16802=CARTESIAN_POINT('Ctrl Pts',(-54.8895810276286,-103.183690695987,
174.985485069079));
#16803=CARTESIAN_POINT('Ctrl Pts',(-55.1378236961386,-105.319345570968,
176.985485069079));
#16804=CARTESIAN_POINT('Ctrl Pts',(-55.1378236961386,-105.319345570968,
174.585485069079));
#16805=CARTESIAN_POINT('Ctrl Pts',(-55.1130435723412,-105.103705439537,
176.985485069079));
#16806=CARTESIAN_POINT('Ctrl Pts',(-55.1130435723412,-105.103705439537,
174.585485069079));
#16807=CARTESIAN_POINT('Ctrl Pts',(-55.0882355096573,-104.888566306789,
176.985485069079));
#16808=CARTESIAN_POINT('Ctrl Pts',(-55.0882355096573,-104.888566306789,
174.585485069079));
#16809=CARTESIAN_POINT('Ctrl Pts',(-55.0633996930072,-104.673926509197,
176.985485069079));
#16810=CARTESIAN_POINT('Ctrl Pts',(-55.0633996930072,-104.673926509197,
174.585485069079));
#16811=CARTESIAN_POINT('',(-55.1373829400023,-105.315510127391,176.985485069079));
#16812=CARTESIAN_POINT('',(-55.1201342919917,-105.165536169418,174.985485069079));
#16813=CARTESIAN_POINT('Ctrl Pts',(-55.1373829400023,-105.315510127391,
176.985485069079));
#16814=CARTESIAN_POINT('Ctrl Pts',(-55.1325913532206,-105.273814769704,
176.740328641451));
#16815=CARTESIAN_POINT('Ctrl Pts',(-55.1285604769881,-105.238766921808,
176.494015528965));
#16816=CARTESIAN_POINT('Ctrl Pts',(-55.1256334249619,-105.213324102528,
176.245996586915));
#16817=CARTESIAN_POINT('Ctrl Pts',(-55.1248690958891,-105.206680323636,
176.181232419308));
#16818=CARTESIAN_POINT('Ctrl Pts',(-55.1241809619153,-105.200699557015,
176.116451480769));
#16819=CARTESIAN_POINT('Ctrl Pts',(-55.12357283239,-105.195414522072,176.051559076556));
#16820=CARTESIAN_POINT('Ctrl Pts',(-55.1234413510252,-105.194271864828,
176.037528937381));
#16821=CARTESIAN_POINT('Ctrl Pts',(-55.1233136386414,-105.193161983333,
176.023496715598));
#16822=CARTESIAN_POINT('Ctrl Pts',(-55.1231897269403,-105.192085149581,
176.009461299477));
#16823=CARTESIAN_POINT('Ctrl Pts',(-55.123153026971,-105.191766214683,176.005304312389));
#16824=CARTESIAN_POINT('Ctrl Pts',(-55.1231166610312,-105.191450184242,
176.001147116187));
#16825=CARTESIAN_POINT('Ctrl Pts',(-55.1230806299025,-105.191137064961,
175.996989681169));
#16826=CARTESIAN_POINT('Ctrl Pts',(-55.1230583616824,-105.190943548706,
175.994420272955));
#16827=CARTESIAN_POINT('Ctrl Pts',(-55.1230362214369,-105.190751145181,
175.991850784019));
#16828=CARTESIAN_POINT('Ctrl Pts',(-55.1230142093449,-105.19055985592,175.989281207067));
#16829=CARTESIAN_POINT('Ctrl Pts',(-55.1230033113244,-105.190465150052,
175.988009028935));
#16830=CARTESIAN_POINT('Ctrl Pts',(-55.1229924249308,-105.190370545369,
175.986734466882));
#16831=CARTESIAN_POINT('Ctrl Pts',(-55.1229817827353,-105.190278062947,
175.985484942294));
#16832=CARTESIAN_POINT('Ctrl Pts',(-55.1229724066987,-105.190196583653,
175.984384080328));
#16833=CARTESIAN_POINT('Ctrl Pts',(-55.1229632158595,-105.190116713862,
175.983302655394));
#16834=CARTESIAN_POINT('Ctrl Pts',(-55.122954366653,-105.190039813004,175.982259421452));
#16835=CARTESIAN_POINT('Ctrl Pts',(-55.1229288184682,-105.189817795657,
175.979247543101));
#16836=CARTESIAN_POINT('Ctrl Pts',(-55.122903415208,-105.189597038515,175.976235574927));
#16837=CARTESIAN_POINT('Ctrl Pts',(-55.1228781571759,-105.189377544189,
175.973223509272));
#16838=CARTESIAN_POINT('Ctrl Pts',(-55.1228259520709,-105.188923877635,
175.966997956796));
#16839=CARTESIAN_POINT('Ctrl Pts',(-55.1227743678426,-105.188475609844,
175.960772043696));
#16840=CARTESIAN_POINT('Ctrl Pts',(-55.1227234071325,-105.188032763539,
175.95454570169));
#16841=CARTESIAN_POINT('Ctrl Pts',(-55.1222451085664,-105.183876370262,
175.896107535319));
#16842=CARTESIAN_POINT('Ctrl Pts',(-55.1218220467802,-105.18020025562,175.837669539353));
#16843=CARTESIAN_POINT('Ctrl Pts',(-55.1214561353611,-105.177020875394,
175.779168406242));
#16844=CARTESIAN_POINT('Ctrl Pts',(-55.1204759308218,-105.168503942696,
175.622455406208));
#16845=CARTESIAN_POINT('Ctrl Pts',(-55.119912702985,-105.16361104624,175.46638507564));
#16846=CARTESIAN_POINT('Ctrl Pts',(-55.1197837579081,-105.162490824725,
175.309429212081));
#16847=CARTESIAN_POINT('Ctrl Pts',(-55.1196949631213,-105.161719412329,
175.201345500861));
#16848=CARTESIAN_POINT('Ctrl Pts',(-55.1198126567061,-105.162741844194,
175.093530246589));
#16849=CARTESIAN_POINT('Ctrl Pts',(-55.120134291992,-105.165536169417,174.985485069079));
#16850=CARTESIAN_POINT('',(-55.0812452693713,-104.828281539026,176.985485069079));
#16851=CARTESIAN_POINT('Ctrl Pts',(-55.0812452693713,-104.828281539026,
176.985485069079));
#16852=CARTESIAN_POINT('Ctrl Pts',(-55.1000058573857,-104.990684924282,
176.985485069079));
#16853=CARTESIAN_POINT('Ctrl Pts',(-55.118718302742,-105.153094468003,176.985485069079));
#16854=CARTESIAN_POINT('Ctrl Pts',(-55.1373829400023,-105.315510127391,
176.985485069079));
#16855=CARTESIAN_POINT('',(-55.0638414338548,-104.677744265764,174.985485069079));
#16856=CARTESIAN_POINT('Ctrl Pts',(-55.0638414338548,-104.677744265764,
174.985485069079));
#16857=CARTESIAN_POINT('Ctrl Pts',(-55.0687838687883,-104.720460258196,
175.235872171748));
#16858=CARTESIAN_POINT('Ctrl Pts',(-55.0729207002077,-104.756243083222,
175.487478675512));
#16859=CARTESIAN_POINT('Ctrl Pts',(-55.075887709271,-104.781914641058,175.740891960796));
#16860=CARTESIAN_POINT('Ctrl Pts',(-55.0767089826743,-104.789020574078,
175.811037210384));
#16861=CARTESIAN_POINT('Ctrl Pts',(-55.0774394594947,-104.795341706919,
175.881194595647));
#16862=CARTESIAN_POINT('Ctrl Pts',(-55.0780744901831,-104.800837317194,
175.951488371148));
#16863=CARTESIAN_POINT('Ctrl Pts',(-55.078137016347,-104.801378424002,175.958409611662));
#16864=CARTESIAN_POINT('Ctrl Pts',(-55.0781986103504,-104.801911468507,
175.96533141422));
#16865=CARTESIAN_POINT('Ctrl Pts',(-55.0782592685639,-104.802436418886,
175.972253915646));
#16866=CARTESIAN_POINT('Ctrl Pts',(-55.0782867446598,-104.802674203452,
175.975389571999));
#16867=CARTESIAN_POINT('Ctrl Pts',(-55.0783140285515,-104.802910325545,
175.978525348855));
#16868=CARTESIAN_POINT('Ctrl Pts',(-55.0783411199121,-104.803144782296,
175.981661259125));
#16869=CARTESIAN_POINT('Ctrl Pts',(-55.0783521912824,-104.803240597252,
175.982942805102));
#16870=CARTESIAN_POINT('Ctrl Pts',(-55.0783632487692,-104.803336292205,
175.984226541533));
#16871=CARTESIAN_POINT('Ctrl Pts',(-55.07837405698,-104.803429829985,175.985484942154));
#16872=CARTESIAN_POINT('Ctrl Pts',(-55.0783835000685,-104.803511553552,
175.986584401511));
#16873=CARTESIAN_POINT('Ctrl Pts',(-55.0783927572475,-104.803591668305,
175.987664518065));
#16874=CARTESIAN_POINT('Ctrl Pts',(-55.078401674109,-104.803668837928,175.988706932021));
#16875=CARTESIAN_POINT('Ctrl Pts',(-55.0784230107973,-104.803853493056,
175.991201269499));
#16876=CARTESIAN_POINT('Ctrl Pts',(-55.0784442471903,-104.80403728074,175.993695669732));
#16877=CARTESIAN_POINT('Ctrl Pts',(-55.0784653831148,-104.804220199467,
175.996190136949));
#16878=CARTESIAN_POINT('Ctrl Pts',(-55.0784980879095,-104.804503239814,
176.000049965188));
#16879=CARTESIAN_POINT('Ctrl Pts',(-55.0785305520266,-104.804784198525,
176.003909939035));
#16880=CARTESIAN_POINT('Ctrl Pts',(-55.0785627748351,-104.805063070084,
176.007770074744));
#16881=CARTESIAN_POINT('Ctrl Pts',(-55.0786597880118,-104.805902668401,
176.01939178135));
#16882=CARTESIAN_POINT('Ctrl Pts',(-55.0787546111034,-104.806723323977,
176.031014620741));
#16883=CARTESIAN_POINT('Ctrl Pts',(-55.0788472273842,-104.807524890555,
176.042639049868));
#16884=CARTESIAN_POINT('Ctrl Pts',(-55.0793396929952,-104.811787035087,
176.104449258049));
#16885=CARTESIAN_POINT('Ctrl Pts',(-55.0797693684961,-104.815506036955,
176.166254628543));
#16886=CARTESIAN_POINT('Ctrl Pts',(-55.0801341086664,-104.818663131394,
176.228133032237));
#16887=CARTESIAN_POINT('Ctrl Pts',(-55.0816280794429,-104.831594547275,
176.481586132073));
#16888=CARTESIAN_POINT('Ctrl Pts',(-55.0820065361088,-104.834871540102,
176.731806878011));
#16889=CARTESIAN_POINT('Ctrl Pts',(-55.0812452693716,-104.828281539026,
176.985485069079));
#16890=CARTESIAN_POINT('Ctrl Pts',(-55.1201342919917,-105.165536169418,
174.985485069079));
#16891=CARTESIAN_POINT('Ctrl Pts',(-55.1014181855903,-105.00293308916,174.985485069079));
#16892=CARTESIAN_POINT('Ctrl Pts',(-55.0826540121559,-104.840335774435,
174.985485069079));
#16893=CARTESIAN_POINT('Ctrl Pts',(-55.0638414338548,-104.677744265764,
174.985485069079));
#16894=CARTESIAN_POINT('Ctrl Pts',(-55.3073953193163,-106.806696489204,
176.985485069079));
#16895=CARTESIAN_POINT('Ctrl Pts',(-55.3073953193163,-106.806696489204,
174.585485069079));
#16896=CARTESIAN_POINT('Ctrl Pts',(-55.2832425016958,-106.593163773849,
176.985485069079));
#16897=CARTESIAN_POINT('Ctrl Pts',(-55.2832425016958,-106.593163773849,
174.585485069079));
#16898=CARTESIAN_POINT('Ctrl Pts',(-55.2590624577512,-106.380115649896,
176.98548506908));
#16899=CARTESIAN_POINT('Ctrl Pts',(-55.2590624577512,-106.380115649896,
174.585485069079));
#16900=CARTESIAN_POINT('Ctrl Pts',(-55.2348553614763,-106.167550552635,
176.98548506908));
#16901=CARTESIAN_POINT('Ctrl Pts',(-55.2348553614763,-106.167550552635,
174.585485069079));
#16902=CARTESIAN_POINT('',(-55.3069657208749,-106.802898527582,176.985485069079));
#16903=CARTESIAN_POINT('',(-55.2899155902424,-106.652286416981,174.985485069079));
#16904=CARTESIAN_POINT('Ctrl Pts',(-55.3069657208749,-106.802898527582,
176.985485069079));
#16905=CARTESIAN_POINT('Ctrl Pts',(-55.3021846112535,-106.76063090408,176.7379137386));
#16906=CARTESIAN_POINT('Ctrl Pts',(-55.2981676012828,-106.725146921386,
176.489140583006));
#16907=CARTESIAN_POINT('Ctrl Pts',(-55.2952666343776,-106.699528891617,
176.238615443194));
#16908=CARTESIAN_POINT('Ctrl Pts',(-55.2945707003288,-106.693383196143,
176.178515145408));
#16909=CARTESIAN_POINT('Ctrl Pts',(-55.2939397417985,-106.687811887529,
176.118397421427));
#16910=CARTESIAN_POINT('Ctrl Pts',(-55.2933767926389,-106.682841442936,
176.058185956496));
#16911=CARTESIAN_POINT('Ctrl Pts',(-55.2932273308083,-106.681521800238,
176.042199937835));
#16912=CARTESIAN_POINT('Ctrl Pts',(-55.293082699797,-106.680244837964,176.026211274459));
#16913=CARTESIAN_POINT('Ctrl Pts',(-55.2929429467073,-106.679010966758,
176.010218314697));
#16914=CARTESIAN_POINT('Ctrl Pts',(-55.2929048856235,-106.678674927852,
176.005862708802));
#16915=CARTESIAN_POINT('Ctrl Pts',(-55.2928671871104,-106.678342091856,
176.001506871925));
#16916=CARTESIAN_POINT('Ctrl Pts',(-55.2928298520657,-106.678012466596,
175.997150769662));
#16917=CARTESIAN_POINT('Ctrl Pts',(-55.2928074568339,-106.677814742603,
175.994537784448));
#16918=CARTESIAN_POINT('Ctrl Pts',(-55.2927851924799,-106.677618174731,
175.99192471504));
#16919=CARTESIAN_POINT('Ctrl Pts',(-55.2927630591915,-106.677422764618,
175.989311553739));
#16920=CARTESIAN_POINT('Ctrl Pts',(-55.2927521482605,-106.67732643432,175.988023357328));
#16921=CARTESIAN_POINT('Ctrl Pts',(-55.2927413177775,-106.67723081443,175.986740835906));
#16922=CARTESIAN_POINT('Ctrl Pts',(-55.2927307423378,-106.677137446396,
175.985484942761));
#16923=CARTESIAN_POINT('Ctrl Pts',(-55.2927237094211,-106.677075354453,
175.984649744227));
#16924=CARTESIAN_POINT('Ctrl Pts',(-55.2927167867966,-106.677014236315,
175.983826323883));
#16925=CARTESIAN_POINT('Ctrl Pts',(-55.2927100251261,-106.676954539256,
175.983020844777));
#16926=CARTESIAN_POINT('Ctrl Pts',(-55.292686356663,-106.676745576449,175.980201356218));
#16927=CARTESIAN_POINT('Ctrl Pts',(-55.2926628136723,-106.6765377221,175.977381788001));
#16928=CARTESIAN_POINT('Ctrl Pts',(-55.2926393964027,-106.676330978384,
175.974562133813));
#16929=CARTESIAN_POINT('Ctrl Pts',(-55.292595410732,-106.675942642716,175.969265855355));
#16930=CARTESIAN_POINT('Ctrl Pts',(-55.2925518689223,-106.675558228158,
175.963969309127));
#16931=CARTESIAN_POINT('Ctrl Pts',(-55.2925087726015,-106.675177748937,
175.958672453013));
#16932=CARTESIAN_POINT('Ctrl Pts',(-55.2922679928291,-106.673052005984,
175.929078840673));
#16933=CARTESIAN_POINT('Ctrl Pts',(-55.2920411600593,-106.671049466951,
175.899480614883));
#16934=CARTESIAN_POINT('Ctrl Pts',(-55.2918285395228,-106.669172449607,
175.869869906562));
#16935=CARTESIAN_POINT('Ctrl Pts',(-55.2914493101741,-106.665824607123,
175.817056336345));
#16936=CARTESIAN_POINT('Ctrl Pts',(-55.2911155951723,-106.662878742094,
175.764245125515));
#16937=CARTESIAN_POINT('Ctrl Pts',(-55.2908286328295,-106.6603456714,175.711385142418));
#16938=CARTESIAN_POINT('Ctrl Pts',(-55.2895101725791,-106.648707374234,
175.468517782654));
#16939=CARTESIAN_POINT('Ctrl Pts',(-55.2891999599628,-106.645969953786,
175.228522961519));
#16940=CARTESIAN_POINT('Ctrl Pts',(-55.2899155902426,-106.652286416981,
174.985485069079));
#16941=CARTESIAN_POINT('',(-55.2524742173424,-106.322390962095,176.985485069079));
#16942=CARTESIAN_POINT('Ctrl Pts',(-55.2524742173424,-106.322390962095,
176.985485069079));
#16943=CARTESIAN_POINT('Ctrl Pts',(-55.2706837641386,-106.482554303022,
176.985485069079));
#16944=CARTESIAN_POINT('Ctrl Pts',(-55.288847495167,-106.642723504755,176.985485069079));
#16945=CARTESIAN_POINT('Ctrl Pts',(-55.3069657208749,-106.802898527582,
176.985485069079));
#16946=CARTESIAN_POINT('',(-55.2352859196244,-106.171331405697,174.985485069079));
#16947=CARTESIAN_POINT('Ctrl Pts',(-55.2352859196244,-106.171331405697,
174.985485069079));
#16948=CARTESIAN_POINT('Ctrl Pts',(-55.2401761452878,-106.214274725582,
175.236405579021));
#16949=CARTESIAN_POINT('Ctrl Pts',(-55.2442697085661,-106.250251755796,
175.488576301999));
#16950=CARTESIAN_POINT('Ctrl Pts',(-55.2472018779028,-106.276029153754,
175.742561083287));
#16951=CARTESIAN_POINT('Ctrl Pts',(-55.2480105996487,-106.28313881895,175.812612636308));
#16952=CARTESIAN_POINT('Ctrl Pts',(-55.2487298340075,-106.289462577533,
175.882676256102));
#16953=CARTESIAN_POINT('Ctrl Pts',(-55.2493549857083,-106.294959540506,
175.952876754899));
#16954=CARTESIAN_POINT('Ctrl Pts',(-55.2494130860916,-106.295470417555,
175.959401052735));
#16955=CARTESIAN_POINT('Ctrl Pts',(-55.2494703678393,-106.295974100495,
175.96592585647));
#16956=CARTESIAN_POINT('Ctrl Pts',(-55.2495268279332,-106.29647056244,175.972451281598));
#16957=CARTESIAN_POINT('Ctrl Pts',(-55.2495533179369,-106.296703492954,
175.975512887116));
#16958=CARTESIAN_POINT('Ctrl Pts',(-55.2495796268868,-106.296934832301,
175.978574608341));
#16959=CARTESIAN_POINT('Ctrl Pts',(-55.2496057544813,-106.297164577793,
175.981636457498));
#16960=CARTESIAN_POINT('Ctrl Pts',(-55.2496167657949,-106.297261402614,
175.982926854955));
#16961=CARTESIAN_POINT('Ctrl Pts',(-55.2496277580784,-106.29735806025,175.984218873501));
#16962=CARTESIAN_POINT('Ctrl Pts',(-55.2496384985501,-106.29745250379,175.985484942653));
#16963=CARTESIAN_POINT('Ctrl Pts',(-55.24964765888,-106.297533052764,175.986564747277));
#16964=CARTESIAN_POINT('Ctrl Pts',(-55.2496566402325,-106.297612028052,
175.987625673427));
#16965=CARTESIAN_POINT('Ctrl Pts',(-55.2496653005445,-106.297688180439,
175.988650615149));
#16966=CARTESIAN_POINT('Ctrl Pts',(-55.2496866484448,-106.297875898109,
175.991177123873));
#16967=CARTESIAN_POINT('Ctrl Pts',(-55.2497078947491,-106.29806272298,175.993703697114));
#16968=CARTESIAN_POINT('Ctrl Pts',(-55.2497290392808,-106.298248653482,
175.996230339542));
#16969=CARTESIAN_POINT('Ctrl Pts',(-55.2497625202032,-106.298543061741,
176.000231105349));
#16970=CARTESIAN_POINT('Ctrl Pts',(-55.2497957458191,-106.29883522639,176.004232028344));
#16971=CARTESIAN_POINT('Ctrl Pts',(-55.2498287154289,-106.299125141216,
176.008233126624));
#16972=CARTESIAN_POINT('Ctrl Pts',(-55.249933865528,-106.30004976765,176.020993844248));
#16973=CARTESIAN_POINT('Ctrl Pts',(-55.2500364079953,-106.300951477765,
176.033755904728));
#16974=CARTESIAN_POINT('Ctrl Pts',(-55.2501363208663,-106.301830076432,
176.046519918487));
#16975=CARTESIAN_POINT('Ctrl Pts',(-55.2506462795165,-106.306314473544,
176.111667873496));
#16976=CARTESIAN_POINT('Ctrl Pts',(-55.2510872689855,-106.310192695347,
176.176807217008));
#16977=CARTESIAN_POINT('Ctrl Pts',(-55.2514568274136,-106.313442863289,
176.242030598198));
#16978=CARTESIAN_POINT('Ctrl Pts',(-55.2528664368204,-106.325840002566,
176.490812616604));
#16979=CARTESIAN_POINT('Ctrl Pts',(-55.253212525286,-106.328884801187,176.736501928978));
#16980=CARTESIAN_POINT('Ctrl Pts',(-55.2524742173427,-106.322390962095,
176.985485069079));
#16981=CARTESIAN_POINT('Ctrl Pts',(-55.2899155902424,-106.652286416981,
174.985485069079));
#16982=CARTESIAN_POINT('Ctrl Pts',(-55.2717515343084,-106.491962582169,
174.985485069079));
#16983=CARTESIAN_POINT('Ctrl Pts',(-55.2535417485206,-106.33164423255,174.985485069079));
#16984=CARTESIAN_POINT('Ctrl Pts',(-55.2352859196244,-106.171331405697,
174.985485069079));
#16985=CARTESIAN_POINT('Ctrl Pts',(-55.4744258120625,-108.295058418442,
176.985485069079));
#16986=CARTESIAN_POINT('Ctrl Pts',(-55.4744258120625,-108.295058418442,
174.585485069079));
#16987=CARTESIAN_POINT('Ctrl Pts',(-55.4508297883282,-108.083139316849,
176.985485069079));
#16988=CARTESIAN_POINT('Ctrl Pts',(-55.4508297883282,-108.083139316849,
174.585485069079));
#16989=CARTESIAN_POINT('Ctrl Pts',(-55.4272071161424,-107.871691103985,
176.985485069079));
#16990=CARTESIAN_POINT('Ctrl Pts',(-55.4272071161424,-107.871691103985,
174.585485069079));
#16991=CARTESIAN_POINT('Ctrl Pts',(-55.403557960387,-107.660712297587,176.985485069079));
#16992=CARTESIAN_POINT('Ctrl Pts',(-55.403557960387,-107.660712297587,174.585485069079));
#16993=CARTESIAN_POINT('',(-55.4740061171306,-108.291289156015,176.985485069079));
#16994=CARTESIAN_POINT('',(-55.4571650701271,-108.140163914373,174.985485069079));
#16995=CARTESIAN_POINT('Ctrl Pts',(-55.4740061171306,-108.291289156015,
176.985485069079));
#16996=CARTESIAN_POINT('Ctrl Pts',(-55.4693413328948,-108.24939575857,176.740856007555));
#16997=CARTESIAN_POINT('Ctrl Pts',(-55.4654107951634,-108.214124398444,
176.495008193215));
#16998=CARTESIAN_POINT('Ctrl Pts',(-55.4625532189185,-108.188488942206,
176.247483542904));
#16999=CARTESIAN_POINT('Ctrl Pts',(-55.4618556309792,-108.182230846687,
176.187058134815));
#17000=CARTESIAN_POINT('Ctrl Pts',(-55.461222711051,-108.176553506821,176.126614262712));
#17001=CARTESIAN_POINT('Ctrl Pts',(-55.4606575648579,-108.171484461937,
176.066074873696));
#17002=CARTESIAN_POINT('Ctrl Pts',(-55.4604862720825,-108.169948061662,
176.047725710083));
#17003=CARTESIAN_POINT('Ctrl Pts',(-55.4603212556149,-108.168467993661,
176.029373169598));
#17004=CARTESIAN_POINT('Ctrl Pts',(-55.4601625869058,-108.167044890835,
176.011014750052));
#17005=CARTESIAN_POINT('Ctrl Pts',(-55.4601231175954,-108.166690889801,
176.006448038934));
#17006=CARTESIAN_POINT('Ctrl Pts',(-55.4600840420122,-108.166340422096,
176.001881072887));
#17007=CARTESIAN_POINT('Ctrl Pts',(-55.4600453611864,-108.165993496843,
175.997313812018));
#17008=CARTESIAN_POINT('Ctrl Pts',(-55.4600228395146,-108.165791501758,
175.994654552605));
#17009=CARTESIAN_POINT('Ctrl Pts',(-55.4600004517715,-108.165590708515,
175.991995205391));
#17010=CARTESIAN_POINT('Ctrl Pts',(-55.4599781981548,-108.165391118863,
175.989335762263));
#17011=CARTESIAN_POINT('Ctrl Pts',(-55.4599673907826,-108.165294189017,
175.988044215281));
#17012=CARTESIAN_POINT('Ctrl Pts',(-55.4599566054665,-108.16519745714,175.986751447536));
#17013=CARTESIAN_POINT('Ctrl Pts',(-55.4599460696997,-108.165102963572,
175.985484943119));
#17014=CARTESIAN_POINT('Ctrl Pts',(-55.4599372288567,-108.165023671498,
175.984422185476));
#17015=CARTESIAN_POINT('Ctrl Pts',(-55.459928559729,-108.164945919612,175.98337792344));
#17016=CARTESIAN_POINT('Ctrl Pts',(-55.4599201945696,-108.16487089405,175.982368397651));
#17017=CARTESIAN_POINT('Ctrl Pts',(-55.4598965177436,-108.164658540993,
175.979511026362));
#17018=CARTESIAN_POINT('Ctrl Pts',(-55.4598729681959,-108.164447330186,
175.97665357274));
#17019=CARTESIAN_POINT('Ctrl Pts',(-55.4598495461846,-108.16423726392,175.973796030276));
#17020=CARTESIAN_POINT('Ctrl Pts',(-55.4598046375839,-108.16383448971,175.968317071527));
#17021=CARTESIAN_POINT('Ctrl Pts',(-55.459760198168,-108.163435926071,175.962837825568));
#17022=CARTESIAN_POINT('Ctrl Pts',(-55.4597162297266,-108.163041588893,
175.957358245394));
#17023=CARTESIAN_POINT('Ctrl Pts',(-55.4594468504626,-108.160625622909,
175.923786773984));
#17024=CARTESIAN_POINT('Ctrl Pts',(-55.4591952088867,-108.158368831915,
175.890210139137));
#17025=CARTESIAN_POINT('Ctrl Pts',(-55.4589616862943,-108.156274601051,
175.856616688176));
#17026=CARTESIAN_POINT('Ctrl Pts',(-55.4584694489019,-108.151860215576,
175.785805754904));
#17027=CARTESIAN_POINT('Ctrl Pts',(-55.4580584070155,-108.148174292196,
175.715019325924));
#17028=CARTESIAN_POINT('Ctrl Pts',(-55.4577313114708,-108.145241240388,
175.644129208805));
#17029=CARTESIAN_POINT('Ctrl Pts',(-55.4567150497223,-108.136128464605,
175.423878839963));
#17030=CARTESIAN_POINT('Ctrl Pts',(-55.4565239118472,-108.134414983333,
175.205818800274));
#17031=CARTESIAN_POINT('Ctrl Pts',(-55.4571650701274,-108.140163914373,
174.985485069079));
#17032=CARTESIAN_POINT('',(-55.4209415581549,-107.815922027774,176.985485069079));
#17033=CARTESIAN_POINT('Ctrl Pts',(-55.4209415581549,-107.815922027774,
176.985485069079));
#17034=CARTESIAN_POINT('Ctrl Pts',(-55.4386735345253,-107.974372135515,
176.98548506908));
#17035=CARTESIAN_POINT('Ctrl Pts',(-55.4563616238889,-108.132827857332,
176.985485069079));
#17036=CARTESIAN_POINT('Ctrl Pts',(-55.4740061171306,-108.291289156015,
176.985485069079));
#17037=CARTESIAN_POINT('',(-55.4039785947519,-107.664464934554,174.985485069079));
#17038=CARTESIAN_POINT('Ctrl Pts',(-55.4039785947519,-107.664464934554,
174.985485069079));
#17039=CARTESIAN_POINT('Ctrl Pts',(-55.4062102741904,-107.684374978846,
175.101539197611));
#17040=CARTESIAN_POINT('Ctrl Pts',(-55.4082754872338,-107.702806195974,
175.217934983052));
#17041=CARTESIAN_POINT('Ctrl Pts',(-55.4101352991462,-107.719408241535,
175.334552884646));
#17042=CARTESIAN_POINT('Ctrl Pts',(-55.4125205153015,-107.740700430823,
175.484115806038));
#17043=CARTESIAN_POINT('Ctrl Pts',(-55.414564175716,-107.758950771819,175.633801866954));
#17044=CARTESIAN_POINT('Ctrl Pts',(-55.416202564948,-107.773584610072,175.784244658626));
#17045=CARTESIAN_POINT('Ctrl Pts',(-55.4168189212164,-107.779089808568,
175.840840707876));
#17046=CARTESIAN_POINT('Ctrl Pts',(-55.4173769391772,-107.784074415306,
175.897450319742));
#17047=CARTESIAN_POINT('Ctrl Pts',(-55.4178742983759,-107.788517451289,
175.954141676001));
#17048=CARTESIAN_POINT('Ctrl Pts',(-55.4179283902715,-107.789000667925,
175.960307326366));
#17049=CARTESIAN_POINT('Ctrl Pts',(-55.4179817602064,-107.789477438801,
175.966473433208));
#17050=CARTESIAN_POINT('Ctrl Pts',(-55.4180344056584,-107.789947741094,
175.972640094678));
#17051=CARTESIAN_POINT('Ctrl Pts',(-55.4180599526251,-107.790175962082,
175.975632556317));
#17052=CARTESIAN_POINT('Ctrl Pts',(-55.4180853288254,-107.790402658372,
175.978625129339));
#17053=CARTESIAN_POINT('Ctrl Pts',(-55.4181105339787,-107.790627827424,
175.981617825086));
#17054=CARTESIAN_POINT('Ctrl Pts',(-55.4181214581951,-107.790725418398,
175.982914895397));
#17055=CARTESIAN_POINT('Ctrl Pts',(-55.4181323593493,-107.7908228035,175.98421311939));
#17056=CARTESIAN_POINT('Ctrl Pts',(-55.418143007908,-107.79091793219,175.985484943039));
#17057=CARTESIAN_POINT('Ctrl Pts',(-55.418151919882,-107.790997547135,175.986549355573));
#17058=CARTESIAN_POINT('Ctrl Pts',(-55.4181606589672,-107.791075617683,
175.987595273717));
#17059=CARTESIAN_POINT('Ctrl Pts',(-55.4181690927828,-107.791150961195,
175.988606543706));
#17060=CARTESIAN_POINT('Ctrl Pts',(-55.4181904567345,-107.791341816108,
175.991168222087));
#17061=CARTESIAN_POINT('Ctrl Pts',(-55.4182117176372,-107.791531751011,
175.993729967309));
#17062=CARTESIAN_POINT('Ctrl Pts',(-55.4182328753062,-107.791720764235,
175.996291784023));
#17063=CARTESIAN_POINT('Ctrl Pts',(-55.4182671838519,-107.792027261554,
176.000445937577));
#17064=CARTESIAN_POINT('Ctrl Pts',(-55.4183012207954,-107.79233133399,176.00460026078));
#17065=CARTESIAN_POINT('Ctrl Pts',(-55.4183349853619,-107.792632974547,
176.008754774191));
#17066=CARTESIAN_POINT('Ctrl Pts',(-55.4184496579914,-107.793657418794,
176.022864506013));
#17067=CARTESIAN_POINT('Ctrl Pts',(-55.4185611841,-107.794653769769,176.036975841278));
#17068=CARTESIAN_POINT('Ctrl Pts',(-55.418669534322,-107.79562176245,176.05108961184));
#17069=CARTESIAN_POINT('Ctrl Pts',(-55.4191639155807,-107.800038527192,
176.115488036934));
#17070=CARTESIAN_POINT('Ctrl Pts',(-55.4195917247742,-107.80386084636,176.179878137561));
#17071=CARTESIAN_POINT('Ctrl Pts',(-55.4199506167913,-107.807067548154,
176.244350243025));
#17072=CARTESIAN_POINT('Ctrl Pts',(-55.4213311808138,-107.819402893928,
176.4923576241));
#17073=CARTESIAN_POINT('Ctrl Pts',(-55.4216681944916,-107.822415133979,
176.73728037898));
#17074=CARTESIAN_POINT('Ctrl Pts',(-55.4209415581552,-107.815922027774,
176.985485069079));
#17075=CARTESIAN_POINT('Ctrl Pts',(-55.4571650701271,-108.140163914373,
174.985485069079));
#17076=CARTESIAN_POINT('Ctrl Pts',(-55.4394801322276,-107.981592323594,
174.985485069079));
#17077=CARTESIAN_POINT('Ctrl Pts',(-55.4217514048672,-107.82302598526,174.985485069079));
#17078=CARTESIAN_POINT('Ctrl Pts',(-55.4039785947519,-107.664464934554,
174.985485069079));
#17079=CARTESIAN_POINT('Origin',(-34.9583934096621,-20.6140499623174,178.485485069079));
#17080=CARTESIAN_POINT('Origin',(-57.7717014757184,-101.417541310487,178.485485069245));
#17081=CARTESIAN_POINT('',(-59.4993129890855,-102.014294800821,178.485485069079));
#17082=CARTESIAN_POINT('',(-43.8144614293464,-103.686404765925,178.485485069079));
#17083=CARTESIAN_POINT('',(-59.520560431892,-102.213601660657,178.485485069079));
#17084=CARTESIAN_POINT('',(-59.4993129890855,-102.014294800821,178.485485069079));
#17085=CARTESIAN_POINT('',(-61.0175785779007,-102.443745017979,178.485485069079));
#17086=CARTESIAN_POINT('Ctrl Pts',(-59.5205604318919,-102.213601660657,
178.485485069079));
#17087=CARTESIAN_POINT('Ctrl Pts',(-59.7687516259883,-102.246139247352,
178.485485069079));
#17088=CARTESIAN_POINT('Ctrl Pts',(-60.0238706481734,-102.283503399127,
178.485485066351));
#17089=CARTESIAN_POINT('Ctrl Pts',(-60.5302050703991,-102.361822081727,
178.485485066351));
#17090=CARTESIAN_POINT('Ctrl Pts',(-60.7757064450282,-102.402354839682,
178.485485069079));
#17091=CARTESIAN_POINT('Ctrl Pts',(-61.0175785779007,-102.443745017979,
178.485485069079));
#17092=CARTESIAN_POINT('',(-61.0705815801248,-102.940927762808,178.485485069079));
#17093=CARTESIAN_POINT('Origin',(-57.9307104902227,-102.909089544544,178.485485069245));
#17094=CARTESIAN_POINT('',(-59.6404105637488,-103.337828874669,178.485485069079));
#17095=CARTESIAN_POINT('Ctrl Pts',(-61.0705815801248,-102.940927762808,
178.485485069079));
#17096=CARTESIAN_POINT('Ctrl Pts',(-60.8351971136389,-103.017001355183,
178.485485069079));
#17097=CARTESIAN_POINT('Ctrl Pts',(-60.5932857657281,-103.091252176655,
178.485485069079));
#17098=CARTESIAN_POINT('Ctrl Pts',(-60.1227897812454,-103.223982772266,
178.485485069079));
#17099=CARTESIAN_POINT('Ctrl Pts',(-59.8821065504266,-103.285479946149,
178.485485069079));
#17100=CARTESIAN_POINT('Ctrl Pts',(-59.6404105637488,-103.337828874669,
178.485485069079));
#17101=CARTESIAN_POINT('',(-59.6795694385642,-103.705149895142,178.485485069079));
#17102=CARTESIAN_POINT('',(-59.4993129890855,-102.014294800821,178.485485069079));
#17103=CARTESIAN_POINT('',(-61.176587584573,-103.935293252465,178.485485069079));
#17104=CARTESIAN_POINT('Ctrl Pts',(-59.6795694385642,-103.705149895142,
178.485485069079));
#17105=CARTESIAN_POINT('Ctrl Pts',(-59.9277575258273,-103.737687074535,
178.485485069079));
#17106=CARTESIAN_POINT('Ctrl Pts',(-60.1828829344089,-103.775052140888,
178.485485066351));
#17107=CARTESIAN_POINT('Ctrl Pts',(-60.6892140770712,-103.853370316212,
178.485485066351));
#17108=CARTESIAN_POINT('Ctrl Pts',(-60.9347154517004,-103.893903074168,
178.485485069079));
#17109=CARTESIAN_POINT('Ctrl Pts',(-61.176587584573,-103.935293252465,178.485485069079));
#17110=CARTESIAN_POINT('',(-61.229590586797,-104.432475997293,178.485485069079));
#17111=CARTESIAN_POINT('Origin',(-58.0897195265028,-104.400637777242,178.485485069234));
#17112=CARTESIAN_POINT('',(-59.7994195704211,-104.829377109155,178.485485069079));
#17113=CARTESIAN_POINT('Ctrl Pts',(-61.229590586797,-104.432475997293,178.485485069079));
#17114=CARTESIAN_POINT('Ctrl Pts',(-60.9942061203117,-104.508549589668,
178.485485069079));
#17115=CARTESIAN_POINT('Ctrl Pts',(-60.7522947724005,-104.58280041114,178.485485069079));
#17116=CARTESIAN_POINT('Ctrl Pts',(-60.281801988239,-104.715530103916,178.485485069079));
#17117=CARTESIAN_POINT('Ctrl Pts',(-60.0411123245086,-104.777028880782,
178.485485069079));
#17118=CARTESIAN_POINT('Ctrl Pts',(-59.7994195704211,-104.829377109155,
178.485485069079));
#17119=CARTESIAN_POINT('',(-59.8385784452364,-105.196698129628,178.485485069079));
#17120=CARTESIAN_POINT('',(-59.4993129890855,-102.014294800821,178.485485069079));
#17121=CARTESIAN_POINT('',(-61.3355965912452,-105.42684148695,178.485485069079));
#17122=CARTESIAN_POINT('Ctrl Pts',(-59.8385784452364,-105.196698129628,
178.485485069079));
#17123=CARTESIAN_POINT('Ctrl Pts',(-60.0867665324994,-105.229235309021,
178.485485069079));
#17124=CARTESIAN_POINT('Ctrl Pts',(-60.3418919410807,-105.266600375374,
178.485485066351));
#17125=CARTESIAN_POINT('Ctrl Pts',(-60.8482230837444,-105.344918550698,
178.485485066351));
#17126=CARTESIAN_POINT('Ctrl Pts',(-61.0937244583751,-105.385451308654,
178.485485069079));
#17127=CARTESIAN_POINT('Ctrl Pts',(-61.3355965912452,-105.42684148695,178.485485069079));
#17128=CARTESIAN_POINT('',(-61.3885995934693,-105.924024231779,178.485485069079));
#17129=CARTESIAN_POINT('Origin',(-58.2487285178737,-105.892186012675,178.48548506924));
#17130=CARTESIAN_POINT('',(-59.9584285770933,-106.32092534364,178.485485069079));
#17131=CARTESIAN_POINT('Ctrl Pts',(-61.3885995934693,-105.924024231779,
178.485485069079));
#17132=CARTESIAN_POINT('Ctrl Pts',(-61.1532151269831,-106.000097824154,
178.485485069079));
#17133=CARTESIAN_POINT('Ctrl Pts',(-60.9113037790725,-106.074348645626,
178.485485069079));
#17134=CARTESIAN_POINT('Ctrl Pts',(-60.4408077945892,-106.207079241237,
178.485485069079));
#17135=CARTESIAN_POINT('Ctrl Pts',(-60.2001245637709,-106.268576415121,
178.485485069079));
#17136=CARTESIAN_POINT('Ctrl Pts',(-59.9584285770933,-106.32092534364,178.485485069079));
#17137=CARTESIAN_POINT('',(-59.9975874519086,-106.688246364113,178.485485069079));
#17138=CARTESIAN_POINT('',(-59.4993129890855,-102.014294800821,178.485485069079));
#17139=CARTESIAN_POINT('',(-61.4946055979174,-106.918389721436,178.485485069079));
#17140=CARTESIAN_POINT('Ctrl Pts',(-59.9975874519086,-106.688246364113,
178.485485069079));
#17141=CARTESIAN_POINT('Ctrl Pts',(-60.2457755391717,-106.720783543507,
178.485485069079));
#17142=CARTESIAN_POINT('Ctrl Pts',(-60.5009009477533,-106.758148609859,
178.485485066351));
#17143=CARTESIAN_POINT('Ctrl Pts',(-61.0072320904167,-106.836466785184,
178.485485066351));
#17144=CARTESIAN_POINT('Ctrl Pts',(-61.2527334650479,-106.876999543139,
178.485485069079));
#17145=CARTESIAN_POINT('Ctrl Pts',(-61.4946055979174,-106.918389721436,
178.485485069079));
#17146=CARTESIAN_POINT('',(-61.5476086001415,-107.415572466264,178.485485069079));
#17147=CARTESIAN_POINT('Origin',(-58.4077375311275,-107.383734246593,178.485485069251));
#17148=CARTESIAN_POINT('',(-60.1174375837655,-107.812473578126,178.485485069079));
#17149=CARTESIAN_POINT('Ctrl Pts',(-61.5476086001415,-107.415572466264,
178.485485069079));
#17150=CARTESIAN_POINT('Ctrl Pts',(-61.3122241336564,-107.49164605864,178.485485069079));
#17151=CARTESIAN_POINT('Ctrl Pts',(-61.0703127857451,-107.565896880111,
178.485485069079));
#17152=CARTESIAN_POINT('Ctrl Pts',(-60.5998168012618,-107.698627475723,
178.485485069079));
#17153=CARTESIAN_POINT('Ctrl Pts',(-60.3591335704432,-107.760124649606,
178.485485069079));
#17154=CARTESIAN_POINT('Ctrl Pts',(-60.1174375837655,-107.812473578126,
178.485485069079));
#17155=CARTESIAN_POINT('',(-60.1565964585809,-108.179794598599,178.485485069079));
#17156=CARTESIAN_POINT('',(-59.4993129890855,-102.014294800821,178.485485069079));
#17157=CARTESIAN_POINT('',(-61.6536146045896,-108.409937955921,178.485485069079));
#17158=CARTESIAN_POINT('Ctrl Pts',(-60.1565964585809,-108.179794598599,
178.485485069079));
#17159=CARTESIAN_POINT('Ctrl Pts',(-60.4047845458449,-108.212331777992,
178.485485069079));
#17160=CARTESIAN_POINT('Ctrl Pts',(-60.6599099544291,-108.249696844346,
178.485485066351));
#17161=CARTESIAN_POINT('Ctrl Pts',(-61.1662410970868,-108.328015019669,
178.485485066351));
#17162=CARTESIAN_POINT('Ctrl Pts',(-61.4117424717138,-108.368547777624,
178.485485069079));
#17163=CARTESIAN_POINT('Ctrl Pts',(-61.6536146045896,-108.409937955921,
178.485485069079));
#17164=CARTESIAN_POINT('',(-61.7066176068137,-108.90712070075,178.485485069079));
#17165=CARTESIAN_POINT('Origin',(-58.5667465453977,-108.875282480713,178.485485069256));
#17166=CARTESIAN_POINT('',(-60.2764465904377,-109.304021812611,178.485485069079));
#17167=CARTESIAN_POINT('Ctrl Pts',(-61.7066176068137,-108.90712070075,178.485485069079));
#17168=CARTESIAN_POINT('Ctrl Pts',(-61.4712331403281,-108.983194293125,
178.485485069079));
#17169=CARTESIAN_POINT('Ctrl Pts',(-61.2293217924171,-109.057445114597,
178.485485069079));
#17170=CARTESIAN_POINT('Ctrl Pts',(-60.7588258079339,-109.190175710208,
178.485485069079));
#17171=CARTESIAN_POINT('Ctrl Pts',(-60.5181425771154,-109.251672884092,
178.485485069079));
#17172=CARTESIAN_POINT('Ctrl Pts',(-60.2764465904377,-109.304021812611,
178.485485069079));
#17173=CARTESIAN_POINT('',(-60.3156054652531,-109.671342833085,178.485485069079));
#17174=CARTESIAN_POINT('',(-59.4993129890855,-102.014294800821,178.485485069079));
#17175=CARTESIAN_POINT('',(-61.8126236112619,-109.901486190407,178.485485069079));
#17176=CARTESIAN_POINT('Ctrl Pts',(-60.3156054652531,-109.671342833085,
178.485485069079));
#17177=CARTESIAN_POINT('Ctrl Pts',(-60.5637966593489,-109.70388041978,178.485485069079));
#17178=CARTESIAN_POINT('Ctrl Pts',(-60.8189156815327,-109.741244571555,
178.485485066351));
#17179=CARTESIAN_POINT('Ctrl Pts',(-61.3252501037601,-109.819563254155,
178.485485066351));
#17180=CARTESIAN_POINT('Ctrl Pts',(-61.5707514783893,-109.86009601211,178.485485069079));
#17181=CARTESIAN_POINT('Ctrl Pts',(-61.8126236112619,-109.901486190407,
178.485485069079));
#17182=CARTESIAN_POINT('',(-61.865626613486,-110.398668935236,178.485485069079));
#17183=CARTESIAN_POINT('Origin',(-58.7257555470878,-110.366830715451,178.485485069251));
#17184=CARTESIAN_POINT('',(-60.43545559711,-110.795570047097,178.485485069079));
#17185=CARTESIAN_POINT('Ctrl Pts',(-61.8656266134859,-110.398668935236,
178.485485069079));
#17186=CARTESIAN_POINT('Ctrl Pts',(-61.6302421469988,-110.474742527611,
178.485485069079));
#17187=CARTESIAN_POINT('Ctrl Pts',(-61.3883307990888,-110.548993349083,
178.485485069079));
#17188=CARTESIAN_POINT('Ctrl Pts',(-60.9178380149293,-110.681723041858,
178.485485069079));
#17189=CARTESIAN_POINT('Ctrl Pts',(-60.677148351198,-110.743221818724,178.485485069079));
#17190=CARTESIAN_POINT('Ctrl Pts',(-60.43545559711,-110.795570047097,178.485485069079));
#17191=CARTESIAN_POINT('',(-60.4746144719253,-111.16289106757,178.485485069079));
#17192=CARTESIAN_POINT('',(-59.4993129890855,-102.014294800821,178.485485069079));
#17193=CARTESIAN_POINT('',(-61.9716326179341,-111.393034424893,178.485485069079));
#17194=CARTESIAN_POINT('Ctrl Pts',(-60.4746144719253,-111.16289106757,178.485485069079));
#17195=CARTESIAN_POINT('Ctrl Pts',(-60.7228025591888,-111.195428246963,
178.485485069079));
#17196=CARTESIAN_POINT('Ctrl Pts',(-60.9779279677714,-111.232793313316,
178.485485066351));
#17197=CARTESIAN_POINT('Ctrl Pts',(-61.4842591104322,-111.31111148864,178.485485066351));
#17198=CARTESIAN_POINT('Ctrl Pts',(-61.7297604850611,-111.351644246595,
178.485485069079));
#17199=CARTESIAN_POINT('Ctrl Pts',(-61.9716326179341,-111.393034424893,
178.485485069079));
#17200=CARTESIAN_POINT('',(-62.0210982548538,-111.802120023171,178.485485069079));
#17201=CARTESIAN_POINT('Ctrl Pts',(-61.9716326179341,-111.393034424893,
178.485485069079));
#17202=CARTESIAN_POINT('Ctrl Pts',(-61.9843448484125,-111.460582087639,
178.485485069079));
#17203=CARTESIAN_POINT('Ctrl Pts',(-61.9948456687939,-111.528527230646,
178.485485069079));
#17204=CARTESIAN_POINT('Ctrl Pts',(-62.0113588747397,-111.665001931148,
178.485485069079));
#17205=CARTESIAN_POINT('Ctrl Pts',(-62.017365779563,-111.733484789515,178.485485069079));
#17206=CARTESIAN_POINT('Ctrl Pts',(-62.0210982548537,-111.802120023171,
178.485485069079));
#17207=CARTESIAN_POINT('',(-62.88786637536,-111.709716750739,178.485485069079));
#17208=CARTESIAN_POINT('',(-53.4413942236179,-112.716773792997,178.485485069079));
#17209=CARTESIAN_POINT('',(-52.5853897920404,-15.069651635714,178.485485069079));
#17210=CARTESIAN_POINT('',(-52.9717383111942,-18.6937070505612,178.485485069079));
#17211=CARTESIAN_POINT('',(-52.5342226896633,-12.3683081541722,178.485485069079));
#17212=CARTESIAN_POINT('Origin',(-67.998054881725,-13.4265585667677,178.485485069079));
#17213=CARTESIAN_POINT('',(-53.9352248596064,8.10403203946808,178.485485069079));
#17214=CARTESIAN_POINT('',(-51.890637311636,-21.772789521366,178.485485069079));
#17215=CARTESIAN_POINT('Origin',(-39.4690592605811,9.0940082318961,178.485485069079));
#17216=CARTESIAN_POINT('',(-25.2666963042872,20.9635176568304,178.485485069079));
#17217=CARTESIAN_POINT('',(-69.5889371886705,15.3762068992854,178.485485069079));
#17218=CARTESIAN_POINT('Ctrl Pts',(-50.7024802268255,-64.597022606232,178.485485069074));
#17219=CARTESIAN_POINT('Ctrl Pts',(-49.9577225357214,-60.5851660064401,
178.485485068971));
#17220=CARTESIAN_POINT('Ctrl Pts',(-49.1559388135441,-56.5870189509198,
178.485485067596));
#17221=CARTESIAN_POINT('Ctrl Pts',(-48.2824671906219,-52.6061072831419,
178.485485067469));
#17222=CARTESIAN_POINT('Ctrl Pts',(-47.5647200183799,-49.3349213424548,
178.485485067364));
#17223=CARTESIAN_POINT('Ctrl Pts',(-46.7984850518727,-46.0753929559384,
178.485485068149));
#17224=CARTESIAN_POINT('Ctrl Pts',(-45.9735869873742,-42.8299680258058,
178.485485068747));
#17225=CARTESIAN_POINT('Ctrl Pts',(-45.7314921849895,-41.8774860878194,
178.485485068923));
#17226=CARTESIAN_POINT('Ctrl Pts',(-45.4843412719279,-40.9262208647867,
178.485485068989));
#17227=CARTESIAN_POINT('Ctrl Pts',(-45.2318774001476,-39.9762334548118,
178.485485069027));
#17228=CARTESIAN_POINT('Ctrl Pts',(-44.5307934654103,-37.3381494127691,
178.485485069132));
#17229=CARTESIAN_POINT('Ctrl Pts',(-43.7882434129997,-34.7100383998247,
178.485485069079));
#17230=CARTESIAN_POINT('Ctrl Pts',(-42.9998272938232,-32.0929433338551,
178.485485069079));
#17231=CARTESIAN_POINT('Ctrl Pts',(-42.536945026492,-30.556436318724,178.485485069079));
#17232=CARTESIAN_POINT('Ctrl Pts',(-42.0582539070797,-29.0237291849288,
178.48548506908));
#17233=CARTESIAN_POINT('Ctrl Pts',(-41.562861354517,-27.4950373025228,178.485485069079));
#17234=CARTESIAN_POINT('Ctrl Pts',(-40.910610725801,-25.4823097468615,178.485485069079));
#17235=CARTESIAN_POINT('Ctrl Pts',(-40.2295198019946,-23.4765157852253,
178.485485069084));
#17236=CARTESIAN_POINT('Ctrl Pts',(-39.5206447744511,-21.477403436665,178.485485069048));
#17237=CARTESIAN_POINT('Ctrl Pts',(-39.5017999516025,-21.4242587826721,
178.485485069047));
#17238=CARTESIAN_POINT('Ctrl Pts',(-39.4829354217113,-21.3711185893304,
178.485485069046));
#17239=CARTESIAN_POINT('Ctrl Pts',(-39.4640512098165,-21.3179828737293,
178.485485069046));
#17240=CARTESIAN_POINT('Ctrl Pts',(-38.8579946469832,-19.6126827351552,
178.485485069021));
#17241=CARTESIAN_POINT('Ctrl Pts',(-38.2315032054965,-17.9121204812206,
178.485485069452));
#17242=CARTESIAN_POINT('Ctrl Pts',(-37.5896039498787,-16.2180717563625,
178.485485068683));
#17243=CARTESIAN_POINT('Ctrl Pts',(-37.4591313137947,-15.8737389021763,
178.485485068526));
#17244=CARTESIAN_POINT('Ctrl Pts',(-37.3280157001481,-15.5296410006451,
178.485485068432));
#17245=CARTESIAN_POINT('Ctrl Pts',(-37.1962973022816,-15.1857911182026,
178.48548506842));
#17246=CARTESIAN_POINT('Ctrl Pts',(-36.6597955345752,-13.7852573071025,
178.485485068374));
#17247=CARTESIAN_POINT('Ctrl Pts',(-36.1130279995534,-12.3883503107043,
178.485485069405));
#17248=CARTESIAN_POINT('Ctrl Pts',(-35.5610537102179,-10.9934715504989,
178.485485068543));
#17249=CARTESIAN_POINT('Ctrl Pts',(-35.3107978101541,-10.3610568776427,
178.485485068152));
#17250=CARTESIAN_POINT('Ctrl Pts',(-35.0594847877249,-9.72903448704139,
178.485485067774));
#17251=CARTESIAN_POINT('Ctrl Pts',(-34.807584751089,-9.09722990883248,178.485485067609));
#17252=CARTESIAN_POINT('Ctrl Pts',(-34.0000823368259,-7.07188791579596,
178.485485067081));
#17253=CARTESIAN_POINT('Ctrl Pts',(-33.1867503081442,-5.04870903840101,
178.485485068358));
#17254=CARTESIAN_POINT('Ctrl Pts',(-32.3920015482318,-3.01863635839204,
178.485485068222));
#17255=CARTESIAN_POINT('Ctrl Pts',(-32.0725147428821,-2.20255275074324,
178.485485068167));
#17256=CARTESIAN_POINT('Ctrl Pts',(-31.7561578556963,-1.38530802264268,
178.485485068002));
#17257=CARTESIAN_POINT('Ctrl Pts',(-31.4446039158297,-0.566281120802405,
178.48548506705));
#17258=CARTESIAN_POINT('Ctrl Pts',(-30.9811424894089,0.652086961355245,
178.485485065634));
#17259=CARTESIAN_POINT('Ctrl Pts',(-30.5284028502065,1.87443509955828,178.485485068243));
#17260=CARTESIAN_POINT('Ctrl Pts',(-30.0917686168577,3.10275613520199,178.485485066804));
#17261=CARTESIAN_POINT('Ctrl Pts',(-29.9026804336469,3.63469104843164,178.485485066181));
#17262=CARTESIAN_POINT('Ctrl Pts',(-29.7166555662945,4.16776221500052,178.485485065225));
#17263=CARTESIAN_POINT('Ctrl Pts',(-29.5339497743812,4.70206521212496,178.485485059336));
#17264=CARTESIAN_POINT('Ctrl Pts',(-29.1679324450908,5.77244264237208,178.48548504754));
#17265=CARTESIAN_POINT('Ctrl Pts',(-28.8155745074676,6.8476686892158,178.485485059056));
#17266=CARTESIAN_POINT('Ctrl Pts',(-28.478719177052,7.92885248014735,178.485485064871));
#17267=CARTESIAN_POINT('Ctrl Pts',(-28.3344155971724,8.39201478589668,178.485485067362));
#17268=CARTESIAN_POINT('Ctrl Pts',(-28.1929573735739,8.85627083216291,178.485485068419));
#17269=CARTESIAN_POINT('Ctrl Pts',(-28.0544916023756,9.32170993752464,178.485485068745));
#17270=CARTESIAN_POINT('Ctrl Pts',(-27.9822645276947,9.56449416305175,178.485485068915));
#17271=CARTESIAN_POINT('Ctrl Pts',(-27.9108481850166,9.80757191347016,178.485485068948));
#17272=CARTESIAN_POINT('Ctrl Pts',(-27.8402559064099,10.0509078082713,178.485485068899));
#17273=CARTESIAN_POINT('Ctrl Pts',(-27.6065126969891,10.8566349237679,178.485485068738));
#17274=CARTESIAN_POINT('Ctrl Pts',(-27.3819521686276,11.6649845310262,178.485485068755));
#17275=CARTESIAN_POINT('Ctrl Pts',(-27.1671077612216,12.4747398429342,178.485485068853));
#17276=CARTESIAN_POINT('Ctrl Pts',(-26.9023082251874,13.4727776019026,178.485485068974));
#17277=CARTESIAN_POINT('Ctrl Pts',(-26.6520104417681,14.4737369620719,178.485485069067));
#17278=CARTESIAN_POINT('Ctrl Pts',(-26.4157730331659,15.4779537724868,178.485485069074));
#17279=CARTESIAN_POINT('Ctrl Pts',(-26.4026358124523,15.5337985176555,178.485485069074));
#17280=CARTESIAN_POINT('Ctrl Pts',(-26.389542235729,15.5896525401592,178.485485069074));
#17281=CARTESIAN_POINT('Ctrl Pts',(-26.3764922522572,15.6455158264978,178.485485069074));
#17282=CARTESIAN_POINT('Ctrl Pts',(-26.0090755642338,17.2183226957897,178.485485069074));
#17283=CARTESIAN_POINT('Ctrl Pts',(-25.6763240448109,18.7984939236132,178.485485068312));
#17284=CARTESIAN_POINT('Ctrl Pts',(-25.3750312441927,20.3853496797055,178.485485068784));
#17285=CARTESIAN_POINT('Ctrl Pts',(-25.3384580343882,20.5779742906419,178.485485068841));
#17286=CARTESIAN_POINT('Ctrl Pts',(-25.3023483140838,20.7706973640245,178.485485068913));
#17287=CARTESIAN_POINT('Ctrl Pts',(-25.2666963042872,20.9635176568304,178.485485068975));
#17288=CARTESIAN_POINT('',(-37.4541011624573,-44.0244753865006,178.485485069079));
#17289=CARTESIAN_POINT('Origin',(-57.4536834643351,-98.4344448420243,178.485485069234));
#17290=CARTESIAN_POINT('Origin',(-57.6126924821839,-99.925993075306,178.485485069234));
#17291=CARTESIAN_POINT('Ctrl Pts',(-56.3380022369383,-103.524730528528,
173.488899497191));
#17292=CARTESIAN_POINT('Ctrl Pts',(-54.948621273746,-103.687204108539,173.583445126328));
#17293=CARTESIAN_POINT('Ctrl Pts',(-54.9486212737461,-103.687204108539,
174.985485069079));
#17294=CARTESIAN_POINT('Ctrl Pts',(-56.3134791922014,-103.315023500967,
173.488899497191));
#17295=CARTESIAN_POINT('Ctrl Pts',(-54.9241403737337,-103.47785747851,173.583445126328));
#17296=CARTESIAN_POINT('Ctrl Pts',(-54.92414037373,-103.477857478511,174.985485069079));
#17297=CARTESIAN_POINT('Ctrl Pts',(-56.2888745073538,-103.105325623786,
173.488899497188));
#17298=CARTESIAN_POINT('Ctrl Pts',(-54.8995781655658,-103.268521622085,
173.583445126281));
#17299=CARTESIAN_POINT('Ctrl Pts',(-54.899578165568,-103.268521622085,174.985485069033));
#17300=CARTESIAN_POINT('Ctrl Pts',(-56.264187433819,-102.895636981445,173.488899497191));
#17301=CARTESIAN_POINT('Ctrl Pts',(-54.8749339071881,-103.059196645868,
173.583445126328));
#17302=CARTESIAN_POINT('Ctrl Pts',(-54.8749339071881,-103.059196645868,
174.985485069079));
#17303=CARTESIAN_POINT('Ctrl Pts',(-56.2951298069877,-103.31239211438,173.490216228525));
#17304=CARTESIAN_POINT('Ctrl Pts',(-56.1168599625939,-103.372824172232,
173.50487235569));
#17305=CARTESIAN_POINT('Ctrl Pts',(-55.9412469787364,-103.427519480035,
173.553480952136));
#17306=CARTESIAN_POINT('Ctrl Pts',(-55.6154923586755,-103.522549593778,
173.714958502574));
#17307=CARTESIAN_POINT('Ctrl Pts',(-55.4681253804373,-103.562403698112,
173.825864100261));
#17308=CARTESIAN_POINT('Ctrl Pts',(-55.3115517495563,-103.602970854155,
173.997534195604));
#17309=CARTESIAN_POINT('Ctrl Pts',(-55.280814671631,-103.610801558914,174.03468048597));
#17310=CARTESIAN_POINT('Ctrl Pts',(-55.2394521645914,-103.621161449704,
174.089882029675));
#17311=CARTESIAN_POINT('Ctrl Pts',(-55.227372087514,-103.624162767105,174.106716353987));
#17312=CARTESIAN_POINT('Ctrl Pts',(-55.2045892632002,-103.629776810059,
174.139889226158));
#17313=CARTESIAN_POINT('Ctrl Pts',(-55.1938496699846,-103.632401432436,
174.156194945232));
#17314=CARTESIAN_POINT('Ctrl Pts',(-55.1053185916828,-103.653854269162,
174.296454686301));
#17315=CARTESIAN_POINT('Ctrl Pts',(-55.0452533006265,-103.667183335149,
174.431403235506));
#17316=CARTESIAN_POINT('Ctrl Pts',(-54.9675549889356,-103.681744085934,
174.707304465526));
#17317=CARTESIAN_POINT('Ctrl Pts',(-54.9481904031526,-103.683519554,174.846067667605));
#17318=CARTESIAN_POINT('Ctrl Pts',(-54.947771193524,-103.67993499333,174.985485069079));
#17319=CARTESIAN_POINT('Ctrl Pts',(-54.8895810276955,-103.183690695995,
174.985485069059));
#17320=CARTESIAN_POINT('Ctrl Pts',(-54.8869443160962,-103.161264788318,
174.853511827955));
#17321=CARTESIAN_POINT('Ctrl Pts',(-54.9019593409972,-103.139808319536,
174.72165986107));
#17322=CARTESIAN_POINT('Ctrl Pts',(-54.9711980898845,-103.096417623673,
174.448996361516));
#17323=CARTESIAN_POINT('Ctrl Pts',(-55.0297082307631,-103.075025668701,
174.310839512231));
#17324=CARTESIAN_POINT('Ctrl Pts',(-55.113651797122,-103.054157978782,174.175160756358));
#17325=CARTESIAN_POINT('Ctrl Pts',(-55.119038710508,-103.052849999777,174.166651653447));
#17326=CARTESIAN_POINT('Ctrl Pts',(-55.1301879436357,-103.050205117004,
174.149436885413));
#17327=CARTESIAN_POINT('Ctrl Pts',(-55.1359564487483,-103.048868971353,
174.140735847771));
#17328=CARTESIAN_POINT('Ctrl Pts',(-55.1544049602056,-103.044695439842,
174.113545908635));
#17329=CARTESIAN_POINT('Ctrl Pts',(-55.1674198033572,-103.041894792854,
174.095282862691));
#17330=CARTESIAN_POINT('Ctrl Pts',(-55.20909085459,-103.033355805697,174.039567190658));
#17331=CARTESIAN_POINT('Ctrl Pts',(-55.2391523612539,-103.027786444963,
174.003181423291));
#17332=CARTESIAN_POINT('Ctrl Pts',(-55.3993921228637,-103.000861959833,
173.827296202087));
#17333=CARTESIAN_POINT('Ctrl Pts',(-55.5542442720682,-102.983503643399,
173.712645716775));
#17334=CARTESIAN_POINT('Ctrl Pts',(-55.8932478530683,-102.957689459523,
173.551401697661));
#17335=CARTESIAN_POINT('Ctrl Pts',(-56.0726931839364,-102.948924353571,
173.503884287599));
#17336=CARTESIAN_POINT('Ctrl Pts',(-56.2564866337797,-102.944965370977,
173.489866571436));
#17337=CARTESIAN_POINT('Ctrl Pts',(-56.4935439071687,-105.015012404135,
173.4901641777));
#17338=CARTESIAN_POINT('Ctrl Pts',(-55.1209916136374,-105.172984763673,
173.59954855975));
#17339=CARTESIAN_POINT('Ctrl Pts',(-55.1209916136374,-105.172984763673,
174.985485069079));
#17340=CARTESIAN_POINT('Ctrl Pts',(-56.469641633236,-104.80733606751,173.490164177706));
#17341=CARTESIAN_POINT('Ctrl Pts',(-55.0971290533058,-104.965653481046,
173.599548559819));
#17342=CARTESIAN_POINT('Ctrl Pts',(-55.0971290532985,-104.965653481047,
174.985485069149));
#17343=CARTESIAN_POINT('Ctrl Pts',(-56.4456610218866,-104.599668529283,
173.4901641777));
#17344=CARTESIAN_POINT('Ctrl Pts',(-55.0731884626156,-104.758332519263,
173.59954855975));
#17345=CARTESIAN_POINT('Ctrl Pts',(-55.0731884626167,-104.758332519263,
174.985485069079));
#17346=CARTESIAN_POINT('Ctrl Pts',(-56.4216013700109,-104.392009869032,
173.4901641777));
#17347=CARTESIAN_POINT('Ctrl Pts',(-55.0491691443755,-104.551021978299,
173.59954855975));
#17348=CARTESIAN_POINT('Ctrl Pts',(-55.0491691443755,-104.551021978299,
174.985485069079));
#17349=CARTESIAN_POINT('Ctrl Pts',(-56.4520785736132,-104.804362764877,
173.491614708057));
#17350=CARTESIAN_POINT('Ctrl Pts',(-56.2764801204879,-104.863475756594,
173.508047709852));
#17351=CARTESIAN_POINT('Ctrl Pts',(-56.1038031321053,-104.916970336167,
173.557406804494));
#17352=CARTESIAN_POINT('Ctrl Pts',(-55.7811932477556,-105.010655798977,
173.719527388766));
#17353=CARTESIAN_POINT('Ctrl Pts',(-55.6343676897392,-105.050165862524,
173.831270860266));
#17354=CARTESIAN_POINT('Ctrl Pts',(-55.4786717532136,-105.090295312868,
174.003823442269));
#17355=CARTESIAN_POINT('Ctrl Pts',(-55.4481316679127,-105.098033854321,
174.041134856339));
#17356=CARTESIAN_POINT('Ctrl Pts',(-55.4071614184955,-105.108237599683,
174.09642283915));
#17357=CARTESIAN_POINT('Ctrl Pts',(-55.3952646257317,-105.111176528091,
174.113183051674));
#17358=CARTESIAN_POINT('Ctrl Pts',(-55.3782751432832,-105.115338825496,
174.138185978057));
#17359=CARTESIAN_POINT('Ctrl Pts',(-55.372919462571,-105.116645561674,174.146232885148));
#17360=CARTESIAN_POINT('Ctrl Pts',(-55.3625173756426,-105.119173055363,
174.162192113799));
#17361=CARTESIAN_POINT('Ctrl Pts',(-55.3574667590035,-105.120395154211,
174.170100905845));
#17362=CARTESIAN_POINT('Ctrl Pts',(-55.2754517253537,-105.140156652778,
174.301203481707));
#17363=CARTESIAN_POINT('Ctrl Pts',(-55.2162337104791,-105.153210404953,
174.435317540761));
#17364=CARTESIAN_POINT('Ctrl Pts',(-55.1396340081755,-105.167422578865,
174.709330975967));
#17365=CARTESIAN_POINT('Ctrl Pts',(-55.1205462794532,-105.169115462503,
174.847088380847));
#17366=CARTESIAN_POINT('Ctrl Pts',(-55.120134291992,-105.165536169417,174.985485069079));
#17367=CARTESIAN_POINT('Ctrl Pts',(-55.0638414339194,-104.677744265774,
174.985485069076));
#17368=CARTESIAN_POINT('Ctrl Pts',(-55.0612613713556,-104.655445553952,
174.854777352187));
#17369=CARTESIAN_POINT('Ctrl Pts',(-55.0759893823669,-104.634087195595,
174.724186106669));
#17370=CARTESIAN_POINT('Ctrl Pts',(-55.1438583050946,-104.590861516158,
174.454137517071));
#17371=CARTESIAN_POINT('Ctrl Pts',(-55.2011654935698,-104.569517652801,
174.317239125928));
#17372=CARTESIAN_POINT('Ctrl Pts',(-55.2889921927481,-104.547221220573,
174.173406546999));
#17373=CARTESIAN_POINT('Ctrl Pts',(-55.3001327143269,-104.544525990686,
174.156002076534));
#17374=CARTESIAN_POINT('Ctrl Pts',(-55.3240161880476,-104.539012928576,
174.120376941088));
#17375=CARTESIAN_POINT('Ctrl Pts',(-55.3368133160102,-104.536201898492,
174.102198371918));
#17376=CARTESIAN_POINT('Ctrl Pts',(-55.3780335382476,-104.527575963677,
174.046393296067));
#17377=CARTESIAN_POINT('Ctrl Pts',(-55.4078751234595,-104.521929130967,
174.009829877401));
#17378=CARTESIAN_POINT('Ctrl Pts',(-55.5673673802023,-104.494548164989,
173.832642158232));
#17379=CARTESIAN_POINT('Ctrl Pts',(-55.7219729516093,-104.476807485154,
173.716842686832));
#17380=CARTESIAN_POINT('Ctrl Pts',(-56.0575151920358,-104.450461151493,
173.555187437059));
#17381=CARTESIAN_POINT('Ctrl Pts',(-56.2331920134854,-104.441405509746,
173.507099973385));
#17382=CARTESIAN_POINT('Ctrl Pts',(-56.4134173387406,-104.436939704692,
173.491276679516));
#17383=CARTESIAN_POINT('Ctrl Pts',(-56.6493388241048,-106.505953769142,
173.491370349032));
#17384=CARTESIAN_POINT('Ctrl Pts',(-55.2907737759503,-106.659861440633,
173.612844366516));
#17385=CARTESIAN_POINT('Ctrl Pts',(-55.2907737759503,-106.659861440633,
174.985485069079));
#17386=CARTESIAN_POINT('Ctrl Pts',(-56.6259915569457,-106.299864099721,
173.491370349032));
#17387=CARTESIAN_POINT('Ctrl Pts',(-55.2674640931904,-106.45410353412,173.612844366521));
#17388=CARTESIAN_POINT('Ctrl Pts',(-55.2674640931895,-106.45410353412,174.985485069085));
#17389=CARTESIAN_POINT('Ctrl Pts',(-56.6025687929303,-106.093782923719,
173.491370349031));
#17390=CARTESIAN_POINT('Ctrl Pts',(-55.2440791994502,-106.248355558005,
173.612844366504));
#17391=CARTESIAN_POINT('Ctrl Pts',(-55.2440791994508,-106.248355558005,
174.985485069068));
#17392=CARTESIAN_POINT('Ctrl Pts',(-56.5790698673243,-105.887710316561,
173.491370349032));
#17393=CARTESIAN_POINT('Ctrl Pts',(-55.2206184354041,-106.042617606657,
173.612844366516));
#17394=CARTESIAN_POINT('Ctrl Pts',(-55.2206184354041,-106.042617606657,
174.985485069079));
#17395=CARTESIAN_POINT('Ctrl Pts',(-56.6091901843102,-106.296300098481,
173.492904904255));
#17396=CARTESIAN_POINT('Ctrl Pts',(-56.4357941643567,-106.354338595723,
173.51075904954));
#17397=CARTESIAN_POINT('Ctrl Pts',(-56.2655234196491,-106.406856990053,
173.560705363963));
#17398=CARTESIAN_POINT('Ctrl Pts',(-55.9455020907631,-106.499444323095,
173.723336101202));
#17399=CARTESIAN_POINT('Ctrl Pts',(-55.7991335388886,-106.53867147263,173.835759261937));
#17400=CARTESIAN_POINT('Ctrl Pts',(-55.644167499606,-106.578442369452,174.009024429013));
#17401=CARTESIAN_POINT('Ctrl Pts',(-55.6137891424861,-106.586105902736,
174.046471025385));
#17402=CARTESIAN_POINT('Ctrl Pts',(-55.5731417121054,-106.596182375197,
174.101826271024));
#17403=CARTESIAN_POINT('Ctrl Pts',(-55.5613960509843,-106.599070390997,
174.118522266282));
#17404=CARTESIAN_POINT('Ctrl Pts',(-55.5392487175406,-106.604470601648,
174.151403158858));
#17405=CARTESIAN_POINT('Ctrl Pts',(-55.5288108760151,-106.606994376912,
174.167556555571));
#17406=CARTESIAN_POINT('Ctrl Pts',(-55.4428037340027,-106.627610764056,
174.306403152543));
#17407=CARTESIAN_POINT('Ctrl Pts',(-55.3845082378286,-106.640382663779,
174.4396024977));
#17408=CARTESIAN_POINT('Ctrl Pts',(-55.3091058140703,-106.654241989031,
174.711549171121));
#17409=CARTESIAN_POINT('Ctrl Pts',(-55.2903198129642,-106.655854262022,
174.848205469326));
#17410=CARTESIAN_POINT('Ctrl Pts',(-55.2899155902427,-106.652286416981,
174.985485069079));
#17411=CARTESIAN_POINT('Ctrl Pts',(-55.2352859196864,-106.171331405706,
174.985485069073));
#17412=CARTESIAN_POINT('Ctrl Pts',(-55.2326665336894,-106.148329373114,
174.851082750799));
#17413=CARTESIAN_POINT('Ctrl Pts',(-55.2483413321261,-106.126315491714,
174.716825828879));
#17414=CARTESIAN_POINT('Ctrl Pts',(-55.3203356455073,-106.081767707275,
174.439384706467));
#17415=CARTESIAN_POINT('Ctrl Pts',(-55.3811169315066,-106.059800227937,
174.299008553436));
#17416=CARTESIAN_POINT('Ctrl Pts',(-55.4681846194273,-106.038387952022,
174.161638426905));
#17417=CARTESIAN_POINT('Ctrl Pts',(-55.4737726492823,-106.037045675612,
174.153023925989));
#17418=CARTESIAN_POINT('Ctrl Pts',(-55.4916498327172,-106.032850156698,
174.126090196313));
#17419=CARTESIAN_POINT('Ctrl Pts',(-55.5042652787232,-106.03003179675,174.107986160937));
#17420=CARTESIAN_POINT('Ctrl Pts',(-55.5451114880963,-106.021335274986,
174.052109135738));
#17421=CARTESIAN_POINT('Ctrl Pts',(-55.5747719738423,-106.015624438621,
174.015396204934));
#17422=CARTESIAN_POINT('Ctrl Pts',(-55.7336532714159,-105.987864066763,
173.837109101904));
#17423=CARTESIAN_POINT('Ctrl Pts',(-55.888067370271,-105.969805160622,173.720342048198));
#17424=CARTESIAN_POINT('Ctrl Pts',(-56.2207366814301,-105.943032892182,
173.558379859302));
#17425=CARTESIAN_POINT('Ctrl Pts',(-56.3932583175807,-105.933753654971,
173.50986981577));
#17426=CARTESIAN_POINT('Ctrl Pts',(-56.5704762085009,-105.92888783639,173.492602186486));
#17427=CARTESIAN_POINT('Ctrl Pts',(-56.8055182225545,-107.997551398667,
173.49242733338));
#17428=CARTESIAN_POINT('Ctrl Pts',(-55.4580190214013,-108.147821158181,
173.623328602317));
#17429=CARTESIAN_POINT('Ctrl Pts',(-55.4580190214013,-108.147821158181,
174.985485069079));
#17430=CARTESIAN_POINT('Ctrl Pts',(-56.782663963309,-107.792612652652,173.49242733338));
#17431=CARTESIAN_POINT('Ctrl Pts',(-55.4352004895909,-107.943202787283,
173.623328602317));
#17432=CARTESIAN_POINT('Ctrl Pts',(-55.4352004895902,-107.943202787283,
174.985485069079));
#17433=CARTESIAN_POINT('Ctrl Pts',(-56.7597366258735,-107.587682138219,
173.49242733338));
#17434=CARTESIAN_POINT('Ctrl Pts',(-55.4123091474965,-107.738594013066,
173.623328602317));
#17435=CARTESIAN_POINT('Ctrl Pts',(-55.4123091475014,-107.738594013066,
174.985485069079));
#17436=CARTESIAN_POINT('Ctrl Pts',(-56.736735577699,-107.382759927281,173.49242733338));
#17437=CARTESIAN_POINT('Ctrl Pts',(-55.3893443675666,-107.533994925185,
173.623328602317));
#17438=CARTESIAN_POINT('Ctrl Pts',(-55.3893443675666,-107.533994925185,
174.985485069079));
#17439=CARTESIAN_POINT('Ctrl Pts',(-56.7665905243134,-107.788178276074,
173.49400046535));
#17440=CARTESIAN_POINT('Ctrl Pts',(-56.5949052326937,-107.845388680746,
173.512938947022));
#17441=CARTESIAN_POINT('Ctrl Pts',(-56.4264957959128,-107.897156142464,
173.56332723609));
#17442=CARTESIAN_POINT('Ctrl Pts',(-56.1084920846803,-107.988893243531,
173.726346578407));
#17443=CARTESIAN_POINT('Ctrl Pts',(-55.9624918596245,-108.027899351649,
173.839287986585));
#17444=CARTESIAN_POINT('Ctrl Pts',(-55.8081013798708,-108.067392125105,
174.013093118869));
#17445=CARTESIAN_POINT('Ctrl Pts',(-55.7778479504432,-108.074998097689,
174.050644783342));
#17446=CARTESIAN_POINT('Ctrl Pts',(-55.7374518773692,-108.084976413728,
174.106049041317));
#17447=CARTESIAN_POINT('Ctrl Pts',(-55.7258247337975,-108.087824947824,
174.122691724583));
#17448=CARTESIAN_POINT('Ctrl Pts',(-55.7039020480952,-108.093150795867,
174.155461392321));
#17449=CARTESIAN_POINT('Ctrl Pts',(-55.6935706101721,-108.095639569752,
174.17155735823));
#17450=CARTESIAN_POINT('Ctrl Pts',(-55.608443919145,-108.115967969813,174.309888289955));
#17451=CARTESIAN_POINT('Ctrl Pts',(-55.5507627722578,-108.12854889235,174.442461042842));
#17452=CARTESIAN_POINT('Ctrl Pts',(-55.4761499414694,-108.142169695467,
174.713017710041));
#17453=CARTESIAN_POINT('Ctrl Pts',(-55.4575623940107,-108.143726509878,
174.848944909728));
#17454=CARTESIAN_POINT('Ctrl Pts',(-55.4571650701274,-108.140163914373,
174.985485069079));
#17455=CARTESIAN_POINT('Ctrl Pts',(-55.4039785948117,-107.664464934563,
174.985485069077));
#17456=CARTESIAN_POINT('Ctrl Pts',(-55.4014083953031,-107.641534765974,
174.851826866554));
#17457=CARTESIAN_POINT('Ctrl Pts',(-55.4169241878019,-107.619574533909,
174.718312672541));
#17458=CARTESIAN_POINT('Ctrl Pts',(-55.4881074621261,-107.575119044012,
174.442449886533));
#17459=CARTESIAN_POINT('Ctrl Pts',(-55.5481519170216,-107.553177440629,
174.30284539021));
#17460=CARTESIAN_POINT('Ctrl Pts',(-55.6341776305828,-107.531750474155,
174.166061967665));
#17461=CARTESIAN_POINT('Ctrl Pts',(-55.6397004507487,-107.53040670336,174.157481019746));
#17462=CARTESIAN_POINT('Ctrl Pts',(-55.6573708437641,-107.526205542954,
174.130647331335));
#17463=CARTESIAN_POINT('Ctrl Pts',(-55.669841458162,-107.523382361785,174.112605920834));
#17464=CARTESIAN_POINT('Ctrl Pts',(-55.7103922997075,-107.514630979822,
174.056672899912));
#17465=CARTESIAN_POINT('Ctrl Pts',(-55.7399114236766,-107.508869519605,
174.019839086604));
#17466=CARTESIAN_POINT('Ctrl Pts',(-55.8983246981518,-107.480807006229,
173.840659718242));
#17467=CARTESIAN_POINT('Ctrl Pts',(-56.0526068341962,-107.462494558611,
173.723111091821));
#17468=CARTESIAN_POINT('Ctrl Pts',(-56.3830049352595,-107.435395780513,
173.560934379101));
#17469=CARTESIAN_POINT('Ctrl Pts',(-56.5529996701729,-107.425951563239,
173.512127246035));
#17470=CARTESIAN_POINT('Ctrl Pts',(-56.7277951555015,-107.420782694947,
173.49375276819));
#17471=CARTESIAN_POINT('Ctrl Pts',(-56.9621866626637,-109.489802972882,
173.493261648264));
#17472=CARTESIAN_POINT('Ctrl Pts',(-55.6227768443799,-109.636849320768,
173.631005581965));
#17473=CARTESIAN_POINT('Ctrl Pts',(-55.6227768443799,-109.636849320768,
174.985485069079));
#17474=CARTESIAN_POINT('Ctrl Pts',(-56.9397670005278,-109.285587662391,
173.493261648264));
#17475=CARTESIAN_POINT('Ctrl Pts',(-55.6003912981915,-109.432944764224,
173.631005581965));
#17476=CARTESIAN_POINT('Ctrl Pts',(-55.600391298188,-109.432944764224,174.985485069079));
#17477=CARTESIAN_POINT('Ctrl Pts',(-56.9172762923776,-109.081380361356,
173.49326164826));
#17478=CARTESIAN_POINT('Ctrl Pts',(-55.5779349587329,-109.22904952246,173.63100558192));
#17479=CARTESIAN_POINT('Ctrl Pts',(-55.5779349587373,-109.229049522459,
174.985485069034));
#17480=CARTESIAN_POINT('Ctrl Pts',(-56.8947139323498,-108.87718113875,173.493261648264));
#17481=CARTESIAN_POINT('Ctrl Pts',(-55.5554072248064,-109.025163681204,
173.631005581965));
#17482=CARTESIAN_POINT('Ctrl Pts',(-55.5554072248065,-109.025163681204,
174.98548506908));
#17483=CARTESIAN_POINT('Ctrl Pts',(-56.9243786881308,-109.279976942607,
173.494832944154));
#17484=CARTESIAN_POINT('Ctrl Pts',(-56.7538963361861,-109.336606160927,
173.514535334738));
#17485=CARTESIAN_POINT('Ctrl Pts',(-56.5867932277359,-109.387847708036,
173.565235192448));
#17486=CARTESIAN_POINT('Ctrl Pts',(-56.2702263316121,-109.478982732056,
173.728531078916));
#17487=CARTESIAN_POINT('Ctrl Pts',(-56.1245025623703,-109.517830055776,
173.841827344492));
#17488=CARTESIAN_POINT('Ctrl Pts',(-55.972216810626,-109.556695013004,174.014088641704));
#17489=CARTESIAN_POINT('Ctrl Pts',(-55.9435627449903,-109.563888754681,
174.049643091631));
#17490=CARTESIAN_POINT('Ctrl Pts',(-55.9044952972728,-109.573534138044,
174.102920514733));
#17491=CARTESIAN_POINT('Ctrl Pts',(-55.8927880988003,-109.576400871192,
174.119583578313));
#17492=CARTESIAN_POINT('Ctrl Pts',(-55.8707107628622,-109.581761653968,
174.152400753911));
#17493=CARTESIAN_POINT('Ctrl Pts',(-55.8603047098438,-109.584267172477,
174.16852362561));
#17494=CARTESIAN_POINT('Ctrl Pts',(-55.7745081060717,-109.604745566871,
174.307181765745));
#17495=CARTESIAN_POINT('Ctrl Pts',(-55.7163483209697,-109.617424971451,
174.440179457196));
#17496=CARTESIAN_POINT('Ctrl Pts',(-55.6410802083126,-109.631163216239,
174.711792204332));
#17497=CARTESIAN_POINT('Ctrl Pts',(-55.6223253405858,-109.632736702427,
174.848327690676));
#17498=CARTESIAN_POINT('Ctrl Pts',(-55.6219312570821,-109.629147380551,
174.985485069079));
#17499=CARTESIAN_POINT('Ctrl Pts',(-55.5699812776884,-109.157156757033,
174.985485069059));
#17500=CARTESIAN_POINT('Ctrl Pts',(-55.5675435745271,-109.135063848326,
174.856923057509));
#17501=CARTESIAN_POINT('Ctrl Pts',(-55.5818331979452,-109.113860418937,
174.728474891724));
#17502=CARTESIAN_POINT('Ctrl Pts',(-55.6474497152721,-109.070906537188,
174.463007451237));
#17503=CARTESIAN_POINT('Ctrl Pts',(-55.7027062177817,-109.049644761822,
174.328376230069));
#17504=CARTESIAN_POINT('Ctrl Pts',(-55.7874222731387,-109.027317500699,
174.18644210645));
#17505=CARTESIAN_POINT('Ctrl Pts',(-55.7981757523871,-109.0246146387,174.169247570115));
#17506=CARTESIAN_POINT('Ctrl Pts',(-55.8212392669884,-109.019079357439,
174.134020636803));
#17507=CARTESIAN_POINT('Ctrl Pts',(-55.8336024294317,-109.016253407579,
174.1160283696));
#17508=CARTESIAN_POINT('Ctrl Pts',(-55.8739377468614,-109.007462323059,
174.060054071408));
#17509=CARTESIAN_POINT('Ctrl Pts',(-55.9033558416481,-109.001663505812,
174.023128360552));
#17510=CARTESIAN_POINT('Ctrl Pts',(-56.0614490778147,-108.97337593563,173.843266153729));
#17511=CARTESIAN_POINT('Ctrl Pts',(-56.2156626186106,-108.954874796232,
173.725124931942));
#17512=CARTESIAN_POINT('Ctrl Pts',(-56.5444000502588,-108.927543158314,
173.562816682292));
#17513=CARTESIAN_POINT('Ctrl Pts',(-56.7125053750529,-108.917985710097,
173.513819867409));
#17514=CARTESIAN_POINT('Ctrl Pts',(-56.8854801878217,-108.912602509009,
173.494655322398));
#17515=CARTESIAN_POINT('Ctrl Pts',(-57.1194187443674,-110.982706994464,
173.493819516807));
#17516=CARTESIAN_POINT('Ctrl Pts',(-55.7850950242185,-111.12692947585,173.63589097676));
#17517=CARTESIAN_POINT('Ctrl Pts',(-55.7850950242185,-111.12692947585,174.98548506908));
#17518=CARTESIAN_POINT('Ctrl Pts',(-57.097378700238,-110.778795971744,173.493819516803));
#17519=CARTESIAN_POINT('Ctrl Pts',(-55.7630877058362,-110.923321226614,
173.635890976726));
#17520=CARTESIAN_POINT('Ctrl Pts',(-55.7630877058354,-110.923321226614,
174.985485069045));
#17521=CARTESIAN_POINT('Ctrl Pts',(-57.0752692869159,-110.574892773011,
173.493819516808));
#17522=CARTESIAN_POINT('Ctrl Pts',(-55.7410112583161,-110.719722057746,
173.635890976772));
#17523=CARTESIAN_POINT('Ctrl Pts',(-55.7410112583178,-110.719722057746,
174.985485069091));
#17524=CARTESIAN_POINT('Ctrl Pts',(-57.0530899203455,-110.370997464803,
173.493819516807));
#17525=CARTESIAN_POINT('Ctrl Pts',(-55.7188651019731,-110.51613205175,173.63589097676));
#17526=CARTESIAN_POINT('Ctrl Pts',(-55.7188651019731,-110.51613205175,174.985485069079));
#17527=CARTESIAN_POINT('Ctrl Pts',(-57.0826240442755,-110.77168183954,173.495354125426));
#17528=CARTESIAN_POINT('Ctrl Pts',(-56.9128280627272,-110.827975820923,
173.515513471879));
#17529=CARTESIAN_POINT('Ctrl Pts',(-56.7464720083201,-110.878915152489,
173.566405745216));
#17530=CARTESIAN_POINT('Ctrl Pts',(-56.4307568142368,-110.969695233241,
173.729873488259));
#17531=CARTESIAN_POINT('Ctrl Pts',(-56.2852156383961,-111.008446018537,
173.843360765196));
#17532=CARTESIAN_POINT('Ctrl Pts',(-56.1332269225956,-111.047185085229,
174.015760442495));
#17533=CARTESIAN_POINT('Ctrl Pts',(-56.1046589569938,-111.05434781301,174.05130245406));
#17534=CARTESIAN_POINT('Ctrl Pts',(-56.0657248932361,-111.063947318451,
174.104535558086));
#17535=CARTESIAN_POINT('Ctrl Pts',(-56.0540665026745,-111.06679822698,174.121170947796));
#17536=CARTESIAN_POINT('Ctrl Pts',(-56.0320806105947,-111.072129489664,
174.153932246034));
#17537=CARTESIAN_POINT('Ctrl Pts',(-56.0217173672487,-111.074621245229,
174.170027146221));
#17538=CARTESIAN_POINT('Ctrl Pts',(-55.9362556453455,-111.094991086755,
174.308465969329));
#17539=CARTESIAN_POINT('Ctrl Pts',(-55.8783248745144,-111.107599808822,
174.441208052489));
#17540=CARTESIAN_POINT('Ctrl Pts',(-55.8033352673517,-111.121252864932,
174.712299263541));
#17541=CARTESIAN_POINT('Ctrl Pts',(-55.7846493192605,-111.122805905128,
174.848582874691));
#17542=CARTESIAN_POINT('Ctrl Pts',(-55.7842612734033,-111.119216054728,
174.985485069078));
#17543=CARTESIAN_POINT('Ctrl Pts',(-55.7333536027297,-110.649417900359,
174.985485069077));
#17544=CARTESIAN_POINT('Ctrl Pts',(-55.7309690326988,-110.627465945723,
174.857863999367));
#17545=CARTESIAN_POINT('Ctrl Pts',(-55.7450628622825,-110.606386714262,
174.730354705224));
#17546=CARTESIAN_POINT('Ctrl Pts',(-55.8097005466027,-110.563683118527,
174.466889269619));
#17547=CARTESIAN_POINT('Ctrl Pts',(-55.8640743698788,-110.542533757114,
174.333251213159));
#17548=CARTESIAN_POINT('Ctrl Pts',(-55.959278319169,-110.517133998281,174.172148090414));
#17549=CARTESIAN_POINT('Ctrl Pts',(-55.9829900909391,-110.511413156019,
174.135807737448));
#17550=CARTESIAN_POINT('Ctrl Pts',(-56.0358028832275,-110.499830988273,
174.062235482721));
#17551=CARTESIAN_POINT('Ctrl Pts',(-56.0651604927824,-110.494007937226,
174.025247036739));
#17552=CARTESIAN_POINT('Ctrl Pts',(-56.2230849566472,-110.465571830551,
173.844911894683));
#17553=CARTESIAN_POINT('Ctrl Pts',(-56.3772962272133,-110.446946615986,
173.726368205424));
#17554=CARTESIAN_POINT('Ctrl Pts',(-56.704987133118,-110.419471069408,173.564004403809));
#17555=CARTESIAN_POINT('Ctrl Pts',(-56.871843629646,-110.409846826172,173.514911464148));
#17556=CARTESIAN_POINT('Ctrl Pts',(-57.043608201862,-110.40433147521,173.495256480951));
#17557=CARTESIAN_POINT('Ctrl Pts',(-57.0822389279392,-110.649056444086,
178.477039335021));
#17558=CARTESIAN_POINT('Ctrl Pts',(-55.7490106450711,-110.793662661806,
178.334126158632));
#17559=CARTESIAN_POINT('Ctrl Pts',(-55.7490106450711,-110.793662661806,
176.985485069079));
#17560=CARTESIAN_POINT('Ctrl Pts',(-57.1044155270742,-110.853518393605,
178.477039335021));
#17561=CARTESIAN_POINT('Ctrl Pts',(-55.7711541904733,-110.997819865288,
178.334126158632));
#17562=CARTESIAN_POINT('Ctrl Pts',(-55.7711541904754,-110.997819865288,
176.985485069079));
#17563=CARTESIAN_POINT('Ctrl Pts',(-57.126522089051,-111.057988548884,178.477039335021));
#17564=CARTESIAN_POINT('Ctrl Pts',(-55.793227942238,-111.201986545103,178.334126158632));
#17565=CARTESIAN_POINT('Ctrl Pts',(-55.7932279422347,-111.201986545103,
176.985485069079));
#17566=CARTESIAN_POINT('Ctrl Pts',(-57.1485591984125,-111.26246684077,178.477039335021));
#17567=CARTESIAN_POINT('Ctrl Pts',(-55.8152324805442,-111.406162616148,
178.334126158632));
#17568=CARTESIAN_POINT('Ctrl Pts',(-55.8152324805442,-111.406162616148,
176.985485069079));
#17569=CARTESIAN_POINT('',(-57.1318490822761,-111.234741954516,178.475522296093));
#17570=CARTESIAN_POINT('Ctrl Pts',(-55.8006548129686,-111.270994369076,
176.985485069082));
#17571=CARTESIAN_POINT('Ctrl Pts',(-55.8030222309522,-111.292930279278,
177.113081070041));
#17572=CARTESIAN_POINT('Ctrl Pts',(-55.8212991787659,-111.31054480159,177.240557658034));
#17573=CARTESIAN_POINT('Ctrl Pts',(-55.8935168729266,-111.338617326837,
177.503776803771));
#17574=CARTESIAN_POINT('Ctrl Pts',(-55.9510512132407,-111.347819958795,
177.637222406408));
#17575=CARTESIAN_POINT('Ctrl Pts',(-56.0492820653997,-111.352596896656,
177.798114695378));
#17576=CARTESIAN_POINT('Ctrl Pts',(-56.0736131933765,-111.353196783989,
177.834404081079));
#17577=CARTESIAN_POINT('Ctrl Pts',(-56.1276211701236,-111.353403281168,
177.907968380396));
#17578=CARTESIAN_POINT('Ctrl Pts',(-56.1575481140501,-111.352916066103,
177.944995033058));
#17579=CARTESIAN_POINT('Ctrl Pts',(-56.3180516517131,-111.347464517362,
178.125655363643));
#17580=CARTESIAN_POINT('Ctrl Pts',(-56.4729341378883,-111.333173910538,
178.244439479484));
#17581=CARTESIAN_POINT('Ctrl Pts',(-56.7988031792984,-111.29103742598,178.406700803439));
#17582=CARTESIAN_POINT('Ctrl Pts',(-56.9633576095936,-111.265401839379,
178.455737245865));
#17583=CARTESIAN_POINT('Ctrl Pts',(-57.1318490822761,-111.234741954516,
178.475522296092));
#17584=CARTESIAN_POINT('',(-57.0927973172532,-110.86741985642,178.475593938758));
#17585=CARTESIAN_POINT('',(-57.1318490822761,-111.234741954516,178.475522296093));
#17586=CARTESIAN_POINT('Ctrl Pts',(-57.0927973172543,-110.867419856423,
178.475593938747));
#17587=CARTESIAN_POINT('Ctrl Pts',(-56.9147592776452,-110.848167673894,
178.455404659106));
#17588=CARTESIAN_POINT('Ctrl Pts',(-56.7412161395771,-110.833424542233,
178.404457924272));
#17589=CARTESIAN_POINT('Ctrl Pts',(-56.413411971825,-110.811230540968,178.240940728206));
#17590=CARTESIAN_POINT('Ctrl Pts',(-56.2630572878917,-110.80402401403,178.12756038466));
#17591=CARTESIAN_POINT('Ctrl Pts',(-56.1062997177754,-110.79818089641,177.95525199714));
#17592=CARTESIAN_POINT('Ctrl Pts',(-56.0768080828725,-110.797196991731,
177.919660793991));
#17593=CARTESIAN_POINT('Ctrl Pts',(-56.0366890993698,-110.796016297223,
177.866398529148));
#17594=CARTESIAN_POINT('Ctrl Pts',(-56.0247049838097,-110.795686419516,
177.849788446774));
#17595=CARTESIAN_POINT('Ctrl Pts',(-56.0021106664059,-110.795108182657,
177.81707364697));
#17596=CARTESIAN_POINT('Ctrl Pts',(-55.9914633711863,-110.794856233593,
177.800999769791));
#17597=CARTESIAN_POINT('Ctrl Pts',(-55.9036287919606,-110.792951291756,
177.662641392075));
#17598=CARTESIAN_POINT('Ctrl Pts',(-55.8443255099797,-110.792830832311,
177.529959747674));
#17599=CARTESIAN_POINT('Ctrl Pts',(-55.76806551622,-110.795283517144,177.258846135829));
#17600=CARTESIAN_POINT('Ctrl Pts',(-55.7494490397083,-110.797704553748,
177.122475998923));
#17601=CARTESIAN_POINT('Ctrl Pts',(-55.7498389523166,-110.801299724063,
176.98548506908));
#17602=CARTESIAN_POINT('Ctrl Pts',(-56.9232540372578,-109.154004151255,
178.477503703266));
#17603=CARTESIAN_POINT('Ctrl Pts',(-55.5858787857402,-109.301345064959,
178.338149647288));
#17604=CARTESIAN_POINT('Ctrl Pts',(-55.5858787857403,-109.301345064959,
176.985485069079));
#17605=CARTESIAN_POINT('Ctrl Pts',(-56.9458762959346,-109.359340524723,
178.477503703266));
#17606=CARTESIAN_POINT('Ctrl Pts',(-55.6084665105141,-109.506367983156,
178.338149647288));
#17607=CARTESIAN_POINT('Ctrl Pts',(-55.6084665105118,-109.506367983157,
176.985485069079));
#17608=CARTESIAN_POINT('Ctrl Pts',(-56.968426419469,-109.564685347002,178.477503703266));
#17609=CARTESIAN_POINT('Ctrl Pts',(-55.6309823578394,-109.7114006768,178.338149647288));
#17610=CARTESIAN_POINT('Ctrl Pts',(-55.630982357837,-109.711400676801,176.985485069079));
#17611=CARTESIAN_POINT('Ctrl Pts',(-56.9909050192882,-109.770038545797,
178.477503703266));
#17612=CARTESIAN_POINT('Ctrl Pts',(-55.6534269344576,-109.916443056728,
178.338149647288));
#17613=CARTESIAN_POINT('Ctrl Pts',(-55.6534269344576,-109.916443056728,
176.985485069079));
#17614=CARTESIAN_POINT('',(-56.9734652393652,-109.7431874274,178.475940356875));
#17615=CARTESIAN_POINT('Ctrl Pts',(-55.6385532353225,-109.78066106394,176.985485069082));
#17616=CARTESIAN_POINT('Ctrl Pts',(-55.6409594189848,-109.802611489716,
177.11336531854));
#17617=CARTESIAN_POINT('Ctrl Pts',(-55.6593416836102,-109.820220945236,
177.24112020221));
#17618=CARTESIAN_POINT('Ctrl Pts',(-55.7318960116661,-109.848235538582,
177.504810124576));
#17619=CARTESIAN_POINT('Ctrl Pts',(-55.7896567465906,-109.857385583657,
177.638440485888));
#17620=CARTESIAN_POINT('Ctrl Pts',(-55.8882344934935,-109.862070690011,
177.799495074151));
#17621=CARTESIAN_POINT('Ctrl Pts',(-55.9126451019893,-109.862647764504,
177.835811023265));
#17622=CARTESIAN_POINT('Ctrl Pts',(-55.9667916934297,-109.862803717785,
177.909375509078));
#17623=CARTESIAN_POINT('Ctrl Pts',(-55.9967740152662,-109.862289944981,
177.946377912396));
#17624=CARTESIAN_POINT('Ctrl Pts',(-56.1575492729998,-109.85670279429,178.126897146243));
#17625=CARTESIAN_POINT('Ctrl Pts',(-56.3126249340782,-109.842303243046,
178.245523765821));
#17626=CARTESIAN_POINT('Ctrl Pts',(-56.6392348626847,-109.799895618343,
178.407624573229));
#17627=CARTESIAN_POINT('Ctrl Pts',(-56.804403867627,-109.774067823015,178.4565096845));
#17628=CARTESIAN_POINT('Ctrl Pts',(-56.9734652393652,-109.7431874274,178.475940356874));
#17629=CARTESIAN_POINT('',(-56.9345361076167,-109.375864092667,178.476093934548));
#17630=CARTESIAN_POINT('',(-56.9734652393652,-109.7431874274,178.475940356875));
#17631=CARTESIAN_POINT('Ctrl Pts',(-56.9345361076177,-109.37586409267,178.476093934536));
#17632=CARTESIAN_POINT('Ctrl Pts',(-56.7555615318508,-109.356409036724,
178.456331596915));
#17633=CARTESIAN_POINT('Ctrl Pts',(-56.5810328056178,-109.341507923764,
178.405522603758));
#17634=CARTESIAN_POINT('Ctrl Pts',(-56.2522717149334,-109.319133494151,
178.242127257605));
#17635=CARTESIAN_POINT('Ctrl Pts',(-56.1018037389524,-109.311861568565,
178.129046621873));
#17636=CARTESIAN_POINT('Ctrl Pts',(-55.9447093653116,-109.305940907224,
177.956969033457));
#17637=CARTESIAN_POINT('Ctrl Pts',(-55.9150694097991,-109.304939856116,
177.921314909201));
#17638=CARTESIAN_POINT('Ctrl Pts',(-55.8747729217627,-109.303737332467,
177.867978487055));
#17639=CARTESIAN_POINT('Ctrl Pts',(-55.8627515212982,-109.303401425641,
177.851366853639));
#17640=CARTESIAN_POINT('Ctrl Pts',(-55.840083744564,-109.302811767932,177.818644194178));
#17641=CARTESIAN_POINT('Ctrl Pts',(-55.8294003481997,-109.302554418962,
177.802564065397));
#17642=CARTESIAN_POINT('Ctrl Pts',(-55.7412161662989,-109.300603909226,
177.664069577128));
#17643=CARTESIAN_POINT('Ctrl Pts',(-55.6816569414381,-109.300454409692,
177.531194877827));
#17644=CARTESIAN_POINT('Ctrl Pts',(-55.6050255745782,-109.302871854621,
177.259535984071));
#17645=CARTESIAN_POINT('Ctrl Pts',(-55.5863131000029,-109.305287236401,
177.122823740951));
#17646=CARTESIAN_POINT('Ctrl Pts',(-55.5867097138724,-109.308887482778,
176.985485069079));
#17647=CARTESIAN_POINT('Ctrl Pts',(-56.7646390135495,-107.658044645611,
178.47825681256));
#17648=CARTESIAN_POINT('Ctrl Pts',(-55.4201132624748,-107.808520799227,
178.344956154987));
#17649=CARTESIAN_POINT('Ctrl Pts',(-55.4201132624748,-107.808520799227,
176.985485069079));
#17650=CARTESIAN_POINT('Ctrl Pts',(-56.7877654331416,-107.864682481035,
178.478256812562));
#17651=CARTESIAN_POINT('Ctrl Pts',(-55.4432034350782,-108.014834762672,
178.34495615501));
#17652=CARTESIAN_POINT('Ctrl Pts',(-55.4432034350741,-108.014834762673,
176.985485069102));
#17653=CARTESIAN_POINT('Ctrl Pts',(-56.8108172327237,-108.071329050187,
178.478256812557));
#17654=CARTESIAN_POINT('Ctrl Pts',(-55.4662192622098,-108.221158854215,
178.344956154953));
#17655=CARTESIAN_POINT('Ctrl Pts',(-55.4662192622078,-108.221158854215,
176.985485069045));
#17656=CARTESIAN_POINT('Ctrl Pts',(-56.8337950559789,-108.277984277046,
178.47825681256));
#17657=CARTESIAN_POINT('Ctrl Pts',(-55.4891613824828,-108.427492979837,
178.344956154987));
#17658=CARTESIAN_POINT('Ctrl Pts',(-55.4891613824828,-108.427492979837,
176.98548506908));
#17659=CARTESIAN_POINT('',(-56.8155634335305,-108.251628031083,178.476680214078));
#17660=CARTESIAN_POINT('Ctrl Pts',(-55.4740061171911,-108.291289155992,
176.985485069082));
#17661=CARTESIAN_POINT('Ctrl Pts',(-55.4764658987439,-108.313379911227,
177.114480114835));
#17662=CARTESIAN_POINT('Ctrl Pts',(-55.4951767887661,-108.33105141348,177.24333814957));
#17663=CARTESIAN_POINT('Ctrl Pts',(-55.5689898174003,-108.359032051728,
177.509171060714));
#17664=CARTESIAN_POINT('Ctrl Pts',(-55.6277353931126,-108.368063831478,
177.6437815552));
#17665=CARTESIAN_POINT('Ctrl Pts',(-55.7154894664664,-108.371922802339,
177.785651423283));
#17666=CARTESIAN_POINT('Ctrl Pts',(-55.7265931139023,-108.372284875476,
177.802828744998));
#17667=CARTESIAN_POINT('Ctrl Pts',(-55.7503497799542,-108.372807237009,
177.838021307392));
#17668=CARTESIAN_POINT('Ctrl Pts',(-55.7630532947064,-108.372950036688,
177.855996422835));
#17669=CARTESIAN_POINT('Ctrl Pts',(-55.804450631013,-108.372999404612,177.911981060336));
#17670=CARTESIAN_POINT('Ctrl Pts',(-55.8345248860353,-108.372437876787,
177.948929958811));
#17671=CARTESIAN_POINT('Ctrl Pts',(-55.9957097052851,-108.366608583803,
178.129104713902));
#17672=CARTESIAN_POINT('Ctrl Pts',(-56.1510382185471,-108.35202200111,178.247387779987));
#17673=CARTESIAN_POINT('Ctrl Pts',(-56.4789706596083,-108.309128697421,
178.409249582182));
#17674=CARTESIAN_POINT('Ctrl Pts',(-56.6453603770763,-108.282932908725,
178.457893915397));
#17675=CARTESIAN_POINT('Ctrl Pts',(-56.8155634335305,-108.251628031083,
178.476680214078));
#17676=CARTESIAN_POINT('',(-56.7767448738944,-107.884303575429,178.476907478761));
#17677=CARTESIAN_POINT('',(-56.8155634335305,-108.251628031083,178.476680214078));
#17678=CARTESIAN_POINT('Ctrl Pts',(-56.7767448738954,-107.884303575432,
178.476907478748));
#17679=CARTESIAN_POINT('Ctrl Pts',(-56.5962729667804,-107.864513578287,
178.457879613496));
#17680=CARTESIAN_POINT('Ctrl Pts',(-56.4201604123224,-107.849352852162,
178.407328813957));
#17681=CARTESIAN_POINT('Ctrl Pts',(-56.0898126794775,-107.826678692935,
178.244160776659));
#17682=CARTESIAN_POINT('Ctrl Pts',(-55.9391249447214,-107.819299905284,
178.131544466062));
#17683=CARTESIAN_POINT('Ctrl Pts',(-55.7814712700151,-107.813254304601,
177.959821319822));
#17684=CARTESIAN_POINT('Ctrl Pts',(-55.7516010922104,-107.812225889799,
177.924078918995));
#17685=CARTESIAN_POINT('Ctrl Pts',(-55.7110190459911,-107.81098815467,177.870628909897));
#17686=CARTESIAN_POINT('Ctrl Pts',(-55.6989308113585,-107.810642364463,
177.854006513428));
#17687=CARTESIAN_POINT('Ctrl Pts',(-55.6761329314457,-107.810034054685,
177.821255733448));
#17688=CARTESIAN_POINT('Ctrl Pts',(-55.6653863067212,-107.809767916626,
177.805158398335));
#17689=CARTESIAN_POINT('Ctrl Pts',(-55.5766160932854,-107.807743752311,
177.666411573885));
#17690=CARTESIAN_POINT('Ctrl Pts',(-55.5166331037104,-107.807547831138,
177.533195240923));
#17691=CARTESIAN_POINT('Ctrl Pts',(-55.4394039866848,-107.809908992442,
177.260632619921));
#17692=CARTESIAN_POINT('Ctrl Pts',(-55.4205378716355,-107.812314749534,
177.123376449463));
#17693=CARTESIAN_POINT('Ctrl Pts',(-55.4209415581552,-107.815922027774,
176.98548506908));
#17694=CARTESIAN_POINT('Ctrl Pts',(-56.6063169754422,-106.161159974594,
178.479251376));
#17695=CARTESIAN_POINT('Ctrl Pts',(-55.2516552698864,-106.315188128166,
178.354564947683));
#17696=CARTESIAN_POINT('Ctrl Pts',(-55.2516552698864,-106.315188128166,
176.985485069079));
#17697=CARTESIAN_POINT('Ctrl Pts',(-56.6300126762584,-106.369561216403,
178.479251375997));
#17698=CARTESIAN_POINT('Ctrl Pts',(-55.2753127466082,-106.523253193008,
178.354564947649));
#17699=CARTESIAN_POINT('Ctrl Pts',(-55.2753127466048,-106.523253193008,
176.985485069044));
#17700=CARTESIAN_POINT('Ctrl Pts',(-56.6536308295825,-106.577971524729,
178.479251376));
#17701=CARTESIAN_POINT('Ctrl Pts',(-55.2988929703655,-106.731328799967,
178.354564947683));
#17702=CARTESIAN_POINT('Ctrl Pts',(-55.2988929703647,-106.731328799967,
176.985485069079));
#17703=CARTESIAN_POINT('Ctrl Pts',(-56.6771721177013,-106.786390819126,
178.479251376));
#17704=CARTESIAN_POINT('Ctrl Pts',(-55.3223966179213,-106.939414849226,
178.354564947683));
#17705=CARTESIAN_POINT('Ctrl Pts',(-55.3223966179213,-106.939414849226,
176.985485069079));
#17706=CARTESIAN_POINT('',(-56.6580826427064,-106.760064354331,178.477700244368));
#17707=CARTESIAN_POINT('Ctrl Pts',(-55.3069657209396,-106.802898527557,
176.985485069082));
#17708=CARTESIAN_POINT('Ctrl Pts',(-55.3095589298666,-106.825823912651,
177.119764397273));
#17709=CARTESIAN_POINT('Ctrl Pts',(-55.329756417029,-106.843953781154,177.253864484605));
#17710=CARTESIAN_POINT('Ctrl Pts',(-55.4096086469019,-106.87214148342,177.530214923199));
#17711=CARTESIAN_POINT('Ctrl Pts',(-55.4732767885331,-106.880780792608,
177.669761195188));
#17712=CARTESIAN_POINT('Ctrl Pts',(-55.5621868299431,-106.883447490003,
177.806441021704));
#17713=CARTESIAN_POINT('Ctrl Pts',(-55.5678844737477,-106.883587748771,
177.815010837929));
#17714=CARTESIAN_POINT('Ctrl Pts',(-55.5860916690433,-106.883941267773,
177.841809516667));
#17715=CARTESIAN_POINT('Ctrl Pts',(-55.5989085506571,-106.884053392005,
177.859827009987));
#17716=CARTESIAN_POINT('Ctrl Pts',(-55.6405535382393,-106.884002227609,
177.915774224524));
#17717=CARTESIAN_POINT('Ctrl Pts',(-55.6707558780194,-106.883371657133,
177.952640181471));
#17718=CARTESIAN_POINT('Ctrl Pts',(-55.8324857653739,-106.877193480759,
178.132266860809));
#17719=CARTESIAN_POINT('Ctrl Pts',(-55.988124979762,-106.86234169041,178.250020609912));
#17720=CARTESIAN_POINT('Ctrl Pts',(-56.3179590299471,-106.81874460688,178.411558382723));
#17721=CARTESIAN_POINT('Ctrl Pts',(-56.4861730086404,-106.792001449029,
178.459861811937));
#17722=CARTESIAN_POINT('Ctrl Pts',(-56.6580826427064,-106.760064354331,
178.477700244367));
#17723=CARTESIAN_POINT('',(-56.6193547970192,-106.392738970839,178.477987698341));
#17724=CARTESIAN_POINT('',(-56.6580826427064,-106.760064354331,178.477700244368));
#17725=CARTESIAN_POINT('Ctrl Pts',(-56.6193547970202,-106.392738970842,
178.477987698327));
#17726=CARTESIAN_POINT('Ctrl Pts',(-56.4368347272708,-106.372479290791,
178.460016009567));
#17727=CARTESIAN_POINT('Ctrl Pts',(-56.2585452960474,-106.356954969072,
178.409857125584));
#17728=CARTESIAN_POINT('Ctrl Pts',(-55.9259821398569,-106.33385926111,178.247031357291));
#17729=CARTESIAN_POINT('Ctrl Pts',(-55.7749667750593,-106.326331504666,
178.135042067197));
#17730=CARTESIAN_POINT('Ctrl Pts',(-55.6165302667828,-106.320112685004,
177.963795620031));
#17731=CARTESIAN_POINT('Ctrl Pts',(-55.5863473744548,-106.319046346214,
177.927940434316));
#17732=CARTESIAN_POINT('Ctrl Pts',(-55.5453711490126,-106.317759594012,
177.874338528708));
#17733=CARTESIAN_POINT('Ctrl Pts',(-55.5331865443366,-106.31739996492,177.857696549508));
#17734=CARTESIAN_POINT('Ctrl Pts',(-55.515785173297,-106.316919677115,177.832865301265));
#17735=CARTESIAN_POINT('Ctrl Pts',(-55.5102973815779,-106.316773369357,
177.824869653524));
#17736=CARTESIAN_POINT('Ctrl Pts',(-55.4943714687919,-106.316363895439,
177.801173623749));
#17737=CARTESIAN_POINT('Ctrl Pts',(-55.4841525646855,-106.316120843354,
177.785328044534));
#17738=CARTESIAN_POINT('Ctrl Pts',(-55.3998699166634,-106.314282856012,
177.649024294688));
#17739=CARTESIAN_POINT('Ctrl Pts',(-55.3430285159645,-106.314163697371,
177.518809435036));
#17740=CARTESIAN_POINT('Ctrl Pts',(-55.2699140586195,-106.31654102514,177.253130960667));
#17741=CARTESIAN_POINT('Ctrl Pts',(-55.2520765286572,-106.318893063481,
177.119599537937));
#17742=CARTESIAN_POINT('Ctrl Pts',(-55.2524742173427,-106.322390962095,
176.985485069079));
#17743=CARTESIAN_POINT('Ctrl Pts',(-56.4481805239386,-104.663337987308,
178.480419827436));
#17744=CARTESIAN_POINT('Ctrl Pts',(-55.0804443419474,-104.821348467162,
178.366983319731));
#17745=CARTESIAN_POINT('Ctrl Pts',(-55.0804443419474,-104.821348467162,
176.98548506908));
#17746=CARTESIAN_POINT('Ctrl Pts',(-56.4725158438094,-104.873984126249,
178.480419827432));
#17747=CARTESIAN_POINT('Ctrl Pts',(-55.1047391646424,-105.031644063198,
178.366983319684));
#17748=CARTESIAN_POINT('Ctrl Pts',(-55.1047391646466,-105.031644063197,
176.985485069032));
#17749=CARTESIAN_POINT('Ctrl Pts',(-56.4967701946591,-105.084639717741,
178.480419827436));
#17750=CARTESIAN_POINT('Ctrl Pts',(-55.1289533365054,-105.241950684034,
178.366983319731));
#17751=CARTESIAN_POINT('Ctrl Pts',(-55.1289533365085,-105.241950684034,
176.985485069079));
#17752=CARTESIAN_POINT('Ctrl Pts',(-56.5209443047536,-105.295304676109,
178.480419827436));
#17753=CARTESIAN_POINT('Ctrl Pts',(-55.1530875797156,-105.452268222959,
178.366983319731));
#17754=CARTESIAN_POINT('Ctrl Pts',(-55.1530875797156,-105.452268222959,
176.985485069079));
#17755=CARTESIAN_POINT('',(-56.5009308898174,-105.268497296389,178.478938088823));
#17756=CARTESIAN_POINT('Ctrl Pts',(-55.1373829400717,-105.315510127364,
176.985485069083));
#17757=CARTESIAN_POINT('Ctrl Pts',(-55.139935036767,-105.337717924091,177.116060375578));
#17758=CARTESIAN_POINT('Ctrl Pts',(-55.1591285187234,-105.355388783739,
177.246478394228));
#17759=CARTESIAN_POINT('Ctrl Pts',(-55.2347312636371,-105.383111126789,
177.515243096824));
#17760=CARTESIAN_POINT('Ctrl Pts',(-55.2948363692995,-105.391860549335,
177.65114778878));
#17761=CARTESIAN_POINT('Ctrl Pts',(-55.3845226483519,-105.39524301998,177.794070257923));
#17762=CARTESIAN_POINT('Ctrl Pts',(-55.3958619777939,-105.395543966573,
177.811358415504));
#17763=CARTESIAN_POINT('Ctrl Pts',(-55.4201164687611,-105.395934349373,
177.846761528336));
#17764=CARTESIAN_POINT('Ctrl Pts',(-55.4330826876001,-105.396005988558,
177.864835189548));
#17765=CARTESIAN_POINT('Ctrl Pts',(-55.475048770948,-105.395822915869,177.920729993758));
#17766=CARTESIAN_POINT('Ctrl Pts',(-55.5054144853479,-105.395102052341,
177.95748353685));
#17767=CARTESIAN_POINT('Ctrl Pts',(-55.6678208283352,-105.388468834203,
178.136360265097));
#17768=CARTESIAN_POINT('Ctrl Pts',(-55.8238259562453,-105.373274146514,
178.253401157095));
#17769=CARTESIAN_POINT('Ctrl Pts',(-56.1561325155399,-105.328751722564,
178.414520859981));
#17770=CARTESIAN_POINT('Ctrl Pts',(-56.3267651109123,-105.301278060031,
178.462368244637));
#17771=CARTESIAN_POINT('Ctrl Pts',(-56.5009308898174,-105.268497296389,
178.478938088822));
#17772=CARTESIAN_POINT('',(-56.462266632785,-104.901171252502,178.479267413549));
#17773=CARTESIAN_POINT('',(-56.5009308898174,-105.268497296389,178.478938088823));
#17774=CARTESIAN_POINT('Ctrl Pts',(-56.4622666327859,-104.901171252505,
178.479267413534));
#17775=CARTESIAN_POINT('Ctrl Pts',(-56.2771642179805,-104.880304301774,
178.46269045673));
#17776=CARTESIAN_POINT('Ctrl Pts',(-56.0961152238312,-104.864309854259,
178.413073717723));
#17777=CARTESIAN_POINT('Ctrl Pts',(-55.7607146838184,-104.840668369511,
178.250716473028));
#17778=CARTESIAN_POINT('Ctrl Pts',(-55.6092642890516,-104.832949042415,
178.139513891316));
#17779=CARTESIAN_POINT('Ctrl Pts',(-55.4486812284957,-104.82646180254,177.967642939846));
#17780=CARTESIAN_POINT('Ctrl Pts',(-55.4170806160678,-104.825313937519,
177.930322194352));
#17781=CARTESIAN_POINT('Ctrl Pts',(-55.3748234624629,-104.823951063456,
177.875140746089));
#17782=CARTESIAN_POINT('Ctrl Pts',(-55.3626241599256,-104.823580554528,
177.85850795651));
#17783=CARTESIAN_POINT('Ctrl Pts',(-55.3452002756585,-104.823084593115,
177.83368874429));
#17784=CARTESIAN_POINT('Ctrl Pts',(-55.3397048128954,-104.822933313132,
177.825696206482));
#17785=CARTESIAN_POINT('Ctrl Pts',(-55.3290289750007,-104.822649521151,
177.809840195386));
#17786=CARTESIAN_POINT('Ctrl Pts',(-55.3238443417221,-104.822516596407,
177.801980167301));
#17787=CARTESIAN_POINT('Ctrl Pts',(-55.2393275090736,-104.820430490539,
177.671169918897));
#17788=CARTESIAN_POINT('Ctrl Pts',(-55.1784777690603,-104.820106204412,
177.537275226144));
#17789=CARTESIAN_POINT('Ctrl Pts',(-55.1000138889637,-104.822301340755,
177.262882339598));
#17790=CARTESIAN_POINT('Ctrl Pts',(-55.0808280652764,-104.824669959404,
177.124510689081));
#17791=CARTESIAN_POINT('Ctrl Pts',(-55.0812452693716,-104.828281539026,
176.985485069079));
#17792=CARTESIAN_POINT('Ctrl Pts',(-56.2900948296076,-103.164573183438,
178.481676597204));
#17793=CARTESIAN_POINT('Ctrl Pts',(-54.9064184039505,-103.327007356746,
178.382209459588));
#17794=CARTESIAN_POINT('Ctrl Pts',(-54.9064184039505,-103.327007356746,
176.985485069079));
#17795=CARTESIAN_POINT('Ctrl Pts',(-56.315136870002,-103.377890863102,178.481676597204));
#17796=CARTESIAN_POINT('Ctrl Pts',(-54.9314173573655,-103.53995800504,178.382209459588));
#17797=CARTESIAN_POINT('Ctrl Pts',(-54.9314173573688,-103.539958005039,
176.985485069079));
#17798=CARTESIAN_POINT('Ctrl Pts',(-56.3400940264076,-103.591218433758,
178.481676597204));
#17799=CARTESIAN_POINT('Ctrl Pts',(-54.9563317726869,-103.752920229724,
178.382209459588));
#17800=CARTESIAN_POINT('Ctrl Pts',(-54.9563317726919,-103.752920229724,
176.985485069079));
#17801=CARTESIAN_POINT('Ctrl Pts',(-56.3649670808697,-103.80455580367,178.481676597204));
#17802=CARTESIAN_POINT('Ctrl Pts',(-54.9811624251918,-103.965893916035,
178.382209459588));
#17803=CARTESIAN_POINT('Ctrl Pts',(-54.9811624251918,-103.965893916035,
176.985485069079));
#17804=CARTESIAN_POINT('',(-56.343987871522,-103.776928050381,178.480312727066));
#17805=CARTESIAN_POINT('Ctrl Pts',(-54.9652072511181,-103.82914600553,176.985485069083));
#17806=CARTESIAN_POINT('Ctrl Pts',(-54.9678127841589,-103.851461015716,
177.117296539967));
#17807=CARTESIAN_POINT('Ctrl Pts',(-54.9873706365605,-103.869145711318,
177.248936771374));
#17808=CARTESIAN_POINT('Ctrl Pts',(-55.064373529731,-103.896698018697,177.520046945381));
#17809=CARTESIAN_POINT('Ctrl Pts',(-55.1255699889516,-103.90523950117,177.657007192595));
#17810=CARTESIAN_POINT('Ctrl Pts',(-55.2110381744666,-103.908065861991,
177.791675329049));
#17811=CARTESIAN_POINT('Ctrl Pts',(-55.2165132019378,-103.908217279327,
177.800118301497));
#17812=CARTESIAN_POINT('Ctrl Pts',(-55.2278316868487,-103.908471032756,
177.817203493515));
#17813=CARTESIAN_POINT('Ctrl Pts',(-55.2336809623173,-103.908571361852,
177.82584119157));
#17814=CARTESIAN_POINT('Ctrl Pts',(-55.2523681669576,-103.908796662826,
177.852841814393));
#17815=CARTESIAN_POINT('Ctrl Pts',(-55.2655194584768,-103.908817732493,
177.870984653547));
#17816=CARTESIAN_POINT('Ctrl Pts',(-55.307878468054,-103.908471243195,177.926811129217));
#17817=CARTESIAN_POINT('Ctrl Pts',(-55.3384414676804,-103.907638988345,
177.963422725913));
#17818=CARTESIAN_POINT('Ctrl Pts',(-55.5016508194093,-103.900445816394,
178.141351970913));
#17819=CARTESIAN_POINT('Ctrl Pts',(-55.6580750812902,-103.884831359886,
178.257501037053));
#17820=CARTESIAN_POINT('Ctrl Pts',(-55.9934121427347,-103.839158416831,
178.418096294027));
#17821=CARTESIAN_POINT('Ctrl Pts',(-56.1670410556707,-103.810767352649,
178.465352870717));
#17822=CARTESIAN_POINT('Ctrl Pts',(-56.343987871522,-103.776928050381,178.480312727065));
#17823=CARTESIAN_POINT('',(-56.3053536374455,-103.40960168206,178.480661415526));
#17824=CARTESIAN_POINT('',(-56.343987871522,-103.776928050381,178.480312727066));
#17825=CARTESIAN_POINT('Ctrl Pts',(-56.3053536374462,-103.409601682063,
178.480661415514));
#17826=CARTESIAN_POINT('Ctrl Pts',(-56.1171541463156,-103.387986491668,
178.46583662156));
#17827=CARTESIAN_POINT('Ctrl Pts',(-55.9327747632696,-103.371412441811,
178.41693017353));
#17828=CARTESIAN_POINT('Ctrl Pts',(-55.5939279603077,-103.347098934845,
178.255178416131));
#17829=CARTESIAN_POINT('Ctrl Pts',(-55.4419403876366,-103.339145250376,
178.144919795626));
#17830=CARTESIAN_POINT('Ctrl Pts',(-55.280402017082,-103.332395517122,177.974063117867));
#17831=CARTESIAN_POINT('Ctrl Pts',(-55.2485609792392,-103.331193876366,
177.936905101778));
#17832=CARTESIAN_POINT('Ctrl Pts',(-55.1679090691248,-103.328475257935,
177.832858015124));
#17833=CARTESIAN_POINT('Ctrl Pts',(-55.1227396789694,-103.327318672735,
177.763371477236));
#17834=CARTESIAN_POINT('Ctrl Pts',(-55.024038606154,-103.325685197287,177.579627296491));
#17835=CARTESIAN_POINT('Ctrl Pts',(-54.9788266623195,-103.325876624763,
177.461694894587));
#17836=CARTESIAN_POINT('Ctrl Pts',(-54.9208912318742,-103.328342249097,
177.223551059475));
#17837=CARTESIAN_POINT('Ctrl Pts',(-54.9068282367496,-103.330498483767,
177.104719966844));
#17838=CARTESIAN_POINT('Ctrl Pts',(-54.9071900358704,-103.333580645004,
176.985485069079));
#17839=CARTESIAN_POINT('Origin',(-57.8503443722502,-102.190085871961,175.985485069079));
#17840=CARTESIAN_POINT('Ctrl Pts',(-60.4746144719253,-111.16289106757,178.485485069079));
#17841=CARTESIAN_POINT('Ctrl Pts',(-59.7173985122241,-111.170711378967,
178.985485106928));
#17842=CARTESIAN_POINT('Ctrl Pts',(-58.8107269732545,-111.198740106278,
178.985485069079));
#17843=CARTESIAN_POINT('Ctrl Pts',(-57.8942367159207,-111.227072368185,
178.985485030821));
#17844=CARTESIAN_POINT('Ctrl Pts',(-57.1318490822761,-111.234741954516,
178.475522296093));
#17845=CARTESIAN_POINT('Ctrl Pts',(-57.0927973172532,-110.86741985642,178.475593938758));
#17846=CARTESIAN_POINT('Ctrl Pts',(-57.8551481998615,-110.85974917265,178.985485030824));
#17847=CARTESIAN_POINT('Ctrl Pts',(-58.7715680984392,-110.831419085805,
178.985485069079));
#17848=CARTESIAN_POINT('Ctrl Pts',(-59.6782396374026,-110.803390358494,
178.985485106928));
#17849=CARTESIAN_POINT('Ctrl Pts',(-60.43545559711,-110.795570047097,178.485485069079));
#17850=CARTESIAN_POINT('Origin',(-57.8503443722502,-102.190085871961,175.985485069079));
#17851=CARTESIAN_POINT('Ctrl Pts',(-60.3156054652531,-109.671342833085,
178.485485069079));
#17852=CARTESIAN_POINT('Ctrl Pts',(-59.5583895055519,-109.679163144481,
178.985485106928));
#17853=CARTESIAN_POINT('Ctrl Pts',(-58.6517179665823,-109.707191871792,
178.985485069079));
#17854=CARTESIAN_POINT('Ctrl Pts',(-57.7356383282381,-109.735511439877,
178.985485030838));
#17855=CARTESIAN_POINT('Ctrl Pts',(-56.9734652393652,-109.7431874274,178.475940356875));
#17856=CARTESIAN_POINT('Ctrl Pts',(-56.9345361076167,-109.375864092667,
178.476093934548));
#17857=CARTESIAN_POINT('Ctrl Pts',(-57.6966303278291,-109.368185755292,
178.985485030845));
#17858=CARTESIAN_POINT('Ctrl Pts',(-58.612559091767,-109.339870851319,178.985485069079));
#17859=CARTESIAN_POINT('Ctrl Pts',(-59.5192306307304,-109.311842124008,
178.985485106928));
#17860=CARTESIAN_POINT('Ctrl Pts',(-60.2764465904377,-109.304021812611,
178.485485069079));
#17861=CARTESIAN_POINT('Origin',(-57.8503443722502,-102.190085871961,175.985485069079));
#17862=CARTESIAN_POINT('Ctrl Pts',(-60.1565964585809,-108.179794598599,
178.485485069079));
#17863=CARTESIAN_POINT('Ctrl Pts',(-59.3993804988796,-108.187614909996,
178.985485106928));
#17864=CARTESIAN_POINT('Ctrl Pts',(-58.4927089599101,-108.215643637307,
178.985485069079));
#17865=CARTESIAN_POINT('Ctrl Pts',(-57.5773563068175,-108.243940731463,
178.985485030869));
#17866=CARTESIAN_POINT('Ctrl Pts',(-56.8155634335305,-108.251628031083,
178.476680214078));
#17867=CARTESIAN_POINT('Ctrl Pts',(-56.7767448738943,-107.884303575429,
178.476907478761));
#17868=CARTESIAN_POINT('Ctrl Pts',(-57.5384208193584,-107.876612805222,
178.985485030878));
#17869=CARTESIAN_POINT('Ctrl Pts',(-58.4535500850947,-107.848322616834,
178.985485069079));
#17870=CARTESIAN_POINT('Ctrl Pts',(-59.3602216240582,-107.820293889523,
178.985485106928));
#17871=CARTESIAN_POINT('Ctrl Pts',(-60.1174375837655,-107.812473578126,
178.485485069079));
#17872=CARTESIAN_POINT('Origin',(-57.8503443722502,-102.190085871961,175.985485069079));
#17873=CARTESIAN_POINT('Ctrl Pts',(-59.9975874519086,-106.688246364113,
178.485485069079));
#17874=CARTESIAN_POINT('Ctrl Pts',(-59.2403714922074,-106.69606667551,178.985485106928));
#17875=CARTESIAN_POINT('Ctrl Pts',(-58.3336999532379,-106.724095402821,
178.985485069079));
#17876=CARTESIAN_POINT('Ctrl Pts',(-57.4193502102051,-106.752361493145,
178.98548503091));
#17877=CARTESIAN_POINT('Ctrl Pts',(-56.6580826427064,-106.760064354331,
178.477700244368));
#17878=CARTESIAN_POINT('Ctrl Pts',(-56.6193547970191,-106.392738970839,
178.477987698341));
#17879=CARTESIAN_POINT('Ctrl Pts',(-57.3804740961378,-106.385031731442,
178.985485030922));
#17880=CARTESIAN_POINT('Ctrl Pts',(-58.2945410784225,-106.356774382348,
178.985485069079));
#17881=CARTESIAN_POINT('Ctrl Pts',(-59.201212617386,-106.328745655037,178.985485106928));
#17882=CARTESIAN_POINT('Ctrl Pts',(-59.9584285770933,-106.32092534364,178.485485069079));
#17883=CARTESIAN_POINT('Origin',(-57.8503443722502,-102.190085871961,175.985485069079));
#17884=CARTESIAN_POINT('Ctrl Pts',(-59.8385784452364,-105.196698129628,
178.485485069079));
#17885=CARTESIAN_POINT('Ctrl Pts',(-59.0813624855352,-105.204518441025,
178.985485106928));
#17886=CARTESIAN_POINT('Ctrl Pts',(-58.1746909465656,-105.232547168336,
178.985485069079));
#17887=CARTESIAN_POINT('Ctrl Pts',(-57.2615592502346,-105.26077560412,178.985485030961));
#17888=CARTESIAN_POINT('Ctrl Pts',(-56.5009308898174,-105.268497296389,
178.478938088823));
#17889=CARTESIAN_POINT('Ctrl Pts',(-56.462266632785,-104.901171252502,178.479267413548));
#17890=CARTESIAN_POINT('Ctrl Pts',(-57.2227246142167,-104.89344456017,178.985485030975));
#17891=CARTESIAN_POINT('Ctrl Pts',(-58.1355320717503,-104.865226147862,
178.985485069079));
#17892=CARTESIAN_POINT('Ctrl Pts',(-59.0422036107137,-104.837197420552,
178.985485106928));
#17893=CARTESIAN_POINT('Ctrl Pts',(-59.7994195704211,-104.829377109155,
178.485485069079));
#17894=CARTESIAN_POINT('Origin',(-57.8503443722502,-102.190085871961,175.985485069079));
#17895=CARTESIAN_POINT('Ctrl Pts',(-59.6795694385642,-103.705149895142,
178.485485069079));
#17896=CARTESIAN_POINT('Ctrl Pts',(-58.922353478863,-103.712970206539,178.985485106928));
#17897=CARTESIAN_POINT('Ctrl Pts',(-58.0156819398934,-103.74099893385,178.985485069079));
#17898=CARTESIAN_POINT('Ctrl Pts',(-57.1039041585715,-103.76918551488,178.985485031018));
#17899=CARTESIAN_POINT('Ctrl Pts',(-56.343987871522,-103.776928050381,178.480312727066));
#17900=CARTESIAN_POINT('Ctrl Pts',(-56.3053536374455,-103.40960168206,178.480661415526));
#17901=CARTESIAN_POINT('Ctrl Pts',(-57.0650889275684,-103.401853871046,
178.985485031032));
#17902=CARTESIAN_POINT('Ctrl Pts',(-57.9765230650781,-103.373677913377,
178.985485069079));
#17903=CARTESIAN_POINT('Ctrl Pts',(-58.8831946040415,-103.345649186066,
178.985485106928));
#17904=CARTESIAN_POINT('Ctrl Pts',(-59.6404105637488,-103.337828874669,
178.485485069079));
#17905=CARTESIAN_POINT('Origin',(-57.8503443722502,-102.190085871961,175.985485069079));
#17906=CARTESIAN_POINT('',(-57.1028900759218,-102.269769493613,178.889785775842));
#17907=CARTESIAN_POINT('Ctrl Pts',(-59.5205604318919,-102.213601660657,
178.485485069079));
#17908=CARTESIAN_POINT('Ctrl Pts',(-58.7633444721907,-102.221421972053,
178.985485106928));
#17909=CARTESIAN_POINT('Ctrl Pts',(-57.8566729332212,-102.249450699364,
178.985485069079));
#17910=CARTESIAN_POINT('Ctrl Pts',(-57.4738337760053,-102.261285739818,
178.985485053098));
#17911=CARTESIAN_POINT('Ctrl Pts',(-57.1028900759218,-102.269769493613,
178.889785775842));
#17912=CARTESIAN_POINT('Origin',(-57.8503443722502,-102.190085871961,175.985485069079));
#17913=CARTESIAN_POINT('Origin',(-57.8503443722502,-102.190085871961,175.985485069079));
#17914=CARTESIAN_POINT('Ctrl Pts',(-53.872882413622,-102.614109889754,175.985485078249));
#17915=CARTESIAN_POINT('Ctrl Pts',(-53.9451038903198,-102.606410597834,
176.390205984865));
#17916=CARTESIAN_POINT('Ctrl Pts',(-54.0841826712686,-102.591583870614,
176.77982118409));
#17917=CARTESIAN_POINT('Ctrl Pts',(-54.4695645888159,-102.550499583507,
177.466598590891));
#17918=CARTESIAN_POINT('Ctrl Pts',(-54.7036701793867,-102.525542363518,
177.764282984435));
#17919=CARTESIAN_POINT('Ctrl Pts',(-55.2319645793612,-102.469222651002,
178.254741908794));
#17920=CARTESIAN_POINT('Ctrl Pts',(-55.5765915421303,-102.432483114354,
178.512021649406));
#17921=CARTESIAN_POINT('Ctrl Pts',(-56.3676195021526,-102.348154249042,
178.819447246742));
#17922=CARTESIAN_POINT('Ctrl Pts',(-56.7334438797843,-102.309154926352,
178.888970429676));
#17923=CARTESIAN_POINT('Ctrl Pts',(-57.1028900759218,-102.269769493613,
178.889785775842));
#17924=CARTESIAN_POINT('Ctrl Pts',(-51.366074883876,-77.3517457257593,176.985485069079));
#17925=CARTESIAN_POINT('Ctrl Pts',(-51.366074883876,-77.3517457257593,174.585485069075));
#17926=CARTESIAN_POINT('Ctrl Pts',(-48.8928953354189,-61.7130539582536,
176.985485069079));
#17927=CARTESIAN_POINT('Ctrl Pts',(-48.8928953354189,-61.7130539582536,
174.585485069075));
#17928=CARTESIAN_POINT('Ctrl Pts',(-46.2601081177707,-49.5877530345566,
176.985485069079));
#17929=CARTESIAN_POINT('Ctrl Pts',(-46.2601081177707,-49.5877530345566,
174.585485069075));
#17930=CARTESIAN_POINT('Ctrl Pts',(-40.9615423766251,-29.8520086479652,
176.985485069079));
#17931=CARTESIAN_POINT('Ctrl Pts',(-40.9615423766251,-29.8520086479652,
174.585485069075));
#17932=CARTESIAN_POINT('Ctrl Pts',(-38.2937855838775,-22.2407276361426,
176.985485069079));
#17933=CARTESIAN_POINT('Ctrl Pts',(-38.2937855838775,-22.2407276361426,
174.585485069075));
#17934=CARTESIAN_POINT('Ctrl Pts',(-34.518838241635,-12.3909742448081,176.985485069079));
#17935=CARTESIAN_POINT('Ctrl Pts',(-34.518838241635,-12.3909742448081,174.585485069075));
#17936=CARTESIAN_POINT('Ctrl Pts',(-33.2992245946195,-9.36991678274843,
176.985485069079));
#17937=CARTESIAN_POINT('Ctrl Pts',(-33.2992245946195,-9.36991678274843,
174.585485069075));
#17938=CARTESIAN_POINT('Ctrl Pts',(-30.9798899307116,-3.54783868987816,
176.985485069079));
#17939=CARTESIAN_POINT('Ctrl Pts',(-30.9798899307116,-3.54783868987816,
174.585485069075));
#17940=CARTESIAN_POINT('Ctrl Pts',(-29.8803502640751,-0.747159372776982,
176.985485069079));
#17941=CARTESIAN_POINT('Ctrl Pts',(-29.8803502640751,-0.747159372776982,
174.585485069075));
#17942=CARTESIAN_POINT('Ctrl Pts',(-26.8076803368812,7.8043162165179,176.985485069079));
#17943=CARTESIAN_POINT('Ctrl Pts',(-26.8076803368812,7.8043162165179,174.585485069075));
#17944=CARTESIAN_POINT('Ctrl Pts',(-25.0550914662622,13.705075012501,176.985485069079));
#17945=CARTESIAN_POINT('Ctrl Pts',(-25.0550914662622,13.705075012501,174.585485069075));
#17946=CARTESIAN_POINT('Ctrl Pts',(-23.70581036359,21.1602846666598,176.985485069079));
#17947=CARTESIAN_POINT('Ctrl Pts',(-23.70581036359,21.1602846666598,174.585485069075));
#17948=CARTESIAN_POINT('',(-23.7058173975717,21.1602848469763,176.985485069079));
#17949=CARTESIAN_POINT('Ctrl Pts',(-23.7058173975717,21.1602848469763,176.985485069079));
#17950=CARTESIAN_POINT('Ctrl Pts',(-24.0609786331059,19.1981320867072,176.985485069079));
#17951=CARTESIAN_POINT('Ctrl Pts',(-24.4622947014093,17.2457191252609,176.985485069079));
#17952=CARTESIAN_POINT('Ctrl Pts',(-24.915822344951,15.30429507165,176.985485069079));
#17953=CARTESIAN_POINT('Ctrl Pts',(-24.9867712230002,15.0005829156591,176.985485069079));
#17954=CARTESIAN_POINT('Ctrl Pts',(-25.0589937084744,14.6971400997934,176.985485069079));
#17955=CARTESIAN_POINT('Ctrl Pts',(-25.1324952265289,14.3939806501629,176.985485069079));
#17956=CARTESIAN_POINT('Ctrl Pts',(-25.3191212342609,13.6242354899502,176.985485069079));
#17957=CARTESIAN_POINT('Ctrl Pts',(-25.5139981706041,12.8562891283856,176.985485069079));
#17958=CARTESIAN_POINT('Ctrl Pts',(-25.7172982514514,12.0900656566086,176.985485069079));
#17959=CARTESIAN_POINT('Ctrl Pts',(-25.977816914546,11.1081894386201,176.985485069079));
#17960=CARTESIAN_POINT('Ctrl Pts',(-26.2524109786123,10.1283936032505,176.985485069079));
#17961=CARTESIAN_POINT('Ctrl Pts',(-26.5400675250715,9.15302099692352,176.985485069079));
#17962=CARTESIAN_POINT('Ctrl Pts',(-26.5655456245349,9.06663102741372,176.985485069079));
#17963=CARTESIAN_POINT('Ctrl Pts',(-26.5911262304682,8.98027576367801,176.985485069079));
#17964=CARTESIAN_POINT('Ctrl Pts',(-26.6168086578218,8.89395683843848,176.985485069079));
#17965=CARTESIAN_POINT('Ctrl Pts',(-26.6778123577222,8.68892272158753,176.985485069079));
#17966=CARTESIAN_POINT('Ctrl Pts',(-26.7393942284263,8.48411023451817,176.985485069079));
#17967=CARTESIAN_POINT('Ctrl Pts',(-26.801542811029,8.27950502525835,176.985485069079));
#17968=CARTESIAN_POINT('Ctrl Pts',(-27.106086550375,7.27688786315808,176.985485069079));
#17969=CARTESIAN_POINT('Ctrl Pts',(-27.4242172429184,6.27931159291589,176.985485069079));
#17970=CARTESIAN_POINT('Ctrl Pts',(-27.7542866099677,5.2861618395196,176.985485069079));
#17971=CARTESIAN_POINT('Ctrl Pts',(-27.9852612027692,4.59117956372655,176.985485069079));
#17972=CARTESIAN_POINT('Ctrl Pts',(-28.2220826504089,3.89836521129347,176.985485069079));
#17973=CARTESIAN_POINT('Ctrl Pts',(-28.4641913869893,3.20751217561695,176.985485069079));
#17974=CARTESIAN_POINT('Ctrl Pts',(-28.5351702186733,3.00497532366267,176.985485069079));
#17975=CARTESIAN_POINT('Ctrl Pts',(-28.6066033326334,2.80260753664105,176.985485069079));
#17976=CARTESIAN_POINT('Ctrl Pts',(-28.6784772662389,2.6004019699,176.985485069079));
#17977=CARTESIAN_POINT('Ctrl Pts',(-29.0461821574925,1.56592434776952,176.985485069079));
#17978=CARTESIAN_POINT('Ctrl Pts',(-29.4252407716952,0.535662626378677,
176.985485069079));
#17979=CARTESIAN_POINT('Ctrl Pts',(-29.8124487382319,-0.491577100740066,
176.985485069079));
#17980=CARTESIAN_POINT('Ctrl Pts',(-30.107037119717,-1.27310257222217,176.985485069079));
#17981=CARTESIAN_POINT('Ctrl Pts',(-30.4063418212305,-2.05287902408378,
176.985485069079));
#17982=CARTESIAN_POINT('Ctrl Pts',(-30.7089334673433,-2.83143712039792,
176.985485069079));
#17983=CARTESIAN_POINT('Ctrl Pts',(-30.8040693059046,-3.07621842322983,
176.985485069079));
#17984=CARTESIAN_POINT('Ctrl Pts',(-30.8995300442216,-3.32087962702539,
176.985485069079));
#17985=CARTESIAN_POINT('Ctrl Pts',(-30.995270588929,-3.56543656328317,176.985485069079));
#17986=CARTESIAN_POINT('Ctrl Pts',(-31.3932109940057,-4.58192426529273,
176.985485069079));
#17987=CARTESIAN_POINT('Ctrl Pts',(-31.7957954668658,-5.59669181926987,
176.985485069079));
#17988=CARTESIAN_POINT('Ctrl Pts',(-32.1999884451959,-6.61086118226492,
176.985485069079));
#17989=CARTESIAN_POINT('Ctrl Pts',(-32.5227346634746,-7.42067071421904,
176.985485069079));
#17990=CARTESIAN_POINT('Ctrl Pts',(-32.8465051550323,-8.23009945981376,
176.985485069079));
#17991=CARTESIAN_POINT('Ctrl Pts',(-33.1697310400329,-9.03972997500453,
176.985485069079));
#17992=CARTESIAN_POINT('Ctrl Pts',(-33.2512988465853,-9.24404463019352,
176.985485069079));
#17993=CARTESIAN_POINT('Ctrl Pts',(-33.3328318656186,-9.44837214946192,
176.985485069079));
#17994=CARTESIAN_POINT('Ctrl Pts',(-33.4143043110506,-9.65272099823434,
176.985485069079));
#17995=CARTESIAN_POINT('Ctrl Pts',(-33.9541840790767,-11.0068451869285,
176.985485069079));
#17996=CARTESIAN_POINT('Ctrl Pts',(-34.4913531539213,-12.3619920566898,
176.985485069079));
#17997=CARTESIAN_POINT('Ctrl Pts',(-35.0211191261436,-13.719879020288,176.985485069079));
#17998=CARTESIAN_POINT('Ctrl Pts',(-35.2812503229336,-14.3866427980076,
176.985485069079));
#17999=CARTESIAN_POINT('Ctrl Pts',(-35.5395970138749,-15.0540710424698,
176.985485069079));
#18000=CARTESIAN_POINT('Ctrl Pts',(-35.7955956003909,-15.7223555157655,
176.985485069079));
#18001=CARTESIAN_POINT('Ctrl Pts',(-36.1833029487603,-16.7344657958424,
176.985485069079));
#18002=CARTESIAN_POINT('Ctrl Pts',(-36.5657733621123,-17.7488150534779,
176.985485069079));
#18003=CARTESIAN_POINT('Ctrl Pts',(-36.9419659969045,-18.7652067279702,
176.985485069079));
#18004=CARTESIAN_POINT('Ctrl Pts',(-37.1160044343593,-19.2354211939403,
176.985485069079));
#18005=CARTESIAN_POINT('Ctrl Pts',(-37.2886992867772,-19.7060727594894,
176.985485069079));
#18006=CARTESIAN_POINT('Ctrl Pts',(-37.4599477597535,-20.177141788797,176.985485069079));
#18007=CARTESIAN_POINT('Ctrl Pts',(-37.6325033302003,-20.6518063721319,
176.985485069079));
#18008=CARTESIAN_POINT('Ctrl Pts',(-37.8035923350539,-21.1269004506383,
176.985485069079));
#18009=CARTESIAN_POINT('Ctrl Pts',(-37.9731001370556,-21.6023762842089,
176.985485069079));
#18010=CARTESIAN_POINT('Ctrl Pts',(-37.9989925350158,-21.6750054455681,
176.985485069079));
#18011=CARTESIAN_POINT('Ctrl Pts',(-38.0248480785516,-21.7476436183096,
176.985485069079));
#18012=CARTESIAN_POINT('Ctrl Pts',(-38.0506664067205,-21.8202907608508,
176.985485069079));
#18013=CARTESIAN_POINT('Ctrl Pts',(-38.4931055792047,-23.0652180628431,
176.985485069079));
#18014=CARTESIAN_POINT('Ctrl Pts',(-38.9246977909074,-24.3127099825977,
176.985485069079));
#18015=CARTESIAN_POINT('Ctrl Pts',(-39.3451931578191,-25.5628721161241,
176.985485069079));
#18016=CARTESIAN_POINT('Ctrl Pts',(-39.5292547595282,-26.1101001305087,
176.985485069079));
#18017=CARTESIAN_POINT('Ctrl Pts',(-39.711191090252,-26.6578421174245,176.985485069079));
#18018=CARTESIAN_POINT('Ctrl Pts',(-39.8909793753221,-27.206099092718,176.985485069079));
#18019=CARTESIAN_POINT('Ctrl Pts',(-39.9730744745014,-27.4564447186574,
176.985485069079));
#18020=CARTESIAN_POINT('Ctrl Pts',(-40.0547213113963,-27.7068964984478,
176.985485069079));
#18021=CARTESIAN_POINT('Ctrl Pts',(-40.1359182742855,-27.9574560644933,
176.985485069079));
#18022=CARTESIAN_POINT('Ctrl Pts',(-40.8013599420204,-30.01089217298,176.985485069079));
#18023=CARTESIAN_POINT('Ctrl Pts',(-41.4364827421166,-32.0716508915739,
176.985485069079));
#18024=CARTESIAN_POINT('Ctrl Pts',(-42.0434667820996,-34.1391767207459,
176.985485069079));
#18025=CARTESIAN_POINT('Ctrl Pts',(-42.4136817475693,-35.4002131781069,
176.985485069079));
#18026=CARTESIAN_POINT('Ctrl Pts',(-42.7734294290581,-36.663766907072,176.985485069079));
#18027=CARTESIAN_POINT('Ctrl Pts',(-43.123209233354,-37.9297105093382,176.985485069079));
#18028=CARTESIAN_POINT('Ctrl Pts',(-43.346909105782,-38.7393382204009,176.985485069079));
#18029=CARTESIAN_POINT('Ctrl Pts',(-43.5665312274966,-39.5499404131169,
176.985485069079));
#18030=CARTESIAN_POINT('Ctrl Pts',(-43.7822103601003,-40.3614968011214,
176.985485069079));
#18031=CARTESIAN_POINT('Ctrl Pts',(-44.519585351179,-43.1360878203846,176.985485069079));
#18032=CARTESIAN_POINT('Ctrl Pts',(-45.211388601689,-45.9216172075444,176.985485069079));
#18033=CARTESIAN_POINT('Ctrl Pts',(-45.8641427980324,-48.7165333394889,
176.985485069079));
#18034=CARTESIAN_POINT('Ctrl Pts',(-46.1914364418981,-50.1179158051206,
176.985485069079));
#18035=CARTESIAN_POINT('Ctrl Pts',(-46.5089121176543,-51.5216577766851,
176.985485069079));
#18036=CARTESIAN_POINT('Ctrl Pts',(-46.8173885348151,-52.9275664406215,
176.985485069079));
#18037=CARTESIAN_POINT('Ctrl Pts',(-47.4870367014129,-55.9795474246911,
176.985485069079));
#18038=CARTESIAN_POINT('Ctrl Pts',(-48.114346647767,-59.0416984673988,176.985485069079));
#18039=CARTESIAN_POINT('Ctrl Pts',(-48.7060174445671,-62.1124135687292,
176.985485069079));
#18040=CARTESIAN_POINT('Ctrl Pts',(-48.9313936321896,-63.2820945240097,
176.985485069079));
#18041=CARTESIAN_POINT('Ctrl Pts',(-49.1515981816455,-64.4530182376069,
176.985485069079));
#18042=CARTESIAN_POINT('Ctrl Pts',(-49.3669995999362,-65.6250971770435,
176.985485069079));
#18043=CARTESIAN_POINT('Ctrl Pts',(-50.0153496236315,-69.1530099186912,
176.985485069079));
#18044=CARTESIAN_POINT('Ctrl Pts',(-50.6201441923267,-72.6913972594903,
176.985485069162));
#18045=CARTESIAN_POINT('Ctrl Pts',(-51.1888177613378,-76.2384559838746,
176.985485069122));
#18046=CARTESIAN_POINT('',(-23.70581036359,21.1602846666598,174.985485069079));
#18047=CARTESIAN_POINT('',(-23.70581036359,21.1602846666598,175.985485069079));
#18048=CARTESIAN_POINT('Ctrl Pts',(-51.1887931847522,-76.2384284136363,
174.985485069079));
#18049=CARTESIAN_POINT('Ctrl Pts',(-50.5213346265716,-72.0755903721384,
174.985485069079));
#18050=CARTESIAN_POINT('Ctrl Pts',(-49.8042721930313,-67.9239395141956,
174.985485069079));
#18051=CARTESIAN_POINT('Ctrl Pts',(-48.2454967538896,-59.6487390071956,
174.985485069079));
#18052=CARTESIAN_POINT('Ctrl Pts',(-47.4038384436995,-55.5251770226586,
174.985485069079));
#18053=CARTESIAN_POINT('Ctrl Pts',(-45.5617895517713,-47.3138520117311,
174.985485069079));
#18054=CARTESIAN_POINT('Ctrl Pts',(-44.5612309815417,-43.2261268718582,
174.985485069079));
#18055=CARTESIAN_POINT('Ctrl Pts',(-42.3590336034264,-35.0960263054489,
174.985485069079));
#18056=CARTESIAN_POINT('Ctrl Pts',(-41.1560792064761,-31.0539475842857,
174.985485069079));
#18057=CARTESIAN_POINT('Ctrl Pts',(-39.1758099410217,-25.0304862486367,
174.985485069079));
#18058=CARTESIAN_POINT('Ctrl Pts',(-38.486561950554,-23.0292418728959,174.985485069079));
#18059=CARTESIAN_POINT('Ctrl Pts',(-37.0529631635479,-19.039180481201,174.985485069079));
#18060=CARTESIAN_POINT('Ctrl Pts',(-36.3087744035167,-17.0515279744533,
174.985485069079));
#18061=CARTESIAN_POINT('Ctrl Pts',(-34.7825960540618,-13.0925681835044,
174.985485069079));
#18062=CARTESIAN_POINT('Ctrl Pts',(-34.0001212951122,-11.1203014222748,
174.985485069079));
#18063=CARTESIAN_POINT('Ctrl Pts',(-32.4270421820337,-7.17879282084528,
174.985485069079));
#18064=CARTESIAN_POINT('Ctrl Pts',(-31.6366800593758,-5.20946084933443,
174.985485069079));
#18065=CARTESIAN_POINT('Ctrl Pts',(-30.0940103202672,-1.25663729890807,
174.985485069079));
#18066=CARTESIAN_POINT('Ctrl Pts',(-29.342391793721,0.727110681771283,174.985485069079));
#18067=CARTESIAN_POINT('Ctrl Pts',(-27.9248341481098,4.7264868826472,174.985485069079));
#18068=CARTESIAN_POINT('Ctrl Pts',(-27.2593908283077,6.74229958356928,174.985485069079));
#18069=CARTESIAN_POINT('Ctrl Pts',(-26.0425659871153,10.8163659588052,174.985485069079));
#18070=CARTESIAN_POINT('Ctrl Pts',(-25.4928841138196,12.8686487455774,174.985485069079));
#18071=CARTESIAN_POINT('Ctrl Pts',(-24.5138232792971,16.9962588567196,174.985485069079));
#18072=CARTESIAN_POINT('Ctrl Pts',(-24.0836324787232,19.072696737701,174.985485069079));
#18073=CARTESIAN_POINT('Ctrl Pts',(-23.7058105558977,21.1602836040985,174.985485069079));
#18074=CARTESIAN_POINT('Ctrl Pts',(-53.0167365461859,-78.193620158077,173.485485069079));
#18075=CARTESIAN_POINT('Ctrl Pts',(-51.5346787297268,-78.4249308337329,
173.485485069079));
#18076=CARTESIAN_POINT('Ctrl Pts',(-51.5346787297268,-78.4249308337329,
174.985485069079));
#18077=CARTESIAN_POINT('Ctrl Pts',(-52.3478408594839,-73.9078599867829,
173.485485069079));
#18078=CARTESIAN_POINT('Ctrl Pts',(-50.8676276544628,-74.1509894892529,
173.485485069079));
#18079=CARTESIAN_POINT('Ctrl Pts',(-50.8676276544411,-74.150989489256,174.985485069079));
#18080=CARTESIAN_POINT('Ctrl Pts',(-51.6285617065834,-69.6334497110788,
173.485485069079));
#18081=CARTESIAN_POINT('Ctrl Pts',(-50.1505302305787,-69.8896731372056,
173.485485069079));
#18082=CARTESIAN_POINT('Ctrl Pts',(-50.150530230561,-69.8896731372089,174.985485069079));
#18083=CARTESIAN_POINT('Ctrl Pts',(-50.0631495457321,-61.113268493176,173.485485069079));
#18084=CARTESIAN_POINT('Ctrl Pts',(-48.5905691191417,-61.3991607376064,
173.485485069079));
#18085=CARTESIAN_POINT('Ctrl Pts',(-48.5905691191594,-61.3991607376031,
174.985485069079));
#18086=CARTESIAN_POINT('Ctrl Pts',(-49.2170840953273,-56.8674733632373,
173.485485069079));
#18087=CARTESIAN_POINT('Ctrl Pts',(-47.7477702624369,-57.16994536236,173.485485069079));
#18088=CARTESIAN_POINT('Ctrl Pts',(-47.7477702623948,-57.1699453623542,
174.985485069079));
#18089=CARTESIAN_POINT('Ctrl Pts',(-47.3628470711911,-48.4124583507524,
173.485485069079));
#18090=CARTESIAN_POINT('Ctrl Pts',(-45.9018015025242,-48.7526322710164,
173.485485069079));
#18091=CARTESIAN_POINT('Ctrl Pts',(-45.9018015025663,-48.7526322710222,
174.985485069079));
#18092=CARTESIAN_POINT('Ctrl Pts',(-46.3545427330907,-44.2032684234675,
173.485485069079));
#18093=CARTESIAN_POINT('Ctrl Pts',(-44.8985120597276,-44.5646201418261,
173.485485069079));
#18094=CARTESIAN_POINT('Ctrl Pts',(-44.8985120596695,-44.5646201418415,
174.985485069079));
#18095=CARTESIAN_POINT('Ctrl Pts',(-44.1311171174038,-35.8315517093622,
173.485485069079));
#18096=CARTESIAN_POINT('Ctrl Pts',(-42.6876656315475,-36.2402670065083,
173.485485069079));
#18097=CARTESIAN_POINT('Ctrl Pts',(-42.6876656316057,-36.2402670064929,
174.985485069079));
#18098=CARTESIAN_POINT('Ctrl Pts',(-42.9147512260831,-31.6693057388972,
173.485485069079));
#18099=CARTESIAN_POINT('Ctrl Pts',(-41.4789698205316,-32.1044366637925,
173.485485069079));
#18100=CARTESIAN_POINT('Ctrl Pts',(-41.4789698205142,-32.1044366638057,
174.985485069079));
#18101=CARTESIAN_POINT('Ctrl Pts',(-40.906208719954,-25.467450415631,173.485485069079));
#18102=CARTESIAN_POINT('Ctrl Pts',(-39.4835575759942,-25.9431241632503,
173.485485069079));
#18103=CARTESIAN_POINT('Ctrl Pts',(-39.4835575760029,-25.9431241632437,
174.985485069079));
#18104=CARTESIAN_POINT('Ctrl Pts',(-40.206142545412,-23.4070586143658,173.485485069079));
#18105=CARTESIAN_POINT('Ctrl Pts',(-38.7881219432854,-23.8963460449173,
173.485485069079));
#18106=CARTESIAN_POINT('Ctrl Pts',(-38.7881219432977,-23.8963460449054,
174.985485069079));
#18107=CARTESIAN_POINT('Ctrl Pts',(-38.7470879355323,-19.2995693663361,
173.485485069079));
#18108=CARTESIAN_POINT('Ctrl Pts',(-37.3381634907308,-19.8144640416042,
173.485485069079));
#18109=CARTESIAN_POINT('Ctrl Pts',(-37.3381634907185,-19.8144640416161,
174.985485069079));
#18110=CARTESIAN_POINT('Ctrl Pts',(-37.9878548350367,-17.2526269837786,
173.485485069079));
#18111=CARTESIAN_POINT('Ctrl Pts',(-36.5834023703057,-17.7795215046325,
173.485485069079));
#18112=CARTESIAN_POINT('Ctrl Pts',(-36.5834023703931,-17.7795215045991,
174.985485069079));
#18113=CARTESIAN_POINT('Ctrl Pts',(-36.4271652313825,-13.1772568450141,
173.485485069079));
#18114=CARTESIAN_POINT('Ctrl Pts',(-35.0300266743469,-13.7232498983064,
173.485485069079));
#18115=CARTESIAN_POINT('Ctrl Pts',(-35.0300266742596,-13.7232498983399,
174.985485069079));
#18116=CARTESIAN_POINT('Ctrl Pts',(-35.6251003133685,-11.1476565297151,
173.485485069079));
#18117=CARTESIAN_POINT('Ctrl Pts',(-34.2307808988101,-11.7007208831933,
173.485485069079));
#18118=CARTESIAN_POINT('Ctrl Pts',(-34.2307808989649,-11.7007208831316,
174.985485069079));
#18119=CARTESIAN_POINT('Ctrl Pts',(-34.008647106654,-7.09304295664572,173.485485069079));
#18120=CARTESIAN_POINT('Ctrl Pts',(-32.6162603377718,-7.65095504179,173.485485069079));
#18121=CARTESIAN_POINT('Ctrl Pts',(-32.616260337617,-7.65095504185172,174.985485069079));
#18122=CARTESIAN_POINT('Ctrl Pts',(-33.1944598949962,-5.06795485306577,
173.485485069079));
#18123=CARTESIAN_POINT('Ctrl Pts',(-31.8011075370691,-5.62352303603581,
173.485485069079));
#18124=CARTESIAN_POINT('Ctrl Pts',(-31.8011075372865,-5.62352303595069,
174.985485069079));
#18125=CARTESIAN_POINT('Ctrl Pts',(-31.6032144550666,-1.00395833775079,
173.485485069079));
#18126=CARTESIAN_POINT('Ctrl Pts',(-30.2030685122845,-1.54217589428156,
173.485485069079));
#18127=CARTESIAN_POINT('Ctrl Pts',(-30.2030685120672,-1.54217589436668,
174.985485069079));
#18128=CARTESIAN_POINT('Ctrl Pts',(-30.8269429206595,1.03524290056039,173.485485069079));
#18129=CARTESIAN_POINT('Ctrl Pts',(-29.420943080133,0.512133922373698,173.485485069079));
#18130=CARTESIAN_POINT('Ctrl Pts',(-29.4209430803042,0.512133922435039,
174.985485069079));
#18131=CARTESIAN_POINT('Ctrl Pts',(-29.364921121899,5.14733958959975,173.485485069079));
#18132=CARTESIAN_POINT('Ctrl Pts',(-27.9442645188942,4.66545436370176,173.485485069079));
#18133=CARTESIAN_POINT('Ctrl Pts',(-27.944264518723,4.66545436364042,174.985485069079));
#18134=CARTESIAN_POINT('Ctrl Pts',(-28.6798159809479,7.22047517089018,173.485485069079));
#18135=CARTESIAN_POINT('Ctrl Pts',(-27.2504765600523,6.76457334823395,173.485485069079));
#18136=CARTESIAN_POINT('Ctrl Pts',(-27.2504765601174,6.76457334825143,174.985485069079));
#18137=CARTESIAN_POINT('Ctrl Pts',(-27.4323595727382,11.4124383027362,173.485485069079));
#18138=CARTESIAN_POINT('Ctrl Pts',(-25.9863143172519,11.0126749088339,173.485485069079));
#18139=CARTESIAN_POINT('Ctrl Pts',(-25.9863143171867,11.0126749088164,174.985485069079));
#18140=CARTESIAN_POINT('Ctrl Pts',(-26.872482605583,13.5225670882055,173.485485069079));
#18141=CARTESIAN_POINT('Ctrl Pts',(-25.418512449069,13.1526523639037,173.485485069079));
#18142=CARTESIAN_POINT('Ctrl Pts',(-25.4185124490178,13.1526523638918,174.985485069079));
#18143=CARTESIAN_POINT('Ctrl Pts',(-25.8817163327183,17.7633008300245,173.485485069079));
#18144=CARTESIAN_POINT('Ctrl Pts',(-24.4143553121838,17.4507024379655,173.485485069079));
#18145=CARTESIAN_POINT('Ctrl Pts',(-24.414355312235,17.4507024379774,174.985485069079));
#18146=CARTESIAN_POINT('Ctrl Pts',(-25.4498962389785,19.8950365279689,173.485485069079));
#18147=CARTESIAN_POINT('Ctrl Pts',(-23.9770093214825,19.6099821711675,173.485485069079));
#18148=CARTESIAN_POINT('Ctrl Pts',(-23.9770093216439,19.6099821711937,174.985485069079));
#18149=CARTESIAN_POINT('Ctrl Pts',(-25.0731194387121,22.0366182599054,173.485485069079));
#18150=CARTESIAN_POINT('Ctrl Pts',(-23.595808607555,21.7767092216907,173.485485069079));
#18151=CARTESIAN_POINT('Ctrl Pts',(-23.595808607555,21.7767092216907,174.985485069079));
#18152=CARTESIAN_POINT('',(-25.2666963042962,20.9635176568293,173.485485069079));
#18153=CARTESIAN_POINT('Ctrl Pts',(-25.2666963042962,20.9635176568293,173.485485069184));
#18154=CARTESIAN_POINT('Ctrl Pts',(-25.5390668113124,19.4904292891436,173.485485069662));
#18155=CARTESIAN_POINT('Ctrl Pts',(-25.8381519757544,18.0230368201297,173.485485069241));
#18156=CARTESIAN_POINT('Ctrl Pts',(-26.1664788972763,16.5619707154367,173.485485069193));
#18157=CARTESIAN_POINT('Ctrl Pts',(-26.2353834496847,16.2553430849141,173.485485069182));
#18158=CARTESIAN_POINT('Ctrl Pts',(-26.3055757539796,15.9489940033786,173.485485069186));
#18159=CARTESIAN_POINT('Ctrl Pts',(-26.3770789088467,15.6429291555935,173.485485069228));
#18160=CARTESIAN_POINT('Ctrl Pts',(-26.3900846439141,15.5872589081597,173.485485069236));
#18161=CARTESIAN_POINT('Ctrl Pts',(-26.4031343886611,15.5315972847617,173.485485069245));
#18162=CARTESIAN_POINT('Ctrl Pts',(-26.4162281158535,15.4759443627374,173.485485069255));
#18163=CARTESIAN_POINT('Ctrl Pts',(-26.6573637297862,14.4510336308838,173.485485069454));
#18164=CARTESIAN_POINT('Ctrl Pts',(-26.9133448526214,13.4293094309892,173.48548507148));
#18165=CARTESIAN_POINT('Ctrl Pts',(-27.1842247243902,12.4107800921172,173.485485073504));
#18166=CARTESIAN_POINT('Ctrl Pts',(-27.3942455790166,11.6210853805271,173.485485075074));
#18167=CARTESIAN_POINT('Ctrl Pts',(-27.6132236088869,10.8333114203593,173.485485075017));
#18168=CARTESIAN_POINT('Ctrl Pts',(-27.8412042451402,10.0474684120255,173.485485072249));
#18169=CARTESIAN_POINT('Ctrl Pts',(-27.9119589207625,9.80357898326325,173.48548507139));
#18170=CARTESIAN_POINT('Ctrl Pts',(-27.9835604982678,9.55990044821291,173.485485071169));
#18171=CARTESIAN_POINT('Ctrl Pts',(-28.056011326395,9.31643398646967,173.4854850712));
#18172=CARTESIAN_POINT('Ctrl Pts',(-28.3631180387437,8.28442115009738,173.485485071334));
#18173=CARTESIAN_POINT('Ctrl Pts',(-28.684880487986,7.25832458735522,173.485485080559));
#18174=CARTESIAN_POINT('Ctrl Pts',(-29.0197368390196,6.23709829128275,173.485485084382));
#18175=CARTESIAN_POINT('Ctrl Pts',(-29.1887218714363,5.72173712756616,173.485485086311));
#18176=CARTESIAN_POINT('Ctrl Pts',(-29.3610422350258,5.20761689664156,173.485485084578));
#18177=CARTESIAN_POINT('Ctrl Pts',(-29.536500843974,4.69460639756019,173.485485078889));
#18178=CARTESIAN_POINT('Ctrl Pts',(-29.7197047622074,4.15894995932641,173.48548507295));
#18179=CARTESIAN_POINT('Ctrl Pts',(-29.9062419246547,3.62453460775134,173.485485071986));
#18180=CARTESIAN_POINT('Ctrl Pts',(-30.0958541508489,3.09126355889583,173.485485071356));
#18181=CARTESIAN_POINT('Ctrl Pts',(-30.5325765715419,1.86301246973321,173.485485069905));
#18182=CARTESIAN_POINT('Ctrl Pts',(-30.9853820483243,0.640745301943924,
173.485485072493));
#18183=CARTESIAN_POINT('Ctrl Pts',(-31.4488862792226,-0.577537461199393,
173.485485071091));
#18184=CARTESIAN_POINT('Ctrl Pts',(-31.7612655378603,-1.39860065974716,
173.485485070145));
#18185=CARTESIAN_POINT('Ctrl Pts',(-32.0784620377525,-2.2178705925264,173.485485069987));
#18186=CARTESIAN_POINT('Ctrl Pts',(-32.3987898977171,-3.0359751066965,173.485485069939));
#18187=CARTESIAN_POINT('Ctrl Pts',(-33.1944157816222,-5.06797172193035,
173.485485069819));
#18188=CARTESIAN_POINT('Ctrl Pts',(-34.0085729745541,-7.09307153439624,
173.485485071134));
#18189=CARTESIAN_POINT('Ctrl Pts',(-34.8168112016355,-9.12037466340095,
173.485485070589));
#18190=CARTESIAN_POINT('Ctrl Pts',(-35.0680967005658,-9.75067382667439,
173.485485070419));
#18191=CARTESIAN_POINT('Ctrl Pts',(-35.3187906222336,-10.3811932006048,
173.485485070032));
#18192=CARTESIAN_POINT('Ctrl Pts',(-35.5684276654212,-11.0121060305728,
173.485485069631));
#18193=CARTESIAN_POINT('Ctrl Pts',(-36.1217247789942,-12.4104651974658,
173.485485068744));
#18194=CARTESIAN_POINT('Ctrl Pts',(-36.6697688098148,-13.8108892372659,
173.485485069808));
#18195=CARTESIAN_POINT('Ctrl Pts',(-37.2074679799087,-15.2149580189824,
173.485485069755));
#18196=CARTESIAN_POINT('Ctrl Pts',(-37.3382977633442,-15.5565877347367,
173.485485069743));
#18197=CARTESIAN_POINT('Ctrl Pts',(-37.468532295522,-15.8984661779842,173.485485069646));
#18198=CARTESIAN_POINT('Ctrl Pts',(-37.5981312331992,-16.2405772327452,
173.485485069487));
#18199=CARTESIAN_POINT('Ctrl Pts',(-38.2042320224057,-17.8405423559423,
173.485485068741));
#18200=CARTESIAN_POINT('Ctrl Pts',(-38.7966004837565,-19.4464162536689,
173.485485069125));
#18201=CARTESIAN_POINT('Ctrl Pts',(-39.3708921954468,-21.0563433907389,
173.485485069113));
#18202=CARTESIAN_POINT('Ctrl Pts',(-39.4061988551619,-21.1553194832674,
173.485485069112));
#18203=CARTESIAN_POINT('Ctrl Pts',(-39.4414372081829,-21.2543108915996,
173.485485069111));
#18204=CARTESIAN_POINT('Ctrl Pts',(-39.4766062520292,-21.3533171832087,
173.48548506911));
#18205=CARTESIAN_POINT('Ctrl Pts',(-39.4944222863477,-21.403472072172,173.485485069109));
#18206=CARTESIAN_POINT('Ctrl Pts',(-39.5122206800506,-21.4536306880927,
173.485485069108));
#18207=CARTESIAN_POINT('Ctrl Pts',(-39.5300014121829,-21.5037930140745,
173.485485069108));
#18208=CARTESIAN_POINT('Ctrl Pts',(-40.2403129504007,-23.5076969401649,
173.485485069076));
#18209=CARTESIAN_POINT('Ctrl Pts',(-40.9225571901282,-25.5179357583437,
173.48548506908));
#18210=CARTESIAN_POINT('Ctrl Pts',(-41.5757221904205,-27.5347357495206,
173.48548506908));
#18211=CARTESIAN_POINT('Ctrl Pts',(-42.0697840289797,-29.0602674470261,
173.485485069079));
#18212=CARTESIAN_POINT('Ctrl Pts',(-42.5471460562807,-30.5895671389256,
173.485485069079));
#18213=CARTESIAN_POINT('Ctrl Pts',(-43.0087134036266,-32.1224297907549,
173.485485069079));
#18214=CARTESIAN_POINT('Ctrl Pts',(-43.7981108509673,-34.744014422848,173.485485069079));
#18215=CARTESIAN_POINT('Ctrl Pts',(-44.5413060994664,-37.376009024523,173.48548506902));
#18216=CARTESIAN_POINT('Ctrl Pts',(-45.2428170647038,-40.017413482018,173.485485069138));
#18217=CARTESIAN_POINT('Ctrl Pts',(-45.493755279941,-40.9622730111334,173.485485069181));
#18218=CARTESIAN_POINT('Ctrl Pts',(-45.7394230807557,-41.9083222817218,
173.485485069254));
#18219=CARTESIAN_POINT('Ctrl Pts',(-45.9800756370086,-42.855504556733,173.485485069449));
#18220=CARTESIAN_POINT('Ctrl Pts',(-46.8055463757926,-46.1044675617001,
173.485485070117));
#18221=CARTESIAN_POINT('Ctrl Pts',(-47.5720486324278,-49.3667352679054,
173.485485070976));
#18222=CARTESIAN_POINT('Ctrl Pts',(-48.2898944467056,-52.6399814576805,
173.485485070847));
#18223=CARTESIAN_POINT('Ctrl Pts',(-49.1606867247392,-56.6106356698621,
173.485485070692));
#18224=CARTESIAN_POINT('Ctrl Pts',(-49.9599970866321,-60.5974185446697,
173.485485069199));
#18225=CARTESIAN_POINT('Ctrl Pts',(-50.7024802268295,-64.5970226062537,
173.485485069085));
#18226=CARTESIAN_POINT('Ctrl Pts',(-23.7058176254365,21.1602837512234,174.985485069079));
#18227=CARTESIAN_POINT('Ctrl Pts',(-23.7058176254338,21.1602837512238,174.885642109295));
#18228=CARTESIAN_POINT('Ctrl Pts',(-23.7161844830976,21.1589768936689,174.786144799866));
#18229=CARTESIAN_POINT('Ctrl Pts',(-23.7586235790639,21.1536269742447,174.584144405165));
#18230=CARTESIAN_POINT('Ctrl Pts',(-23.7919598395692,21.1494245683377,174.482671933397));
#18231=CARTESIAN_POINT('Ctrl Pts',(-23.9170832171616,21.1336513768272,174.206914149823));
#18232=CARTESIAN_POINT('Ctrl Pts',(-24.0329636094545,21.1190433662763,174.046600077944));
#18233=CARTESIAN_POINT('Ctrl Pts',(-24.3205549456233,21.0827892840302,173.776548691605));
#18234=CARTESIAN_POINT('Ctrl Pts',(-24.4902654671712,21.0613953877858,173.670082332604));
#18235=CARTESIAN_POINT('Ctrl Pts',(-24.8631831017534,21.0143849778922,173.523272452218));
#18236=CARTESIAN_POINT('Ctrl Pts',(-25.0642980581857,20.9890322038205,173.485487368252));
#18237=CARTESIAN_POINT('Ctrl Pts',(-25.2666963042962,20.9635176568293,173.485485069184));
#18238=CARTESIAN_POINT('Ctrl Pts',(-25.0731721461106,22.0363186756089,178.485485069079));
#18239=CARTESIAN_POINT('Ctrl Pts',(-23.5958619350554,21.7764061127883,178.485485069079));
#18240=CARTESIAN_POINT('Ctrl Pts',(-23.5958619350554,21.7764061127883,176.985485069079));
#18241=CARTESIAN_POINT('Ctrl Pts',(-25.449767355314,19.8957990247877,178.485485069079));
#18242=CARTESIAN_POINT('Ctrl Pts',(-23.9768789732964,19.6107533436813,178.485485069079));
#18243=CARTESIAN_POINT('Ctrl Pts',(-23.9768789734403,19.6107533437049,176.985485069079));
#18244=CARTESIAN_POINT('Ctrl Pts',(-25.8813662389046,17.7650280978455,178.485485069079));
#18245=CARTESIAN_POINT('Ctrl Pts',(-24.4140007103611,17.4524520931911,178.485485069079));
#18246=CARTESIAN_POINT('Ctrl Pts',(-24.4140007103993,17.4524520932,176.985485069079));
#18247=CARTESIAN_POINT('Ctrl Pts',(-26.6240610131928,14.5857610350515,178.485485069079));
#18248=CARTESIAN_POINT('Ctrl Pts',(-25.166733162246,14.2302165608794,178.485485069079));
#18249=CARTESIAN_POINT('Ctrl Pts',(-25.1667331622269,14.230216560875,176.985485069079));
#18250=CARTESIAN_POINT('Ctrl Pts',(-26.8874605581482,13.5288117467589,178.485485069079));
#18251=CARTESIAN_POINT('Ctrl Pts',(-25.4337662241453,13.1586775991956,178.485485069079));
#18252=CARTESIAN_POINT('Ctrl Pts',(-25.4337662241455,13.1586775991956,176.985485069079));
#18253=CARTESIAN_POINT('Ctrl Pts',(-27.446805326032,11.4206813014582,178.485485069079));
#18254=CARTESIAN_POINT('Ctrl Pts',(-26.0008302787574,11.0214537140216,178.485485069079));
#18255=CARTESIAN_POINT('Ctrl Pts',(-26.0008302787573,11.0214537140216,176.985485069079));
#18256=CARTESIAN_POINT('Ctrl Pts',(-27.7430372661709,10.3686225285901,178.485485069079));
#18257=CARTESIAN_POINT('Ctrl Pts',(-26.3011521526689,9.95488187865359,178.485485069079));
#18258=CARTESIAN_POINT('Ctrl Pts',(-26.3011521526342,9.95488187864326,176.985485069079));
#18259=CARTESIAN_POINT('Ctrl Pts',(-28.6774913665414,7.22791185787921,178.485485069079));
#18260=CARTESIAN_POINT('Ctrl Pts',(-27.2481216681276,6.77210675800827,178.485485069079));
#18261=CARTESIAN_POINT('Ctrl Pts',(-27.248121668197,6.77210675802894,176.985485069079));
#18262=CARTESIAN_POINT('Ctrl Pts',(-29.3617331966933,5.15683817240694,178.485485069079));
#18263=CARTESIAN_POINT('Ctrl Pts',(-27.9410378920011,4.67506713939723,178.485485069079));
#18264=CARTESIAN_POINT('Ctrl Pts',(-27.9410378918206,4.67506713933211,176.985485069079));
#18265=CARTESIAN_POINT('Ctrl Pts',(-30.8219597323256,1.04872943986564,178.485485069079));
#18266=CARTESIAN_POINT('Ctrl Pts',(-29.4159166404766,0.525736800402789,
178.485485069079));
#18267=CARTESIAN_POINT('Ctrl Pts',(-29.4159166406572,0.525736800467916,
176.985485069079));
#18268=CARTESIAN_POINT('Ctrl Pts',(-31.5973036296917,-0.988543361219867,
178.485485069079));
#18269=CARTESIAN_POINT('Ctrl Pts',(-30.1971187077986,-1.52665999924347,
178.485485069079));
#18270=CARTESIAN_POINT('Ctrl Pts',(-30.1971187075851,-1.52665999932655,
176.985485069079));
#18271=CARTESIAN_POINT('Ctrl Pts',(-33.1867939298434,-5.04869237462202,
178.485485069079));
#18272=CARTESIAN_POINT('Ctrl Pts',(-31.7934224700594,-5.60421312732288,
178.485485069079));
#18273=CARTESIAN_POINT('Ctrl Pts',(-31.7934224702728,-5.6042131272398,176.985485069079));
#18274=CARTESIAN_POINT('Ctrl Pts',(-34.0001554699584,-7.07185978834832,
178.485485069079));
#18275=CARTESIAN_POINT('Ctrl Pts',(-32.6077646596627,-7.62976159871099,
178.485485069079));
#18276=CARTESIAN_POINT('Ctrl Pts',(-32.6077646595,-7.62976159877585,176.985485069079));
#18277=CARTESIAN_POINT('Ctrl Pts',(-35.6151374324291,-11.1225508305231,
178.485485069079));
#18278=CARTESIAN_POINT('Ctrl Pts',(-34.2208439624386,-11.6756803977577,
178.485485069079));
#18279=CARTESIAN_POINT('Ctrl Pts',(-34.2208439626013,-11.6756803976928,
176.985485069079));
#18280=CARTESIAN_POINT('Ctrl Pts',(-36.4165552279516,-13.1501496379901,
178.485485069079));
#18281=CARTESIAN_POINT('Ctrl Pts',(-35.019457301644,-13.6962459918701,178.485485069079));
#18282=CARTESIAN_POINT('Ctrl Pts',(-35.0194573015643,-13.6962459919006,
176.985485069079));
#18283=CARTESIAN_POINT('Ctrl Pts',(-37.9761224198699,-17.2214007871766,
178.485485069079));
#18284=CARTESIAN_POINT('Ctrl Pts',(-36.5717338991378,-17.7484650396609,
178.485485069079));
#18285=CARTESIAN_POINT('Ctrl Pts',(-36.5717338992174,-17.7484650396304,
176.985485069079));
#18286=CARTESIAN_POINT('Ctrl Pts',(-38.734830150851,-19.2660838657735,178.485485069079));
#18287=CARTESIAN_POINT('Ctrl Pts',(-37.325978725329,-19.7811777344504,178.485485069079));
#18288=CARTESIAN_POINT('Ctrl Pts',(-37.3259787253131,-19.7811777344522,
176.985485069079));
#18289=CARTESIAN_POINT('Ctrl Pts',(-40.1932912302604,-23.3698751428974,
178.485485069079));
#18290=CARTESIAN_POINT('Ctrl Pts',(-38.775354088112,-23.8594037872512,178.485485069079));
#18291=CARTESIAN_POINT('Ctrl Pts',(-38.7753540881279,-23.8594037872493,
176.985485069079));
#18292=CARTESIAN_POINT('Ctrl Pts',(-40.8932729804717,-25.4288026626252,
178.485485069079));
#18293=CARTESIAN_POINT('Ctrl Pts',(-39.4707067838494,-25.9047302427165,
178.485485069079));
#18294=CARTESIAN_POINT('Ctrl Pts',(-39.4707067838488,-25.9047302427205,
176.985485069079));
#18295=CARTESIAN_POINT('Ctrl Pts',(-42.9020403232724,-31.6275058626836,
178.485485069079));
#18296=CARTESIAN_POINT('Ctrl Pts',(-41.4663412551578,-32.062907708047,178.485485069079));
#18297=CARTESIAN_POINT('Ctrl Pts',(-41.466341255159,-32.062907708039,176.985485069079));
#18298=CARTESIAN_POINT('Ctrl Pts',(-44.1191756103108,-35.7893157557914,
178.485485069079));
#18299=CARTESIAN_POINT('Ctrl Pts',(-42.6757961471886,-36.1982867984866,
178.485485069079));
#18300=CARTESIAN_POINT('Ctrl Pts',(-42.6757961472487,-36.1982867984707,
176.985485069079));
#18301=CARTESIAN_POINT('Ctrl Pts',(-46.3446034332256,-44.1631447109512,
178.485485069079));
#18302=CARTESIAN_POINT('Ctrl Pts',(-44.8886245730121,-44.5247068037562,
178.485485069079));
#18303=CARTESIAN_POINT('Ctrl Pts',(-44.888624572952,-44.5247068037722,176.985485069079));
#18304=CARTESIAN_POINT('Ctrl Pts',(-47.3541432037895,-48.3748639172974,
178.485485069079));
#18305=CARTESIAN_POINT('Ctrl Pts',(-45.8931392134411,-48.7152180852625,
178.485485069079));
#18306=CARTESIAN_POINT('Ctrl Pts',(-45.8931392134804,-48.7152180852388,
176.985485069079));
#18307=CARTESIAN_POINT('Ctrl Pts',(-49.2109269784403,-56.8373208523129,
178.485485069079));
#18308=CARTESIAN_POINT('Ctrl Pts',(-47.7416378561892,-57.1399147959804,
178.485485069079));
#18309=CARTESIAN_POINT('Ctrl Pts',(-47.7416378561499,-57.1399147960041,
176.985485069079));
#18310=CARTESIAN_POINT('Ctrl Pts',(-50.0583093223098,-61.0880253217963,
178.485485069079));
#18311=CARTESIAN_POINT('Ctrl Pts',(-48.5857467556546,-61.3740109382993,
178.485485069079));
#18312=CARTESIAN_POINT('Ctrl Pts',(-48.5857467557009,-61.3740109382908,
176.985485069079));
#18313=CARTESIAN_POINT('Ctrl Pts',(-51.6262769651782,-69.6199183168499,
178.485485069079));
#18314=CARTESIAN_POINT('Ctrl Pts',(-50.1482524442177,-69.8761834157877,
178.485485069079));
#18315=CARTESIAN_POINT('Ctrl Pts',(-50.1482524441714,-69.8761834157962,
176.985485069079));
#18316=CARTESIAN_POINT('Ctrl Pts',(-52.3467978062058,-73.9011331254681,
178.485485069079));
#18317=CARTESIAN_POINT('Ctrl Pts',(-50.8665874458362,-74.144280974491,178.4854850692));
#18318=CARTESIAN_POINT('Ctrl Pts',(-50.8665874457456,-74.1442809745042,
176.9854850692));
#18319=CARTESIAN_POINT('Ctrl Pts',(-53.0168669615071,-78.1944557616716,
178.485485069079));
#18320=CARTESIAN_POINT('Ctrl Pts',(-51.5348087855333,-78.4257641338267,
178.485485069079));
#18321=CARTESIAN_POINT('Ctrl Pts',(-51.5348087855333,-78.4257641338267,
176.985485069079));
#18322=CARTESIAN_POINT('Ctrl Pts',(-25.2666963042872,20.9635176568304,178.485485068975));
#18323=CARTESIAN_POINT('Ctrl Pts',(-25.0646700006886,20.9889853163368,178.485482782905));
#18324=CARTESIAN_POINT('Ctrl Pts',(-24.8639197630959,21.0142921135478,178.44783645175));
#18325=CARTESIAN_POINT('Ctrl Pts',(-24.491242863047,21.0612721761796,178.301420092223));
#18326=CARTESIAN_POINT('Ctrl Pts',(-24.3214536667684,21.0826759902477,178.195070264549));
#18327=CARTESIAN_POINT('Ctrl Pts',(-24.0336437827003,21.1189576228839,177.925200211993));
#18328=CARTESIAN_POINT('Ctrl Pts',(-23.917632133555,21.1335821798189,177.76494125067));
#18329=CARTESIAN_POINT('Ctrl Pts',(-23.7922348975327,21.1493898942263,177.489079529908));
#18330=CARTESIAN_POINT('Ctrl Pts',(-23.758791421472,21.1536058158449,177.387454832855));
#18331=CARTESIAN_POINT('Ctrl Pts',(-23.71621735197,21.1589727501825,177.185140312999));
#18332=CARTESIAN_POINT('Ctrl Pts',(-23.7058175952175,21.1602837550329,177.085486338622));
#18333=CARTESIAN_POINT('Ctrl Pts',(-23.70581759522,21.1602837550326,176.985485069079));
#18334=CARTESIAN_POINT('Origin',(-53.4413942236179,-112.716773792997,173.485485069079));
#18335=CARTESIAN_POINT('',(-41.1490507210046,24.0009423880185,173.485485069079));
#18336=CARTESIAN_POINT('',(-55.4013296080738,22.2042843320105,173.485485069079));
#18337=CARTESIAN_POINT('',(-41.1020539958444,25.42062214227,173.485485069079));
#18338=CARTESIAN_POINT('Origin',(-36.6843857876575,24.5637629925993,173.485485069079));
#18339=CARTESIAN_POINT('',(-37.1738630900728,31.4290895869696,173.485485069079));
#18340=CARTESIAN_POINT('Origin',(-31.7758655563387,23.6116972707429,173.485485069079));
#18341=CARTESIAN_POINT('Origin',(-44.1060283439209,41.4682670878081,173.485485069079));
#18342=CARTESIAN_POINT('',(-7.55021677450188,-106.931681155043,173.485485069079));
#18343=CARTESIAN_POINT('Origin',(-55.4013296080738,22.2042843320105,180.985485069079));
#18344=CARTESIAN_POINT('',(-20.9569943874949,26.5463753651883,174.985485069079));
#18345=CARTESIAN_POINT('',(-24.5594210254598,26.0922494747562,171.485485069079));
#18346=CARTESIAN_POINT('Ctrl Pts',(-20.9569943874949,26.5463753651883,174.985485069079));
#18347=CARTESIAN_POINT('Ctrl Pts',(-20.9569943874949,26.5463753651883,174.886701580263));
#18348=CARTESIAN_POINT('Ctrl Pts',(-20.9613070986962,26.5458317000395,174.788168805464));
#18349=CARTESIAN_POINT('Ctrl Pts',(-20.9698519031794,26.5447545325259,174.690100174553));
#18350=CARTESIAN_POINT('Ctrl Pts',(-20.9784443243535,26.5436713623995,174.591485047383));
#18351=CARTESIAN_POINT('Ctrl Pts',(-20.991316196275,26.5420487199739,174.493338524244));
#18352=CARTESIAN_POINT('Ctrl Pts',(-21.0084374856327,26.5398903912816,174.395878356477));
#18353=CARTESIAN_POINT('Ctrl Pts',(-21.0149108898769,26.5390743467755,174.359029550847));
#18354=CARTESIAN_POINT('Ctrl Pts',(-21.0219922837033,26.5381816584295,174.322278925862));
#18355=CARTESIAN_POINT('Ctrl Pts',(-21.0296819391904,26.5372122919451,174.28563861018));
#18356=CARTESIAN_POINT('Ctrl Pts',(-21.0779351095987,26.5311294438597,174.055717855038));
#18357=CARTESIAN_POINT('Ctrl Pts',(-21.148865448191,26.5221878868457,173.834574324614));
#18358=CARTESIAN_POINT('Ctrl Pts',(-21.2414406256354,26.5105177574819,173.62180845516));
#18359=CARTESIAN_POINT('Ctrl Pts',(-21.3340158030797,26.498847628118,173.409042585707));
#18360=CARTESIAN_POINT('Ctrl Pts',(-21.4500317046224,26.4842225351218,173.202497940917));
#18361=CARTESIAN_POINT('Ctrl Pts',(-21.5836610718905,26.4673770691353,173.012195588691));
#18362=CARTESIAN_POINT('Ctrl Pts',(-21.7172904391586,26.4505316031489,172.821893236465));
#18363=CARTESIAN_POINT('Ctrl Pts',(-21.8682914407053,26.4314962497122,172.646838591098));
#18364=CARTESIAN_POINT('Ctrl Pts',(-22.0362862751098,26.4103186348906,172.486700043083));
#18365=CARTESIAN_POINT('Ctrl Pts',(-22.2042811095142,26.3891410200689,172.326561495067));
#18366=CARTESIAN_POINT('Ctrl Pts',(-22.390389099386,26.365680040815,172.181282504032));
#18367=CARTESIAN_POINT('Ctrl Pts',(-22.5853450510322,26.3411036777037,172.057259029844));
#18368=CARTESIAN_POINT('Ctrl Pts',(-22.7803010026784,26.3165273145925,171.933235555656));
#18369=CARTESIAN_POINT('Ctrl Pts',(-22.985880824076,26.290611694698,171.828488317195));
#18370=CARTESIAN_POINT('Ctrl Pts',(-23.2021330341362,26.2633507016728,171.743105349009));
#18371=CARTESIAN_POINT('Ctrl Pts',(-23.4183852441963,26.2360897086476,171.657722380822));
#18372=CARTESIAN_POINT('Ctrl Pts',(-23.6431960794103,26.2077498058597,171.593014493226));
#18373=CARTESIAN_POINT('Ctrl Pts',(-23.8695731252959,26.1792124648205,171.550160201754));
#18374=CARTESIAN_POINT('Ctrl Pts',(-24.0959501711816,26.1506751237814,171.507305910282));
#18375=CARTESIAN_POINT('Ctrl Pts',(-24.325855444624,26.1216930104701,171.485485069079));
#18376=CARTESIAN_POINT('Ctrl Pts',(-24.5594210254598,26.0922494747562,171.485485069079));
#18377=CARTESIAN_POINT('',(-55.4013296080738,22.2042843320105,171.485485069079));
#18378=CARTESIAN_POINT('Origin',(-41.1490507210046,24.0009423880185,173.985485069079));
#18379=CARTESIAN_POINT('',(-21.3209582807514,26.5004936738394,178.485485069079));
#18380=CARTESIAN_POINT('',(-41.1490507210046,24.0009423880185,178.485485069079));
#18381=CARTESIAN_POINT('',(-55.4013296080738,22.2042843320105,178.485485069079));
#18382=CARTESIAN_POINT('Origin',(-41.1490507210046,24.0009423880185,177.985485069079));
#18383=CARTESIAN_POINT('',(-24.559421025453,26.0922494747571,180.485485069079));
#18384=CARTESIAN_POINT('',(-24.4216473560585,26.109617376058,180.485485069079));
#18385=CARTESIAN_POINT('',(-20.9569943874949,26.5463753651883,176.985485069079));
#18386=CARTESIAN_POINT('Ctrl Pts',(-24.559421025453,26.0922494747571,180.485485069079));
#18387=CARTESIAN_POINT('Ctrl Pts',(-24.4824800351446,26.1019487411811,180.485485069079));
#18388=CARTESIAN_POINT('Ctrl Pts',(-24.4058343548432,26.1116107822155,180.48308261772));
#18389=CARTESIAN_POINT('Ctrl Pts',(-24.3294786223864,26.1212362572639,180.47833836426));
#18390=CARTESIAN_POINT('Ctrl Pts',(-24.2518299481371,26.1310247217639,180.473513775724));
#18391=CARTESIAN_POINT('Ctrl Pts',(-24.1744804020117,26.1407754583192,180.466267294623));
#18392=CARTESIAN_POINT('Ctrl Pts',(-24.0974265496722,26.1504889123961,180.456608401495));
#18393=CARTESIAN_POINT('Ctrl Pts',(-24.0203726973327,26.160202366473,180.446949508367));
#18394=CARTESIAN_POINT('Ctrl Pts',(-23.9436138073681,26.1698786341731,180.434877975413));
#18395=CARTESIAN_POINT('Ctrl Pts',(-23.8671595938527,26.1795165367008,180.420352216777));
#18396=CARTESIAN_POINT('Ctrl Pts',(-23.7777409465118,26.1907887500636,180.40336330761));
#18397=CARTESIAN_POINT('Ctrl Pts',(-23.6887478791473,26.202007371553,180.383010105823));
#18398=CARTESIAN_POINT('Ctrl Pts',(-23.600672382606,26.2131103107849,180.359405636771));
#18399=CARTESIAN_POINT('Ctrl Pts',(-23.5135638682412,26.2240913506831,180.336060321533));
#18400=CARTESIAN_POINT('Ctrl Pts',(-23.4273536194521,26.2349591363698,180.309535144864));
#18401=CARTESIAN_POINT('Ctrl Pts',(-23.3424927384906,26.2456567990874,180.279983354262));
#18402=CARTESIAN_POINT('Ctrl Pts',(-23.294289980915,26.2517332955456,180.263197318314));
#18403=CARTESIAN_POINT('Ctrl Pts',(-23.2465220763462,26.2577549698662,180.245435520943));
#18404=CARTESIAN_POINT('Ctrl Pts',(-23.1992667660851,26.2637120265967,180.226731704473));
#18405=CARTESIAN_POINT('Ctrl Pts',(-22.9847021376151,26.2907602812183,180.141806276839));
#18406=CARTESIAN_POINT('Ctrl Pts',(-22.7786882935836,26.3167306144865,180.037038838794));
#18407=CARTESIAN_POINT('Ctrl Pts',(-22.5816792108732,26.3415657975729,179.911375942728));
#18408=CARTESIAN_POINT('Ctrl Pts',(-22.3846701281627,26.3664009806592,179.785713046663));
#18409=CARTESIAN_POINT('Ctrl Pts',(-22.2017889982585,26.389455178373,179.642261663978));
#18410=CARTESIAN_POINT('Ctrl Pts',(-22.0344375412165,26.410551688332,179.482506548126));
#18411=CARTESIAN_POINT('Ctrl Pts',(-21.8670860841744,26.431648198291,179.322751432275));
#18412=CARTESIAN_POINT('Ctrl Pts',(-21.7133004196351,26.4510345894276,179.144165737668));
#18413=CARTESIAN_POINT('Ctrl Pts',(-21.5797898545736,26.4678650790763,178.953250199313));
#18414=CARTESIAN_POINT('Ctrl Pts',(-21.4462792895122,26.4846955687251,178.762334660957));
#18415=CARTESIAN_POINT('Ctrl Pts',(-21.3330091361679,26.4989745296635,178.560114310074));
#18416=CARTESIAN_POINT('Ctrl Pts',(-21.2402555850145,26.5106671450146,178.346434887201));
#18417=CARTESIAN_POINT('Ctrl Pts',(-21.147502033861,26.5223597603657,178.132755464328));
#18418=CARTESIAN_POINT('Ctrl Pts',(-21.0757990733503,26.5313987149541,177.906973211641));
#18419=CARTESIAN_POINT('Ctrl Pts',(-21.0284937221365,26.5373620799025,177.679645756147));
#18420=CARTESIAN_POINT('Ctrl Pts',(-20.9811883709227,26.5433254448509,177.452318300652));
#18421=CARTESIAN_POINT('Ctrl Pts',(-20.9569943874949,26.5463753651884,177.220993816469));
#18422=CARTESIAN_POINT('Ctrl Pts',(-20.9569943874949,26.5463753651884,176.985485069079));
#18423=CARTESIAN_POINT('',(-20.9569943874949,26.5463753651883,180.985485069079));
#18424=CARTESIAN_POINT('Origin',(-52.9434576820456,-13.7117130172939,180.985485069079));
#18425=CARTESIAN_POINT('',(-53.0330559861815,-12.4024452642559,171.485485069079));
#18426=CARTESIAN_POINT('',(-52.9434576820456,-13.7117130172939,171.485485069079));
#18427=CARTESIAN_POINT('',(-53.0330559861815,-12.4024452642559,173.485485069079));
#18428=CARTESIAN_POINT('',(-53.0330559861815,-12.4024452642559,180.985485069079));
#18429=CARTESIAN_POINT('',(-52.9434576820456,-13.7117130172939,173.485485069079));
#18430=CARTESIAN_POINT('Origin',(-63.3850491201885,-111.656713748515,180.985485069079));
#18431=CARTESIAN_POINT('',(-53.082572536869,-15.0166486334899,173.485485069079));
#18432=CARTESIAN_POINT('',(-53.082572536869,-15.0166486334899,171.485485069079));
#18433=CARTESIAN_POINT('',(-53.082572536869,-15.0166486334899,170.985485069079));
#18434=CARTESIAN_POINT('',(-63.3850491201885,-111.656713748515,171.485485069079));
#18435=CARTESIAN_POINT('',(-63.3850491201885,-111.656713748515,171.485485069079));
#18436=CARTESIAN_POINT('',(-63.3850491201885,-111.656713748515,173.485485069079));
#18437=CARTESIAN_POINT('',(-63.3850491201885,-111.656713748515,180.985485069079));
#18438=CARTESIAN_POINT('',(-63.3850491201885,-111.656713748515,173.485485069079));
#18439=CARTESIAN_POINT('Origin',(-53.4413942236179,-112.716773792997,180.985485069079));
#18440=CARTESIAN_POINT('',(-57.0153382075497,-112.335767487168,173.541420416595));
#18441=CARTESIAN_POINT('',(-60.8888270505344,-111.922827698136,172.515418850865));
#18442=CARTESIAN_POINT('Ctrl Pts',(-57.0153382075498,-112.335767487168,
173.541420416595));
#18443=CARTESIAN_POINT('Ctrl Pts',(-57.2280258358028,-112.313093565052,
173.272225027772));
#18444=CARTESIAN_POINT('Ctrl Pts',(-57.4821106107221,-112.286006430532,
173.039327830791));
#18445=CARTESIAN_POINT('Ctrl Pts',(-58.0784446078591,-112.222433242393,
172.646611798095));
#18446=CARTESIAN_POINT('Ctrl Pts',(-58.4215062269221,-112.185860581843,
172.497875229972));
#18447=CARTESIAN_POINT('Ctrl Pts',(-58.9537897151705,-112.129115605866,
172.368671149366));
#18448=CARTESIAN_POINT('Ctrl Pts',(-59.1339560066465,-112.109908675522,
172.340024858843));
#18449=CARTESIAN_POINT('Ctrl Pts',(-59.5707164861963,-112.063347090452,
172.299854718465));
#18450=CARTESIAN_POINT('Ctrl Pts',(-59.8357943853675,-112.035088015443,
172.303335717215));
#18451=CARTESIAN_POINT('Ctrl Pts',(-60.3675672608762,-111.978397474195,
172.366333772718));
#18452=CARTESIAN_POINT('Ctrl Pts',(-60.6324827847851,-111.950155709474,
172.427035584321));
#18453=CARTESIAN_POINT('Ctrl Pts',(-60.8888270505344,-111.922827698136,
172.515418850865));
#18454=CARTESIAN_POINT('',(-62.0210982548684,-111.80212002317,173.485485069079));
#18455=CARTESIAN_POINT('Ctrl Pts',(-60.8888270505344,-111.922827698136,
172.515418850865));
#18456=CARTESIAN_POINT('Ctrl Pts',(-61.1058388649012,-111.899692788891,
172.639451350805));
#18457=CARTESIAN_POINT('Ctrl Pts',(-61.310701839086,-111.877853027175,172.783834155405));
#18458=CARTESIAN_POINT('Ctrl Pts',(-61.6906606007499,-111.837346884718,
173.109414086522));
#18459=CARTESIAN_POINT('Ctrl Pts',(-61.8649365864974,-111.818767900318,
173.289924177764));
#18460=CARTESIAN_POINT('Ctrl Pts',(-62.0210982548684,-111.80212002317,173.485485069079));
#18461=CARTESIAN_POINT('',(-53.4413942236179,-112.716773792997,173.485485069079));
#18462=CARTESIAN_POINT('',(-62.88786637536,-111.709716750739,170.985485069079));
#18463=CARTESIAN_POINT('Origin',(-62.88786637536,-111.709716750739,171.485485069079));
#18464=CARTESIAN_POINT('',(-57.4188561822461,-112.292749775204,170.985485069079));
#18465=CARTESIAN_POINT('',(-53.4413942236179,-112.716773792997,170.985485069079));
#18466=CARTESIAN_POINT('',(-53.4413942236179,-112.716773792997,174.985485069079));
#18467=CARTESIAN_POINT('Origin',(-57.4188561822461,-112.292749775204,174.985485069079));
#18468=CARTESIAN_POINT('',(-53.4413942236179,-112.716773792997,176.985485069079));
#18469=CARTESIAN_POINT('',(-53.4413942236179,-112.716773792997,180.985485069079));
#18470=CARTESIAN_POINT('',(-57.4188561822461,-112.292749775204,180.985485069079));
#18471=CARTESIAN_POINT('Origin',(-57.4188561822461,-112.292749775204,176.985485069079));
#18472=CARTESIAN_POINT('',(-62.88786637536,-111.709716750739,180.985485069079));
#18473=CARTESIAN_POINT('',(-53.4413942236179,-112.716773792997,180.985485069079));
#18474=CARTESIAN_POINT('',(-63.3850491201885,-111.656713748515,180.485485069079));
#18475=CARTESIAN_POINT('Origin',(-62.88786637536,-111.709716750739,180.485485069079));
#18476=CARTESIAN_POINT('',(-63.3850491201885,-111.656713748515,178.985485069079));
#18477=CARTESIAN_POINT('',(-63.3850491201885,-111.656713748515,180.985485069079));
#18478=CARTESIAN_POINT('Origin',(-62.88786637536,-111.709716750739,178.985485069079));
#18479=CARTESIAN_POINT('',(-60.8888270454861,-111.922827698674,179.455551290205));
#18480=CARTESIAN_POINT('Ctrl Pts',(-62.0210982548537,-111.802120023171,
178.485485069079));
#18481=CARTESIAN_POINT('Ctrl Pts',(-61.8656334742916,-111.818693607423,
178.680173249399));
#18482=CARTESIAN_POINT('Ctrl Pts',(-61.6922139029917,-111.837181292321,
178.859946907849));
#18483=CARTESIAN_POINT('Ctrl Pts',(-61.3125284291585,-111.87765830047,179.185847773914));
#18484=CARTESIAN_POINT('Ctrl Pts',(-61.1068076160046,-111.899589513552,
179.330965100789));
#18485=CARTESIAN_POINT('Ctrl Pts',(-60.8888270454861,-111.922827698674,
179.455551290205));
#18486=CARTESIAN_POINT('',(-57.0153371209007,-112.335767603012,178.42954834513));
#18487=CARTESIAN_POINT('Ctrl Pts',(-60.888827045486,-111.922827698674,179.455551290205));
#18488=CARTESIAN_POINT('Ctrl Pts',(-60.6328315485644,-111.950118528925,
179.543814307164));
#18489=CARTESIAN_POINT('Ctrl Pts',(-60.3682870318124,-111.978320741804,
179.604471510014));
#18490=CARTESIAN_POINT('Ctrl Pts',(-59.8372616671249,-112.034931593404,
179.667537944491));
#18491=CARTESIAN_POINT('Ctrl Pts',(-59.5725535707745,-112.063151244962,
179.671129691791));
#18492=CARTESIAN_POINT('Ctrl Pts',(-59.136191489744,-112.109670358089,179.631251769103));
#18493=CARTESIAN_POINT('Ctrl Pts',(-58.956303432779,-112.128847626775,179.602744942888));
#18494=CARTESIAN_POINT('Ctrl Pts',(-58.4237297979111,-112.18562353432,179.473976739277));
#18495=CARTESIAN_POINT('Ctrl Pts',(-58.0800579015758,-112.222261254505,
179.325242151835));
#18496=CARTESIAN_POINT('Ctrl Pts',(-57.4827491337447,-112.285938359712,
178.932226803426));
#18497=CARTESIAN_POINT('Ctrl Pts',(-57.228292602565,-112.313065125933,178.699083057342));
#18498=CARTESIAN_POINT('Ctrl Pts',(-57.0153371209008,-112.335767603012,
178.42954834513));
#18499=CARTESIAN_POINT('',(-55.9273125369417,-112.451758292321,176.985485069089));
#18500=CARTESIAN_POINT('Origin',(-57.4188631216847,-112.292749035413,176.985488314375));
#18501=CARTESIAN_POINT('',(-55.9273079477605,-112.451758781876,174.985485069079));
#18502=CARTESIAN_POINT('',(-55.9273079477605,-112.451758781876,176.985485069079));
#18503=CARTESIAN_POINT('Origin',(-57.4188561822461,-112.292749775204,174.985485069079));
#18504=CARTESIAN_POINT('Origin',(-67.998054881725,-13.4265585667677,180.985485069079));
#18505=CARTESIAN_POINT('',(-53.0330559861815,-12.4024452642559,178.985485069079));
#18506=CARTESIAN_POINT('',(-53.0330559861815,-12.4024452642559,180.485485069079));
#18507=CARTESIAN_POINT('',(-53.0330559861815,-12.4024452642559,180.985485069079));
#18508=CARTESIAN_POINT('',(-53.082572536869,-15.0166486334899,178.985485069079));
#18509=CARTESIAN_POINT('Origin',(-67.998054881725,-13.4265585667677,178.985485069079));
#18510=CARTESIAN_POINT('',(-53.082572536869,-15.0166486334899,180.485485069079));
#18511=CARTESIAN_POINT('',(-53.082572536869,-15.0166486334899,170.985485069079));
#18512=CARTESIAN_POINT('Origin',(-67.998054881725,-13.4265585667677,180.485485069079));
#18513=CARTESIAN_POINT('Ctrl Pts',(-53.4413942236179,-112.716773792997,
176.985485069079));
#18514=CARTESIAN_POINT('Ctrl Pts',(-53.4413942236179,-112.716773792997,
174.585485069079));
#18515=CARTESIAN_POINT('Ctrl Pts',(-42.7208173800685,-12.1548131952256,
176.985485069079));
#18516=CARTESIAN_POINT('Ctrl Pts',(-42.7208173800685,-12.1548131952256,
174.585485069079));
#18517=CARTESIAN_POINT('Ctrl Pts',(-26.1502242325394,-14.6226249149956,
176.985485069079));
#18518=CARTESIAN_POINT('Ctrl Pts',(-26.1502242325394,-14.6226249149956,
174.585485069079));
#18519=CARTESIAN_POINT('Ctrl Pts',(-20.3993997473094,25.9801832318931,176.985485069079));
#18520=CARTESIAN_POINT('Ctrl Pts',(-20.3993997473094,25.9801832318931,174.585485069079));
#18521=CARTESIAN_POINT('',(-20.3993997459831,25.9801832412571,174.985485069079));
#18522=CARTESIAN_POINT('Ctrl Pts',(-53.4413942236179,-112.716773792997,
174.985485069079));
#18523=CARTESIAN_POINT('Ctrl Pts',(-52.8096223112116,-106.790579420312,
174.985485069079));
#18524=CARTESIAN_POINT('Ctrl Pts',(-52.1206641754933,-100.87124426812,174.98548506908));
#18525=CARTESIAN_POINT('Ctrl Pts',(-50.5942726079286,-89.0503828822984,
174.98548506908));
#18526=CARTESIAN_POINT('Ctrl Pts',(-49.757265425744,-83.1507260725826,174.985485069079));
#18527=CARTESIAN_POINT('Ctrl Pts',(-47.888174002584,-71.4000958425799,174.985485069079));
#18528=CARTESIAN_POINT('Ctrl Pts',(-46.8562222321137,-65.5467331693134,
174.985485069079));
#18529=CARTESIAN_POINT('Ctrl Pts',(-44.5210591976856,-53.901141681327,174.985485069079));
#18530=CARTESIAN_POINT('Ctrl Pts',(-43.2178767803996,-48.1089063654215,
174.985485069079));
#18531=CARTESIAN_POINT('Ctrl Pts',(-40.9750678687189,-39.4854680169988,
174.985485069079));
#18532=CARTESIAN_POINT('Ctrl Pts',(-40.1790492411628,-36.6219000231504,
174.985485069079));
#18533=CARTESIAN_POINT('Ctrl Pts',(-38.4756477469119,-30.9198622377508,
174.985485069079));
#18534=CARTESIAN_POINT('Ctrl Pts',(-37.5677629527721,-28.0815055657851,
174.985485069079));
#18535=CARTESIAN_POINT('Ctrl Pts',(-35.6349943284908,-22.4311603405326,
174.985485069079));
#18536=CARTESIAN_POINT('Ctrl Pts',(-34.608328317987,-19.6177595316176,174.985485069079));
#18537=CARTESIAN_POINT('Ctrl Pts',(-32.4706666932395,-14.0256929237095,
174.985485069079));
#18538=CARTESIAN_POINT('Ctrl Pts',(-31.3585525008225,-11.2457550461466,
174.985485069079));
#18539=CARTESIAN_POINT('Ctrl Pts',(-29.1380236708638,-5.6845035686739,174.985485069079));
#18540=CARTESIAN_POINT('Ctrl Pts',(-28.0318787018384,-2.90234596622778,
174.985485069079));
#18541=CARTESIAN_POINT('Ctrl Pts',(-25.959804002289,2.7141098997671,174.985485069079));
#18542=CARTESIAN_POINT('Ctrl Pts',(-24.9969151286383,5.54953894117839,174.985485069079));
#18543=CARTESIAN_POINT('Ctrl Pts',(-23.2984117431506,11.3049116288563,174.985485069079));
#18544=CARTESIAN_POINT('Ctrl Pts',(-22.5666401222046,14.2084908208118,174.985485069079));
#18545=CARTESIAN_POINT('Ctrl Pts',(-21.3283637469275,20.0618248638162,174.985485069079));
#18546=CARTESIAN_POINT('Ctrl Pts',(-20.8198378348718,23.0117450437847,174.985485069079));
#18547=CARTESIAN_POINT('Ctrl Pts',(-20.3993997459139,25.9801832417458,174.985485069079));
#18548=CARTESIAN_POINT('',(-20.399399745983,25.9801832412581,176.985485069079));
#18549=CARTESIAN_POINT('',(-20.3993997459139,25.9801832417458,174.985485069079));
#18550=CARTESIAN_POINT('Ctrl Pts',(-20.3993997459139,25.9801832417458,176.985485069079));
#18551=CARTESIAN_POINT('Ctrl Pts',(-20.8194918499154,23.0141878171383,176.985485069079));
#18552=CARTESIAN_POINT('Ctrl Pts',(-21.32754882053,20.0665006828847,176.985485069079));
#18553=CARTESIAN_POINT('Ctrl Pts',(-22.2553679339636,15.6794644341189,176.985485069079));
#18554=CARTESIAN_POINT('Ctrl Pts',(-22.5922397393381,14.2228632003925,176.985485069079));
#18555=CARTESIAN_POINT('Ctrl Pts',(-23.3244477728418,11.3218290413609,176.985485069079));
#18556=CARTESIAN_POINT('Ctrl Pts',(-23.7201299995547,9.87649782832845,176.985485069079));
#18557=CARTESIAN_POINT('Ctrl Pts',(-24.9920882209669,5.56474808425753,176.985485069079));
#18558=CARTESIAN_POINT('Ctrl Pts',(-25.9534941549082,2.73229051813628,176.985485069079));
#18559=CARTESIAN_POINT('Ctrl Pts',(-28.0226448730915,-2.87838666024527,
176.985485069079));
#18560=CARTESIAN_POINT('Ctrl Pts',(-29.1273699516833,-5.65772547397114,
176.985485069079));
#18561=CARTESIAN_POINT('Ctrl Pts',(-31.3455088620405,-11.2131827659292,
176.985485069079));
#18562=CARTESIAN_POINT('Ctrl Pts',(-32.4566496657803,-13.9901437025305,
176.985485069079));
#18563=CARTESIAN_POINT('Ctrl Pts',(-34.5927847123162,-19.5759943027127,
176.985485069079));
#18564=CARTESIAN_POINT('Ctrl Pts',(-35.6188539822851,-22.3860236816944,
176.985485069079));
#18565=CARTESIAN_POINT('Ctrl Pts',(-37.5513960609844,-28.0316432492908,
176.985485069079));
#18566=CARTESIAN_POINT('Ctrl Pts',(-38.4595477409101,-30.8684137262953,
176.985485069079));
#18567=CARTESIAN_POINT('Ctrl Pts',(-40.1639162339715,-36.5688422501229,
176.985485069079));
#18568=CARTESIAN_POINT('Ctrl Pts',(-40.9606327724711,-39.4323802592758,
176.98548506908));
#18569=CARTESIAN_POINT('Ctrl Pts',(-43.2058271638625,-48.0578135867489,
176.985485069079));
#18570=CARTESIAN_POINT('Ctrl Pts',(-44.5109607325329,-53.8541412455957,
176.98548506908));
#18571=CARTESIAN_POINT('Ctrl Pts',(-46.8499201547131,-65.5119666514209,
176.98548506908));
#18572=CARTESIAN_POINT('Ctrl Pts',(-47.8837400389295,-71.3734658322673,
176.98548506908));
#18573=CARTESIAN_POINT('Ctrl Pts',(-49.7562860675246,-83.1433271304293,
176.98548506908));
#18574=CARTESIAN_POINT('Ctrl Pts',(-50.5938605211195,-89.0473685697446,
176.985485069079));
#18575=CARTESIAN_POINT('Ctrl Pts',(-52.120387756833,-100.868926655335,176.985485069079));
#18576=CARTESIAN_POINT('Ctrl Pts',(-52.8094746128609,-106.789193969142,
176.985485069079));
#18577=CARTESIAN_POINT('Ctrl Pts',(-53.4413942236179,-112.716773792997,
176.985485069079));
#18578=CARTESIAN_POINT('Origin',(-52.9434576820456,-13.7117130172939,180.985485069079));
#18579=CARTESIAN_POINT('',(-52.9434576820456,-13.7117130172939,178.985485069079));
#18580=CARTESIAN_POINT('',(-54.4340581561246,8.06989492938438,180.485485069079));
#18581=CARTESIAN_POINT('Origin',(-63.3850491201885,-111.656713748515,180.985485069079));
#18582=CARTESIAN_POINT('',(-63.3850491201885,-111.656713748515,178.985485069079));
#18583=CARTESIAN_POINT('',(-53.082572536869,-15.0166486334899,180.485485069079));
#18584=CARTESIAN_POINT('Origin',(-34.9583934096621,-20.6140499623174,180.985485069079));
#18585=CARTESIAN_POINT('',(-24.4968853993556,25.596175592946,180.985485069079));
#18586=CARTESIAN_POINT('Ctrl Pts',(-57.4188561822461,-112.292749775204,
180.985485069079));
#18587=CARTESIAN_POINT('Ctrl Pts',(-56.790512649408,-106.398714547387,180.985485069079));
#18588=CARTESIAN_POINT('Ctrl Pts',(-56.1058731125984,-100.511880940133,
180.98548506906));
#18589=CARTESIAN_POINT('Ctrl Pts',(-55.3484913384761,-94.6343530226705,
180.985485069073));
#18590=CARTESIAN_POINT('Ctrl Pts',(-55.338924151294,-94.5601085508923,180.985485069073));
#18591=CARTESIAN_POINT('Ctrl Pts',(-55.3293453578738,-94.4858656122032,
180.985485069073));
#18592=CARTESIAN_POINT('Ctrl Pts',(-55.3197549249144,-94.4116242090743,
180.985485069073));
#18593=CARTESIAN_POINT('Ctrl Pts',(-54.9352546151986,-91.4351326765513,
180.985485069079));
#18594=CARTESIAN_POINT('Ctrl Pts',(-54.5319470084521,-88.4611202257547,
180.985485069078));
#18595=CARTESIAN_POINT('Ctrl Pts',(-54.1069203483626,-85.4898333910159,
180.985485069077));
#18596=CARTESIAN_POINT('Ctrl Pts',(-53.7033042231981,-82.6682238507177,
180.985485069076));
#18597=CARTESIAN_POINT('Ctrl Pts',(-53.2799637223225,-79.8481667017225,
180.985485069075));
#18598=CARTESIAN_POINT('Ctrl Pts',(-52.8343681747547,-77.0334451025294,
180.985485069077));
#18599=CARTESIAN_POINT('Ctrl Pts',(-52.8106597636878,-76.8836846817239,
180.985485069077));
#18600=CARTESIAN_POINT('Ctrl Pts',(-52.7868882204028,-76.7339390343581,
180.985485069077));
#18601=CARTESIAN_POINT('Ctrl Pts',(-52.7630531680916,-76.5842087401903,
180.985485069077));
#18602=CARTESIAN_POINT('Ctrl Pts',(-51.8554066519163,-70.8824306155612,
180.985485069076));
#18603=CARTESIAN_POINT('Ctrl Pts',(-50.8566834398535,-65.2025739806144,
180.985485068139));
#18604=CARTESIAN_POINT('Ctrl Pts',(-49.7333492755762,-59.5526619928141,
180.985485068761));
#18605=CARTESIAN_POINT('Ctrl Pts',(-49.6887622529058,-59.3284074816482,
180.985485068785));
#18606=CARTESIAN_POINT('Ctrl Pts',(-49.643978469431,-59.1042002714389,180.985485068806));
#18607=CARTESIAN_POINT('Ctrl Pts',(-49.5989958321339,-58.8800408668684,
180.985485068823));
#18608=CARTESIAN_POINT('Ctrl Pts',(-48.480916301155,-53.3083790660962,180.985485069247));
#18609=CARTESIAN_POINT('Ctrl Pts',(-47.2399537491611,-47.7662638000103,
180.985485068065));
#18610=CARTESIAN_POINT('Ctrl Pts',(-45.8293087716645,-42.2649422848648,
180.985485068732));
#18611=CARTESIAN_POINT('Ctrl Pts',(-45.7533507434525,-41.9687164154809,
180.985485068768));
#18612=CARTESIAN_POINT('Ctrl Pts',(-45.6769001981415,-41.6726090103213,
180.985485068799));
#18613=CARTESIAN_POINT('Ctrl Pts',(-45.5999497834957,-41.3766218285166,
180.985485068827));
#18614=CARTESIAN_POINT('Ctrl Pts',(-44.8469362038317,-38.4801804210025,
180.985485069096));
#18615=CARTESIAN_POINT('Ctrl Pts',(-44.0456768427767,-35.5953424896882,
180.985485069068));
#18616=CARTESIAN_POINT('Ctrl Pts',(-43.1891752015397,-32.7237825622821,
180.985485069046));
#18617=CARTESIAN_POINT('Ctrl Pts',(-42.4423310849265,-30.2198671766812,
180.985485069027));
#18618=CARTESIAN_POINT('Ctrl Pts',(-41.6531322686351,-27.7261321945819,
180.985485069014));
#18619=CARTESIAN_POINT('Ctrl Pts',(-40.8200495521006,-25.2429405912916,
180.985485068515));
#18620=CARTESIAN_POINT('Ctrl Pts',(-40.6977329751789,-24.8783483476563,
180.985485068442));
#18621=CARTESIAN_POINT('Ctrl Pts',(-40.5744720942236,-24.5139805152869,
180.985485068402));
#18622=CARTESIAN_POINT('Ctrl Pts',(-40.4502615514014,-24.1498393561786,
180.98548506839));
#18623=CARTESIAN_POINT('Ctrl Pts',(-39.616810792004,-21.7064579918356,180.985485068307));
#18624=CARTESIAN_POINT('Ctrl Pts',(-38.739353495722,-19.2722820499251,180.985485070954));
#18625=CARTESIAN_POINT('Ctrl Pts',(-37.8282880086107,-16.8505834688252,
180.985485066549));
#18626=CARTESIAN_POINT('Ctrl Pts',(-37.6788085609924,-16.4532529022283,
180.985485065826));
#18627=CARTESIAN_POINT('Ctrl Pts',(-37.5284339691997,-16.056244665969,180.985485065289));
#18628=CARTESIAN_POINT('Ctrl Pts',(-37.3772084254297,-15.6595731913905,
180.985485065039));
#18629=CARTESIAN_POINT('Ctrl Pts',(-36.4693625270572,-13.2782521379502,
180.985485063537));
#18630=CARTESIAN_POINT('Ctrl Pts',(-35.5299993620731,-10.9085007698185,
180.985485072686));
#18631=CARTESIAN_POINT('Ctrl Pts',(-34.5852825795174,-8.54078321761435,
180.985485064032));
#18632=CARTESIAN_POINT('Ctrl Pts',(-34.4134917762452,-8.11022867711563,
180.985485062458));
#18633=CARTESIAN_POINT('Ctrl Pts',(-34.2415483012594,-7.67973099356383,
180.985485061337));
#18634=CARTESIAN_POINT('Ctrl Pts',(-34.0696087116074,-7.24923200405654,
180.98548506096));
#18635=CARTESIAN_POINT('Ctrl Pts',(-33.138509657603,-4.91796436120965,180.985485058921));
#18636=CARTESIAN_POINT('Ctrl Pts',(-32.2088990960437,-2.58615052122322,
180.985485069115));
#18637=CARTESIAN_POINT('Ctrl Pts',(-31.3204104332397,-0.23907854190687,
180.985485069028));
#18638=CARTESIAN_POINT('Ctrl Pts',(-31.1425632790713,0.230730572857145,
180.985485069011));
#18639=CARTESIAN_POINT('Ctrl Pts',(-30.9663469447662,0.701142876122788,
180.985485068984));
#18640=CARTESIAN_POINT('Ctrl Pts',(-30.7920966781887,1.17228422073675,180.985485067611));
#18641=CARTESIAN_POINT('Ctrl Pts',(-30.2848140693334,2.54388505171172,180.985485063616));
#18642=CARTESIAN_POINT('Ctrl Pts',(-29.7950938569279,3.9220018739976,180.985485032927));
#18643=CARTESIAN_POINT('Ctrl Pts',(-29.3283958544553,5.30867284540019,180.985485020463));
#18644=CARTESIAN_POINT('Ctrl Pts',(-29.006637155384,6.26469460987012,180.985485011869));
#18645=CARTESIAN_POINT('Ctrl Pts',(-28.6958217757076,7.22478169314873,180.985485026902));
#18646=CARTESIAN_POINT('Ctrl Pts',(-28.3977441390982,8.18958797408848,180.985485051181));
#18647=CARTESIAN_POINT('Ctrl Pts',(-28.2377424180365,8.70747541843852,180.985485064214));
#18648=CARTESIAN_POINT('Ctrl Pts',(-28.0812847212611,9.22671577439412,180.985485065958));
#18649=CARTESIAN_POINT('Ctrl Pts',(-27.9286546962701,9.74743161800556,180.985485067269));
#18650=CARTESIAN_POINT('Ctrl Pts',(-27.6620631180387,10.6569411235348,180.985485069558));
#18651=CARTESIAN_POINT('Ctrl Pts',(-27.4072505288242,11.5694243155145,180.98548506854));
#18652=CARTESIAN_POINT('Ctrl Pts',(-27.1645811034528,12.4843659981785,180.985485068803));
#18653=CARTESIAN_POINT('Ctrl Pts',(-27.0208715104168,13.0261973255743,180.985485068958));
#18654=CARTESIAN_POINT('Ctrl Pts',(-26.8813686318622,13.5689896620425,180.985485068973));
#18655=CARTESIAN_POINT('Ctrl Pts',(-26.7461389996539,14.1125915128495,180.985485068982));
#18656=CARTESIAN_POINT('Ctrl Pts',(-26.5222826941656,15.01245864989,180.985485068997));
#18657=CARTESIAN_POINT('Ctrl Pts',(-26.3100078534052,15.9148533438117,180.985485068952));
#18658=CARTESIAN_POINT('Ctrl Pts',(-26.1088919070564,16.8196034741691,180.985485069001));
#18659=CARTESIAN_POINT('Ctrl Pts',(-25.9838202837391,17.3822568567309,180.985485069031));
#18660=CARTESIAN_POINT('Ctrl Pts',(-25.8630558838012,17.9458267556442,180.985485069048));
#18661=CARTESIAN_POINT('Ctrl Pts',(-25.7464863690264,18.5102872637228,180.985485069058));
#18662=CARTESIAN_POINT('Ctrl Pts',(-25.4428718519307,19.9804692826755,180.985485069085));
#18663=CARTESIAN_POINT('Ctrl Pts',(-25.1676456839084,21.4566808478938,180.985485069079));
#18664=CARTESIAN_POINT('Ctrl Pts',(-24.9177905698878,22.9382808324062,180.985485069079));
#18665=CARTESIAN_POINT('Ctrl Pts',(-24.7929746613216,23.6784187676397,180.98548506908));
#18666=CARTESIAN_POINT('Ctrl Pts',(-24.6744808830026,24.4198997434739,180.985485069079));
#18667=CARTESIAN_POINT('Ctrl Pts',(-24.5619054245002,25.1626388829568,180.985485069079));
#18668=CARTESIAN_POINT('Ctrl Pts',(-24.5400091817329,25.3071037310443,180.985485069079));
#18669=CARTESIAN_POINT('Ctrl Pts',(-24.5183368251832,25.4516161749795,180.985485069079));
#18670=CARTESIAN_POINT('Ctrl Pts',(-24.4968853949886,25.5961755921264,180.985485069079));
#18671=CARTESIAN_POINT('',(-41.2825923197859,23.4801507949034,180.985485069079));
#18672=CARTESIAN_POINT('',(-41.2825923197859,23.4801507949034,180.985485069079));
#18673=CARTESIAN_POINT('',(-53.9352248596064,8.10403203946808,180.985485069079));
#18674=CARTESIAN_POINT('Origin',(-39.4690592605811,9.0940082318961,180.985485069079));
#18675=CARTESIAN_POINT('',(-52.5342226896633,-12.3683081541722,180.985485069079));
#18676=CARTESIAN_POINT('',(-52.5342226896634,-12.3683081541722,180.985485069079));
#18677=CARTESIAN_POINT('',(-52.5853897920404,-15.069651635714,180.985485069079));
#18678=CARTESIAN_POINT('Origin',(-67.998054881725,-13.4265585667677,180.985485069079));
#18679=CARTESIAN_POINT('',(-62.88786637536,-111.709716750739,180.985485069079));
#18680=CARTESIAN_POINT('Origin',(-34.9583934096621,-20.6140499623174,170.985485069079));
#18681=CARTESIAN_POINT('',(-52.5853897920404,-15.069651635714,170.985485069079));
#18682=CARTESIAN_POINT('',(-52.9717383111942,-18.6937070505612,170.985485069079));
#18683=CARTESIAN_POINT('',(-52.5342226896633,-12.3683081541722,170.985485069079));
#18684=CARTESIAN_POINT('Origin',(-67.998054881725,-13.4265585667677,170.985485069079));
#18685=CARTESIAN_POINT('',(-53.9352248596064,8.10403203946808,170.985485069079));
#18686=CARTESIAN_POINT('',(-51.890637311636,-21.772789521366,170.985485069079));
#18687=CARTESIAN_POINT('',(-41.2825923197859,23.4801507949034,170.985485069079));
#18688=CARTESIAN_POINT('Origin',(-39.4690592605811,9.0940082318961,170.985485069079));
#18689=CARTESIAN_POINT('',(-24.4968853993885,25.5961755929473,170.985485069079));
#18690=CARTESIAN_POINT('',(-40.5289338663117,23.5751578139663,170.985485069079));
#18691=CARTESIAN_POINT('Ctrl Pts',(-24.4968853950575,25.5961755921349,170.985485069079));
#18692=CARTESIAN_POINT('Ctrl Pts',(-24.5183775783598,25.4513415431335,170.985485069079));
#18693=CARTESIAN_POINT('Ctrl Pts',(-24.5400914677881,25.3065550532397,170.985485069079));
#18694=CARTESIAN_POINT('Ctrl Pts',(-24.5620299993144,25.1618167559765,170.985485069079));
#18695=CARTESIAN_POINT('Ctrl Pts',(-24.6746763176248,24.4186386501074,170.985485069079));
#18696=CARTESIAN_POINT('Ctrl Pts',(-24.7932455255501,23.6767312043179,170.985485069073));
#18697=CARTESIAN_POINT('Ctrl Pts',(-24.9181365313699,22.9361802250035,170.985485069089));
#18698=CARTESIAN_POINT('Ctrl Pts',(-25.1681453406982,21.4537334517548,170.985485069122));
#18699=CARTESIAN_POINT('Ctrl Pts',(-25.4435247881484,19.9767295764349,170.985485068169));
#18700=CARTESIAN_POINT('Ctrl Pts',(-25.7472506552232,18.5058117725121,170.985485072688));
#18701=CARTESIAN_POINT('Ctrl Pts',(-25.8639593378723,17.9406018322643,170.985485074424));
#18702=CARTESIAN_POINT('Ctrl Pts',(-25.9849446272495,17.3763067468434,170.985485077132));
#18703=CARTESIAN_POINT('Ctrl Pts',(-26.1102556574466,16.8129413020526,170.985485082236));
#18704=CARTESIAN_POINT('Ctrl Pts',(-26.3996867343658,15.5117352779024,170.985485094025));
#18705=CARTESIAN_POINT('Ctrl Pts',(-26.7122276139814,14.2154907367009,170.985485119168));
#18706=CARTESIAN_POINT('Ctrl Pts',(-27.0488579985707,12.9244120340896,170.985485101699));
#18707=CARTESIAN_POINT('Ctrl Pts',(-27.0879359754081,12.7745362476317,170.985485099671));
#18708=CARTESIAN_POINT('Ctrl Pts',(-27.1273385599953,12.6247301299435,170.985485097187));
#18709=CARTESIAN_POINT('Ctrl Pts',(-27.1670672687997,12.4749940432329,170.985485094385));
#18710=CARTESIAN_POINT('Ctrl Pts',(-27.4097208281513,11.560441431352,170.985485077277));
#18711=CARTESIAN_POINT('Ctrl Pts',(-27.6643178615963,10.6485868038839,170.985485072147));
#18712=CARTESIAN_POINT('Ctrl Pts',(-27.9310501337635,9.73907607216142,170.985485072818));
#18713=CARTESIAN_POINT('Ctrl Pts',(-28.0841852446823,9.2169119348693,170.985485073203));
#18714=CARTESIAN_POINT('Ctrl Pts',(-28.2411510909769,8.69623022151272,170.985485073994));
#18715=CARTESIAN_POINT('Ctrl Pts',(-28.4016770094243,8.17685932462075,170.985485087244));
#18716=CARTESIAN_POINT('Ctrl Pts',(-28.8331432557161,6.78087907742721,170.985485122858));
#18717=CARTESIAN_POINT('Ctrl Pts',(-29.2912634424619,5.3947931577226,170.985485123205));
#18718=CARTESIAN_POINT('Ctrl Pts',(-29.770586941813,4.01662412744066,170.985485101063));
#18719=CARTESIAN_POINT('Ctrl Pts',(-30.1035894227145,3.05916281622453,170.98548508568));
#18720=CARTESIAN_POINT('Ctrl Pts',(-30.4468264422819,2.10552126126155,170.985485073463));
#18721=CARTESIAN_POINT('Ctrl Pts',(-30.7984770656628,1.15502342646039,170.985485070612));
#18722=CARTESIAN_POINT('Ctrl Pts',(-30.9733231577022,0.682421301348085,
170.985485069194));
#18723=CARTESIAN_POINT('Ctrl Pts',(-31.15014353561,0.210551172825435,170.985485069155));
#18724=CARTESIAN_POINT('Ctrl Pts',(-31.3286006360414,-0.260715918856281,
170.985485069136));
#18725=CARTESIAN_POINT('Ctrl Pts',(-32.2178889544888,-2.60913645515496,
170.98548506904));
#18726=CARTESIAN_POINT('Ctrl Pts',(-33.1482064936523,-4.9422839287474,170.985485079299));
#18727=CARTESIAN_POINT('Ctrl Pts',(-34.079873038293,-7.27493507937169,170.985485077263));
#18728=CARTESIAN_POINT('Ctrl Pts',(-34.2524227913675,-7.70695486409456,
170.985485076885));
#18729=CARTESIAN_POINT('Ctrl Pts',(-34.4249718336375,-8.13897504114208,
170.985485075754));
#18730=CARTESIAN_POINT('Ctrl Pts',(-34.5973624686691,-8.57105438556268,
170.985485074165));
#18731=CARTESIAN_POINT('Ctrl Pts',(-35.5425661780249,-10.9401099842479,
170.98548506545));
#18732=CARTESIAN_POINT('Ctrl Pts',(-36.4822688726745,-13.3112613391608,
170.985485074703));
#18733=CARTESIAN_POINT('Ctrl Pts',(-37.3903504544009,-15.6940571120185,
170.985485073188));
#18734=CARTESIAN_POINT('Ctrl Pts',(-37.542139679303,-16.0923503168805,170.985485072934));
#18735=CARTESIAN_POINT('Ctrl Pts',(-37.6930696748215,-16.4909865893479,
170.985485072388));
#18736=CARTESIAN_POINT('Ctrl Pts',(-37.8430949741869,-16.8899478627579,
170.985485071651));
#18737=CARTESIAN_POINT('Ctrl Pts',(-38.7542950670207,-19.3130961644508,
170.985485067177));
#18738=CARTESIAN_POINT('Ctrl Pts',(-39.6317664375482,-21.7487445692906,
170.985485069843));
#18739=CARTESIAN_POINT('Ctrl Pts',(-40.464924739775,-24.1928394847348,170.985485069762));
#18740=CARTESIAN_POINT('Ctrl Pts',(-40.5896004612047,-24.5585794599729,
170.98548506975));
#18741=CARTESIAN_POINT('Ctrl Pts',(-40.7133135695025,-24.9245349475724,
170.98548506971));
#18742=CARTESIAN_POINT('Ctrl Pts',(-40.8360698007184,-25.2907036421335,
170.985485069638));
#18743=CARTESIAN_POINT('Ctrl Pts',(-41.6687056219754,-27.7743671490236,
170.985485069145));
#18744=CARTESIAN_POINT('Ctrl Pts',(-42.4572397555062,-30.2679730819714,
170.985485069131));
#18745=CARTESIAN_POINT('Ctrl Pts',(-43.2033006997277,-32.7711592916608,
170.985485069113));
#18746=CARTESIAN_POINT('Ctrl Pts',(-44.0593573456883,-35.6434034527833,
170.985485069092));
#18747=CARTESIAN_POINT('Ctrl Pts',(-44.859958903692,-38.5281560241757,170.985485069062));
#18748=CARTESIAN_POINT('Ctrl Pts',(-45.6122146833682,-41.423821403948,170.985485069353));
#18749=CARTESIAN_POINT('Ctrl Pts',(-45.6894902577951,-41.721279012936,170.985485069383));
#18750=CARTESIAN_POINT('Ctrl Pts',(-45.7662597309399,-42.0188508621958,
170.985485069417));
#18751=CARTESIAN_POINT('Ctrl Pts',(-45.8425306268857,-42.3165352636523,
170.985485069456));
#18752=CARTESIAN_POINT('Ctrl Pts',(-47.2512086805445,-47.8145889845178,
170.985485070179));
#18753=CARTESIAN_POINT('Ctrl Pts',(-48.490005626333,-53.3509733909632,170.98548506891));
#18754=CARTESIAN_POINT('Ctrl Pts',(-49.6060214953918,-58.9150621777573,
170.985485069344));
#18755=CARTESIAN_POINT('Ctrl Pts',(-49.6512921438859,-59.1407667708916,
170.985485069362));
#18756=CARTESIAN_POINT('Ctrl Pts',(-49.6963607743348,-59.3665169394474,
170.985485069382));
#18757=CARTESIAN_POINT('Ctrl Pts',(-49.7412295360745,-59.5923121966672,
170.985485069408));
#18758=CARTESIAN_POINT('Ctrl Pts',(-50.8623576811791,-65.2342200203911,
170.985485070049));
#18759=CARTESIAN_POINT('Ctrl Pts',(-51.8590090750871,-70.9043245719156,
170.985485069059));
#18760=CARTESIAN_POINT('Ctrl Pts',(-52.7647123253029,-76.5947288226584,
170.985485069125));
#18761=CARTESIAN_POINT('Ctrl Pts',(-52.7888259492539,-76.7462312802221,
170.985485069127));
#18762=CARTESIAN_POINT('Ctrl Pts',(-52.8128750527938,-76.8977498306085,
170.985485069129));
#18763=CARTESIAN_POINT('Ctrl Pts',(-52.8368600283206,-77.049284227944,170.985485069132));
#18764=CARTESIAN_POINT('Ctrl Pts',(-53.7497954202113,-82.8171081000875,
170.985485069235));
#18765=CARTESIAN_POINT('Ctrl Pts',(-54.5700444916928,-88.6081190949848,
170.985485069075));
#18766=CARTESIAN_POINT('Ctrl Pts',(-55.3194711561834,-94.4094288582262,
170.985485069086));
#18767=CARTESIAN_POINT('Ctrl Pts',(-55.3292569335755,-94.4851805342949,
170.985485069086));
#18768=CARTESIAN_POINT('Ctrl Pts',(-55.3390305632831,-94.5609336213681,
170.985485069086));
#18769=CARTESIAN_POINT('Ctrl Pts',(-55.3487920806066,-94.6366881163334,
170.985485069086));
#18770=CARTESIAN_POINT('Ctrl Pts',(-56.1061223474536,-100.513968254811,
170.9854850691));
#18771=CARTESIAN_POINT('Ctrl Pts',(-56.7906477111516,-106.399981462517,
170.985485069079));
#18772=CARTESIAN_POINT('Ctrl Pts',(-57.4188561822461,-112.292749775204,
170.985485069079));
#18773=CARTESIAN_POINT('Origin',(-67.998054881725,-13.4265585667677,180.985485069079));
#18774=CARTESIAN_POINT('Origin',(-67.998054881725,-13.4265585667677,171.485485069079));
#18775=CARTESIAN_POINT('Origin',(-67.998054881725,-13.4265585667677,173.485485069079));
#18776=CARTESIAN_POINT('Ctrl Pts',(-57.4188561822461,-112.292749775204,
170.985485069079));
#18777=CARTESIAN_POINT('Ctrl Pts',(-53.4413942236179,-112.716773792997,
170.985485069079));
#18778=CARTESIAN_POINT('Ctrl Pts',(-53.4413942236179,-112.716773792997,
174.985485069079));
#18779=CARTESIAN_POINT('Ctrl Pts',(-56.7826130392591,-106.324614029273,
170.985485069079));
#18780=CARTESIAN_POINT('Ctrl Pts',(-52.8079181997713,-106.774594389709,
170.985485067414));
#18781=CARTESIAN_POINT('Ctrl Pts',(-52.8079182001533,-106.774594389693,
174.98548506783));
#18782=CARTESIAN_POINT('Ctrl Pts',(-56.0885640554346,-100.362870586925,
170.985485069079));
#18783=CARTESIAN_POINT('Ctrl Pts',(-52.1171985560672,-100.841826095817,
170.985485068746));
#18784=CARTESIAN_POINT('Ctrl Pts',(-52.1171985561525,-100.841826095775,
174.985485068829));
#18785=CARTESIAN_POINT('Ctrl Pts',(-54.5503923877258,-88.455985304064,170.985485069079));
#18786=CARTESIAN_POINT('Ctrl Pts',(-50.587687217705,-89.0019798491525,170.985485069413));
#18787=CARTESIAN_POINT('Ctrl Pts',(-50.5876872176197,-89.0019798491944,
174.985485069329));
#18788=CARTESIAN_POINT('Ctrl Pts',(-53.7067133387789,-82.5129732641369,
170.985485069079));
#18789=CARTESIAN_POINT('Ctrl Pts',(-49.7493162082364,-83.0969773147974,
170.985485069079));
#18790=CARTESIAN_POINT('Ctrl Pts',(-49.7493162081637,-83.096977314809,174.985485069079));
#18791=CARTESIAN_POINT('Ctrl Pts',(-51.8227490518109,-70.6764783742679,
170.985485069079));
#18792=CARTESIAN_POINT('Ctrl Pts',(-47.879595467558,-71.3499712035021,170.985485069079));
#18793=CARTESIAN_POINT('Ctrl Pts',(-47.8795954676306,-71.3499712034905,
174.985485069079));
#18794=CARTESIAN_POINT('Ctrl Pts',(-50.7825461626129,-64.7803920175373,
170.985485069079));
#18795=CARTESIAN_POINT('Ctrl Pts',(-46.8482928517823,-65.5053796921416,
170.985485069079));
#18796=CARTESIAN_POINT('Ctrl Pts',(-46.8482928517271,-65.5053796921527,
174.985485069079));
#18797=CARTESIAN_POINT('Ctrl Pts',(-48.429587030133,-53.0497142451155,170.985485069079));
#18798=CARTESIAN_POINT('Ctrl Pts',(-44.5200735879382,-53.8980425350056,
170.985485069079));
#18799=CARTESIAN_POINT('Ctrl Pts',(-44.5200735879935,-53.8980425349946,
174.985485069079));
#18800=CARTESIAN_POINT('Ctrl Pts',(-47.116819037505,-47.2151254801378,170.985485069079));
#18801=CARTESIAN_POINT('Ctrl Pts',(-43.2231877084345,-48.1356655301653,
170.985485069079));
#18802=CARTESIAN_POINT('Ctrl Pts',(-43.2231877083669,-48.1356655301828,
174.985485069079));
#18803=CARTESIAN_POINT('Ctrl Pts',(-44.8599803826999,-38.5281517318545,
170.985485069079));
#18804=CARTESIAN_POINT('Ctrl Pts',(-40.9995722140334,-39.5765736406343,
170.985485069079));
#18805=CARTESIAN_POINT('Ctrl Pts',(-40.9995722140672,-39.5765736406255,
174.985485069079));
#18806=CARTESIAN_POINT('Ctrl Pts',(-44.0593677242217,-35.6433989890554,
170.985485069079));
#18807=CARTESIAN_POINT('Ctrl Pts',(-40.2116389363166,-36.7377081133746,
170.985485069079));
#18808=CARTESIAN_POINT('Ctrl Pts',(-40.2116389362875,-36.7377081133832,
174.985485069079));
#18809=CARTESIAN_POINT('Ctrl Pts',(-42.3472650417746,-29.8989102456991,
170.985485069079));
#18810=CARTESIAN_POINT('Ctrl Pts',(-38.5282657072424,-31.0896131337399,
170.985485069079));
#18811=CARTESIAN_POINT('Ctrl Pts',(-38.5282657072715,-31.0896131337312,
174.985485069079));
#18812=CARTESIAN_POINT('Ctrl Pts',(-41.4353095848977,-27.039279258621,170.985485069079));
#18813=CARTESIAN_POINT('Ctrl Pts',(-37.6324604140697,-28.2806667005876,
170.985485069079));
#18814=CARTESIAN_POINT('Ctrl Pts',(-37.6324604140849,-28.2806667005877,
174.985485069079));
#18815=CARTESIAN_POINT('Ctrl Pts',(-39.4946798076272,-21.3463520167058,
170.985485069079));
#18816=CARTESIAN_POINT('Ctrl Pts',(-35.7253902478902,-22.686188130551,170.985485069079));
#18817=CARTESIAN_POINT('Ctrl Pts',(-35.725390247875,-22.6861881305509,174.985485069079));
#18818=CARTESIAN_POINT('Ctrl Pts',(-38.4642123465852,-18.5114604936425,
170.985485069079));
#18819=CARTESIAN_POINT('Ctrl Pts',(-34.7124817228929,-19.8992827188875,
170.985485069079));
#18820=CARTESIAN_POINT('Ctrl Pts',(-34.712481722994,-19.899282718849,174.985485069079));
#18821=CARTESIAN_POINT('Ctrl Pts',(-36.316827378144,-12.8765246130018,170.985485069079));
#18822=CARTESIAN_POINT('Ctrl Pts',(-32.5929839678225,-14.3375254538628,
170.985485069079));
#18823=CARTESIAN_POINT('Ctrl Pts',(-32.5929839677214,-14.3375254539014,
174.985485069079));
#18824=CARTESIAN_POINT('Ctrl Pts',(-35.1986985564766,-10.0755969552936,
170.985485069079));
#18825=CARTESIAN_POINT('Ctrl Pts',(-31.4848789139723,-11.5613793000778,
170.985485069079));
#18826=CARTESIAN_POINT('Ctrl Pts',(-31.4848789142267,-11.561379299971,174.985485069079));
#18827=CARTESIAN_POINT('Ctrl Pts',(-32.9615227473215,-4.47408340352996,
170.985485069079));
#18828=CARTESIAN_POINT('Ctrl Pts',(-29.2459613632304,-5.95550471904053,
170.985485069079));
#18829=CARTESIAN_POINT('Ctrl Pts',(-29.2459613629761,-5.95550471914736,
174.985485069079));
#18830=CARTESIAN_POINT('Ctrl Pts',(-31.8444493580227,-1.67276288830323,
170.985485069079));
#18831=CARTESIAN_POINT('Ctrl Pts',(-28.1161190404298,-3.12330252930428,
170.985485069079));
#18832=CARTESIAN_POINT('Ctrl Pts',(-28.1161190407185,-3.12330252919715,
174.985485069079));
#18833=CARTESIAN_POINT('Ctrl Pts',(-29.7527124597669,3.98288655387735,170.985485069079));
#18834=CARTESIAN_POINT('Ctrl Pts',(-25.9777796362599,2.65835101834502,170.985485069079));
#18835=CARTESIAN_POINT('Ctrl Pts',(-25.9777796359711,2.6583510182379,174.985485069079));
#18836=CARTESIAN_POINT('Ctrl Pts',(-28.7818376120864,6.83882893219871,170.985485069079));
#18837=CARTESIAN_POINT('Ctrl Pts',(-24.9741240759836,5.6087285236563,170.985485069079));
#18838=CARTESIAN_POINT('Ctrl Pts',(-24.9741240760463,5.60872852367469,174.985485069079));
#18839=CARTESIAN_POINT('Ctrl Pts',(-27.0805945471387,12.6394205519279,170.985485069079));
#18840=CARTESIAN_POINT('Ctrl Pts',(-23.2116619383549,11.618053890714,170.985485069079));
#18841=CARTESIAN_POINT('Ctrl Pts',(-23.2116619382922,11.6180538906956,174.985485069079));
#18842=CARTESIAN_POINT('Ctrl Pts',(-26.3554676902183,15.562162940868,170.985485069079));
#18843=CARTESIAN_POINT('Ctrl Pts',(-22.4590134306381,14.65207208465,170.985485069079));
#18844=CARTESIAN_POINT('Ctrl Pts',(-22.4590134305428,14.6520720846303,174.985485069079));
#18845=CARTESIAN_POINT('Ctrl Pts',(-25.4433917160236,19.9776877415196,170.985485069079));
#18846=CARTESIAN_POINT('Ctrl Pts',(-21.5156656424655,19.2189893943357,170.985485069079));
#18847=CARTESIAN_POINT('Ctrl Pts',(-21.5156656425132,19.2189893943455,174.985485069079));
#18848=CARTESIAN_POINT('Ctrl Pts',(-25.1680142641662,21.4546534375747,170.985485069079));
#18849=CARTESIAN_POINT('Ctrl Pts',(-21.2313563309936,20.7441370734468,170.985485069079));
#18850=CARTESIAN_POINT('Ctrl Pts',(-21.2313563309339,20.7441370734394,174.985485069079));
#18851=CARTESIAN_POINT('Ctrl Pts',(-24.7932108072927,23.6769458352522,170.985485069079));
#18852=CARTESIAN_POINT('Ctrl Pts',(-20.8450961455913,23.0343589425206,170.985485069079));
#18853=CARTESIAN_POINT('Ctrl Pts',(-20.8450961456211,23.0343589425243,174.985485069079));
#18854=CARTESIAN_POINT('Ctrl Pts',(-24.6746446772461,24.418849042421,170.985485069079));
#18855=CARTESIAN_POINT('Ctrl Pts',(-20.7230313702667,23.7981943284674,170.985485069079));
#18856=CARTESIAN_POINT('Ctrl Pts',(-20.7230313702386,23.7981943284632,174.985485069079));
#18857=CARTESIAN_POINT('Ctrl Pts',(-24.505722723831,25.5333006223766,170.985485069079));
#18858=CARTESIAN_POINT('Ctrl Pts',(-20.5492881240966,24.9444540731779,170.985485069079));
#18859=CARTESIAN_POINT('Ctrl Pts',(-20.5492881241107,24.94445407318,174.985485069079));
#18860=CARTESIAN_POINT('Ctrl Pts',(-24.4509032451114,25.9050506043959,170.985485069079));
#18861=CARTESIAN_POINT('Ctrl Pts',(-20.4929326108229,25.3266255922602,170.985485069079));
#18862=CARTESIAN_POINT('Ctrl Pts',(-20.4929326108094,25.3266255922583,174.985485069079));
#18863=CARTESIAN_POINT('Ctrl Pts',(-24.3441364534122,26.6490642977548,170.985485069079));
#18864=CARTESIAN_POINT('Ctrl Pts',(-20.3832266462647,26.0911211678509,170.985485069079));
#18865=CARTESIAN_POINT('Ctrl Pts',(-20.3832266462781,26.0911211678529,174.985485069079));
#18866=CARTESIAN_POINT('Ctrl Pts',(-24.2925780488274,27.0213863993399,170.985485069079));
#18867=CARTESIAN_POINT('Ctrl Pts',(-20.3297617855482,26.4772473384921,170.985485069079));
#18868=CARTESIAN_POINT('Ctrl Pts',(-20.3297617855514,26.4772473384925,174.985485069079));
#18869=CARTESIAN_POINT('Ctrl Pts',(-24.2414621684861,27.3938099964894,170.985485069079));
#18870=CARTESIAN_POINT('Ctrl Pts',(-20.2786142962294,26.8499012345166,170.985485069079));
#18871=CARTESIAN_POINT('Ctrl Pts',(-20.2786142962294,26.8499012345166,174.985485069079));
#18872=CARTESIAN_POINT('Ctrl Pts',(-24.4968853994471,25.5961755935782,170.985485069079));
#18873=CARTESIAN_POINT('Ctrl Pts',(-24.2311967766072,25.620873127159,170.985485069285));
#18874=CARTESIAN_POINT('Ctrl Pts',(-23.9697295431316,25.6452190869017,171.010442378523));
#18875=CARTESIAN_POINT('Ctrl Pts',(-23.7123793162008,25.6692186217661,171.059399504179));
#18876=CARTESIAN_POINT('Ctrl Pts',(-23.7113153156031,25.6693178465452,171.059601914768));
#18877=CARTESIAN_POINT('Ctrl Pts',(-23.7102513470147,25.6694170689936,171.059804751606));
#18878=CARTESIAN_POINT('Ctrl Pts',(-23.7091874109976,25.6695162890582,171.060008014593));
#18879=CARTESIAN_POINT('Ctrl Pts',(-23.5057804574324,25.6884855228749,171.098868532867));
#18880=CARTESIAN_POINT('Ctrl Pts',(-23.3035081474716,25.7073729132474,171.153320157475));
#18881=CARTESIAN_POINT('Ctrl Pts',(-23.1063670980905,25.7258021132664,171.222655786241));
#18882=CARTESIAN_POINT('Ctrl Pts',(-23.0549689640615,25.7306069293897,171.240732802426));
#18883=CARTESIAN_POINT('Ctrl Pts',(-23.0039194998808,25.7353806115,171.259821295379));
#18884=CARTESIAN_POINT('Ctrl Pts',(-22.9532892035529,25.7401165199994,171.279908231871));
#18885=CARTESIAN_POINT('Ctrl Pts',(-22.9514181264669,25.7402915387237,171.280650558291));
#18886=CARTESIAN_POINT('Ctrl Pts',(-22.9495477609699,25.7404664927989,171.281394161589));
#18887=CARTESIAN_POINT('Ctrl Pts',(-22.9476781070859,25.7406413822181,171.282139041655));
#18888=CARTESIAN_POINT('Ctrl Pts',(-22.749261664958,25.759201467923,171.361189209017));
#18889=CARTESIAN_POINT('Ctrl Pts',(-22.5588332490509,25.7770361827933,171.454634081597));
#18890=CARTESIAN_POINT('Ctrl Pts',(-22.3764129335352,25.7941386741052,171.562330579903));
#18891=CARTESIAN_POINT('Ctrl Pts',(-22.3344346010229,25.7980742777963,171.587113562016));
#18892=CARTESIAN_POINT('Ctrl Pts',(-22.2928802296816,25.8019711166271,171.612651042871));
#18893=CARTESIAN_POINT('Ctrl Pts',(-22.2517498765304,25.8058291246237,171.63894093754));
#18894=CARTESIAN_POINT('Ctrl Pts',(-22.249557397228,25.8060347781626,171.640342336884));
#18895=CARTESIAN_POINT('Ctrl Pts',(-22.2473659252672,25.8062403399649,171.641746095296));
#18896=CARTESIAN_POINT('Ctrl Pts',(-22.2451754709029,25.8064458090578,171.643152205469));
#18897=CARTESIAN_POINT('Ctrl Pts',(-22.0863321814473,25.8213456340087,171.74511788384));
#18898=CARTESIAN_POINT('Ctrl Pts',(-21.9327437650712,25.8357658974467,171.859516657719));
#18899=CARTESIAN_POINT('Ctrl Pts',(-21.7883375934458,25.849334383468,171.983584558283));
#18900=CARTESIAN_POINT('Ctrl Pts',(-21.733215969023,25.8545136426509,172.030942812718));
#18901=CARTESIAN_POINT('Ctrl Pts',(-21.6794318011014,25.8595688351721,172.079709652122));
#18902=CARTESIAN_POINT('Ctrl Pts',(-21.6272015230238,25.8644794472182,172.1297306957));
#18903=CARTESIAN_POINT('Ctrl Pts',(-21.6251536123851,25.8646719886908,172.131691983886));
#18904=CARTESIAN_POINT('Ctrl Pts',(-21.6231079442685,25.8648643215606,172.133655207642));
#18905=CARTESIAN_POINT('Ctrl Pts',(-21.6210645192453,25.8650564457624,172.135620367119));
#18906=CARTESIAN_POINT('Ctrl Pts',(-21.4322727467778,25.8828067758117,172.317181196012));
#18907=CARTESIAN_POINT('Ctrl Pts',(-21.2625723923638,25.8987813228249,172.515322627133));
#18908=CARTESIAN_POINT('Ctrl Pts',(-21.1123142886195,25.9129371819159,172.730296947743));
#18909=CARTESIAN_POINT('Ctrl Pts',(-21.1108026321242,25.9130795955083,172.73245967521));
#18910=CARTESIAN_POINT('Ctrl Pts',(-21.1092929703707,25.9132218225119,172.734624218554));
#18911=CARTESIAN_POINT('Ctrl Pts',(-21.1077853097955,25.913363862311,172.736790566379));
#18912=CARTESIAN_POINT('Ctrl Pts',(-20.9825286565164,25.9251645488611,172.916771049295));
#18913=CARTESIAN_POINT('Ctrl Pts',(-20.871068234139,25.9356720301901,173.109226845106));
#18914=CARTESIAN_POINT('Ctrl Pts',(-20.7770687387732,25.9445374993322,173.307711809801));
#18915=CARTESIAN_POINT('Ctrl Pts',(-20.758343486239,25.9463035529463,173.347251182578));
#18916=CARTESIAN_POINT('Ctrl Pts',(-20.7403111257963,25.9480044477976,173.387029977365));
#18917=CARTESIAN_POINT('Ctrl Pts',(-20.7230006234092,25.9496374272564,173.426997467644));
#18918=CARTESIAN_POINT('Ctrl Pts',(-20.7221958278602,25.9497133473291,173.42885562621));
#18919=CARTESIAN_POINT('Ctrl Pts',(-20.7213924732957,25.9497891318426,173.430714336564));
#18920=CARTESIAN_POINT('Ctrl Pts',(-20.7205905601952,25.9498647807505,173.432573598924));
#18921=CARTESIAN_POINT('Ctrl Pts',(-20.6265972034254,25.9587316951138,173.650500342107));
#18922=CARTESIAN_POINT('Ctrl Pts',(-20.5524177598076,25.9657340826921,173.875976284431));
#18923=CARTESIAN_POINT('Ctrl Pts',(-20.4988179155159,25.9707948958704,174.109381554084));
#18924=CARTESIAN_POINT('Ctrl Pts',(-20.4930004344399,25.9713441733037,174.134714290721));
#18925=CARTESIAN_POINT('Ctrl Pts',(-20.4874254268857,25.9718705746878,174.160140452629));
#18926=CARTESIAN_POINT('Ctrl Pts',(-20.4820939068001,25.9723739982273,174.18566053939));
#18927=CARTESIAN_POINT('Ctrl Pts',(-20.481863032781,25.9723957982795,174.186765651047));
#18928=CARTESIAN_POINT('Ctrl Pts',(-20.481632638324,25.972417553073,174.187870862314));
#18929=CARTESIAN_POINT('Ctrl Pts',(-20.4814027234763,25.9724392626033,174.188976172781));
#18930=CARTESIAN_POINT('Ctrl Pts',(-20.4595046689509,25.9745069693321,174.294250578148));
#18931=CARTESIAN_POINT('Ctrl Pts',(-20.4419804524051,25.9761618272396,174.400292622434));
#18932=CARTESIAN_POINT('Ctrl Pts',(-20.4288329501748,25.9774034459845,174.50689626372));
#18933=CARTESIAN_POINT('Ctrl Pts',(-20.4157271529572,25.9786411262074,174.613161749047));
#18934=CARTESIAN_POINT('Ctrl Pts',(-20.4069702858337,25.9794681908885,174.71998596903));
#18935=CARTESIAN_POINT('Ctrl Pts',(-20.4026160570217,25.9798794514795,174.82717079242));
#18936=CARTESIAN_POINT('Ctrl Pts',(-20.4004755131676,25.9800816276554,174.879862973944));
#18937=CARTESIAN_POINT('Ctrl Pts',(-20.3993997459139,25.9801832417458,174.932642329276));
#18938=CARTESIAN_POINT('Ctrl Pts',(-20.3993997459139,25.9801832417458,174.985485069079));
#18939=CARTESIAN_POINT('Ctrl Pts',(-24.2415334023097,27.3932909961974,180.985485069079));
#18940=CARTESIAN_POINT('Ctrl Pts',(-20.278685530053,26.8493822342246,180.985485069079));
#18941=CARTESIAN_POINT('Ctrl Pts',(-20.278685530053,26.8493822342246,176.985485069079));
#18942=CARTESIAN_POINT('Ctrl Pts',(-24.2926179909382,27.0210953863739,180.985485069079));
#18943=CARTESIAN_POINT('Ctrl Pts',(-20.3298036372618,26.4769424124262,180.985485069079));
#18944=CARTESIAN_POINT('Ctrl Pts',(-20.3298036372611,26.4769424124265,176.985485069079));
#18945=CARTESIAN_POINT('Ctrl Pts',(-24.3441461251675,26.6489998256275,180.985485069079));
#18946=CARTESIAN_POINT('Ctrl Pts',(-20.3832365919444,26.0910548674088,180.985485069079));
#18947=CARTESIAN_POINT('Ctrl Pts',(-20.3832365919587,26.0910548674102,176.985485069079));
#18948=CARTESIAN_POINT('Ctrl Pts',(-24.4508478987634,25.9054333651556,180.985485069079));
#18949=CARTESIAN_POINT('Ctrl Pts',(-20.4928757331822,25.3270189434495,180.985485069079));
#18950=CARTESIAN_POINT('Ctrl Pts',(-20.4928757331679,25.3270189434481,176.985485069079));
#18951=CARTESIAN_POINT('Ctrl Pts',(-24.5056334618508,25.5339044052764,180.985485069079));
#18952=CARTESIAN_POINT('Ctrl Pts',(-20.5491963566518,24.9450748104871,180.985485069079));
#18953=CARTESIAN_POINT('Ctrl Pts',(-20.5491963566663,24.9450748104893,176.985485069079));
#18954=CARTESIAN_POINT('Ctrl Pts',(-24.6744493717257,24.4201078416409,180.985485069079));
#18955=CARTESIAN_POINT('Ctrl Pts',(-20.7228304061464,23.7994896118014,180.985485069079));
#18956=CARTESIAN_POINT('Ctrl Pts',(-20.7228304061173,23.799489611797,176.985485069079));
#18957=CARTESIAN_POINT('Ctrl Pts',(-24.7929390693147,23.6786305769485,180.985485069079));
#18958=CARTESIAN_POINT('Ctrl Pts',(-20.844816338285,23.0360937770448,180.985485069079));
#18959=CARTESIAN_POINT('Ctrl Pts',(-20.8448163383128,23.0360937770495,176.985485069079));
#18960=CARTESIAN_POINT('Ctrl Pts',(-25.1674956400503,21.4575816922395,180.985485069079));
#18961=CARTESIAN_POINT('Ctrl Pts',(-21.2308213810126,20.7471576413164,180.985485069079));
#18962=CARTESIAN_POINT('Ctrl Pts',(-21.2308213809569,20.747157641307,176.985485069079));
#18963=CARTESIAN_POINT('Ctrl Pts',(-25.4426848277649,19.9813991557405,180.985485069079));
#18964=CARTESIAN_POINT('Ctrl Pts',(-21.514935511514,19.2228232467,180.985485069079));
#18965=CARTESIAN_POINT('Ctrl Pts',(-21.5149355115658,19.2228232467107,176.985485069079));
#18966=CARTESIAN_POINT('Ctrl Pts',(-26.0503136106968,17.0391806793695,180.985485069079));
#18967=CARTESIAN_POINT('Ctrl Pts',(-22.1433957211981,16.1797362624707,180.985485069079));
#18968=CARTESIAN_POINT('Ctrl Pts',(-22.1433957211464,16.17973626246,176.985485069079));
#18969=CARTESIAN_POINT('Ctrl Pts',(-26.3828251631526,15.5731574926212,180.985485069079));
#18970=CARTESIAN_POINT('Ctrl Pts',(-22.4878342294287,14.6609731726812,180.985485069079));
#18971=CARTESIAN_POINT('Ctrl Pts',(-22.4878342294486,14.6609731726861,176.985485069079));
#18972=CARTESIAN_POINT('Ctrl Pts',(-27.109507055406,12.6520390211126,180.985485069079));
#18973=CARTESIAN_POINT('Ctrl Pts',(-23.241113420143,11.6329387856295,180.985485069079));
#18974=CARTESIAN_POINT('Ctrl Pts',(-23.2411134201231,11.6329387856246,176.985485069079));
#18975=CARTESIAN_POINT('Ctrl Pts',(-27.5040176966898,11.1961293872236,180.985485069079));
#18976=CARTESIAN_POINT('Ctrl Pts',(-23.6503198129769,10.1228332499071,180.985485069079));
#18977=CARTESIAN_POINT('Ctrl Pts',(-23.6503198129348,10.1228332498947,176.985485069079));
#18978=CARTESIAN_POINT('Ctrl Pts',(-28.7782751940985,6.85013767399355,180.985485069079));
#18979=CARTESIAN_POINT('Ctrl Pts',(-24.97043768125,5.62042982854441,180.985485069079));
#18980=CARTESIAN_POINT('Ctrl Pts',(-24.9704376813344,5.62042982856915,176.985485069079));
#18981=CARTESIAN_POINT('Ctrl Pts',(-29.7477097626479,3.99730639154945,180.985485069079));
#18982=CARTESIAN_POINT('Ctrl Pts',(-25.9726213257473,2.67321154894945,180.985485069079));
#18983=CARTESIAN_POINT('Ctrl Pts',(-25.972621325458,2.67321154884444,176.985485069079));
#18984=CARTESIAN_POINT('Ctrl Pts',(-31.8366868970815,-1.65266278222268,
180.985485069079));
#18985=CARTESIAN_POINT('Ctrl Pts',(-28.1082275246236,-3.10287330721842,
180.985485069079));
#18986=CARTESIAN_POINT('Ctrl Pts',(-28.1082275249129,-3.10287330711342,
176.985485069079));
#18987=CARTESIAN_POINT('Ctrl Pts',(-32.9524088799731,-4.4512181944314,180.985485069079));
#18988=CARTESIAN_POINT('Ctrl Pts',(-29.2367745540547,-5.93245683765708,
180.985485069079));
#18989=CARTESIAN_POINT('Ctrl Pts',(-29.2367745537956,-5.93245683776055,
176.985485069079));
#18990=CARTESIAN_POINT('Ctrl Pts',(-35.1872819016544,-10.0470567632054,
180.985485069079));
#18991=CARTESIAN_POINT('Ctrl Pts',(-31.4735186150714,-11.5329802516063,
180.985485069079));
#18992=CARTESIAN_POINT('Ctrl Pts',(-31.4735186153305,-11.5329802515028,
176.985485069079));
#18993=CARTESIAN_POINT('Ctrl Pts',(-36.3044540496635,-12.8450741320516,
180.985485069079));
#18994=CARTESIAN_POINT('Ctrl Pts',(-32.5807344389687,-14.3063866454124,
180.985485069079));
#18995=CARTESIAN_POINT('Ctrl Pts',(-32.5807344388679,-14.3063866454508,
176.985485069079));
#18996=CARTESIAN_POINT('Ctrl Pts',(-38.4502987871715,-18.4739441657436,
180.985485069079));
#18997=CARTESIAN_POINT('Ctrl Pts',(-34.6987852921578,-19.8623491849324,
180.985485069079));
#18998=CARTESIAN_POINT('Ctrl Pts',(-34.6987852922586,-19.862349184894,176.985485069079));
#18999=CARTESIAN_POINT('Ctrl Pts',(-39.4801549046855,-21.3055854274631,
180.985485069079));
#19000=CARTESIAN_POINT('Ctrl Pts',(-35.7111108093928,-22.6461097640756,
180.985485069079));
#19001=CARTESIAN_POINT('Ctrl Pts',(-35.7111108093873,-22.6461097640774,
176.985485069079));
#19002=CARTESIAN_POINT('Ctrl Pts',(-41.4205088263372,-26.9940453161076,
180.985485069079));
#19003=CARTESIAN_POINT('Ctrl Pts',(-37.6179212387892,-28.2362315051643,
180.985485069079));
#19004=CARTESIAN_POINT('Ctrl Pts',(-37.6179212387947,-28.2362315051624,
176.985485069079));
#19005=CARTESIAN_POINT('Ctrl Pts',(-42.3326945401042,-29.8522172923435,
180.985485069079));
#19006=CARTESIAN_POINT('Ctrl Pts',(-38.5139474648075,-31.0437297254249,
180.985485069079));
#19007=CARTESIAN_POINT('Ctrl Pts',(-38.5139474648464,-31.0437297254133,
176.985485069079));
#19008=CARTESIAN_POINT('Ctrl Pts',(-44.0456869733603,-35.5953385529714,
180.985485069079));
#19009=CARTESIAN_POINT('Ctrl Pts',(-40.1981801154455,-36.6904285408454,
180.985485069079));
#19010=CARTESIAN_POINT('Ctrl Pts',(-40.1981801154065,-36.690428540857,176.985485069079));
#19011=CARTESIAN_POINT('Ctrl Pts',(-44.8469569069594,-38.4801764731839,
180.985485069079));
#19012=CARTESIAN_POINT('Ctrl Pts',(-40.986749817546,-39.5293406298925,180.985485069079));
#19013=CARTESIAN_POINT('Ctrl Pts',(-40.986749817569,-39.5293406298865,176.985485069079));
#19014=CARTESIAN_POINT('Ctrl Pts',(-47.1060660254085,-47.1694786137269,
180.985485069079));
#19015=CARTESIAN_POINT('Ctrl Pts',(-43.2125745008618,-48.0906195108081,
180.985485069079));
#19016=CARTESIAN_POINT('Ctrl Pts',(-43.2125745008157,-48.0906195108201,
176.985485069079));
#19017=CARTESIAN_POINT('Ctrl Pts',(-48.4207181977957,-53.0083673031996,
180.985485069079));
#19018=CARTESIAN_POINT('Ctrl Pts',(-44.5113064894929,-53.8571726050397,
180.985485069079));
#19019=CARTESIAN_POINT('Ctrl Pts',(-44.5113064895194,-53.8571726050551,
176.985485069079));
#19020=CARTESIAN_POINT('Ctrl Pts',(-50.7773623574713,-64.7516965919457,
180.985485069079));
#19021=CARTESIAN_POINT('Ctrl Pts',(-46.8431551177289,-65.4769439569077,
180.985485069079));
#19022=CARTESIAN_POINT('Ctrl Pts',(-46.8431551177024,-65.4769439568923,
176.985485069079));
#19023=CARTESIAN_POINT('Ctrl Pts',(-51.8193876826615,-70.6561291763739,
180.985485069079));
#19024=CARTESIAN_POINT('Ctrl Pts',(-47.8762608373712,-71.3297841813875,
180.985485069079));
#19025=CARTESIAN_POINT('Ctrl Pts',(-47.8762608373576,-71.3297841813897,
176.985485069079));
#19026=CARTESIAN_POINT('Ctrl Pts',(-53.2348917042471,-79.5482475998618,
180.985485069079));
#19027=CARTESIAN_POINT('Ctrl Pts',(-49.2810610786228,-80.1546620454955,
180.985485069079));
#19028=CARTESIAN_POINT('Ctrl Pts',(-49.2810610786295,-80.1546620454944,
176.985485069079));
#19029=CARTESIAN_POINT('Ctrl Pts',(-53.6818624435884,-82.518291930448,180.985485069079));
#19030=CARTESIAN_POINT('Ctrl Pts',(-49.7249287002307,-83.1040011999898,
180.985485069079));
#19031=CARTESIAN_POINT('Ctrl Pts',(-49.7249287002415,-83.1040011999882,
176.985485069079));
#19032=CARTESIAN_POINT('Ctrl Pts',(-54.5319871398436,-88.4613735803899,
180.985485069079));
#19033=CARTESIAN_POINT('Ctrl Pts',(-50.5695327094811,-89.0084886370079,
180.985485069079));
#19034=CARTESIAN_POINT('Ctrl Pts',(-50.5695327094702,-89.0084886370094,
176.985485069079));
#19035=CARTESIAN_POINT('Ctrl Pts',(-54.9352946649178,-91.4354154550141,
180.985485069079));
#19036=CARTESIAN_POINT('Ctrl Pts',(-50.9704223157392,-91.9646344207502,
180.985485069079));
#19037=CARTESIAN_POINT('Ctrl Pts',(-50.970422315736,-91.9646344207298,176.985485069079));
#19038=CARTESIAN_POINT('Ctrl Pts',(-56.0886961413402,-100.364039043625,
180.985485069079));
#19039=CARTESIAN_POINT('Ctrl Pts',(-52.1173300454227,-100.842989112103,
180.985485069079));
#19040=CARTESIAN_POINT('Ctrl Pts',(-52.1173300454289,-100.842989112144,
176.985485069079));
#19041=CARTESIAN_POINT('Ctrl Pts',(-56.7826622117359,-106.325075281961,
180.985485069079));
#19042=CARTESIAN_POINT('Ctrl Pts',(-52.807967153609,-106.775053587525,180.985485069079));
#19043=CARTESIAN_POINT('Ctrl Pts',(-52.8079671537057,-106.775053587484,
176.985485069079));
#19044=CARTESIAN_POINT('Ctrl Pts',(-57.4188561822461,-112.292749775204,
180.985485069079));
#19045=CARTESIAN_POINT('Ctrl Pts',(-53.4413942236179,-112.716773792997,
180.985485069079));
#19046=CARTESIAN_POINT('Ctrl Pts',(-53.4413942236179,-112.716773792997,
176.985485069079));
#19047=CARTESIAN_POINT('Ctrl Pts',(-20.3993997459139,25.9801832417458,176.985485069079));
#19048=CARTESIAN_POINT('Ctrl Pts',(-20.3993997459139,25.9801832417458,177.253460354772));
#19049=CARTESIAN_POINT('Ctrl Pts',(-20.4266849103993,25.9776057723927,177.516770554086));
#19050=CARTESIAN_POINT('Ctrl Pts',(-20.4800815464371,25.9725641538593,177.775616151056));
#19051=CARTESIAN_POINT('Ctrl Pts',(-20.4803012881147,25.9725434062281,177.776681371076));
#19052=CARTESIAN_POINT('Ctrl Pts',(-20.4805214718867,25.9725226168914,177.77774651468));
#19053=CARTESIAN_POINT('Ctrl Pts',(-20.480742097672,25.9725017858569,177.778811581889));
#19054=CARTESIAN_POINT('Ctrl Pts',(-20.5234236436048,25.9684718817652,177.984856015713));
#19055=CARTESIAN_POINT('Ctrl Pts',(-20.5835648824924,25.9627948754604,178.189817520743));
#19056=CARTESIAN_POINT('Ctrl Pts',(-20.6593131446062,25.9556471231507,178.387733685858));
#19057=CARTESIAN_POINT('Ctrl Pts',(-20.6783192713366,25.9538536683249,178.437393171253));
#19058=CARTESIAN_POINT('Ctrl Pts',(-20.6983081455396,25.9519676032949,178.486608932719));
#19059=CARTESIAN_POINT('Ctrl Pts',(-20.7192508383654,25.9499916825274,178.535286354135));
#19060=CARTESIAN_POINT('Ctrl Pts',(-20.7200499813087,25.9499162842417,178.537143814307));
#19061=CARTESIAN_POINT('Ctrl Pts',(-20.7208505133994,25.9498407552781,178.539000491351));
#19062=CARTESIAN_POINT('Ctrl Pts',(-20.721652433009,25.949765095793,178.540856379937));
#19063=CARTESIAN_POINT('Ctrl Pts',(-20.8260553070923,25.9399148968435,178.782476736931));
#19064=CARTESIAN_POINT('Ctrl Pts',(-20.9533828010123,25.9279083222768,179.011452496788));
#19065=CARTESIAN_POINT('Ctrl Pts',(-21.1034139583469,25.9137749684792,179.227886442344));
#19066=CARTESIAN_POINT('Ctrl Pts',(-21.1049105333212,25.9136339869393,179.230045391406));
#19067=CARTESIAN_POINT('Ctrl Pts',(-21.1064093715489,25.913492793354,179.232203098791));
#19068=CARTESIAN_POINT('Ctrl Pts',(-21.1079104727703,25.9133513877557,179.234359564478));
#19069=CARTESIAN_POINT('Ctrl Pts',(-21.2244365213831,25.9023744893363,179.401759618492));
#19070=CARTESIAN_POINT('Ctrl Pts',(-21.3546271641416,25.8901176743735,179.560987606355));
#19071=CARTESIAN_POINT('Ctrl Pts',(-21.4950259385074,25.8769104720021,179.708596225131));
#19072=CARTESIAN_POINT('Ctrl Pts',(-21.535526013038,25.8731006618183,179.751176084456));
#19073=CARTESIAN_POINT('Ctrl Pts',(-21.5768751842987,25.8692118004005,179.792789103293));
#19074=CARTESIAN_POINT('Ctrl Pts',(-21.61898973787,25.8652518683145,179.833352682713));
#19075=CARTESIAN_POINT('Ctrl Pts',(-21.621024213633,25.8650605713597,179.835312233799));
#19076=CARTESIAN_POINT('Ctrl Pts',(-21.623060483137,25.8648691080782,179.83726934325));
#19077=CARTESIAN_POINT('Ctrl Pts',(-21.625098537302,25.8646774793371,179.839224002025));
#19078=CARTESIAN_POINT('Ctrl Pts',(-21.7635610963668,25.8516584897863,179.972020794527));
#19079=CARTESIAN_POINT('Ctrl Pts',(-21.9114405909342,25.83776470468,180.095037456217));
#19080=CARTESIAN_POINT('Ctrl Pts',(-22.0682312152839,25.8230479395925,180.207628051587));
#19081=CARTESIAN_POINT('Ctrl Pts',(-22.124650811608,25.817752253394,180.248142693117));
#19082=CARTESIAN_POINT('Ctrl Pts',(-22.1822245235746,25.8123499802544,180.287306902747));
#19083=CARTESIAN_POINT('Ctrl Pts',(-22.2409296003261,25.8068434610663,180.325089138399));
#19084=CARTESIAN_POINT('Ctrl Pts',(-22.2431448782432,25.8066356686396,180.326514877993));
#19085=CARTESIAN_POINT('Ctrl Pts',(-22.2453617235553,25.8064277318171,180.327938621455));
#19086=CARTESIAN_POINT('Ctrl Pts',(-22.2475801350017,25.806219650729,180.329360367391));
#19087=CARTESIAN_POINT('Ctrl Pts',(-22.3925906417591,25.7926180512291,180.422295381327));
#19088=CARTESIAN_POINT('Ctrl Pts',(-22.5418509440023,25.7786290931416,180.505212509635));
#19089=CARTESIAN_POINT('Ctrl Pts',(-22.695315785544,25.76425946275,180.578485420675));
#19090=CARTESIAN_POINT('Ctrl Pts',(-22.7771613042894,25.7565958842928,180.61756316222));
#19091=CARTESIAN_POINT('Ctrl Pts',(-22.8602030711131,25.7488239991733,180.653896980504));
#19092=CARTESIAN_POINT('Ctrl Pts',(-22.9444365893079,25.7409446072073,180.687538032982));
#19093=CARTESIAN_POINT('Ctrl Pts',(-22.9463001496801,25.7407702855959,180.688282298847));
#19094=CARTESIAN_POINT('Ctrl Pts',(-22.9481643583708,25.7405959068607,180.689025272588));
#19095=CARTESIAN_POINT('Ctrl Pts',(-22.9500292139766,25.740421471109,180.689766953873));
#19096=CARTESIAN_POINT('Ctrl Pts',(-23.04271460306,25.7317518210453,180.726629335191));
#19097=CARTESIAN_POINT('Ctrl Pts',(-23.1371806620555,25.7229245611075,180.760230126284));
#19098=CARTESIAN_POINT('Ctrl Pts',(-23.2329365689234,25.7139823855379,180.790422755679));
#19099=CARTESIAN_POINT('Ctrl Pts',(-23.3296368764114,25.7049520170156,180.820913162401));
#19100=CARTESIAN_POINT('Ctrl Pts',(-23.4276518178533,25.695804527105,180.847927609303));
#19101=CARTESIAN_POINT('Ctrl Pts',(-23.5264561919686,25.6865857564093,180.871364287284));
#19102=CARTESIAN_POINT('Ctrl Pts',(-23.586216777123,25.6810098986994,180.885539667704));
#19103=CARTESIAN_POINT('Ctrl Pts',(-23.646265830258,25.6754079958158,180.898407166228));
#19104=CARTESIAN_POINT('Ctrl Pts',(-23.7064855675305,25.6697903447738,180.909953373108));
#19105=CARTESIAN_POINT('Ctrl Pts',(-23.7907662810468,25.6619281444462,180.926112901499));
#19106=CARTESIAN_POINT('Ctrl Pts',(-23.8753692960766,25.6540391323433,180.939687708742));
#19107=CARTESIAN_POINT('Ctrl Pts',(-23.9602961099603,25.6461240023457,180.950688406402));
#19108=CARTESIAN_POINT('Ctrl Pts',(-24.0490096964407,25.6378559473296,180.962179610401));
#19109=CARTESIAN_POINT('Ctrl Pts',(-24.1380773688624,25.6295593207584,180.970862622925));
#19110=CARTESIAN_POINT('Ctrl Pts',(-24.2275069672944,25.6212344136867,180.976688931065));
#19111=CARTESIAN_POINT('Ctrl Pts',(-24.311208662952,25.613442711048,180.982142068274));
#19112=CARTESIAN_POINT('Ctrl Pts',(-24.3952280469572,25.6056261751778,180.985092314052));
#19113=CARTESIAN_POINT('Ctrl Pts',(-24.4795664985897,25.5977855805591,180.985448489195));
#19114=CARTESIAN_POINT('Ctrl Pts',(-24.4853379760646,25.5972490303337,180.985472863093));
#19115=CARTESIAN_POINT('Ctrl Pts',(-24.491110943542,25.596712367858,180.985485069075));
#19116=CARTESIAN_POINT('Ctrl Pts',(-24.4968853994148,25.596175593583,180.985485069079));
#19117=CARTESIAN_POINT('Ctrl Pts',(-55.9273079477605,-112.451758781876,
176.985485069079));
#19118=CARTESIAN_POINT('Ctrl Pts',(-55.9273079477605,-112.451758781876,
174.985485069079));
#19119=CARTESIAN_POINT('Ctrl Pts',(-55.9161963178522,-112.347528635931,
176.985485069079));
#19120=CARTESIAN_POINT('Ctrl Pts',(-55.9161963178522,-112.347528635931,
174.985485069079));
#19121=CARTESIAN_POINT('Ctrl Pts',(-55.9050783560045,-112.243408267559,
176.985485069079));
#19122=CARTESIAN_POINT('Ctrl Pts',(-55.9050783560045,-112.243408267559,
174.985485069079));
#19123=CARTESIAN_POINT('Ctrl Pts',(-55.893954080246,-112.139397514846,176.985485069079));
#19124=CARTESIAN_POINT('Ctrl Pts',(-55.893954080246,-112.139397514846,174.985485069079));
#19125=CARTESIAN_POINT('',(-55.8941531222797,-112.141258553928,174.985485069079));
#19126=CARTESIAN_POINT('',(-55.9103881299845,-112.293170927494,176.98548507057));
#19127=CARTESIAN_POINT('Ctrl Pts',(-55.8941531222797,-112.141258553928,
174.985485069079));
#19128=CARTESIAN_POINT('Ctrl Pts',(-55.8985635545636,-112.182496407459,
175.225173349436));
#19129=CARTESIAN_POINT('Ctrl Pts',(-55.9022915288212,-112.217379919497,
175.466099548914));
#19130=CARTESIAN_POINT('Ctrl Pts',(-55.905634973815,-112.248674438416,175.762105987673));
#19131=CARTESIAN_POINT('Ctrl Pts',(-55.9061908793933,-112.253878190418,
175.815650974815));
#19132=CARTESIAN_POINT('Ctrl Pts',(-55.9069724331886,-112.261194689414,
175.898612699006));
#19133=CARTESIAN_POINT('Ctrl Pts',(-55.9072335279748,-112.26363902673,175.927964564546));
#19134=CARTESIAN_POINT('Ctrl Pts',(-55.90752307931,-112.266349861729,175.962609843277));
#19135=CARTESIAN_POINT('Ctrl Pts',(-55.9075666685364,-112.266757955063,
175.967886313802));
#19136=CARTESIAN_POINT('Ctrl Pts',(-55.90763270527,-112.26737621146,175.975974940967));
#19137=CARTESIAN_POINT('Ctrl Pts',(-55.907655516467,-112.267589777688,175.978786794323));
#19138=CARTESIAN_POINT('Ctrl Pts',(-55.9076972825353,-112.267980807186,
175.983968189128));
#19139=CARTESIAN_POINT('Ctrl Pts',(-55.9077162836962,-112.268158703655,
175.986339383711));
#19140=CARTESIAN_POINT('Ctrl Pts',(-55.9077553600245,-112.268524552788,
175.99123478032));
#19141=CARTESIAN_POINT('Ctrl Pts',(-55.9077767006682,-112.26872435356,175.993921954021));
#19142=CARTESIAN_POINT('Ctrl Pts',(-55.9078351002393,-112.269271118478,
176.001313380653));
#19143=CARTESIAN_POINT('Ctrl Pts',(-55.9078719345754,-112.269615981164,
176.006017771104));
#19144=CARTESIAN_POINT('Ctrl Pts',(-55.9080645843082,-112.271419680157,
176.030849218023));
#19145=CARTESIAN_POINT('Ctrl Pts',(-55.908214601632,-112.272824262972,176.050978879581));
#19146=CARTESIAN_POINT('Ctrl Pts',(-55.9087759640173,-112.278080294568,
176.129579022445));
#19147=CARTESIAN_POINT('Ctrl Pts',(-55.9091407847523,-112.281496343087,
176.188039682372));
#19148=CARTESIAN_POINT('Ctrl Pts',(-55.9107627717114,-112.296684608531,
176.493833485863));
#19149=CARTESIAN_POINT('Ctrl Pts',(-55.9110811044381,-112.299666462952,
176.738023108658));
#19150=CARTESIAN_POINT('Ctrl Pts',(-55.9103874835559,-112.293170814203,
176.985485065785));
#19151=CARTESIAN_POINT('Ctrl Pts',(-55.9273079477605,-112.451758781876,
174.985485069079));
#19152=CARTESIAN_POINT('Ctrl Pts',(-55.9162739233362,-112.348256596724,
174.985485069079));
#19153=CARTESIAN_POINT('Ctrl Pts',(-55.9052223395644,-112.244756517776,
174.985485069079));
#19154=CARTESIAN_POINT('Ctrl Pts',(-55.8941531222797,-112.141258553928,
174.985485069079));
#19155=CARTESIAN_POINT('',(-55.9103874835467,-112.293170814116,176.985485069079));
#19156=CARTESIAN_POINT('Origin',(-34.9583934096621,-20.6140499623174,173.485485069079));
#19157=CARTESIAN_POINT('',(-60.9459236613779,-101.771602184887,173.485485069079));
#19158=CARTESIAN_POINT('Origin',(-57.8714679378161,-101.961142909682,173.485484935551));
#19159=CARTESIAN_POINT('Origin',(-57.7124589446281,-100.469594673199,173.485484935556));
#19160=CARTESIAN_POINT('Origin',(-57.5534499237749,-98.9780464405567,173.485484935551));
#19161=CARTESIAN_POINT('',(-37.4541011624573,-44.0244753865006,173.485485069079));
#19162=CARTESIAN_POINT('',(-69.5889371886705,15.3762068992854,173.485485069079));
#19163=CARTESIAN_POINT('',(-62.0059837058594,-111.715257081458,173.485485069079));
#19164=CARTESIAN_POINT('Origin',(-58.5743664423751,-112.487668859306,173.485458785641));
#19165=CARTESIAN_POINT('Ctrl Pts',(-60.5242814633668,-111.628781113343,
173.485485069079));
#19166=CARTESIAN_POINT('Ctrl Pts',(-60.7715770916306,-111.628999793736,
173.485485069079));
#19167=CARTESIAN_POINT('Ctrl Pts',(-61.0198212492056,-111.638374754475,
173.485485069079));
#19168=CARTESIAN_POINT('Ctrl Pts',(-61.5077217781315,-111.668933227103,
173.485485069079));
#19169=CARTESIAN_POINT('Ctrl Pts',(-61.7598509417045,-111.690516273231,
173.485485069079));
#19170=CARTESIAN_POINT('Ctrl Pts',(-62.0059837058594,-111.715257081458,
173.485485069079));
#19171=CARTESIAN_POINT('',(-61.8999777014113,-110.7208915918,173.485485069079));
#19172=CARTESIAN_POINT('Ctrl Pts',(-61.8999777014113,-110.7208915918,173.485485069079));
#19173=CARTESIAN_POINT('Ctrl Pts',(-61.6722691809327,-110.812341651549,
173.485485069079));
#19174=CARTESIAN_POINT('Ctrl Pts',(-61.4408313059547,-110.903719063423,
173.485485070806));
#19175=CARTESIAN_POINT('Ctrl Pts',(-60.9623872716977,-111.087021812589,
173.485485070806));
#19176=CARTESIAN_POINT('Ctrl Pts',(-60.720877573809,-111.177330293225,173.485485069079));
#19177=CARTESIAN_POINT('Ctrl Pts',(-60.4851225885515,-111.26146009287,173.485485069079));
#19178=CARTESIAN_POINT('',(-61.8469746991872,-110.223708846972,173.485485069079));
#19179=CARTESIAN_POINT('Origin',(-58.8255219851367,-110.9104323152,173.485484935551));
#19180=CARTESIAN_POINT('Ctrl Pts',(-60.3652724566946,-110.137232878857,
173.485485069079));
#19181=CARTESIAN_POINT('Ctrl Pts',(-60.612568084958,-110.13745155925,173.485485069079));
#19182=CARTESIAN_POINT('Ctrl Pts',(-60.8608122425326,-110.146826519989,
173.485485069079));
#19183=CARTESIAN_POINT('Ctrl Pts',(-61.3487127714596,-110.177384992617,
173.485485069079));
#19184=CARTESIAN_POINT('Ctrl Pts',(-61.6008419350333,-110.198968038745,
173.485485069079));
#19185=CARTESIAN_POINT('Ctrl Pts',(-61.8469746991872,-110.223708846972,
173.485485069079));
#19186=CARTESIAN_POINT('',(-61.740968694739,-109.229343357315,173.485485069079));
#19187=CARTESIAN_POINT('Ctrl Pts',(-61.740968694739,-109.229343357315,173.485485069079));
#19188=CARTESIAN_POINT('Ctrl Pts',(-61.5132601742589,-109.320793417064,
173.485485069079));
#19189=CARTESIAN_POINT('Ctrl Pts',(-61.281822299282,-109.412170828938,173.485485070806));
#19190=CARTESIAN_POINT('Ctrl Pts',(-60.8033813639377,-109.595472390839,
173.485485070806));
#19191=CARTESIAN_POINT('Ctrl Pts',(-60.5618656159965,-109.685783111862,
173.485485069079));
#19192=CARTESIAN_POINT('Ctrl Pts',(-60.3261135818793,-109.769911858384,
173.485485069079));
#19193=CARTESIAN_POINT('',(-61.687965692515,-108.732160612486,173.485485069079));
#19194=CARTESIAN_POINT('Origin',(-58.6665129885927,-109.418884079281,173.485484935562));
#19195=CARTESIAN_POINT('Ctrl Pts',(-60.2062634500224,-108.645684644372,
173.485485069079));
#19196=CARTESIAN_POINT('Ctrl Pts',(-60.4535623858286,-108.645903327689,
173.485485069079));
#19197=CARTESIAN_POINT('Ctrl Pts',(-60.7017999171308,-108.655278077643,
173.485485069079));
#19198=CARTESIAN_POINT('Ctrl Pts',(-61.1897037647873,-108.685836758131,
173.485485069079));
#19199=CARTESIAN_POINT('Ctrl Pts',(-61.4418329283609,-108.70741980426,173.485485069079));
#19200=CARTESIAN_POINT('Ctrl Pts',(-61.687965692515,-108.732160612486,173.485485069079));
#19201=CARTESIAN_POINT('',(-61.5819596880668,-107.737795122829,173.485485069079));
#19202=CARTESIAN_POINT('Ctrl Pts',(-61.5819596880668,-107.737795122829,
173.485485069079));
#19203=CARTESIAN_POINT('Ctrl Pts',(-61.3542511675849,-107.829245182579,
173.485485069079));
#19204=CARTESIAN_POINT('Ctrl Pts',(-61.122813292609,-107.920622594452,173.485485070806));
#19205=CARTESIAN_POINT('Ctrl Pts',(-60.6443692583563,-108.103925343616,
173.485485070806));
#19206=CARTESIAN_POINT('Ctrl Pts',(-60.4028595604654,-108.194233824254,
173.485485069079));
#19207=CARTESIAN_POINT('Ctrl Pts',(-60.1671045752071,-108.278363623899,
173.485485069079));
#19208=CARTESIAN_POINT('',(-61.5289566858427,-107.240612378001,173.485485069079));
#19209=CARTESIAN_POINT('Origin',(-58.5075039863327,-107.927335844292,173.485484935562));
#19210=CARTESIAN_POINT('Ctrl Pts',(-60.0472544433501,-107.154136409886,
173.485485069079));
#19211=CARTESIAN_POINT('Ctrl Pts',(-60.2945500716139,-107.154355090279,
173.485485069079));
#19212=CARTESIAN_POINT('Ctrl Pts',(-60.542794229189,-107.163730051018,173.485485069079));
#19213=CARTESIAN_POINT('Ctrl Pts',(-61.0306947581148,-107.194288523646,
173.485485069079));
#19214=CARTESIAN_POINT('Ctrl Pts',(-61.282823921688,-107.215871569774,173.485485069079));
#19215=CARTESIAN_POINT('Ctrl Pts',(-61.5289566858427,-107.240612378001,
173.485485069079));
#19216=CARTESIAN_POINT('',(-61.4229506813946,-106.246246888344,173.485485069079));
#19217=CARTESIAN_POINT('Ctrl Pts',(-61.4229506813946,-106.246246888344,
173.485485069079));
#19218=CARTESIAN_POINT('Ctrl Pts',(-61.1952421609126,-106.337696948094,
173.485485069079));
#19219=CARTESIAN_POINT('Ctrl Pts',(-60.9638042859369,-106.429074359967,
173.485485070806));
#19220=CARTESIAN_POINT('Ctrl Pts',(-60.4853633505951,-106.612375921868,
173.485485070806));
#19221=CARTESIAN_POINT('Ctrl Pts',(-60.2438476026526,-106.702686642891,
173.485485069079));
#19222=CARTESIAN_POINT('Ctrl Pts',(-60.0080955685348,-106.786815389413,
173.485485069079));
#19223=CARTESIAN_POINT('',(-61.3699476791705,-105.749064143515,173.485485069079));
#19224=CARTESIAN_POINT('Origin',(-58.3484949741263,-106.435787610392,173.485484935551));
#19225=CARTESIAN_POINT('Ctrl Pts',(-59.8882454366779,-105.662588175401,
173.485485069079));
#19226=CARTESIAN_POINT('Ctrl Pts',(-60.1355410649418,-105.662806855793,
173.485485069079));
#19227=CARTESIAN_POINT('Ctrl Pts',(-60.3837852225172,-105.672181816532,
173.485485069079));
#19228=CARTESIAN_POINT('Ctrl Pts',(-60.8716857514425,-105.70274028916,173.485485069079));
#19229=CARTESIAN_POINT('Ctrl Pts',(-61.1238149150156,-105.724323335288,
173.485485069079));
#19230=CARTESIAN_POINT('Ctrl Pts',(-61.3699476791705,-105.749064143515,
173.485485069079));
#19231=CARTESIAN_POINT('',(-61.2639416747223,-104.754698653858,173.485485069079));
#19232=CARTESIAN_POINT('Ctrl Pts',(-61.2639416747223,-104.754698653858,
173.485485069079));
#19233=CARTESIAN_POINT('Ctrl Pts',(-61.0362331542402,-104.846148713608,
173.485485069079));
#19234=CARTESIAN_POINT('Ctrl Pts',(-60.8047952792646,-104.937526125481,
173.485485070806));
#19235=CARTESIAN_POINT('Ctrl Pts',(-60.3263543439242,-105.120827687381,
173.485485070806));
#19236=CARTESIAN_POINT('Ctrl Pts',(-60.0848385959808,-105.211138408405,
173.485485069079));
#19237=CARTESIAN_POINT('Ctrl Pts',(-59.8490865618626,-105.295267154927,
173.485485069079));
#19238=CARTESIAN_POINT('',(-61.2109386724983,-104.25751590903,173.485485069079));
#19239=CARTESIAN_POINT('Origin',(-58.189485943239,-104.944239379307,173.485484935551));
#19240=CARTESIAN_POINT('Ctrl Pts',(-59.7292364300057,-104.171039940915,
173.485485069079));
#19241=CARTESIAN_POINT('Ctrl Pts',(-59.9765353658119,-104.171258624233,
173.485485069079));
#19242=CARTESIAN_POINT('Ctrl Pts',(-60.2247728971142,-104.180633374186,
173.485485069079));
#19243=CARTESIAN_POINT('Ctrl Pts',(-60.7126767447704,-104.211192054675,
173.485485069079));
#19244=CARTESIAN_POINT('Ctrl Pts',(-60.9648059083435,-104.232775100803,
173.485485069079));
#19245=CARTESIAN_POINT('Ctrl Pts',(-61.2109386724983,-104.25751590903,173.485485069079));
#19246=CARTESIAN_POINT('',(-61.1049326680501,-103.263150419372,173.485485069079));
#19247=CARTESIAN_POINT('Ctrl Pts',(-61.1049326680501,-103.263150419373,
173.485485069079));
#19248=CARTESIAN_POINT('Ctrl Pts',(-60.8772241475705,-103.354600479122,
173.485485069079));
#19249=CARTESIAN_POINT('Ctrl Pts',(-60.6457862725931,-103.445977890995,
173.485485070806));
#19250=CARTESIAN_POINT('Ctrl Pts',(-60.167345337252,-103.629279452896,173.485485070806));
#19251=CARTESIAN_POINT('Ctrl Pts',(-59.9258295893085,-103.719590173919,
173.485485069079));
#19252=CARTESIAN_POINT('Ctrl Pts',(-59.6900775551904,-103.803718920442,
173.485485069079));
#19253=CARTESIAN_POINT('',(-61.0519296658261,-102.765967674544,173.485485069079));
#19254=CARTESIAN_POINT('Origin',(-58.0304769626648,-103.452691141352,173.485484935545));
#19255=CARTESIAN_POINT('Ctrl Pts',(-59.5702274233335,-102.679491706429,
173.485485069079));
#19256=CARTESIAN_POINT('Ctrl Pts',(-59.8175230515967,-102.679710386822,
173.485485069079));
#19257=CARTESIAN_POINT('Ctrl Pts',(-60.0657672091708,-102.689085347561,
173.485485069079));
#19258=CARTESIAN_POINT('Ctrl Pts',(-60.5536677380983,-102.719643820189,
173.485485069079));
#19259=CARTESIAN_POINT('Ctrl Pts',(-60.8057969016718,-102.741226866317,
173.485485069079));
#19260=CARTESIAN_POINT('Ctrl Pts',(-61.0519296658261,-102.765967674544,
173.485485069079));
#19261=CARTESIAN_POINT('',(-60.6425873069478,-101.892414120442,173.485485069077));
#19262=CARTESIAN_POINT('Ctrl Pts',(-60.642587306948,-101.892414120443,173.485485069079));
#19263=CARTESIAN_POINT('Ctrl Pts',(-60.4342503547387,-101.974634832253,
173.485485069079));
#19264=CARTESIAN_POINT('Ctrl Pts',(-60.2480095641541,-102.046444777389,
173.485485069079));
#19265=CARTESIAN_POINT('Ctrl Pts',(-59.8845339623614,-102.183752672436,
173.485485069079));
#19266=CARTESIAN_POINT('Ctrl Pts',(-59.7067146857557,-102.249490890159,
173.485485069079));
#19267=CARTESIAN_POINT('Ctrl Pts',(-59.5310685485181,-102.312170685956,
173.485485069079));
#19268=CARTESIAN_POINT('',(-60.9552496185426,-101.859082229163,173.485485069079));
#19269=CARTESIAN_POINT('',(-43.8144614293464,-103.686404765925,173.485485069079));
#19270=CARTESIAN_POINT('',(-54.5948893516535,-42.1971528497386,173.485485069079));
#19271=CARTESIAN_POINT('Ctrl Pts',(-57.259519543175,-112.30973612544,173.494068527883));
#19272=CARTESIAN_POINT('Ctrl Pts',(-55.9273079477605,-112.451758781876,
173.638013937363));
#19273=CARTESIAN_POINT('Ctrl Pts',(-55.9273079477605,-112.451758781876,
174.985485069079));
#19274=CARTESIAN_POINT('Ctrl Pts',(-57.2437226572379,-112.161556988779,
173.494068527878));
#19275=CARTESIAN_POINT('Ctrl Pts',(-55.9115340572459,-112.303795348611,
173.638013937322));
#19276=CARTESIAN_POINT('Ctrl Pts',(-55.9115340572464,-112.303795348611,
174.985485069038));
#19277=CARTESIAN_POINT('Ctrl Pts',(-57.2278898065789,-112.013381908907,
173.494068527883));
#19278=CARTESIAN_POINT('Ctrl Pts',(-55.8957243236821,-112.155836616448,
173.638013937363));
#19279=CARTESIAN_POINT('Ctrl Pts',(-55.8957243236832,-112.155836616448,
174.985485069079));
#19280=CARTESIAN_POINT('Ctrl Pts',(-57.2120207737176,-111.865210910606,
173.494068527883));
#19281=CARTESIAN_POINT('Ctrl Pts',(-55.879878531177,-112.007882616058,173.638013937363));
#19282=CARTESIAN_POINT('Ctrl Pts',(-55.879878531177,-112.007882616058,174.985485069079));
#19283=CARTESIAN_POINT('Ctrl Pts',(-57.2413645753253,-112.263285154288,
173.495537439996));
#19284=CARTESIAN_POINT('Ctrl Pts',(-57.2033140047626,-112.275892356383,
173.500095525992));
#19285=CARTESIAN_POINT('Ctrl Pts',(-57.1653918170167,-112.288244330645,
173.506200883917));
#19286=CARTESIAN_POINT('Ctrl Pts',(-57.0899544352199,-112.312424168425,
173.521506336905));
#19287=CARTESIAN_POINT('Ctrl Pts',(-57.0524790264818,-112.324239249128,
173.530698662253));
#19288=CARTESIAN_POINT('Ctrl Pts',(-57.0153382075498,-112.335767487168,
173.541420416595));
#19289=CARTESIAN_POINT('Ctrl Pts',(-55.8941531223023,-112.141258553931,
174.985485069071));
#19290=CARTESIAN_POINT('Ctrl Pts',(-55.8916773175805,-112.118109604864,
174.850935587984));
#19291=CARTESIAN_POINT('Ctrl Pts',(-55.9075132742012,-112.095933400872,
174.716548833312));
#19292=CARTESIAN_POINT('Ctrl Pts',(-55.9811754973074,-112.050187383497,
174.433829597845));
#19293=CARTESIAN_POINT('Ctrl Pts',(-56.0450398693184,-112.027296731103,
174.288799639065));
#19294=CARTESIAN_POINT('Ctrl Pts',(-56.1432872646253,-112.003471991653,
174.137658259513));
#19295=CARTESIAN_POINT('Ctrl Pts',(-56.1559725791695,-112.000546571712,
174.119092857142));
#19296=CARTESIAN_POINT('Ctrl Pts',(-56.1964158282439,-111.991665771564,
174.062734827425));
#19297=CARTESIAN_POINT('Ctrl Pts',(-56.2255745057671,-111.985870655016,
174.025962079021));
#19298=CARTESIAN_POINT('Ctrl Pts',(-56.3847089020071,-111.957140194668,
173.843960050512));
#19299=CARTESIAN_POINT('Ctrl Pts',(-56.5410272906302,-111.938298267507,
173.724180636921));
#19300=CARTESIAN_POINT('Ctrl Pts',(-56.8689932673701,-111.910937177978,
173.563255743881));
#19301=CARTESIAN_POINT('Ctrl Pts',(-57.0332189978765,-111.901459989199,
173.515132800414));
#19302=CARTESIAN_POINT('Ctrl Pts',(-57.2022249863543,-111.895960177099,
173.495524270213));
#19303=CARTESIAN_POINT('Origin',(-57.4101169644616,-112.210813934705,176.985487255437));
#19304=CARTESIAN_POINT('Ctrl Pts',(-57.0153371209007,-112.335767603012,
178.42954834513));
#19305=CARTESIAN_POINT('Ctrl Pts',(-56.8473564372785,-112.320853466685,
178.38305319844));
#19306=CARTESIAN_POINT('Ctrl Pts',(-56.6884637490847,-112.310226558581,
178.308320841682));
#19307=CARTESIAN_POINT('Ctrl Pts',(-56.4556453066853,-112.297678205632,
178.144602855094));
#19308=CARTESIAN_POINT('Ctrl Pts',(-56.3728898125372,-112.293947382744,
178.071756401203));
#19309=CARTESIAN_POINT('Ctrl Pts',(-56.2709933701936,-112.290154253653,
177.959937124381));
#19310=CARTESIAN_POINT('Ctrl Pts',(-56.2444363725251,-112.28925807319,177.928257007469));
#19311=CARTESIAN_POINT('Ctrl Pts',(-56.2046433208664,-112.288053998207,
177.876578050907));
#19312=CARTESIAN_POINT('Ctrl Pts',(-56.1905182651179,-112.287657594759,
177.857294323186));
#19313=CARTESIAN_POINT('Ctrl Pts',(-56.1744975949982,-112.287243742126,
177.834282953652));
#19314=CARTESIAN_POINT('Ctrl Pts',(-56.1721473696133,-112.287183975266,
177.830877075062));
#19315=CARTESIAN_POINT('Ctrl Pts',(-56.1684117420286,-112.287090485813,
177.825415042612));
#19316=CARTESIAN_POINT('Ctrl Pts',(-56.1670172505921,-112.287055927343,
177.823365146775));
#19317=CARTESIAN_POINT('Ctrl Pts',(-56.1645609823913,-112.286995657481,
177.819735019072));
#19318=CARTESIAN_POINT('Ctrl Pts',(-56.1634971100675,-112.286969754496,
177.818156215516));
#19319=CARTESIAN_POINT('Ctrl Pts',(-56.1613001770806,-112.286916680793,
177.814882425266));
#19320=CARTESIAN_POINT('Ctrl Pts',(-56.160167562911,-112.286889550508,177.813187143314));
#19321=CARTESIAN_POINT('Ctrl Pts',(-56.1572702675728,-112.286820743249,
177.808831200865));
#19322=CARTESIAN_POINT('Ctrl Pts',(-56.1555106437809,-112.286779523379,
177.806167182541));
#19323=CARTESIAN_POINT('Ctrl Pts',(-56.1483293226769,-112.286613629846,
177.795218581503));
#19324=CARTESIAN_POINT('Ctrl Pts',(-56.1429816031708,-112.286495587941,
177.786885698674));
#19325=CARTESIAN_POINT('Ctrl Pts',(-56.1089735505856,-112.285780346088,
177.732713914608));
#19326=CARTESIAN_POINT('Ctrl Pts',(-56.0827423503488,-112.285394420431,
177.685398052236));
#19327=CARTESIAN_POINT('Ctrl Pts',(-56.0139383163625,-112.284873827523,
177.543566166655));
#19328=CARTESIAN_POINT('Ctrl Pts',(-55.9786013530088,-112.285290965373,
177.445922321661));
#19329=CARTESIAN_POINT('Ctrl Pts',(-55.9245999086427,-112.287723313926,
177.227616441256));
#19330=CARTESIAN_POINT('Ctrl Pts',(-55.9100488748278,-112.289987551767,
177.106767079342));
#19331=CARTESIAN_POINT('Ctrl Pts',(-55.9103887977622,-112.293171089531,
176.985485076695));
#19332=CARTESIAN_POINT('Origin',(-69.5889371886705,15.3762068992854,178.485485069079));
#19333=CARTESIAN_POINT('Origin',(-53.4413942236179,-112.716773792997,178.485485069079));
#19334=CARTESIAN_POINT('',(-37.1738630900728,31.4290895869696,178.485485069079));
#19335=CARTESIAN_POINT('Origin',(-44.1060283439209,41.4682670878081,178.485485069079));
#19336=CARTESIAN_POINT('',(-41.1020539958444,25.42062214227,178.485485069079));
#19337=CARTESIAN_POINT('Origin',(-31.7758655563387,23.6116972707429,178.485485069079));
#19338=CARTESIAN_POINT('Origin',(-36.6843857876575,24.5637629925993,178.485485069079));
#19339=CARTESIAN_POINT('',(-26.3222158483506,41.9802195673193,178.485485069079));
#19340=CARTESIAN_POINT('Origin',(-60.1632027754914,33.6789365837495,178.485485069079));
#19341=CARTESIAN_POINT('',(-31.0667656272414,60.393115748013,179.845797336032));
#19342=CARTESIAN_POINT('',(-31.066765828848,60.3931158153939,172.125173944189));
#19343=CARTESIAN_POINT('',(-31.0667661651747,60.3931159007681,178.485485069079));
#19344=CARTESIAN_POINT('',(-28.9197092925293,57.8469757052857,178.485485069079));
#19345=CARTESIAN_POINT('Ctrl Pts',(-31.0667654102549,60.3931159213539,179.845797430829));
#19346=CARTESIAN_POINT('Ctrl Pts',(-30.9091769682086,60.2214795244379,179.79892929946));
#19347=CARTESIAN_POINT('Ctrl Pts',(-30.7556527061396,60.0512411160334,179.742114967035));
#19348=CARTESIAN_POINT('Ctrl Pts',(-30.6059165456662,59.8823450585327,179.676490357673));
#19349=CARTESIAN_POINT('Ctrl Pts',(-30.4442591103229,59.7000023070635,179.605641031689));
#19350=CARTESIAN_POINT('Ctrl Pts',(-30.2870169389526,59.5192241310761,179.524523032668));
#19351=CARTESIAN_POINT('Ctrl Pts',(-30.1338194315574,59.3399324111494,179.434622622711));
#19352=CARTESIAN_POINT('Ctrl Pts',(-30.0717866024173,59.267333497384,179.398220093288));
#19353=CARTESIAN_POINT('Ctrl Pts',(-30.010416692512,59.1949782192853,179.360378177063));
#19354=CARTESIAN_POINT('Ctrl Pts',(-29.949684172152,59.1228610766146,179.321197665583));
#19355=CARTESIAN_POINT('Ctrl Pts',(-29.9426383506173,59.1144944797101,179.316652178422));
#19356=CARTESIAN_POINT('Ctrl Pts',(-29.9356009897824,59.106130933026,179.312088584704));
#19357=CARTESIAN_POINT('Ctrl Pts',(-29.9285720599821,59.0977704247621,179.307506991655));
#19358=CARTESIAN_POINT('Ctrl Pts',(-29.6522634383716,58.7691171902053,179.127403662113));
#19359=CARTESIAN_POINT('Ctrl Pts',(-29.3887247237273,58.4448506261122,178.919335958335));
#19360=CARTESIAN_POINT('Ctrl Pts',(-29.1356651950541,58.1236205383787,178.68935857041));
#19361=CARTESIAN_POINT('Ctrl Pts',(-29.0628302196002,58.0311648791201,178.623167040329));
#19362=CARTESIAN_POINT('Ctrl Pts',(-28.9908632147143,57.9389607063399,178.55516084433));
#19363=CARTESIAN_POINT('Ctrl Pts',(-28.9197092925293,57.8469757052856,178.485485069079));
#19364=CARTESIAN_POINT('',(-27.6932740952942,56.17235187585,177.985895857994));
#19365=CARTESIAN_POINT('Ctrl Pts',(-28.9197092925293,57.8469757052856,178.485485069079));
#19366=CARTESIAN_POINT('Ctrl Pts',(-28.8695639852542,57.7821498179569,178.4363815229));
#19367=CARTESIAN_POINT('Ctrl Pts',(-28.8180944967583,57.7151863974902,178.393590440407));
#19368=CARTESIAN_POINT('Ctrl Pts',(-28.765769451896,57.6466415487446,178.35528260832));
#19369=CARTESIAN_POINT('Ctrl Pts',(-28.7186055717574,57.5848577310937,178.320753330693));
#19370=CARTESIAN_POINT('Ctrl Pts',(-28.6707461547263,57.5217885156425,178.289868104488));
#19371=CARTESIAN_POINT('Ctrl Pts',(-28.6225281965413,57.4578315766418,178.261313090149));
#19372=CARTESIAN_POINT('Ctrl Pts',(-28.6223170910684,57.4575515635438,178.261188072002));
#19373=CARTESIAN_POINT('Ctrl Pts',(-28.6221059794197,57.4572715343512,178.261063099026));
#19374=CARTESIAN_POINT('Ctrl Pts',(-28.6218948616221,57.4569914890959,178.260938171111));
#19375=CARTESIAN_POINT('Ctrl Pts',(-28.5576206106114,57.3717324572002,178.222904200128));
#19376=CARTESIAN_POINT('Ctrl Pts',(-28.4924136963644,57.2845038762807,178.18938357879));
#19377=CARTESIAN_POINT('Ctrl Pts',(-28.4269389977876,57.1961490995419,178.159893050851));
#19378=CARTESIAN_POINT('Ctrl Pts',(-28.3890105999134,57.1449666550392,178.142809681222));
#19379=CARTESIAN_POINT('Ctrl Pts',(-28.3509920646441,57.0934057548245,178.12707974697));
#19380=CARTESIAN_POINT('Ctrl Pts',(-28.313012572032,57.0416287203634,178.112616869885));
#19381=CARTESIAN_POINT('Ctrl Pts',(-28.3124798542368,57.0409024719134,178.112414006933));
#19382=CARTESIAN_POINT('Ctrl Pts',(-28.3119471450267,57.0401761821527,178.112211393752));
#19383=CARTESIAN_POINT('Ctrl Pts',(-28.3114144448134,57.0394498516033,178.11200903013));
#19384=CARTESIAN_POINT('Ctrl Pts',(-28.1791184150512,56.8590657526497,178.061752050421));
#19385=CARTESIAN_POINT('Ctrl Pts',(-28.0471800611791,56.6759576351996,178.026148692935));
#19386=CARTESIAN_POINT('Ctrl Pts',(-27.9156412222414,56.4900036591952,178.005762137669));
#19387=CARTESIAN_POINT('Ctrl Pts',(-27.8413887382427,56.3850343228436,177.994254111744));
#19388=CARTESIAN_POINT('Ctrl Pts',(-27.7672636383413,56.2791580302122,177.987595826179));
#19389=CARTESIAN_POINT('Ctrl Pts',(-27.6932740952942,56.1723518758501,177.985895857994));
#19390=CARTESIAN_POINT('Ctrl Pts',(-27.6932740952942,56.17235187585,177.985895857994));
#19391=CARTESIAN_POINT('Ctrl Pts',(-27.681334674434,56.1551169589298,177.985621541128));
#19392=CARTESIAN_POINT('Ctrl Pts',(-27.6694076934204,56.137870682049,177.985485069079));
#19393=CARTESIAN_POINT('Ctrl Pts',(-27.6574947146374,56.1206152968612,177.985485069079));
#19394=CARTESIAN_POINT('',(-27.6932740952942,56.1723518758501,173.985074280165));
#19395=CARTESIAN_POINT('Ctrl Pts',(-27.6574947146374,56.1206152968612,173.985485069079));
#19396=CARTESIAN_POINT('Ctrl Pts',(-27.6694076934205,56.137870682049,173.985485069079));
#19397=CARTESIAN_POINT('Ctrl Pts',(-27.681334674434,56.1551169589298,173.985348597031));
#19398=CARTESIAN_POINT('Ctrl Pts',(-27.6932740952942,56.1723518758501,173.985074280165));
#19399=CARTESIAN_POINT('',(-28.9197092925293,57.8469757052857,173.485485069079));
#19400=CARTESIAN_POINT('Ctrl Pts',(-27.6932740952942,56.1723518758501,173.985074280165));
#19401=CARTESIAN_POINT('Ctrl Pts',(-27.8243471320476,56.3615597884776,173.98206277363));
#19402=CARTESIAN_POINT('Ctrl Pts',(-27.9558453121505,56.547849976542,173.963493852483));
#19403=CARTESIAN_POINT('Ctrl Pts',(-28.0877242229479,56.7313482308063,173.929959739527));
#19404=CARTESIAN_POINT('Ctrl Pts',(-28.1621686748946,56.8349313351047,173.91103003617));
#19405=CARTESIAN_POINT('Ctrl Pts',(-28.236734533152,56.9376246600296,173.887330718302));
#19406=CARTESIAN_POINT('Ctrl Pts',(-28.3114144448134,57.0394498516033,173.858961108029));
#19407=CARTESIAN_POINT('Ctrl Pts',(-28.3119471450267,57.0401761821527,173.858758744407));
#19408=CARTESIAN_POINT('Ctrl Pts',(-28.3124798542368,57.0409024719135,173.858556131226));
#19409=CARTESIAN_POINT('Ctrl Pts',(-28.313012572032,57.0416287203635,173.858353268274));
#19410=CARTESIAN_POINT('Ctrl Pts',(-28.3785754740065,57.1310099206225,173.833386420974));
#19411=CARTESIAN_POINT('Ctrl Pts',(-28.4442544486703,57.2197472411231,173.80464629479));
#19412=CARTESIAN_POINT('Ctrl Pts',(-28.5093860560218,57.3070049527639,173.77167881297));
#19413=CARTESIAN_POINT('Ctrl Pts',(-28.5471157068459,57.3575518857476,173.752581302127));
#19414=CARTESIAN_POINT('Ctrl Pts',(-28.5846618629718,57.4076023578408,173.732064410334));
#19415=CARTESIAN_POINT('Ctrl Pts',(-28.6218948616218,57.4569914890955,173.710031967047));
#19416=CARTESIAN_POINT('Ctrl Pts',(-28.6221059794194,57.4572715343509,173.709907039132));
#19417=CARTESIAN_POINT('Ctrl Pts',(-28.6223170910682,57.4575515635435,173.709782066156));
#19418=CARTESIAN_POINT('Ctrl Pts',(-28.622528196541,57.4578315766415,173.709657048009));
#19419=CARTESIAN_POINT('Ctrl Pts',(-28.6793546949681,57.5332069975494,173.676003995527));
#19420=CARTESIAN_POINT('Ctrl Pts',(-28.7356833945105,57.6073497472281,173.639115263873));
#19421=CARTESIAN_POINT('Ctrl Pts',(-28.7909620326999,57.6796078112931,173.596837451893));
#19422=CARTESIAN_POINT('Ctrl Pts',(-28.8346253447626,57.7366827773859,173.563443190417));
#19423=CARTESIAN_POINT('Ctrl Pts',(-28.8776335649023,57.7925818541628,173.526686679897));
#19424=CARTESIAN_POINT('Ctrl Pts',(-28.9197092925293,57.8469757052856,173.485485069079));
#19425=CARTESIAN_POINT('Ctrl Pts',(-28.9197092925293,57.8469757052857,173.485485069079));
#19426=CARTESIAN_POINT('Ctrl Pts',(-29.0790134324243,58.0529178519195,173.329490304359));
#19427=CARTESIAN_POINT('Ctrl Pts',(-29.2423834600949,58.2599171593523,173.181896823521));
#19428=CARTESIAN_POINT('Ctrl Pts',(-29.410398257058,58.4683499340291,173.044312541129));
#19429=CARTESIAN_POINT('Ctrl Pts',(-29.5682295040916,58.6641493835094,172.915067383829));
#19430=CARTESIAN_POINT('Ctrl Pts',(-29.7301598671435,58.8612136717954,172.79465486008));
#19431=CARTESIAN_POINT('Ctrl Pts',(-29.8967040919158,59.0598163446466,172.684407875314));
#19432=CARTESIAN_POINT('Ctrl Pts',(-29.9074498185088,59.0726305387503,172.677294545761));
#19433=CARTESIAN_POINT('Ctrl Pts',(-29.9182147646746,59.0854511235265,172.670223535932));
#19434=CARTESIAN_POINT('Ctrl Pts',(-29.9289990735725,59.0982781667031,172.663195203856));
#19435=CARTESIAN_POINT('Ctrl Pts',(-30.0800102141939,59.2778934243173,172.564778471406));
#19436=CARTESIAN_POINT('Ctrl Pts',(-30.2348076625985,59.4587693147239,172.474706081542));
#19437=CARTESIAN_POINT('Ctrl Pts',(-30.3939297630228,59.6412243163263,172.394408698027));
#19438=CARTESIAN_POINT('Ctrl Pts',(-30.5498223183852,59.8199762078775,172.315741031677));
#19439=CARTESIAN_POINT('Ctrl Pts',(-30.7098658175238,60.0002439081216,172.246455610862));
#19440=CARTESIAN_POINT('Ctrl Pts',(-30.8745987125149,60.1822886744227,172.187897745043));
#19441=CARTESIAN_POINT('Ctrl Pts',(-30.9379500098726,60.25229759476,172.165378157985));
#19442=CARTESIAN_POINT('Ctrl Pts',(-31.0019951796934,60.3225689131167,172.14444511125));
#19443=CARTESIAN_POINT('Ctrl Pts',(-31.0667661288183,60.3931158611695,172.125175120043));
#19444=CARTESIAN_POINT('Origin',(-13.1705752052125,56.1246475259002,178.485485069079));
#19445=CARTESIAN_POINT('',(-34.8117175582729,61.2863342745896,179.985485069079));
#19446=CARTESIAN_POINT('',(-31.0975708454296,60.4004632081127,179.985485069769));
#19447=CARTESIAN_POINT('',(-13.1705752052126,56.1246475259002,179.985485069079));
#19448=CARTESIAN_POINT('Ctrl Pts',(-31.0975708439929,60.4004632071099,179.985485070495));
#19449=CARTESIAN_POINT('Ctrl Pts',(-31.0877379564735,60.3981179388064,179.962800941576));
#19450=CARTESIAN_POINT('Ctrl Pts',(-31.0798430692015,60.3962349080896,179.939231997035));
#19451=CARTESIAN_POINT('Ctrl Pts',(-31.0694893305528,60.3937654101902,179.892276273643));
#19452=CARTESIAN_POINT('Ctrl Pts',(-31.0667653038197,60.393115695324,179.869118012909));
#19453=CARTESIAN_POINT('Ctrl Pts',(-31.0667651743783,60.3931156644506,179.845797336034));
#19454=CARTESIAN_POINT('',(-31.0975708454298,60.4004632081127,171.98548506839));
#19455=CARTESIAN_POINT('Ctrl Pts',(-31.0667651743779,60.3931156644505,172.125172868157));
#19456=CARTESIAN_POINT('Ctrl Pts',(-31.0667652986773,60.3931156940975,172.101852061251));
#19457=CARTESIAN_POINT('Ctrl Pts',(-31.0694893609766,60.3937654174737,172.078693606888));
#19458=CARTESIAN_POINT('Ctrl Pts',(-31.0798431515216,60.3962349277511,172.031737895439));
#19459=CARTESIAN_POINT('Ctrl Pts',(-31.0877380076616,60.3981179510155,172.008169078495));
#19460=CARTESIAN_POINT('Ctrl Pts',(-31.0975708439932,60.4004632071099,171.985485067664));
#19461=CARTESIAN_POINT('',(-34.8117175582729,61.2863342745896,171.985485069079));
#19462=CARTESIAN_POINT('',(-13.1705752052126,56.1246475259002,171.985485069079));
#19463=CARTESIAN_POINT('',(-34.8117175582729,61.2863342745896,178.485485069079));
#19464=CARTESIAN_POINT('Origin',(-13.5112392801691,-107.683134251892,178.485485069079));
#19465=CARTESIAN_POINT('',(-34.5615750673481,59.3020387486575,171.985485069079));
#19466=CARTESIAN_POINT('',(-34.5615750673481,59.3020387486575,179.985485069079));
#19467=CARTESIAN_POINT('',(-34.5615750673481,59.3020387486575,165.645237852233));
#19468=CARTESIAN_POINT('',(-13.511239280169,-107.683134251892,179.985485069079));
#19469=CARTESIAN_POINT('',(-13.511239280169,-107.683134251892,171.985485069079));
#19470=CARTESIAN_POINT('Origin',(-44.1060283439209,41.4682670878081,178.485485069079));
#19471=CARTESIAN_POINT('',(-33.3398524910169,36.8879333106141,171.985485068901));
#19472=CARTESIAN_POINT('',(-32.4060870603391,41.4312001114371,171.985485069079));
#19473=CARTESIAN_POINT('Origin',(-44.1060283439209,41.4682670878081,171.985485069079));
#19474=CARTESIAN_POINT('',(-33.7101944105682,36.1001541204655,173.485485069079));
#19475=CARTESIAN_POINT('Ctrl Pts',(-33.3398524911435,36.8879333109887,171.985485069079));
#19476=CARTESIAN_POINT('Ctrl Pts',(-33.4532592756956,36.621368155505,172.485877932252));
#19477=CARTESIAN_POINT('Ctrl Pts',(-33.5767107475439,36.3586572484842,172.985815014066));
#19478=CARTESIAN_POINT('Ctrl Pts',(-33.7101944105682,36.1001541204655,173.485485069079));
#19479=CARTESIAN_POINT('',(-34.1412494001895,35.3369392868692,173.985485069079));
#19480=CARTESIAN_POINT('Ctrl Pts',(-33.7101944105682,36.1001541204655,173.485485069079));
#19481=CARTESIAN_POINT('Ctrl Pts',(-33.7173223371263,36.0863502491167,173.512167058454));
#19482=CARTESIAN_POINT('Ctrl Pts',(-33.7250068081281,36.0715415783123,173.53788693616));
#19483=CARTESIAN_POINT('Ctrl Pts',(-33.7332256693475,36.0557977306796,173.56269943543));
#19484=CARTESIAN_POINT('Ctrl Pts',(-33.7415673687971,36.0398185771658,173.587882779689));
#19485=CARTESIAN_POINT('Ctrl Pts',(-33.7504597671664,36.0228754836816,173.612131975538));
#19486=CARTESIAN_POINT('Ctrl Pts',(-33.7599017013052,36.0050016280506,173.635474291225));
#19487=CARTESIAN_POINT('Ctrl Pts',(-33.7672835911654,35.9910274960872,173.65372377284));
#19488=CARTESIAN_POINT('Ctrl Pts',(-33.7750018538206,35.9764835561052,173.671418424909));
#19489=CARTESIAN_POINT('Ctrl Pts',(-33.7830638223894,35.9613727471357,173.688555375548));
#19490=CARTESIAN_POINT('Ctrl Pts',(-33.7891998689,35.9498717562971,173.701598483478));
#19491=CARTESIAN_POINT('Ctrl Pts',(-33.7955340084333,35.9380444037457,173.714314450847));
#19492=CARTESIAN_POINT('Ctrl Pts',(-33.80205321792,35.9259228315441,173.726665343328));
#19493=CARTESIAN_POINT('Ctrl Pts',(-33.8040994034126,35.9221182314254,173.730541920246));
#19494=CARTESIAN_POINT('Ctrl Pts',(-33.8061638904978,35.9182845158034,173.734382709747));
#19495=CARTESIAN_POINT('Ctrl Pts',(-33.8082463328237,35.9144225718301,173.738186738285));
#19496=CARTESIAN_POINT('Ctrl Pts',(-33.8216183462776,35.889623821763,173.762613595228));
#19497=CARTESIAN_POINT('Ctrl Pts',(-33.8357333107594,35.8636566094212,173.785523526798));
#19498=CARTESIAN_POINT('Ctrl Pts',(-33.8504811981783,35.8367881814026,173.80666357432));
#19499=CARTESIAN_POINT('Ctrl Pts',(-33.8619180624397,35.8159519385266,173.823057505676));
#19500=CARTESIAN_POINT('Ctrl Pts',(-33.8737350879047,35.7945745828219,173.838387610758));
#19501=CARTESIAN_POINT('Ctrl Pts',(-33.8858739421569,35.7727914017629,173.852553342878));
#19502=CARTESIAN_POINT('Ctrl Pts',(-33.8864939107968,35.7716788676759,173.853276830407));
#19503=CARTESIAN_POINT('Ctrl Pts',(-33.887114918358,35.7705649165669,173.853997532403));
#19504=CARTESIAN_POINT('Ctrl Pts',(-33.8877369560626,35.7694495689522,173.854715427453));
#19505=CARTESIAN_POINT('Ctrl Pts',(-33.9011175249542,35.7454574773375,173.870157970747));
#19506=CARTESIAN_POINT('Ctrl Pts',(-33.9150376519582,35.7207195066863,173.884371926662));
#19507=CARTESIAN_POINT('Ctrl Pts',(-33.9293809697622,35.6954582180761,173.89723673113));
#19508=CARTESIAN_POINT('Ctrl Pts',(-33.9342982268056,35.6867980007511,173.901647115899));
#19509=CARTESIAN_POINT('Ctrl Pts',(-33.9392650649815,35.6780764980385,173.905899303386));
#19510=CARTESIAN_POINT('Ctrl Pts',(-33.9442763474657,35.6693032844709,173.909989611581));
#19511=CARTESIAN_POINT('Ctrl Pts',(-33.9595076554056,35.642637951217,173.922421707334));
#19512=CARTESIAN_POINT('Ctrl Pts',(-33.9751531092322,35.6154891438031,173.933361803908));
#19513=CARTESIAN_POINT('Ctrl Pts',(-33.9910791468951,35.588102646381,173.942754134747));
#19514=CARTESIAN_POINT('Ctrl Pts',(-33.9982885995841,35.5757052339386,173.947005886893));
#19515=CARTESIAN_POINT('Ctrl Pts',(-34.0055541831447,35.5632613568449,173.950940413097));
#19516=CARTESIAN_POINT('Ctrl Pts',(-34.0128674167925,35.5507867018521,173.954557379261));
#19517=CARTESIAN_POINT('Ctrl Pts',(-34.0279475134156,35.5250636070225,173.962015666779));
#19518=CARTESIAN_POINT('Ctrl Pts',(-34.0432386359242,35.4991945765188,173.968132509407));
#19519=CARTESIAN_POINT('Ctrl Pts',(-34.0587493304729,35.4731802876461,173.972914111171));
#19520=CARTESIAN_POINT('Ctrl Pts',(-34.0739448242849,35.4476946484089,173.977598543567));
#19521=CARTESIAN_POINT('Ctrl Pts',(-34.0893515965258,35.4220686096455,173.98100154487));
#19522=CARTESIAN_POINT('Ctrl Pts',(-34.1049834076364,35.3963015527894,173.983080513186));
#19523=CARTESIAN_POINT('Ctrl Pts',(-34.1169386417112,35.3765948665997,173.984670511471));
#19524=CARTESIAN_POINT('Ctrl Pts',(-34.1290254559346,35.35680593016,173.985485066055));
#19525=CARTESIAN_POINT('Ctrl Pts',(-34.1412494001895,35.3369392868692,173.985485069079));
#19526=CARTESIAN_POINT('',(-37.4579682234273,31.8405312878237,173.985485069079));
#19527=CARTESIAN_POINT('Origin',(-44.1060283439209,41.4682670878081,173.985485069079));
#19528=CARTESIAN_POINT('',(-37.4579682234273,31.8405312878237,177.985485069079));
#19529=CARTESIAN_POINT('',(-37.4579682234273,31.8405312878237,178.485485069079));
#19530=CARTESIAN_POINT('',(-34.1412494001895,35.3369392868692,177.985485069079));
#19531=CARTESIAN_POINT('Origin',(-44.1060283439209,41.4682670878081,177.985485069079));
#19532=CARTESIAN_POINT('',(-33.7101944105682,36.1001541204655,178.485485069079));
#19533=CARTESIAN_POINT('Ctrl Pts',(-34.1412494001895,35.3369392868692,177.985485069079));
#19534=CARTESIAN_POINT('Ctrl Pts',(-34.1216095524896,35.3688584318198,177.98548506929));
#19535=CARTESIAN_POINT('Ctrl Pts',(-34.1022530974808,35.4006888588025,177.987571320185));
#19536=CARTESIAN_POINT('Ctrl Pts',(-34.0832209590391,35.4323178174378,177.991637372604));
#19537=CARTESIAN_POINT('Ctrl Pts',(-34.0638728223472,35.4644719243962,177.995770935327));
#19538=CARTESIAN_POINT('Ctrl Pts',(-34.0448594190002,35.496418670158,178.001950696189));
#19539=CARTESIAN_POINT('Ctrl Pts',(-34.026224496512,35.5280487026682,178.010118542669));
#19540=CARTESIAN_POINT('Ctrl Pts',(-34.0212915827807,35.5364215961852,178.012280681099));
#19541=CARTESIAN_POINT('Ctrl Pts',(-34.0163852148609,35.544772305989,178.014582413863));
#19542=CARTESIAN_POINT('Ctrl Pts',(-34.0115062740386,35.5530987904069,178.017023265722));
#19543=CARTESIAN_POINT('Ctrl Pts',(-34.007479623835,35.5599707409795,178.01903773095));
#19544=CARTESIAN_POINT('Ctrl Pts',(-34.0034718839124,35.5668257850579,178.021146733784));
#19545=CARTESIAN_POINT('Ctrl Pts',(-33.999477173576,35.5736737697792,178.023353970292));
#19546=CARTESIAN_POINT('Ctrl Pts',(-33.9833988783172,35.6012361988427,178.032237868573));
#19547=CARTESIAN_POINT('Ctrl Pts',(-33.9675632094865,35.6286311820355,178.042702346422));
#19548=CARTESIAN_POINT('Ctrl Pts',(-33.9521138058932,35.6555970548587,178.054698671223));
#19549=CARTESIAN_POINT('Ctrl Pts',(-33.9494502518773,35.6602461054461,178.056766897282));
#19550=CARTESIAN_POINT('Ctrl Pts',(-33.9467981555019,35.6648824218227,178.058880533764));
#19551=CARTESIAN_POINT('Ctrl Pts',(-33.9441582204118,35.6695046945796,178.061039180225));
#19552=CARTESIAN_POINT('Ctrl Pts',(-33.9297962098085,35.6946511955657,178.072782841451));
#19553=CARTESIAN_POINT('Ctrl Pts',(-33.9157941348307,35.7193826009939,178.085866381542));
#19554=CARTESIAN_POINT('Ctrl Pts',(-33.9022674318341,35.7434803909662,178.100186584167));
#19555=CARTESIAN_POINT('Ctrl Pts',(-33.8973136760764,35.7523054953435,178.105430935745));
#19556=CARTESIAN_POINT('Ctrl Pts',(-33.892423522062,35.7610458255236,178.110840715817));
#19557=CARTESIAN_POINT('Ctrl Pts',(-33.8876020576637,35.769691455901,178.116409398955));
#19558=CARTESIAN_POINT('Ctrl Pts',(-33.8869772780581,35.7708117822357,178.117131005373));
#19559=CARTESIAN_POINT('Ctrl Pts',(-33.8863535630653,35.7719306524527,178.117855401103));
#19560=CARTESIAN_POINT('Ctrl Pts',(-33.8857309216736,35.7730480455806,178.118582564087));
#19561=CARTESIAN_POINT('Ctrl Pts',(-33.8698601234795,35.8015298026145,178.137117562145));
#19562=CARTESIAN_POINT('Ctrl Pts',(-33.8545548409672,35.829289317426,178.157619748358));
#19563=CARTESIAN_POINT('Ctrl Pts',(-33.8399353901162,35.8560417099049,178.179865523891));
#19564=CARTESIAN_POINT('Ctrl Pts',(-33.8374692589998,35.8605545269871,178.183618127173));
#19565=CARTESIAN_POINT('Ctrl Pts',(-33.835022606309,35.8650387401053,178.187420245313));
#19566=CARTESIAN_POINT('Ctrl Pts',(-33.8325959619353,35.8694930537462,178.191270687453));
#19567=CARTESIAN_POINT('Ctrl Pts',(-33.8199869512839,35.8926379730227,178.211277848981));
#19568=CARTESIAN_POINT('Ctrl Pts',(-33.8079193627232,35.9149734889198,178.232590487925));
#19569=CARTESIAN_POINT('Ctrl Pts',(-33.7964576639897,35.9363350562286,178.255037515312));
#19570=CARTESIAN_POINT('Ctrl Pts',(-33.7900321528711,35.9483105051952,178.26762148104));
#19571=CARTESIAN_POINT('Ctrl Pts',(-33.7837965875609,35.9599807277839,178.280562417347));
#19572=CARTESIAN_POINT('Ctrl Pts',(-33.7777632759112,35.9713148162947,178.293822172451));
#19573=CARTESIAN_POINT('Ctrl Pts',(-33.7675348173914,35.9905298446117,178.31630184248));
#19574=CARTESIAN_POINT('Ctrl Pts',(-33.7578783351679,36.0087958173318,178.339710187513));
#19575=CARTESIAN_POINT('Ctrl Pts',(-33.7487823904955,36.0260993702412,178.364051408715));
#19576=CARTESIAN_POINT('Ctrl Pts',(-33.7398557276015,36.0430808921452,178.387939623072));
#19577=CARTESIAN_POINT('Ctrl Pts',(-33.7314687603436,36.0591360073105,178.412726903841));
#19578=CARTESIAN_POINT('Ctrl Pts',(-33.7236293478618,36.0742203564055,178.438450236595));
#19579=CARTESIAN_POINT('Ctrl Pts',(-33.7189541482838,36.0832162272936,178.453790890593));
#19580=CARTESIAN_POINT('Ctrl Pts',(-33.7144740589414,36.091866196189,178.469465048149));
#19581=CARTESIAN_POINT('Ctrl Pts',(-33.7101944105682,36.1001541204655,178.485485069079));
#19582=CARTESIAN_POINT('',(-33.3398524910169,36.8879333106141,179.985485069258));
#19583=CARTESIAN_POINT('Ctrl Pts',(-33.7101944105682,36.1001541204655,178.485485069079));
#19584=CARTESIAN_POINT('Ctrl Pts',(-33.5767107475439,36.3586572484842,178.985155124093));
#19585=CARTESIAN_POINT('Ctrl Pts',(-33.4532592756956,36.621368155505,179.485092205907));
#19586=CARTESIAN_POINT('Ctrl Pts',(-33.3398524911435,36.8879333109887,179.985485069079));
#19587=CARTESIAN_POINT('',(-32.4060870603391,41.431200111437,179.985485069079));
#19588=CARTESIAN_POINT('Origin',(-44.1060283439209,41.4682670878081,179.985485069079));
#19589=CARTESIAN_POINT('',(-32.4060870603391,41.431200111437,178.485485069079));
#19590=CARTESIAN_POINT('Origin',(-53.4413942236179,-112.716773792997,179.985485069079));
#19591=CARTESIAN_POINT('Ctrl Pts',(-33.3398524907636,36.8879333098646,179.985485069079));
#19592=CARTESIAN_POINT('Ctrl Pts',(-33.3574892950243,36.8464776027502,179.985485069079));
#19593=CARTESIAN_POINT('Ctrl Pts',(-33.3710414244414,36.8032694853988,179.985485069083));
#19594=CARTESIAN_POINT('Ctrl Pts',(-33.3899087453465,36.7118220614565,179.985485069083));
#19595=CARTESIAN_POINT('Ctrl Pts',(-33.3945539764798,36.6634335677105,179.985485069079));
#19596=CARTESIAN_POINT('Ctrl Pts',(-33.3922298082537,36.5460366143256,179.985485069079));
#19597=CARTESIAN_POINT('Ctrl Pts',(-33.3793951963956,36.4773565513148,179.985485069079));
#19598=CARTESIAN_POINT('Ctrl Pts',(-33.3300887502201,36.3532182089249,179.985485069079));
#19599=CARTESIAN_POINT('Ctrl Pts',(-33.2955167311449,36.2981567358835,179.985485069079));
#19600=CARTESIAN_POINT('Ctrl Pts',(-33.2141725090471,36.2148346472178,179.985485069079));
#19601=CARTESIAN_POINT('Ctrl Pts',(-33.1719475707044,36.184379905615,179.985485069079));
#19602=CARTESIAN_POINT('Ctrl Pts',(-33.0822769881238,36.1419052727305,179.985485069079));
#19603=CARTESIAN_POINT('Ctrl Pts',(-33.0367157125635,36.1289877482769,179.985485069079));
#19604=CARTESIAN_POINT('Ctrl Pts',(-32.9897426468184,36.123524749977,179.985485069079));
#19605=CARTESIAN_POINT('',(-29.2214842185525,55.7467898368407,179.985485069079));
#19606=CARTESIAN_POINT('',(-8.69585033055052,-107.076100989514,179.985485069079));
#19607=CARTESIAN_POINT('',(-30.7570310015667,59.9437472274033,179.985510844164));
#19608=CARTESIAN_POINT('Origin',(-39.1429618482127,54.4960773822167,179.985485069079));
#19609=CARTESIAN_POINT('Ctrl Pts',(-30.757020815632,59.9437588539596,179.985485069079));
#19610=CARTESIAN_POINT('Ctrl Pts',(-30.8085788556864,60.0230926458723,179.985485069079));
#19611=CARTESIAN_POINT('Ctrl Pts',(-30.8639970094185,60.1012773870114,179.98548506805));
#19612=CARTESIAN_POINT('Ctrl Pts',(-30.9777147231709,60.2527014471581,179.98548506805));
#19613=CARTESIAN_POINT('Ctrl Pts',(-31.0371822006902,60.3274835122335,179.985485069079));
#19614=CARTESIAN_POINT('Ctrl Pts',(-31.097570844777,60.4004632086527,179.985485069079));
#19615=CARTESIAN_POINT('',(-33.4443560589197,58.4349622311539,179.985485069079));
#19616=CARTESIAN_POINT('',(36.9742820842401,3.78287784314388,179.985485069079));
#19617=CARTESIAN_POINT('',(-34.3114325764233,57.3177432227255,179.985485069079));
#19618=CARTESIAN_POINT('',(-123.860032366778,-58.0646894049869,179.985485069079));
#19619=CARTESIAN_POINT('',(-33.1942135679949,56.4506667052219,179.985485069079));
#19620=CARTESIAN_POINT('',(36.1072055667355,2.66565883471801,179.985485069079));
#19621=CARTESIAN_POINT('',(-34.0612900854985,55.3334476967935,179.985485069079));
#19622=CARTESIAN_POINT('',(-122.742813358349,-58.9317659224909,179.985485069079));
#19623=CARTESIAN_POINT('',(-32.94407107707,54.4663711792899,179.985485069079));
#19624=CARTESIAN_POINT('',(35.240129049233,1.54843982628677,179.985485069079));
#19625=CARTESIAN_POINT('',(-33.8111475945737,53.3491521708615,179.985485069079));
#19626=CARTESIAN_POINT('',(-121.625594349921,-59.7988424399945,179.985485069079));
#19627=CARTESIAN_POINT('',(-32.6939285861452,52.4820756533578,179.985485069079));
#19628=CARTESIAN_POINT('',(34.3730525317294,0.43122081785836,179.985485069079));
#19629=CARTESIAN_POINT('',(-33.5610051036489,51.3648566449294,179.985485069079));
#19630=CARTESIAN_POINT('',(-120.508375341492,-60.6659189574982,179.985485069079));
#19631=CARTESIAN_POINT('',(-32.4437860952204,50.4977801274258,179.985485069079));
#19632=CARTESIAN_POINT('',(33.5059760142258,-0.685998190570039,179.985485069079));
#19633=CARTESIAN_POINT('',(-33.3108626127241,49.3805611189974,179.985485069079));
#19634=CARTESIAN_POINT('',(-119.391156333064,-61.5329954750018,179.985485069079));
#19635=CARTESIAN_POINT('',(-32.1936436042956,48.5134846014937,179.985485069079));
#19636=CARTESIAN_POINT('',(32.6388994967221,-1.80321719899848,179.985485069079));
#19637=CARTESIAN_POINT('',(-33.0607201217992,47.3962655930653,179.985485069079));
#19638=CARTESIAN_POINT('',(-118.273937324635,-62.4000719925054,179.985485069079));
#19639=CARTESIAN_POINT('',(-31.9435011133708,46.5291890755617,179.985485069079));
#19640=CARTESIAN_POINT('',(31.7718229792185,-2.92043620742687,179.985485069079));
#19641=CARTESIAN_POINT('',(-32.8105776308745,45.4119700671332,179.985485069079));
#19642=CARTESIAN_POINT('',(-117.156718316207,-63.267148510009,179.985485069079));
#19643=CARTESIAN_POINT('',(-31.693358622446,44.5448935496296,179.985485069079));
#19644=CARTESIAN_POINT('',(30.9047464617149,-4.03765521585528,179.985485069079));
#19645=CARTESIAN_POINT('',(-32.5604351399496,43.4276745412012,179.985485069079));
#19646=CARTESIAN_POINT('',(-116.039499307778,-64.1342250275126,179.985485069079));
#19647=CARTESIAN_POINT('',(-31.4432161315212,42.5605980236976,179.985485069079));
#19648=CARTESIAN_POINT('',(30.0376699442113,-5.15487422428371,179.985485069079));
#19649=CARTESIAN_POINT('',(-32.3102926490249,41.4433790152692,179.985485069079));
#19650=CARTESIAN_POINT('',(-114.92228029935,-65.0013015450162,179.985485069079));
#19651=CARTESIAN_POINT('',(-72.3928015643781,36.3474552058043,179.985485069079));
#19652=CARTESIAN_POINT('Origin',(-8.69585033055052,-107.076100989514,179.985485069079));
#19653=CARTESIAN_POINT('',(-28.5054632460221,55.8370522333852,178.735485069079));
#19654=CARTESIAN_POINT('',(-28.5054632460221,55.8370522333853,178.735485069079));
#19655=CARTESIAN_POINT('',(-29.2214842185525,55.7467898368407,179.985485069079));
#19656=CARTESIAN_POINT('Origin',(-8.69585033055052,-107.076100989514,171.985485069079));
#19657=CARTESIAN_POINT('',(-29.2214842185525,55.7467898368408,171.985485069079));
#19658=CARTESIAN_POINT('',(-28.5054632460221,55.8370522333853,173.235485069079));
#19659=CARTESIAN_POINT('',(-29.2214842185525,55.7467898368408,171.985485069079));
#19660=CARTESIAN_POINT('',(-7.97982935802012,-106.98583859297,173.235485069079));
#19661=CARTESIAN_POINT('',(-8.69585033055052,-107.076100989514,171.985485069079));
#19662=CARTESIAN_POINT('Origin',(-53.4413942236179,-112.716773792997,171.985485069079));
#19663=CARTESIAN_POINT('Ctrl Pts',(-32.9897426468162,36.1235247499768,171.985485069079));
#19664=CARTESIAN_POINT('Ctrl Pts',(-33.0365950120472,36.128973710728,171.985485069079));
#19665=CARTESIAN_POINT('Ctrl Pts',(-33.082044287583,36.1418391062218,171.985485069079));
#19666=CARTESIAN_POINT('Ctrl Pts',(-33.1715122949256,36.1841256819134,171.985485069079));
#19667=CARTESIAN_POINT('Ctrl Pts',(-33.2136614374764,36.2144401514148,171.98548506908));
#19668=CARTESIAN_POINT('Ctrl Pts',(-33.2950202919873,36.2974900115958,171.98548506908));
#19669=CARTESIAN_POINT('Ctrl Pts',(-33.3296649319802,36.3524534103143,171.985485069079));
#19670=CARTESIAN_POINT('Ctrl Pts',(-33.3791527024948,36.4764276694108,171.985485069079));
#19671=CARTESIAN_POINT('Ctrl Pts',(-33.3920941031955,36.54504181561,171.985485069079));
#19672=CARTESIAN_POINT('Ctrl Pts',(-33.3946169229336,36.6625737676883,171.985485069079));
#19673=CARTESIAN_POINT('Ctrl Pts',(-33.3900102035898,36.7111525376301,171.985485069076));
#19674=CARTESIAN_POINT('Ctrl Pts',(-33.3711403825,36.8029537917995,171.985485069076));
#19675=CARTESIAN_POINT('Ctrl Pts',(-33.3575537145651,36.8463261831631,171.985485069079));
#19676=CARTESIAN_POINT('Ctrl Pts',(-33.3398524907635,36.8879333098647,171.985485069079));
#19677=CARTESIAN_POINT('',(-32.3102926490249,41.4433790152692,171.985485069079));
#19678=CARTESIAN_POINT('',(-72.3928015643781,36.3474552058043,171.985485069079));
#19679=CARTESIAN_POINT('',(-31.4432161315212,42.5605980236976,171.985485069079));
#19680=CARTESIAN_POINT('',(-114.92228029935,-65.0013015450162,171.985485069079));
#19681=CARTESIAN_POINT('',(-32.5604351399496,43.4276745412012,171.985485069079));
#19682=CARTESIAN_POINT('',(30.0376699442113,-5.15487422428371,171.985485069079));
#19683=CARTESIAN_POINT('',(-31.693358622446,44.5448935496296,171.985485069079));
#19684=CARTESIAN_POINT('',(-116.039499307778,-64.1342250275126,171.985485069079));
#19685=CARTESIAN_POINT('',(-32.8105776308745,45.4119700671332,171.985485069079));
#19686=CARTESIAN_POINT('',(30.9047464617149,-4.03765521585528,171.985485069079));
#19687=CARTESIAN_POINT('',(-31.9435011133708,46.5291890755617,171.985485069079));
#19688=CARTESIAN_POINT('',(-117.156718316207,-63.267148510009,171.985485069079));
#19689=CARTESIAN_POINT('',(-33.0607201217992,47.3962655930653,171.985485069079));
#19690=CARTESIAN_POINT('',(31.7718229792185,-2.92043620742687,171.985485069079));
#19691=CARTESIAN_POINT('',(-32.1936436042956,48.5134846014937,171.985485069079));
#19692=CARTESIAN_POINT('',(-118.273937324635,-62.4000719925054,171.985485069079));
#19693=CARTESIAN_POINT('',(-33.3108626127241,49.3805611189974,171.985485069079));
#19694=CARTESIAN_POINT('',(32.6388994967221,-1.80321719899848,171.985485069079));
#19695=CARTESIAN_POINT('',(-32.4437860952204,50.4977801274258,171.985485069079));
#19696=CARTESIAN_POINT('',(-119.391156333064,-61.5329954750018,171.985485069079));
#19697=CARTESIAN_POINT('',(-33.5610051036489,51.3648566449294,171.985485069079));
#19698=CARTESIAN_POINT('',(33.5059760142258,-0.685998190570039,171.985485069079));
#19699=CARTESIAN_POINT('',(-32.6939285861452,52.4820756533578,171.985485069079));
#19700=CARTESIAN_POINT('',(-120.508375341492,-60.6659189574982,171.985485069079));
#19701=CARTESIAN_POINT('',(-33.8111475945737,53.3491521708615,171.985485069079));
#19702=CARTESIAN_POINT('',(34.3730525317294,0.43122081785836,171.985485069079));
#19703=CARTESIAN_POINT('',(-32.94407107707,54.4663711792899,171.985485069079));
#19704=CARTESIAN_POINT('',(-121.625594349921,-59.7988424399945,171.985485069079));
#19705=CARTESIAN_POINT('',(-34.0612900854985,55.3334476967935,171.985485069079));
#19706=CARTESIAN_POINT('',(35.240129049233,1.54843982628677,171.985485069079));
#19707=CARTESIAN_POINT('',(-33.1942135679949,56.4506667052219,171.985485069079));
#19708=CARTESIAN_POINT('',(-122.742813358349,-58.9317659224909,171.985485069079));
#19709=CARTESIAN_POINT('',(-34.3114325764233,57.3177432227255,171.985485069079));
#19710=CARTESIAN_POINT('',(36.1072055667355,2.66565883471801,171.985485069079));
#19711=CARTESIAN_POINT('',(-33.4443560589197,58.4349622311539,171.985485069079));
#19712=CARTESIAN_POINT('',(-123.860032366778,-58.0646894049869,171.985485069079));
#19713=CARTESIAN_POINT('',(36.9742820842401,3.78287784314388,171.985485069079));
#19714=CARTESIAN_POINT('',(-30.7570310015667,59.9437472274033,171.985459293995));
#19715=CARTESIAN_POINT('Ctrl Pts',(-31.0975708447772,60.4004632086527,171.985485069079));
#19716=CARTESIAN_POINT('Ctrl Pts',(-31.0371822006902,60.3274835122321,171.985485069079));
#19717=CARTESIAN_POINT('Ctrl Pts',(-30.9777147231722,60.2527014471572,171.985485070109));
#19718=CARTESIAN_POINT('Ctrl Pts',(-30.8639970094202,60.1012773870101,171.985485070109));
#19719=CARTESIAN_POINT('Ctrl Pts',(-30.8085788556878,60.0230926458712,171.985485069079));
#19720=CARTESIAN_POINT('Ctrl Pts',(-30.757020815632,59.9437588539596,171.985485069079));
#19721=CARTESIAN_POINT('Origin',(-39.1429618482127,54.4960773822167,171.985485069079));
#19722=CARTESIAN_POINT('Origin',(-39.1429618482127,54.4960773822167,171.985485069079));
#19723=CARTESIAN_POINT('',(-28.9015818590613,57.6692029676422,173.235485069079));
#19724=CARTESIAN_POINT('Ctrl Pts',(-30.7570310015667,59.9437472274033,171.985459293995));
#19725=CARTESIAN_POINT('Ctrl Pts',(-30.4721900266403,59.6217336312295,172.09525140435));
#19726=CARTESIAN_POINT('Ctrl Pts',(-30.2017002008111,59.3043637535052,172.235659045439));
#19727=CARTESIAN_POINT('Ctrl Pts',(-29.9430583375974,58.990922442063,172.399845773266));
#19728=CARTESIAN_POINT('Ctrl Pts',(-29.6729880538802,58.6636313266262,172.571287301006));
#19729=CARTESIAN_POINT('Ctrl Pts',(-29.4156601420299,58.3403948799334,172.768784715011));
#19730=CARTESIAN_POINT('Ctrl Pts',(-29.1687750801219,58.0200685378704,172.987248162164));
#19731=CARTESIAN_POINT('Ctrl Pts',(-29.0783477005634,57.9027415862418,173.067265466178));
#19732=CARTESIAN_POINT('Ctrl Pts',(-28.9893211789838,57.7858051107646,173.150095083597));
#19733=CARTESIAN_POINT('Ctrl Pts',(-28.9015818590613,57.6692029676421,173.235485069079));
#19734=CARTESIAN_POINT('Origin',(-39.1429618482127,54.4960773822167,173.235485069079));
#19735=CARTESIAN_POINT('Origin',(-39.1429618482127,54.4960773822167,179.985485069079));
#19736=CARTESIAN_POINT('',(-28.9015818590613,57.6692029676422,178.735485069079));
#19737=CARTESIAN_POINT('Origin',(-39.1429618482127,54.4960773822167,178.735485069079));
#19738=CARTESIAN_POINT('Ctrl Pts',(-28.9015818590613,57.6692029676422,178.735485069079));
#19739=CARTESIAN_POINT('Ctrl Pts',(-29.1411279737203,57.9875504356935,178.968617024867));
#19740=CARTESIAN_POINT('Ctrl Pts',(-29.390270556352,58.3083899273538,179.182659656602));
#19741=CARTESIAN_POINT('Ctrl Pts',(-29.6513150897315,58.632864293538,179.372505039673));
#19742=CARTESIAN_POINT('Ctrl Pts',(-29.7469287040763,58.7517105551756,179.442040314007));
#19743=CARTESIAN_POINT('Ctrl Pts',(-29.8441388328647,58.8710444806848,179.508329929376));
#19744=CARTESIAN_POINT('Ctrl Pts',(-29.9430583375964,58.9909224420661,179.571124364888));
#19745=CARTESIAN_POINT('Ctrl Pts',(-30.2017002008109,59.3043637535053,179.735311092719));
#19746=CARTESIAN_POINT('Ctrl Pts',(-30.4721900266405,59.6217336312296,179.875718733809));
#19747=CARTESIAN_POINT('Ctrl Pts',(-30.7570310015667,59.9437472274033,179.985510844164));
#19748=CARTESIAN_POINT('Origin',(-34.5615750673481,59.3020387486575,165.645237852233));
#19749=CARTESIAN_POINT('',(-33.4443560589197,58.4349622311539,165.645237852233));
#19750=CARTESIAN_POINT('Origin',(-33.4443560589197,58.4349622311539,165.645237852233));
#19751=CARTESIAN_POINT('',(-34.3114325764233,57.3177432227255,165.645237852233));
#19752=CARTESIAN_POINT('Origin',(-34.3114325764233,57.3177432227255,165.645237852233));
#19753=CARTESIAN_POINT('',(-33.1942135679949,56.4506667052219,165.645237852233));
#19754=CARTESIAN_POINT('Origin',(-33.1942135679949,56.4506667052219,165.645237852233));
#19755=CARTESIAN_POINT('',(-34.0612900854985,55.3334476967935,165.645237852233));
#19756=CARTESIAN_POINT('Origin',(-34.0612900854985,55.3334476967935,165.645237852233));
#19757=CARTESIAN_POINT('',(-32.94407107707,54.4663711792899,165.645237852233));
#19758=CARTESIAN_POINT('Origin',(-32.94407107707,54.4663711792899,165.645237852233));
#19759=CARTESIAN_POINT('',(-33.8111475945737,53.3491521708615,165.645237852233));
#19760=CARTESIAN_POINT('Origin',(-33.8111475945737,53.3491521708615,165.645237852233));
#19761=CARTESIAN_POINT('',(-32.6939285861452,52.4820756533578,165.645237852233));
#19762=CARTESIAN_POINT('Origin',(-32.6939285861452,52.4820756533578,165.645237852233));
#19763=CARTESIAN_POINT('',(-33.5610051036489,51.3648566449294,165.645237852233));
#19764=CARTESIAN_POINT('Origin',(-33.5610051036489,51.3648566449294,165.645237852233));
#19765=CARTESIAN_POINT('',(-32.4437860952204,50.4977801274258,165.645237852233));
#19766=CARTESIAN_POINT('Origin',(-32.4437860952204,50.4977801274258,165.645237852233));
#19767=CARTESIAN_POINT('',(-33.3108626127241,49.3805611189974,165.645237852233));
#19768=CARTESIAN_POINT('Origin',(-33.3108626127241,49.3805611189974,165.645237852233));
#19769=CARTESIAN_POINT('',(-32.1936436042956,48.5134846014937,165.645237852233));
#19770=CARTESIAN_POINT('Origin',(-32.1936436042956,48.5134846014937,165.645237852233));
#19771=CARTESIAN_POINT('',(-33.0607201217992,47.3962655930653,165.645237852233));
#19772=CARTESIAN_POINT('Origin',(-33.0607201217992,47.3962655930653,165.645237852233));
#19773=CARTESIAN_POINT('',(-31.9435011133708,46.5291890755617,165.645237852233));
#19774=CARTESIAN_POINT('Origin',(-31.9435011133708,46.5291890755617,165.645237852233));
#19775=CARTESIAN_POINT('',(-32.8105776308745,45.4119700671332,165.645237852233));
#19776=CARTESIAN_POINT('Origin',(-32.8105776308745,45.4119700671332,165.645237852233));
#19777=CARTESIAN_POINT('',(-31.693358622446,44.5448935496296,165.645237852233));
#19778=CARTESIAN_POINT('Origin',(-31.693358622446,44.5448935496296,165.645237852233));
#19779=CARTESIAN_POINT('',(-32.5604351399496,43.4276745412012,165.645237852233));
#19780=CARTESIAN_POINT('Origin',(-32.5604351399496,43.4276745412012,165.645237852233));
#19781=CARTESIAN_POINT('',(-31.4432161315212,42.5605980236976,165.645237852233));
#19782=CARTESIAN_POINT('Origin',(-31.4432161315212,42.5605980236976,165.645237852233));
#19783=CARTESIAN_POINT('',(-32.3102926490249,41.4433790152692,165.645237852233));
#19784=CARTESIAN_POINT('Origin',(-37.2830935213589,40.8111577534073,165.645237852233));
#19785=CARTESIAN_POINT('Origin',(-7.55021677450188,-106.931681155043,172.985485069079));
#19786=CARTESIAN_POINT('',(-28.0900682566218,55.8894173856563,173.485279674622));
#19787=CARTESIAN_POINT('Origin',(-28.0758506625039,55.8912096713119,172.985485069079));
#19788=CARTESIAN_POINT('Origin',(-26.8530188945057,47.5592063900784,158.714565891));
#19789=CARTESIAN_POINT('Origin',(-39.1429618482127,54.4960773822167,172.985485069079));
#19790=CARTESIAN_POINT('Ctrl Pts',(-28.9015818590613,57.6692029676421,173.235485069079));
#19791=CARTESIAN_POINT('Ctrl Pts',(-28.8783957075631,57.6244523537673,173.250906112447));
#19792=CARTESIAN_POINT('Ctrl Pts',(-28.8552578884252,57.5793410334276,173.264929290539));
#19793=CARTESIAN_POINT('Ctrl Pts',(-28.832206350973,57.5339462931836,173.277868929688));
#19794=CARTESIAN_POINT('Ctrl Pts',(-28.8065664597265,57.4834543810741,173.292261502906));
#19795=CARTESIAN_POINT('Ctrl Pts',(-28.7810331273392,57.4326117098059,173.305313364622));
#19796=CARTESIAN_POINT('Ctrl Pts',(-28.7556446263524,57.3814869308062,173.317399481028));
#19797=CARTESIAN_POINT('Ctrl Pts',(-28.7329260654482,57.3357386053725,173.328214580818));
#19798=CARTESIAN_POINT('Ctrl Pts',(-28.7103230594705,57.2897634704848,173.33825497767));
#19799=CARTESIAN_POINT('Ctrl Pts',(-28.6878575715527,57.2435917682567,173.347760399718));
#19800=CARTESIAN_POINT('Ctrl Pts',(-28.6871251437978,57.2420864621477,173.348070298838));
#19801=CARTESIAN_POINT('Ctrl Pts',(-28.6863928067171,57.2405808318857,173.34837957377));
#19802=CARTESIAN_POINT('Ctrl Pts',(-28.6856605607426,57.2390748787108,173.348688226559));
#19803=CARTESIAN_POINT('Ctrl Pts',(-28.6546983128659,57.1753972387935,173.361739283828));
#19804=CARTESIAN_POINT('Ctrl Pts',(-28.6239686550817,57.111288866525,173.373652144523));
#19805=CARTESIAN_POINT('Ctrl Pts',(-28.5935146468786,57.0468622475461,173.384569672603));
#19806=CARTESIAN_POINT('Ctrl Pts',(-28.5594104597168,56.9747135353897,173.396795761809));
#19807=CARTESIAN_POINT('Ctrl Pts',(-28.5256504453393,56.9021633205751,173.407773929404));
#19808=CARTESIAN_POINT('Ctrl Pts',(-28.4923003004926,56.8293357844001,173.417654178831));
#19809=CARTESIAN_POINT('Ctrl Pts',(-28.4872778889987,56.818368220198,173.419142108749));
#19810=CARTESIAN_POINT('Ctrl Pts',(-28.4822648091068,56.8073943548846,173.420605050385));
#19811=CARTESIAN_POINT('Ctrl Pts',(-28.4772613313079,56.7964146162697,173.422043425076));
#19812=CARTESIAN_POINT('Ctrl Pts',(-28.4770521713326,56.7959556311497,173.422103553336));
#19813=CARTESIAN_POINT('Ctrl Pts',(-28.4768430287364,56.7954966370769,173.422163638491));
#19814=CARTESIAN_POINT('Ctrl Pts',(-28.4766339035806,56.7950376341736,173.422223680559));
#19815=CARTESIAN_POINT('Ctrl Pts',(-28.4066282600523,56.641384222626,173.442323049322));
#19816=CARTESIAN_POINT('Ctrl Pts',(-28.3384533787665,56.4865756844121,173.457833018597));
#19817=CARTESIAN_POINT('Ctrl Pts',(-28.2720423773652,56.3306091186088,173.468472689585));
#19818=CARTESIAN_POINT('Ctrl Pts',(-28.2098532731482,56.184557699259,173.478435972685));
#19819=CARTESIAN_POINT('Ctrl Pts',(-28.1492110828377,56.0374907574936,173.484128243792));
#19820=CARTESIAN_POINT('Ctrl Pts',(-28.0900682566218,55.8894173856563,173.485279674622));
#19821=CARTESIAN_POINT('Origin',(-7.55021677450188,-106.931681155043,178.985485069079));
#19822=CARTESIAN_POINT('',(-28.0900682566218,55.8894173856563,178.485690463537));
#19823=CARTESIAN_POINT('Origin',(-26.8543432602028,47.5681742429628,193.240450635157));
#19824=CARTESIAN_POINT('Origin',(-28.0758506625039,55.8912096713119,178.985485069079));
#19825=CARTESIAN_POINT('Origin',(-39.1429618482127,54.4960773822167,178.985485069079));
#19826=CARTESIAN_POINT('Ctrl Pts',(-28.0900682566218,55.8894173856563,178.485690463537));
#19827=CARTESIAN_POINT('Ctrl Pts',(-28.1532261741964,56.0475431705021,178.486920062765));
#19828=CARTESIAN_POINT('Ctrl Pts',(-28.2180938553462,56.2045210764306,178.493327449093));
#19829=CARTESIAN_POINT('Ctrl Pts',(-28.2847294808783,56.3603405304585,178.504585631502));
#19830=CARTESIAN_POINT('Ctrl Pts',(-28.34712892925,56.5062541899956,178.515128105837));
#19831=CARTESIAN_POINT('Ctrl Pts',(-28.4110786768076,56.6511523167797,178.529924851071));
#19832=CARTESIAN_POINT('Ctrl Pts',(-28.4766339035804,56.7950376341737,178.5487464576));
#19833=CARTESIAN_POINT('Ctrl Pts',(-28.4768430287362,56.7954966370769,178.548806499668));
#19834=CARTESIAN_POINT('Ctrl Pts',(-28.4770521713324,56.7959556311498,178.548866584823));
#19835=CARTESIAN_POINT('Ctrl Pts',(-28.4772613313078,56.7964146162698,178.548926713083));
#19836=CARTESIAN_POINT('Ctrl Pts',(-28.5112094816522,56.8709111629163,178.558685956994));
#19837=CARTESIAN_POINT('Ctrl Pts',(-28.54559760442,56.9451372173971,178.569572016831));
#19838=CARTESIAN_POINT('Ctrl Pts',(-28.5803527484962,57.0189613364396,178.581737771227));
#19839=CARTESIAN_POINT('Ctrl Pts',(-28.610726409608,57.0834786570626,178.592369823289));
#19840=CARTESIAN_POINT('Ctrl Pts',(-28.6413817046753,57.1476909918109,178.603979625781));
#19841=CARTESIAN_POINT('Ctrl Pts',(-28.6722760253921,57.2114911539207,178.616704729058));
#19842=CARTESIAN_POINT('Ctrl Pts',(-28.6767326149162,57.2206945002802,178.618540359706));
#19843=CARTESIAN_POINT('Ctrl Pts',(-28.6811941725409,57.2298892065096,178.620399261204));
#19844=CARTESIAN_POINT('Ctrl Pts',(-28.6856605607423,57.2390748787112,178.6222819116));
#19845=CARTESIAN_POINT('Ctrl Pts',(-28.6863928067167,57.2405808318861,178.622590564388));
#19846=CARTESIAN_POINT('Ctrl Pts',(-28.6871251437975,57.2420864621481,178.62289983932));
#19847=CARTESIAN_POINT('Ctrl Pts',(-28.6878575715524,57.2435917682571,178.62320973844));
#19848=CARTESIAN_POINT('Ctrl Pts',(-28.7136979020017,57.2966995417155,178.634143097541));
#19849=CARTESIAN_POINT('Ctrl Pts',(-28.7397203004661,57.3495477961519,178.645783407186));
#19850=CARTESIAN_POINT('Ctrl Pts',(-28.7658909284461,57.4020887705021,178.658498134593));
#19851=CARTESIAN_POINT('Ctrl Pts',(-28.7890925824529,57.4486691394938,178.669770416874));
#19852=CARTESIAN_POINT('Ctrl Pts',(-28.8124109552486,57.495008155114,178.681886920562));
#19853=CARTESIAN_POINT('Ctrl Pts',(-28.8358161917034,57.5410513416207,178.695136076362));
#19854=CARTESIAN_POINT('Ctrl Pts',(-28.8576730368229,57.584048505876,178.707508724118));
#19855=CARTESIAN_POINT('Ctrl Pts',(-28.8796057823956,57.6267878682054,178.720868843039));
#19856=CARTESIAN_POINT('Ctrl Pts',(-28.9015818590613,57.6692029676421,178.735485069079));
#19857=CARTESIAN_POINT('Ctrl Pts',(-27.6574947146374,56.1206152968612,177.985485069079));
#19858=CARTESIAN_POINT('Ctrl Pts',(-27.6574947146374,56.1206152968612,178.485485069079));
#19859=CARTESIAN_POINT('Ctrl Pts',(-28.0689593736356,55.8365434144167,178.485485069079));
#19860=CARTESIAN_POINT('Ctrl Pts',(-27.6694079641717,56.1378710742194,177.985485068867));
#19861=CARTESIAN_POINT('Ctrl Pts',(-27.6681144406602,56.1359974667813,178.481269766953));
#19862=CARTESIAN_POINT('Ctrl Pts',(-28.0759896722413,55.8541773044658,178.485485069079));
#19863=CARTESIAN_POINT('Ctrl Pts',(-27.6813344276784,56.1551166027306,177.985621535458));
#19864=CARTESIAN_POINT('Ctrl Pts',(-27.6788158552697,56.1514749213828,178.477207837903));
#19865=CARTESIAN_POINT('Ctrl Pts',(-28.083025968225,55.871801963558,178.485553302133));
#19866=CARTESIAN_POINT('Ctrl Pts',(-27.6932740952942,56.17235187585,177.985895857994));
#19867=CARTESIAN_POINT('Ctrl Pts',(-27.6895961064823,56.1670425872045,178.473302706478));
#19868=CARTESIAN_POINT('Ctrl Pts',(-28.0900682566218,55.8894173856562,178.485690463537));
#19869=CARTESIAN_POINT('Origin',(-28.1042858507397,55.8876251000007,177.985895857994));
#19870=CARTESIAN_POINT('Ctrl Pts',(-28.9015818590613,57.6692029676421,178.735485069079));
#19871=CARTESIAN_POINT('Ctrl Pts',(-28.8684594052104,57.7807218601806,178.623519943881));
#19872=CARTESIAN_POINT('Ctrl Pts',(-28.9197092925293,57.8469757052856,178.485485069079));
#19873=CARTESIAN_POINT('Ctrl Pts',(-28.8312423460306,57.5334435982818,178.688702479453));
#19874=CARTESIAN_POINT('Ctrl Pts',(-28.7721100878092,57.6556162573135,178.558964673111));
#19875=CARTESIAN_POINT('Ctrl Pts',(-28.8243214284443,57.72366201422,178.392078873294));
#19876=CARTESIAN_POINT('Ctrl Pts',(-28.7591862218731,57.3901866577354,178.653390254656));
#19877=CARTESIAN_POINT('Ctrl Pts',(-28.672354550029,57.5244839151744,178.515152190406));
#19878=CARTESIAN_POINT('Ctrl Pts',(-28.7239047060481,57.5923063305154,178.321295444065));
#19879=CARTESIAN_POINT('Ctrl Pts',(-28.6165295181076,57.0969960951184,178.593029960819));
#19880=CARTESIAN_POINT('Ctrl Pts',(-28.471590439667,57.2570348653644,178.447866227612));
#19881=CARTESIAN_POINT('Ctrl Pts',(-28.5198863309438,57.3216783903814,178.200574848726));
#19882=CARTESIAN_POINT('Ctrl Pts',(-28.5454048906478,56.9459811395567,178.568491345164));
#19883=CARTESIAN_POINT('Ctrl Pts',(-28.3690672047113,57.1185646996549,178.425946256232));
#19884=CARTESIAN_POINT('Ctrl Pts',(-28.4153684876184,57.1811899787714,178.151497622782));
#19885=CARTESIAN_POINT('Ctrl Pts',(-28.3390919900902,56.4931505677619,178.509256722049));
#19886=CARTESIAN_POINT('Ctrl Pts',(-28.0597531656501,56.6952271283425,178.389517436387));
#19887=CARTESIAN_POINT('Ctrl Pts',(-28.1035068265426,56.7559702344856,178.033028371953));
#19888=CARTESIAN_POINT('Ctrl Pts',(-28.2104907674039,56.1909140904525,178.48803492694));
#19889=CARTESIAN_POINT('Ctrl Pts',(-27.8614033472109,56.415147805598,178.410967591661));
#19890=CARTESIAN_POINT('Ctrl Pts',(-27.897368693661,56.4669686322174,177.990585092576));
#19891=CARTESIAN_POINT('Ctrl Pts',(-28.0900682566218,55.8894173856563,178.485690463537));
#19892=CARTESIAN_POINT('Ctrl Pts',(-27.6895961064823,56.1670425872046,178.473302706478));
#19893=CARTESIAN_POINT('Ctrl Pts',(-27.6932740952942,56.1723518758501,177.985895857994));
#19894=CARTESIAN_POINT('Origin',(-29.3151965518073,57.5410511594434,178.485485069079));
#19895=CARTESIAN_POINT('Ctrl Pts',(-28.9197092925293,57.8469757052856,178.485485069079));
#19896=CARTESIAN_POINT('Ctrl Pts',(-28.8684594052104,57.7807218601806,178.623519943881));
#19897=CARTESIAN_POINT('Ctrl Pts',(-28.9015818590613,57.6692029676421,178.735485069079));
#19898=CARTESIAN_POINT('Ctrl Pts',(-29.2441517252768,58.2664021627722,178.803187555911));
#19899=CARTESIAN_POINT('Ctrl Pts',(-29.1960592199985,58.2060626206576,178.939525960898));
#19900=CARTESIAN_POINT('Ctrl Pts',(-29.2280229684941,58.1030305019131,179.053185293937));
#19901=CARTESIAN_POINT('Ctrl Pts',(-29.5857084336898,58.6906563012156,179.086383412666));
#19902=CARTESIAN_POINT('Ctrl Pts',(-29.5424509131589,58.6380170915417,179.222334391769));
#19903=CARTESIAN_POINT('Ctrl Pts',(-29.5732144254148,58.5426646457117,179.336383412017));
#19904=CARTESIAN_POINT('Ctrl Pts',(-30.3136646322233,59.5550714589887,179.555994501918));
#19905=CARTESIAN_POINT('Ctrl Pts',(-30.2815269581094,59.5181763377526,179.690677583542));
#19906=CARTESIAN_POINT('Ctrl Pts',(-30.3129364447101,59.439080359551,179.805994502568));
#19907=CARTESIAN_POINT('Ctrl Pts',(-30.7003778315039,59.9956453799363,179.742653148955));
#19908=CARTESIAN_POINT('Ctrl Pts',(-30.6749317799783,59.967435021151,179.877207841684));
#19909=CARTESIAN_POINT('Ctrl Pts',(-30.707799046115,59.8962927399543,179.992649949041));
#19910=CARTESIAN_POINT('Ctrl Pts',(-31.1165943278663,60.4472861348584,179.860245913625));
#19911=CARTESIAN_POINT('Ctrl Pts',(-31.0989366204049,60.4281255768369,179.994612574165));
#19912=CARTESIAN_POINT('Ctrl Pts',(-31.1350022734637,60.3643955167689,180.110245913625));
#19913=CARTESIAN_POINT('Ctrl Pts',(-28.0689593736356,55.8365434144167,173.485485069079));
#19914=CARTESIAN_POINT('Ctrl Pts',(-27.6574947146374,56.1206152968612,173.485485069079));
#19915=CARTESIAN_POINT('Ctrl Pts',(-27.6574947146374,56.1206152968612,173.985485069079));
#19916=CARTESIAN_POINT('Ctrl Pts',(-28.0759896722412,55.8541773044657,173.485485069079));
#19917=CARTESIAN_POINT('Ctrl Pts',(-27.6681144406602,56.1359974667812,173.489700371206));
#19918=CARTESIAN_POINT('Ctrl Pts',(-27.6694079641718,56.1378710742195,173.985485069291));
#19919=CARTESIAN_POINT('Ctrl Pts',(-28.0830259682254,55.8718019635579,173.485416836026));
#19920=CARTESIAN_POINT('Ctrl Pts',(-27.6788158552703,56.1514749213822,173.493762300257));
#19921=CARTESIAN_POINT('Ctrl Pts',(-27.6813344276784,56.1551166027305,173.9853486027));
#19922=CARTESIAN_POINT('Ctrl Pts',(-28.0900682566218,55.8894173856563,173.485279674622));
#19923=CARTESIAN_POINT('Ctrl Pts',(-27.6895961064823,56.1670425872046,173.497667431681));
#19924=CARTESIAN_POINT('Ctrl Pts',(-27.6932740952942,56.1723518758501,173.985074280165));
#19925=CARTESIAN_POINT('Origin',(-28.1042858507397,55.8876251000007,173.985074280165));
#19926=CARTESIAN_POINT('Ctrl Pts',(-28.9197092925293,57.8469757052856,173.485485069079));
#19927=CARTESIAN_POINT('Ctrl Pts',(-28.8684594052104,57.7807218601806,173.347450194278));
#19928=CARTESIAN_POINT('Ctrl Pts',(-28.9015818590613,57.6692029676421,173.235485069079));
#19929=CARTESIAN_POINT('Ctrl Pts',(-28.8243214284456,57.7236620142217,173.578891264868));
#19930=CARTESIAN_POINT('Ctrl Pts',(-28.7721100878089,57.6556162573148,173.412005465051));
#19931=CARTESIAN_POINT('Ctrl Pts',(-28.8312423460299,57.5334435982831,173.282267658708));
#19932=CARTESIAN_POINT('Ctrl Pts',(-28.7239047060486,57.592306330516,173.649674694096));
#19933=CARTESIAN_POINT('Ctrl Pts',(-28.6723545500293,57.5244839151751,173.455817947753));
#19934=CARTESIAN_POINT('Ctrl Pts',(-28.7591862218723,57.3901866577358,173.317579883503));
#19935=CARTESIAN_POINT('Ctrl Pts',(-28.5198863309434,57.3216783903809,173.77039528943));
#19936=CARTESIAN_POINT('Ctrl Pts',(-28.4715904396667,57.2570348653639,173.523103910547));
#19937=CARTESIAN_POINT('Ctrl Pts',(-28.6165295181085,57.096996095118,173.377940177339));
#19938=CARTESIAN_POINT('Ctrl Pts',(-28.4153684876182,57.1811899787712,173.819472515376));
#19939=CARTESIAN_POINT('Ctrl Pts',(-28.3690672047116,57.1185646996537,173.545023881929));
#19940=CARTESIAN_POINT('Ctrl Pts',(-28.5454048906478,56.9459811395561,173.402478792994));
#19941=CARTESIAN_POINT('Ctrl Pts',(-28.103506826543,56.7559702344862,173.937941766205));
#19942=CARTESIAN_POINT('Ctrl Pts',(-28.0597531656494,56.695227128345,173.581452701767));
#19943=CARTESIAN_POINT('Ctrl Pts',(-28.3390919900903,56.4931505677632,173.46171341611));
#19944=CARTESIAN_POINT('Ctrl Pts',(-27.8973686936607,56.4669686322171,173.980385045582));
#19945=CARTESIAN_POINT('Ctrl Pts',(-27.8614033472118,56.4151478055982,173.560002546493));
#19946=CARTESIAN_POINT('Ctrl Pts',(-28.2104907674024,56.1909140904522,173.482935211219));
#19947=CARTESIAN_POINT('Ctrl Pts',(-27.6932740952942,56.1723518758501,173.985074280165));
#19948=CARTESIAN_POINT('Ctrl Pts',(-27.6895961064823,56.1670425872046,173.497667431681));
#19949=CARTESIAN_POINT('Ctrl Pts',(-28.0900682566218,55.8894173856563,173.485279674622));
#19950=CARTESIAN_POINT('Origin',(-29.3151965518073,57.5410511594434,173.485485069079));
#19951=CARTESIAN_POINT('Ctrl Pts',(-28.9015818590613,57.6692029676421,173.235485069079));
#19952=CARTESIAN_POINT('Ctrl Pts',(-28.8684594052104,57.7807218601806,173.347450194278));
#19953=CARTESIAN_POINT('Ctrl Pts',(-28.9197092925293,57.8469757052856,173.485485069079));
#19954=CARTESIAN_POINT('Ctrl Pts',(-29.2280229684935,58.1030305019142,172.917784844223));
#19955=CARTESIAN_POINT('Ctrl Pts',(-29.1960592200032,58.2060626206536,173.03144417726));
#19956=CARTESIAN_POINT('Ctrl Pts',(-29.244151725278,58.2664021627738,173.167782582254));
#19957=CARTESIAN_POINT('Ctrl Pts',(-29.5732144254162,58.5426646457073,172.634586726136));
#19958=CARTESIAN_POINT('Ctrl Pts',(-29.5424509131556,58.6380170915374,172.748635746381));
#19959=CARTESIAN_POINT('Ctrl Pts',(-29.5857084336879,58.6906563012133,172.884586725484));
#19960=CARTESIAN_POINT('Ctrl Pts',(-30.3129364447087,59.4390803595552,172.164975635597));
#19961=CARTESIAN_POINT('Ctrl Pts',(-30.2815269581124,59.5181763377567,172.280292554625));
#19962=CARTESIAN_POINT('Ctrl Pts',(-30.3136646322252,59.555071458991,172.414975636249));
#19963=CARTESIAN_POINT('Ctrl Pts',(-30.7077990461131,59.8962927399557,171.978320189122));
#19964=CARTESIAN_POINT('Ctrl Pts',(-30.6749317799805,59.9674350211545,172.093762296512));
#19965=CARTESIAN_POINT('Ctrl Pts',(-30.7003778315034,59.9956453799358,172.228316989206));
#19966=CARTESIAN_POINT('Ctrl Pts',(-31.1350022734636,60.3643955167688,171.860724224534));
#19967=CARTESIAN_POINT('Ctrl Pts',(-31.0989366204048,60.4281255768368,171.976357563994));
#19968=CARTESIAN_POINT('Ctrl Pts',(-31.1165943278662,60.4472861348583,172.110724224534));
#19969=CARTESIAN_POINT('Origin',(-51.4899841053611,-42.5281564925371,175.985485069079));
#19970=CARTESIAN_POINT('Origin',(-51.4899841053611,-42.5281564925371,175.985485069079));
#19971=CARTESIAN_POINT('',(-59.8287670060529,-101.979172801565,172.515418850865));
#19972=CARTESIAN_POINT('Origin',(-57.8503443722502,-102.190085871961,175.985485069079));
#19973=CARTESIAN_POINT('Ctrl Pts',(-59.8287670060529,-101.979172801565,
172.515418850865));
#19974=CARTESIAN_POINT('Ctrl Pts',(-60.2848547374583,-101.898008987142,
172.780385782992));
#19975=CARTESIAN_POINT('Ctrl Pts',(-60.6562094364539,-101.828107748012,
173.157058062683));
#19976=CARTESIAN_POINT('Ctrl Pts',(-60.8101044574071,-101.799139614069,
173.313156769748));
#19977=CARTESIAN_POINT('Ctrl Pts',(-60.9459236613779,-101.771602184887,
173.485485069079));
#19978=CARTESIAN_POINT('Origin',(-57.8503443722502,-102.190085871961,175.985485069079));
#19979=CARTESIAN_POINT('Ctrl Pts',(-60.6425873069478,-101.892414120442,
173.485485069077));
#19980=CARTESIAN_POINT('Ctrl Pts',(-60.507560609551,-101.906808868484,173.25618146547));
#19981=CARTESIAN_POINT('Ctrl Pts',(-60.3677502586115,-101.921713585952,
173.078920934662));
#19982=CARTESIAN_POINT('Ctrl Pts',(-60.1377190475615,-101.946236449864,
172.805174418299));
#19983=CARTESIAN_POINT('Ctrl Pts',(-59.9888386836434,-101.962108091312,
172.654046519857));
#19984=CARTESIAN_POINT('Ctrl Pts',(-59.8287670060529,-101.979172801565,
172.515418850865));
#19985=CARTESIAN_POINT('Origin',(-51.4899841053611,-42.5281564925371,175.985485069079));
#19986=CARTESIAN_POINT('Origin',(-62.88786637536,-111.709716750739,178.985485069079));
#19987=CARTESIAN_POINT('Origin',(-52.5853897920404,-15.069651635714,178.985485069079));
#19988=CARTESIAN_POINT('Origin',(-67.998054881725,-13.4265585667677,178.985485069079));
#19989=CARTESIAN_POINT('Origin',(-52.5342226896633,-12.3683081541722,178.985485069079));
#19990=CARTESIAN_POINT('Origin',(-52.4446243855275,-13.6775759072102,178.985485069079));
#19991=CARTESIAN_POINT('Origin',(-53.9352248596064,8.10403203946808,178.985485069079));
#19992=CARTESIAN_POINT('Origin',(-39.4690592605811,9.0940082318961,178.985485069079));
#19993=CARTESIAN_POINT('Origin',(-52.9717383111942,-18.6937070505612,180.485485069079));
#19994=CARTESIAN_POINT('Origin',(-52.5853897920404,-15.069651635714,180.485485069079));
#19995=CARTESIAN_POINT('Origin',(-67.998054881725,-13.4265585667677,180.485485069079));
#19996=CARTESIAN_POINT('Origin',(-52.5342226896633,-12.3683081541722,180.485485069079));
#19997=CARTESIAN_POINT('Origin',(-51.890637311636,-21.772789521366,180.485485069079));
#19998=CARTESIAN_POINT('Origin',(-53.9352248596064,8.10403203946808,180.485485069079));
#19999=CARTESIAN_POINT('Origin',(-39.4690592605811,9.0940082318961,180.485485069079));
#20000=CARTESIAN_POINT('Origin',(-41.2825923197859,23.4801507949034,180.485485069079));
#20001=CARTESIAN_POINT('Origin',(-40.5289338663118,23.5751578139663,180.485485069079));
#20002=CARTESIAN_POINT('Origin',(-24.4968854027218,25.596175593274,180.485485069079));
#20003=CARTESIAN_POINT('Ctrl Pts',(-20.9569943874949,26.5463753651884,176.985485069079));
#20004=CARTESIAN_POINT('Ctrl Pts',(-20.3076118873532,26.6282372421243,176.985485069079));
#20005=CARTESIAN_POINT('Ctrl Pts',(-20.3993997459139,25.9801832417458,176.985485069079));
#20006=CARTESIAN_POINT('Ctrl Pts',(-20.9569943910055,26.5463753647458,177.220977963401));
#20007=CARTESIAN_POINT('Ctrl Pts',(-20.3076118917219,26.6282372415765,177.266627063424));
#20008=CARTESIAN_POINT('Ctrl Pts',(-20.3993997460441,25.9801832408266,177.254619805483));
#20009=CARTESIAN_POINT('Ctrl Pts',(-20.9811883709224,26.543325444851,177.45231830065));
#20010=CARTESIAN_POINT('Ctrl Pts',(-20.3376037120335,26.6244564394995,177.542172659695));
#20011=CARTESIAN_POINT('Ctrl Pts',(-20.4269246477449,25.9775831262692,177.519008762253));
#20012=CARTESIAN_POINT('Ctrl Pts',(-21.0757990735786,26.5313987149253,177.906973211595));
#20013=CARTESIAN_POINT('Ctrl Pts',(-20.4549506534422,26.6096635541441,178.083132559644));
#20014=CARTESIAN_POINT('Ctrl Pts',(-20.5345596128582,25.9674199466701,178.038614374861));
#20015=CARTESIAN_POINT('Ctrl Pts',(-21.1475020349058,26.522359760234,178.13275546379));
#20016=CARTESIAN_POINT('Ctrl Pts',(-20.5433816467323,26.5985158452194,178.350325889774));
#20017=CARTESIAN_POINT('Ctrl Pts',(-20.6161329571035,25.9597188096215,178.296651234969));
#20018=CARTESIAN_POINT('Ctrl Pts',(-21.3330091361947,26.4989745296601,178.56011431014));
#20019=CARTESIAN_POINT('Ctrl Pts',(-20.7717245231082,26.5697306894192,178.853810146054));
#20020=CARTESIAN_POINT('Ctrl Pts',(-20.8271720934702,25.9398095413006,178.785061344071));
#20021=CARTESIAN_POINT('Ctrl Pts',(-21.4462792894842,26.4846955687286,178.762334660914));
#20022=CARTESIAN_POINT('Ctrl Pts',(-20.9100975499512,26.5522872324514,179.090130315615));
#20023=CARTESIAN_POINT('Ctrl Pts',(-20.9560304163274,25.9276586659783,179.01617031644));
#20024=CARTESIAN_POINT('Ctrl Pts',(-21.7133004202462,26.4510345893506,179.144165737296));
#20025=CARTESIAN_POINT('Ctrl Pts',(-21.2350328903241,26.5113255236894,179.532928715243));
#20026=CARTESIAN_POINT('Ctrl Pts',(-21.2597905826465,25.8990431476073,179.452548690349));
#20027=CARTESIAN_POINT('Ctrl Pts',(-21.8670860845458,26.4316481982441,179.322751431888));
#20028=CARTESIAN_POINT('Ctrl Pts',(-21.4205619530434,26.4879375246306,179.737877540268));
#20029=CARTESIAN_POINT('Ctrl Pts',(-21.4347317392525,25.8825753022298,179.656646627006));
#20030=CARTESIAN_POINT('Ctrl Pts',(-22.2017889982529,26.3894551783737,179.642261663974));
#20031=CARTESIAN_POINT('Ctrl Pts',(-21.8221797156734,26.4373091448254,180.100434649856));
#20032=CARTESIAN_POINT('Ctrl Pts',(-21.8154653408504,25.8467781859745,180.0218011771));
#20033=CARTESIAN_POINT('Ctrl Pts',(-22.3846701288836,26.3664009805684,179.785713045127));
#20034=CARTESIAN_POINT('Ctrl Pts',(-22.0396265413609,26.4098975572291,180.261103787136));
#20035=CARTESIAN_POINT('Ctrl Pts',(-22.0234918530467,25.827238523971,180.185745614722));
#20036=CARTESIAN_POINT('Ctrl Pts',(-22.7786882937544,26.3167306144649,180.037038838909));
#20037=CARTESIAN_POINT('Ctrl Pts',(-22.5053049632146,26.3511936197905,180.538045339618));
#20038=CARTESIAN_POINT('Ctrl Pts',(-22.4716684057107,25.785200536956,180.472975090153));
#20039=CARTESIAN_POINT('Ctrl Pts',(-22.9847021376152,26.2907602812183,180.141806276838));
#20040=CARTESIAN_POINT('Ctrl Pts',(-22.7466972207022,26.3207634445538,180.651430961495));
#20041=CARTESIAN_POINT('Ctrl Pts',(-22.7059910527553,25.7632488339365,180.592709306442));
#20042=CARTESIAN_POINT('Ctrl Pts',(-23.6283960230643,26.2096155173486,180.39658255964));
#20043=CARTESIAN_POINT('Ctrl Pts',(-23.4895764797135,26.2271152626769,180.917343237008));
#20044=CARTESIAN_POINT('Ctrl Pts',(-23.4381054919345,25.6947662436456,180.883882201301));
#20045=CARTESIAN_POINT('Ctrl Pts',(-24.0961299454542,26.1506524612375,180.485485065088));
#20046=CARTESIAN_POINT('Ctrl Pts',(-24.0256564111632,26.1595364330049,181.003088599679));
#20047=CARTESIAN_POINT('Ctrl Pts',(-23.9700486532876,25.6451485909903,180.985485069078));
#20048=CARTESIAN_POINT('Ctrl Pts',(-24.559421025453,26.0922494747571,180.485485069079));
#20049=CARTESIAN_POINT('Ctrl Pts',(-24.5594210254521,26.0922494747572,180.98548506908));
#20050=CARTESIAN_POINT('Ctrl Pts',(-24.4968854027209,25.5961755932739,180.985485069079));
#20051=CARTESIAN_POINT('Origin',(-20.8944587647637,26.0503014837053,176.985485069079));
#20052=CARTESIAN_POINT('Origin',(-20.8944587647637,26.0503014837054,176.985485069079));
#20053=CARTESIAN_POINT('Origin',(-20.8944587647637,26.0503014837053,174.985485069079));
#20054=CARTESIAN_POINT('Ctrl Pts',(-24.5594210254598,26.0922494747562,171.485485069079));
#20055=CARTESIAN_POINT('Ctrl Pts',(-24.5594210254598,26.0922494747562,170.985485069079));
#20056=CARTESIAN_POINT('Ctrl Pts',(-24.4968854027286,25.5961755932732,170.985485069079));
#20057=CARTESIAN_POINT('Ctrl Pts',(-24.3258682437323,26.1216913970003,171.485485071833));
#20058=CARTESIAN_POINT('Ctrl Pts',(-24.2925991176692,26.1258853398606,170.976685296256));
#20059=CARTESIAN_POINT('Ctrl Pts',(-24.2312974837435,25.6208637654299,170.985485069079));
#20060=CARTESIAN_POINT('Ctrl Pts',(-24.0959501711783,26.1506751237818,171.507305910281));
#20061=CARTESIAN_POINT('Ctrl Pts',(-24.0306335816867,26.1589090053693,170.99304475765));
#20062=CARTESIAN_POINT('Ctrl Pts',(-23.9698304921285,25.6452096731348,171.010423173625));
#20063=CARTESIAN_POINT('Ctrl Pts',(-23.6431960794649,26.2077498058528,171.593014493502));
#20064=CARTESIAN_POINT('Ctrl Pts',(-23.5111338715838,26.2243977139913,171.073389718607));
#20065=CARTESIAN_POINT('Ctrl Pts',(-23.4549281292755,25.6932274759485,171.108375839534));
#20066=CARTESIAN_POINT('Ctrl Pts',(-23.4183852446137,26.2360897085949,171.657722381639));
#20067=CARTESIAN_POINT('Ctrl Pts',(-23.2514992137756,26.2571275464109,171.139086040182));
#20068=CARTESIAN_POINT('Ctrl Pts',(-23.1992466423954,25.717109596163,171.182327711039));
#20069=CARTESIAN_POINT('Ctrl Pts',(-22.9858808239905,26.2906116947088,171.828488317232));
#20070=CARTESIAN_POINT('Ctrl Pts',(-22.7480513169311,26.3205927456837,171.318813609326));
#20071=CARTESIAN_POINT('Ctrl Pts',(-22.7073317369307,25.7631231310235,171.37748878222));
#20072=CARTESIAN_POINT('Ctrl Pts',(-22.780301002694,26.3165273145905,171.933235555643));
#20073=CARTESIAN_POINT('Ctrl Pts',(-22.5072292845117,26.3509510377182,171.432160965498));
#20074=CARTESIAN_POINT('Ctrl Pts',(-22.473502682735,25.7850288237937,171.497199911615));
#20075=CARTESIAN_POINT('Ctrl Pts',(-22.3903890997892,26.3656800407642,172.181282504714));
#20076=CARTESIAN_POINT('Ctrl Pts',(-22.046448768076,26.4090375397752,171.705429397239));
#20077=CARTESIAN_POINT('Ctrl Pts',(-22.029997004347,25.8266280231631,171.780682137627));
#20078=CARTESIAN_POINT('Ctrl Pts',(-22.2042811099175,26.3891410200181,172.326561495445));
#20079=CARTESIAN_POINT('Ctrl Pts',(-21.8251478033509,26.4369349844039,171.86812412086));
#20080=CARTESIAN_POINT('Ctrl Pts',(-21.8183001416767,25.8465117976671,171.946715270196));
#20081=CARTESIAN_POINT('Ctrl Pts',(-21.8682914406808,26.4314962497153,172.646838591123));
#20082=CARTESIAN_POINT('Ctrl Pts',(-21.4220077743163,26.4877552628029,172.231518296184));
#20083=CARTESIAN_POINT('Ctrl Pts',(-21.4361029074071,25.8824462409076,172.312746237574));
#20084=CARTESIAN_POINT('Ctrl Pts',(-21.7172904392047,26.4505316031431,172.821893236395));
#20085=CARTESIAN_POINT('Ctrl Pts',(-21.23986603748,26.510716251808,172.432383047633));
#20086=CARTESIAN_POINT('Ctrl Pts',(-21.2643295137859,25.8986157996259,172.512808689673));
#20087=CARTESIAN_POINT('Ctrl Pts',(-21.4500317056124,26.484222534997,173.202497941726));
#20088=CARTESIAN_POINT('Ctrl Pts',(-20.9146824604562,26.5517092535569,172.873679335507));
#20089=CARTESIAN_POINT('Ctrl Pts',(-20.9602991882961,25.9272562971409,172.947785494157));
#20090=CARTESIAN_POINT('Ctrl Pts',(-21.3340158032727,26.4988476280937,173.409042585785));
#20091=CARTESIAN_POINT('Ctrl Pts',(-20.7729608251139,26.569574839814,173.115030751227));
#20092=CARTESIAN_POINT('Ctrl Pts',(-20.8283172958717,25.9397015531057,173.183836516651));
#20093=CARTESIAN_POINT('Ctrl Pts',(-21.1488654481888,26.522187886846,173.83457432462));
#20094=CARTESIAN_POINT('Ctrl Pts',(-20.5450665743191,26.598303441388,173.616334746953));
#20095=CARTESIAN_POINT('Ctrl Pts',(-20.6176840378571,25.9595724331803,173.670158504074));
#20096=CARTESIAN_POINT('Ctrl Pts',(-21.0779351096429,26.5311294438541,174.055717854822));
#20097=CARTESIAN_POINT('Ctrl Pts',(-20.4575919717946,26.6093305866297,173.878021756473));
#20098=CARTESIAN_POINT('Ctrl Pts',(-20.5369896936467,25.9671905184219,173.922893967463));
#20099=CARTESIAN_POINT('Ctrl Pts',(-20.9814287704556,26.5432951398197,174.515559365905));
#20100=CARTESIAN_POINT('Ctrl Pts',(-20.3378990677518,26.6244192066291,174.425122401938));
#20101=CARTESIAN_POINT('Ctrl Pts',(-20.427198146352,25.9775572759958,174.448427122202));
#20102=CARTESIAN_POINT('Ctrl Pts',(-20.9569943894572,26.546375364941,174.750471985775));
#20103=CARTESIAN_POINT('Ctrl Pts',(-20.3076118897997,26.6282372418308,174.704913517301));
#20104=CARTESIAN_POINT('Ctrl Pts',(-20.3993997459849,25.9801832412446,174.716898688454));
#20105=CARTESIAN_POINT('Ctrl Pts',(-20.9569943874949,26.5463753651883,174.985485069079));
#20106=CARTESIAN_POINT('Ctrl Pts',(-20.3076118873532,26.6282372421243,174.985485069079));
#20107=CARTESIAN_POINT('Ctrl Pts',(-20.3993997459139,25.9801832417458,174.985485069079));
#20108=CARTESIAN_POINT('Origin',(-24.4968854027286,25.5961755932732,171.485485069079));
#20109=CARTESIAN_POINT('Origin',(-55.3387939853426,21.7082104505275,171.485485069079));
#20110=CARTESIAN_POINT('Origin',(-41.2825923197859,23.4801507949034,171.485485069079));
#20111=CARTESIAN_POINT('Origin',(-39.4690592605811,9.0940082318961,171.485485069079));
#20112=CARTESIAN_POINT('Origin',(-53.9352248596064,8.10403203946808,171.485485069079));
#20113=CARTESIAN_POINT('Origin',(-52.4446243855275,-13.6775759072102,171.485485069079));
#20114=CARTESIAN_POINT('Origin',(-52.5342226896633,-12.3683081541722,171.485485069079));
#20115=CARTESIAN_POINT('Origin',(-67.998054881725,-13.4265585667677,171.485485069079));
#20116=CARTESIAN_POINT('Origin',(-52.5853897920404,-15.069651635714,171.485485069079));
#20117=CARTESIAN_POINT('Origin',(-62.88786637536,-111.709716750739,171.485485069079));
#20118=CARTESIAN_POINT('Ctrl Pts',(-56.2237961054143,-113.614380048479,
178.813912075476));
#20119=CARTESIAN_POINT('Ctrl Pts',(-55.0488864554725,-113.645352038053,
177.6423391512));
#20120=CARTESIAN_POINT('Ctrl Pts',(-55.0389484614927,-113.552130266048,
175.985484901707));
#20121=CARTESIAN_POINT('Ctrl Pts',(-55.0290104675128,-113.458908494044,
174.328630652215));
#20122=CARTESIAN_POINT('Ctrl Pts',(-56.1840440891124,-113.241492964766,
173.157057825983));
#20123=CARTESIAN_POINT('Ctrl Pts',(-57.3390777107121,-113.024077435489,
171.985484999752));
#20124=CARTESIAN_POINT('Ctrl Pts',(-58.9766583348819,-112.755219171892,
171.985485069079));
#20125=CARTESIAN_POINT('Ctrl Pts',(-60.6142389590518,-112.486360908295,
171.985485138407));
#20126=CARTESIAN_POINT('Ctrl Pts',(-61.7692724831595,-112.268945389411,
173.157058062683));
#20127=CARTESIAN_POINT('Ctrl Pts',(-62.9243060072673,-112.051529870527,
174.328630986959));
#20128=CARTESIAN_POINT('Ctrl Pts',(-62.9143678754131,-111.95830811322,175.985485236451));
#20129=CARTESIAN_POINT('Ctrl Pts',(-62.9044297435589,-111.865086355914,
177.642339485944));
#20130=CARTESIAN_POINT('Ctrl Pts',(-61.7295199961253,-111.896058355881,
178.813912312176));
#20131=CARTESIAN_POINT('Ctrl Pts',(-60.5546102486917,-111.927030355848,
179.985485138407));
#20132=CARTESIAN_POINT('Ctrl Pts',(-58.8971534986878,-112.009445090134,
179.985485069079));
#20133=CARTESIAN_POINT('Ctrl Pts',(-57.2396967486839,-112.09185982442,179.985484999752));
#20134=CARTESIAN_POINT('Ctrl Pts',(-56.0647870987421,-112.122831813994,
178.813912075476));
#20135=CARTESIAN_POINT('Ctrl Pts',(-54.8898774488003,-112.153803803567,
177.6423391512));
#20136=CARTESIAN_POINT('Ctrl Pts',(-54.8799394548205,-112.060582031563,
175.985484901707));
#20137=CARTESIAN_POINT('Ctrl Pts',(-54.8700014608406,-111.967360259558,
174.328630652215));
#20138=CARTESIAN_POINT('Ctrl Pts',(-56.0250350824402,-111.749944730281,
173.157057825983));
#20139=CARTESIAN_POINT('Ctrl Pts',(-57.1800687040398,-111.532529201003,
171.985484999752));
#20140=CARTESIAN_POINT('Ctrl Pts',(-58.8176493282097,-111.263670937406,
171.985485069079));
#20141=CARTESIAN_POINT('Ctrl Pts',(-60.4552299523796,-110.994812673809,
171.985485138407));
#20142=CARTESIAN_POINT('Ctrl Pts',(-61.6102634764873,-110.777397154925,
173.157058062683));
#20143=CARTESIAN_POINT('Ctrl Pts',(-62.7652970005951,-110.559981636041,
174.328630986959));
#20144=CARTESIAN_POINT('Ctrl Pts',(-62.7553588687409,-110.466759878735,
175.985485236451));
#20145=CARTESIAN_POINT('Ctrl Pts',(-62.7454207368867,-110.373538121429,
177.642339485944));
#20146=CARTESIAN_POINT('Ctrl Pts',(-61.5705109894531,-110.404510121395,
178.813912312176));
#20147=CARTESIAN_POINT('Ctrl Pts',(-60.3956012420194,-110.435482121362,
179.985485138407));
#20148=CARTESIAN_POINT('Ctrl Pts',(-58.7381444920155,-110.517896855648,
179.985485069079));
#20149=CARTESIAN_POINT('Ctrl Pts',(-57.0806877420116,-110.600311589935,
179.985484999752));
#20150=CARTESIAN_POINT('Ctrl Pts',(-55.9057780920699,-110.631283579508,
178.813912075476));
#20151=CARTESIAN_POINT('Ctrl Pts',(-54.7308684421281,-110.662255569082,
177.6423391512));
#20152=CARTESIAN_POINT('Ctrl Pts',(-54.7209304481482,-110.569033797077,
175.985484901707));
#20153=CARTESIAN_POINT('Ctrl Pts',(-54.7109924541684,-110.475812025073,
174.328630652215));
#20154=CARTESIAN_POINT('Ctrl Pts',(-55.866026075768,-110.258396495795,173.157057825983));
#20155=CARTESIAN_POINT('Ctrl Pts',(-57.0210596973676,-110.040980966518,
171.985484999752));
#20156=CARTESIAN_POINT('Ctrl Pts',(-58.6586403215375,-109.772122702921,
171.985485069079));
#20157=CARTESIAN_POINT('Ctrl Pts',(-60.2962209457073,-109.503264439324,
171.985485138407));
#20158=CARTESIAN_POINT('Ctrl Pts',(-61.4512544698151,-109.28584892044,173.157058062683));
#20159=CARTESIAN_POINT('Ctrl Pts',(-62.6062879939228,-109.068433401555,
174.328630986959));
#20160=CARTESIAN_POINT('Ctrl Pts',(-62.5963498620687,-108.975211644249,
175.985485236451));
#20161=CARTESIAN_POINT('Ctrl Pts',(-62.5864117302145,-108.881989886943,
177.642339485944));
#20162=CARTESIAN_POINT('Ctrl Pts',(-61.4115019827808,-108.91296188691,178.813912312176));
#20163=CARTESIAN_POINT('Ctrl Pts',(-60.2365922353472,-108.943933886877,
179.985485138407));
#20164=CARTESIAN_POINT('Ctrl Pts',(-58.5791354853433,-109.026348621163,
179.985485069079));
#20165=CARTESIAN_POINT('Ctrl Pts',(-56.9216787353394,-109.108763355449,
179.985484999752));
#20166=CARTESIAN_POINT('Ctrl Pts',(-55.7467690853976,-109.139735345023,
178.813912075476));
#20167=CARTESIAN_POINT('Ctrl Pts',(-54.5718594354559,-109.170707334596,
177.6423391512));
#20168=CARTESIAN_POINT('Ctrl Pts',(-54.561921441476,-109.077485562592,175.985484901707));
#20169=CARTESIAN_POINT('Ctrl Pts',(-54.5519834474962,-108.984263790587,
174.328630652215));
#20170=CARTESIAN_POINT('Ctrl Pts',(-55.7070170690958,-108.76684826131,173.157057825983));
#20171=CARTESIAN_POINT('Ctrl Pts',(-56.8620506906954,-108.549432732032,
171.985484999752));
#20172=CARTESIAN_POINT('Ctrl Pts',(-58.4996313148652,-108.280574468435,
171.985485069079));
#20173=CARTESIAN_POINT('Ctrl Pts',(-60.1372119390351,-108.011716204838,
171.985485138407));
#20174=CARTESIAN_POINT('Ctrl Pts',(-61.2922454631428,-107.794300685954,
173.157058062683));
#20175=CARTESIAN_POINT('Ctrl Pts',(-62.4472789872506,-107.57688516707,174.328630986959));
#20176=CARTESIAN_POINT('Ctrl Pts',(-62.4373408553964,-107.483663409764,
175.985485236451));
#20177=CARTESIAN_POINT('Ctrl Pts',(-62.4274027235423,-107.390441652457,
177.642339485944));
#20178=CARTESIAN_POINT('Ctrl Pts',(-61.2524929761086,-107.421413652424,
178.813912312176));
#20179=CARTESIAN_POINT('Ctrl Pts',(-60.077583228675,-107.452385652391,179.985485138407));
#20180=CARTESIAN_POINT('Ctrl Pts',(-58.4201264786711,-107.534800386677,
179.985485069079));
#20181=CARTESIAN_POINT('Ctrl Pts',(-56.7626697286672,-107.617215120964,
179.985484999752));
#20182=CARTESIAN_POINT('Ctrl Pts',(-55.5877600787254,-107.648187110537,
178.813912075476));
#20183=CARTESIAN_POINT('Ctrl Pts',(-54.4128504287836,-107.67915910011,177.6423391512));
#20184=CARTESIAN_POINT('Ctrl Pts',(-54.4029124348038,-107.585937328106,
175.985484901707));
#20185=CARTESIAN_POINT('Ctrl Pts',(-54.3929744408239,-107.492715556102,
174.328630652215));
#20186=CARTESIAN_POINT('Ctrl Pts',(-55.5480080624235,-107.275300026824,
173.157057825983));
#20187=CARTESIAN_POINT('Ctrl Pts',(-56.7030416840231,-107.057884497547,
171.985484999752));
#20188=CARTESIAN_POINT('Ctrl Pts',(-58.340622308193,-106.78902623395,171.985485069079));
#20189=CARTESIAN_POINT('Ctrl Pts',(-59.9782029323629,-106.520167970353,
171.985485138407));
#20190=CARTESIAN_POINT('Ctrl Pts',(-61.1332364564706,-106.302752451468,
173.157058062683));
#20191=CARTESIAN_POINT('Ctrl Pts',(-62.2882699805784,-106.085336932584,
174.328630986959));
#20192=CARTESIAN_POINT('Ctrl Pts',(-62.2783318487242,-105.992115175278,
175.985485236451));
#20193=CARTESIAN_POINT('Ctrl Pts',(-62.26839371687,-105.898893417972,177.642339485944));
#20194=CARTESIAN_POINT('Ctrl Pts',(-61.0934839694364,-105.929865417939,
178.813912312176));
#20195=CARTESIAN_POINT('Ctrl Pts',(-59.9185742220028,-105.960837417905,
179.985485138407));
#20196=CARTESIAN_POINT('Ctrl Pts',(-58.2611174719989,-106.043252152192,
179.985485069079));
#20197=CARTESIAN_POINT('Ctrl Pts',(-56.603660721995,-106.125666886478,179.985484999752));
#20198=CARTESIAN_POINT('Ctrl Pts',(-55.4287510720532,-106.156638876051,
178.813912075476));
#20199=CARTESIAN_POINT('Ctrl Pts',(-54.2538414221114,-106.187610865625,
177.6423391512));
#20200=CARTESIAN_POINT('Ctrl Pts',(-54.2439034281315,-106.09438909362,175.985484901707));
#20201=CARTESIAN_POINT('Ctrl Pts',(-54.2339654341517,-106.001167321616,
174.328630652215));
#20202=CARTESIAN_POINT('Ctrl Pts',(-55.3889990557513,-105.783751792338,
173.157057825983));
#20203=CARTESIAN_POINT('Ctrl Pts',(-56.5440326773509,-105.566336263061,
171.985484999752));
#20204=CARTESIAN_POINT('Ctrl Pts',(-58.1816133015208,-105.297477999464,
171.985485069079));
#20205=CARTESIAN_POINT('Ctrl Pts',(-59.8191939256906,-105.028619735867,
171.985485138407));
#20206=CARTESIAN_POINT('Ctrl Pts',(-60.9742274497984,-104.811204216983,
173.157058062683));
#20207=CARTESIAN_POINT('Ctrl Pts',(-62.1292609739061,-104.593788698099,
174.328630986959));
#20208=CARTESIAN_POINT('Ctrl Pts',(-62.119322842052,-104.500566940792,175.985485236451));
#20209=CARTESIAN_POINT('Ctrl Pts',(-62.1093847101978,-104.407345183486,
177.642339485944));
#20210=CARTESIAN_POINT('Ctrl Pts',(-60.9344749627642,-104.438317183453,
178.813912312176));
#20211=CARTESIAN_POINT('Ctrl Pts',(-59.7595652153305,-104.46928918342,179.985485138407));
#20212=CARTESIAN_POINT('Ctrl Pts',(-58.1021084653266,-104.551703917706,
179.985485069079));
#20213=CARTESIAN_POINT('Ctrl Pts',(-56.4446517153227,-104.634118651992,
179.985484999752));
#20214=CARTESIAN_POINT('Ctrl Pts',(-55.269742065381,-104.665090641566,178.813912075476));
#20215=CARTESIAN_POINT('Ctrl Pts',(-54.0948324154392,-104.696062631139,
177.6423391512));
#20216=CARTESIAN_POINT('Ctrl Pts',(-54.0848944214593,-104.602840859135,
175.985484901707));
#20217=CARTESIAN_POINT('Ctrl Pts',(-54.0749564274795,-104.50961908713,174.328630652215));
#20218=CARTESIAN_POINT('Ctrl Pts',(-55.2299900490791,-104.292203557853,
173.157057825983));
#20219=CARTESIAN_POINT('Ctrl Pts',(-56.3850236706787,-104.074788028575,
171.985484999752));
#20220=CARTESIAN_POINT('Ctrl Pts',(-58.0226042948486,-103.805929764978,
171.985485069079));
#20221=CARTESIAN_POINT('Ctrl Pts',(-59.6601849190184,-103.537071501381,
171.985485138407));
#20222=CARTESIAN_POINT('Ctrl Pts',(-60.8152184431262,-103.319655982497,
173.157058062683));
#20223=CARTESIAN_POINT('Ctrl Pts',(-61.9702519672339,-103.102240463613,
174.328630986959));
#20224=CARTESIAN_POINT('Ctrl Pts',(-61.9603138353797,-103.009018706307,
175.985485236451));
#20225=CARTESIAN_POINT('Ctrl Pts',(-61.9503757035256,-102.915796949001,
177.642339485944));
#20226=CARTESIAN_POINT('Ctrl Pts',(-60.7754659560919,-102.946768948967,
178.813912312176));
#20227=CARTESIAN_POINT('Ctrl Pts',(-59.6005562086583,-102.977740948934,
179.985485138407));
#20228=CARTESIAN_POINT('Ctrl Pts',(-57.9430994586544,-103.06015568322,179.985485069079));
#20229=CARTESIAN_POINT('Ctrl Pts',(-56.2856427086505,-103.142570417507,
179.985484999752));
#20230=CARTESIAN_POINT('Ctrl Pts',(-55.1107330587087,-103.17354240708,178.813912075476));
#20231=CARTESIAN_POINT('Ctrl Pts',(-53.935823408767,-103.204514396654,177.6423391512));
#20232=CARTESIAN_POINT('Ctrl Pts',(-53.9258854147871,-103.111292624649,
175.985484901707));
#20233=CARTESIAN_POINT('Ctrl Pts',(-53.9159474208072,-103.018070852645,
174.328630652215));
#20234=CARTESIAN_POINT('Ctrl Pts',(-55.0709810424069,-102.800655323367,
173.157057825983));
#20235=CARTESIAN_POINT('Ctrl Pts',(-56.2260146640065,-102.58323979409,171.985484999752));
#20236=CARTESIAN_POINT('Ctrl Pts',(-57.8635952881763,-102.314381530493,
171.985485069079));
#20237=CARTESIAN_POINT('Ctrl Pts',(-59.5011759123462,-102.045523266896,
171.985485138407));
#20238=CARTESIAN_POINT('Ctrl Pts',(-60.6562094364539,-101.828107748012,
173.157058062683));
#20239=CARTESIAN_POINT('Ctrl Pts',(-61.8112429605617,-101.610692229127,
174.328630986959));
#20240=CARTESIAN_POINT('Ctrl Pts',(-61.8013048287075,-101.517470471821,
175.985485236451));
#20241=CARTESIAN_POINT('Ctrl Pts',(-61.7913666968533,-101.424248714515,
177.642339485944));
#20242=CARTESIAN_POINT('Ctrl Pts',(-60.6164569494197,-101.455220714482,
178.813912312176));
#20243=CARTESIAN_POINT('Ctrl Pts',(-59.4415472019861,-101.486192714449,
179.985485138407));
#20244=CARTESIAN_POINT('Ctrl Pts',(-57.7840904519822,-101.568607448735,
179.985485069079));
#20245=CARTESIAN_POINT('Ctrl Pts',(-56.1266337019783,-101.651022183021,
179.985484999752));
#20246=CARTESIAN_POINT('Ctrl Pts',(-54.9517240520365,-101.681994172595,
178.813912075476));
#20247=CARTESIAN_POINT('Ctrl Pts',(-53.7768144020947,-101.712966162168,
177.6423391512));
#20248=CARTESIAN_POINT('Ctrl Pts',(-53.7668764081149,-101.619744390164,
175.985484901707));
#20249=CARTESIAN_POINT('Ctrl Pts',(-53.756938414135,-101.526522618159,174.328630652215));
#20250=CARTESIAN_POINT('Ctrl Pts',(-54.9119720357346,-101.309107088882,
173.157057825983));
#20251=CARTESIAN_POINT('Ctrl Pts',(-56.0670056573342,-101.091691559604,
171.985484999752));
#20252=CARTESIAN_POINT('Ctrl Pts',(-57.7045862815041,-100.822833296007,
171.985485069079));
#20253=CARTESIAN_POINT('Ctrl Pts',(-59.342166905674,-100.55397503241,171.985485138407));
#20254=CARTESIAN_POINT('Ctrl Pts',(-60.4972004297817,-100.336559513526,
173.157058062683));
#20255=CARTESIAN_POINT('Ctrl Pts',(-61.6522339538895,-100.119143994642,
174.328630986959));
#20256=CARTESIAN_POINT('Ctrl Pts',(-61.6422958220353,-100.025922237336,
175.985485236451));
#20257=CARTESIAN_POINT('Ctrl Pts',(-61.6323576901811,-99.9327004800294,
177.642339485944));
#20258=CARTESIAN_POINT('Ctrl Pts',(-60.4574479427475,-99.9636724799962,
178.813912312176));
#20259=CARTESIAN_POINT('Ctrl Pts',(-59.2825381953138,-99.994644479963,179.985485138407));
#20260=CARTESIAN_POINT('Ctrl Pts',(-57.6250814453099,-100.077059214249,
179.985485069079));
#20261=CARTESIAN_POINT('Ctrl Pts',(-55.9676246953061,-100.159473948536,
179.985484999752));
#20262=CARTESIAN_POINT('Ctrl Pts',(-54.7927150453643,-100.190445938109,
178.813912075476));
#20263=CARTESIAN_POINT('Ctrl Pts',(-53.6178053954225,-100.221417927683,
177.6423391512));
#20264=CARTESIAN_POINT('Ctrl Pts',(-53.6078674014426,-100.128196155678,
175.985484901707));
#20265=CARTESIAN_POINT('Ctrl Pts',(-53.5979294074628,-100.034974383673,
174.328630652215));
#20266=CARTESIAN_POINT('Ctrl Pts',(-54.7529630290624,-99.817558854396,173.157057825983));
#20267=CARTESIAN_POINT('Ctrl Pts',(-55.907996650662,-99.6001433251185,171.985484999752));
#20268=CARTESIAN_POINT('Ctrl Pts',(-57.5455772748319,-99.3312850615215,
171.985485069079));
#20269=CARTESIAN_POINT('Ctrl Pts',(-59.1831578990017,-99.0624267979246,
171.985485138407));
#20270=CARTESIAN_POINT('Ctrl Pts',(-60.3381914231095,-98.8450112790404,
173.157058062683));
#20271=CARTESIAN_POINT('Ctrl Pts',(-61.4932249472172,-98.6275957601562,
174.328630986959));
#20272=CARTESIAN_POINT('Ctrl Pts',(-61.4832868153631,-98.53437400285,175.985485236451));
#20273=CARTESIAN_POINT('Ctrl Pts',(-61.4733486835089,-98.4411522455438,
177.642339485944));
#20274=CARTESIAN_POINT('Ctrl Pts',(-60.2984389360752,-98.4721242455106,
178.813912312176));
#20275=CARTESIAN_POINT('Ctrl Pts',(-59.1235291886416,-98.5030962454774,
179.985485138407));
#20276=CARTESIAN_POINT('Ctrl Pts',(-57.4660724386377,-98.5855109797636,
179.985485069079));
#20277=CARTESIAN_POINT('Ctrl Pts',(-55.8086156886338,-98.6679257140499,
179.985484999752));
#20278=CARTESIAN_POINT('Ctrl Pts',(-54.633706038692,-98.6988977036234,178.813912075476));
#20279=CARTESIAN_POINT('Ctrl Pts',(-56.9964983346804,-113.864655531781,
178.072094410988));
#20280=CARTESIAN_POINT('Ctrl Pts',(-56.1271283009022,-113.863054956993,
177.207792449865));
#20281=CARTESIAN_POINT('Ctrl Pts',(-56.117190288842,-113.769833186916,175.985484945604));
#20282=CARTESIAN_POINT('Ctrl Pts',(-56.1072522767819,-113.676611416839,
174.763177441344));
#20283=CARTESIAN_POINT('Ctrl Pts',(-56.9567462566485,-113.491768454648,
173.89887555255));
#20284=CARTESIAN_POINT('Ctrl Pts',(-57.8062402365152,-113.306925492458,
173.034573663757));
#20285=CARTESIAN_POINT('Ctrl Pts',(-59.011722573584,-113.084131793069,173.034573714903));
#20286=CARTESIAN_POINT('Ctrl Pts',(-60.2172049106529,-112.86133809368,173.034573766048));
#20287=CARTESIAN_POINT('Ctrl Pts',(-61.0666988185971,-112.676495139156,
173.898875727171));
#20288=CARTESIAN_POINT('Ctrl Pts',(-61.9161927265413,-112.491652184633,
174.763177688294));
#20289=CARTESIAN_POINT('Ctrl Pts',(-61.9062546127674,-112.398430425399,
175.985485192554));
#20290=CARTESIAN_POINT('Ctrl Pts',(-61.8963164989935,-112.305208666166,
177.207792696815));
#20291=CARTESIAN_POINT('Ctrl Pts',(-61.0269463932928,-112.303608099046,
178.072094585608));
#20292=CARTESIAN_POINT('Ctrl Pts',(-60.1575762875921,-112.302007531926,
178.936396474401));
#20293=CARTESIAN_POINT('Ctrl Pts',(-58.9322178246893,-112.338357702004,
178.936396423256));
#20294=CARTESIAN_POINT('Ctrl Pts',(-57.7068593617864,-112.374707872082,
178.936396372111));
#20295=CARTESIAN_POINT('Ctrl Pts',(-56.8374893280082,-112.373107297295,
178.072094410988));
#20296=CARTESIAN_POINT('Ctrl Pts',(-55.9681192942299,-112.371506722508,
177.207792449865));
#20297=CARTESIAN_POINT('Ctrl Pts',(-55.9581812821698,-112.278284952431,
175.985484945604));
#20298=CARTESIAN_POINT('Ctrl Pts',(-55.9482432701096,-112.185063182354,
174.763177441344));
#20299=CARTESIAN_POINT('Ctrl Pts',(-56.7977372499763,-112.000220220163,
173.89887555255));
#20300=CARTESIAN_POINT('Ctrl Pts',(-57.647231229843,-111.815377257972,173.034573663757));
#20301=CARTESIAN_POINT('Ctrl Pts',(-58.8527135669118,-111.592583558583,
173.034573714903));
#20302=CARTESIAN_POINT('Ctrl Pts',(-60.0581959039807,-111.369789859194,
173.034573766048));
#20303=CARTESIAN_POINT('Ctrl Pts',(-60.9076898119249,-111.184946904671,
173.898875727171));
#20304=CARTESIAN_POINT('Ctrl Pts',(-61.7571837198691,-111.000103950148,
174.763177688294));
#20305=CARTESIAN_POINT('Ctrl Pts',(-61.7472456060952,-110.906882190914,
175.985485192554));
#20306=CARTESIAN_POINT('Ctrl Pts',(-61.7373074923213,-110.81366043168,177.207792696815));
#20307=CARTESIAN_POINT('Ctrl Pts',(-60.8679373866206,-110.81205986456,178.072094585608));
#20308=CARTESIAN_POINT('Ctrl Pts',(-59.9985672809199,-110.81045929744,178.936396474401));
#20309=CARTESIAN_POINT('Ctrl Pts',(-58.7732088180171,-110.846809467519,
178.936396423256));
#20310=CARTESIAN_POINT('Ctrl Pts',(-57.5478503551142,-110.883159637597,
178.936396372111));
#20311=CARTESIAN_POINT('Ctrl Pts',(-56.6784803213359,-110.881559062809,
178.072094410988));
#20312=CARTESIAN_POINT('Ctrl Pts',(-55.8091102875577,-110.879958488022,
177.207792449865));
#20313=CARTESIAN_POINT('Ctrl Pts',(-55.7991722754976,-110.786736717945,
175.985484945604));
#20314=CARTESIAN_POINT('Ctrl Pts',(-55.7892342634374,-110.693514947868,
174.763177441344));
#20315=CARTESIAN_POINT('Ctrl Pts',(-56.6387282433041,-110.508671985677,
173.89887555255));
#20316=CARTESIAN_POINT('Ctrl Pts',(-57.4882222231708,-110.323829023487,
173.034573663757));
#20317=CARTESIAN_POINT('Ctrl Pts',(-58.6937045602396,-110.101035324098,
173.034573714903));
#20318=CARTESIAN_POINT('Ctrl Pts',(-59.8991868973084,-109.878241624709,
173.034573766048));
#20319=CARTESIAN_POINT('Ctrl Pts',(-60.7486808052526,-109.693398670185,
173.898875727171));
#20320=CARTESIAN_POINT('Ctrl Pts',(-61.5981747131968,-109.508555715662,
174.763177688294));
#20321=CARTESIAN_POINT('Ctrl Pts',(-61.588236599423,-109.415333956428,175.985485192554));
#20322=CARTESIAN_POINT('Ctrl Pts',(-61.5782984856491,-109.322112197195,
177.207792696815));
#20323=CARTESIAN_POINT('Ctrl Pts',(-60.7089283799484,-109.320511630075,
178.072094585608));
#20324=CARTESIAN_POINT('Ctrl Pts',(-59.8395582742477,-109.318911062955,
178.936396474401));
#20325=CARTESIAN_POINT('Ctrl Pts',(-58.6141998113448,-109.355261233033,
178.936396423256));
#20326=CARTESIAN_POINT('Ctrl Pts',(-57.388841348442,-109.391611403111,178.936396372111));
#20327=CARTESIAN_POINT('Ctrl Pts',(-56.5194713146637,-109.390010828324,
178.072094410988));
#20328=CARTESIAN_POINT('Ctrl Pts',(-55.6501012808855,-109.388410253536,
177.207792449865));
#20329=CARTESIAN_POINT('Ctrl Pts',(-55.6401632688253,-109.295188483459,
175.985484945604));
#20330=CARTESIAN_POINT('Ctrl Pts',(-55.6302252567652,-109.201966713382,
174.763177441344));
#20331=CARTESIAN_POINT('Ctrl Pts',(-56.4797192366319,-109.017123751192,
173.89887555255));
#20332=CARTESIAN_POINT('Ctrl Pts',(-57.3292132164985,-108.832280789001,
173.034573663757));
#20333=CARTESIAN_POINT('Ctrl Pts',(-58.5346955535674,-108.609487089612,
173.034573714903));
#20334=CARTESIAN_POINT('Ctrl Pts',(-59.7401778906362,-108.386693390223,
173.034573766048));
#20335=CARTESIAN_POINT('Ctrl Pts',(-60.5896717985804,-108.2018504357,173.898875727171));
#20336=CARTESIAN_POINT('Ctrl Pts',(-61.4391657065246,-108.017007481176,
174.763177688294));
#20337=CARTESIAN_POINT('Ctrl Pts',(-61.4292275927507,-107.923785721943,
175.985485192554));
#20338=CARTESIAN_POINT('Ctrl Pts',(-61.4192894789769,-107.830563962709,
177.207792696815));
#20339=CARTESIAN_POINT('Ctrl Pts',(-60.5499193732762,-107.828963395589,
178.072094585608));
#20340=CARTESIAN_POINT('Ctrl Pts',(-59.6805492675755,-107.827362828469,
178.936396474401));
#20341=CARTESIAN_POINT('Ctrl Pts',(-58.4551908046726,-107.863712998547,
178.936396423256));
#20342=CARTESIAN_POINT('Ctrl Pts',(-57.2298323417698,-107.900063168626,
178.936396372111));
#20343=CARTESIAN_POINT('Ctrl Pts',(-56.3604623079915,-107.898462593838,
178.072094410988));
#20344=CARTESIAN_POINT('Ctrl Pts',(-55.4910922742133,-107.896862019051,
177.207792449865));
#20345=CARTESIAN_POINT('Ctrl Pts',(-55.4811542621531,-107.803640248974,
175.985484945604));
#20346=CARTESIAN_POINT('Ctrl Pts',(-55.471216250093,-107.710418478897,174.763177441344));
#20347=CARTESIAN_POINT('Ctrl Pts',(-56.3207102299596,-107.525575516706,
173.89887555255));
#20348=CARTESIAN_POINT('Ctrl Pts',(-57.1702042098263,-107.340732554515,
173.034573663757));
#20349=CARTESIAN_POINT('Ctrl Pts',(-58.3756865468951,-107.117938855126,
173.034573714903));
#20350=CARTESIAN_POINT('Ctrl Pts',(-59.581168883964,-106.895145155737,173.034573766048));
#20351=CARTESIAN_POINT('Ctrl Pts',(-60.4306627919082,-106.710302201214,
173.898875727171));
#20352=CARTESIAN_POINT('Ctrl Pts',(-61.2801566998524,-106.525459246691,
174.763177688294));
#20353=CARTESIAN_POINT('Ctrl Pts',(-61.2702185860785,-106.432237487457,
175.985485192554));
#20354=CARTESIAN_POINT('Ctrl Pts',(-61.2602804723046,-106.339015728223,
177.207792696815));
#20355=CARTESIAN_POINT('Ctrl Pts',(-60.3909103666039,-106.337415161103,
178.072094585608));
#20356=CARTESIAN_POINT('Ctrl Pts',(-59.5215402609032,-106.335814593983,
178.936396474401));
#20357=CARTESIAN_POINT('Ctrl Pts',(-58.2961817980004,-106.372164764062,
178.936396423256));
#20358=CARTESIAN_POINT('Ctrl Pts',(-57.0708233350975,-106.40851493414,178.936396372111));
#20359=CARTESIAN_POINT('Ctrl Pts',(-56.2014533013193,-106.406914359353,
178.072094410988));
#20360=CARTESIAN_POINT('Ctrl Pts',(-55.332083267541,-106.405313784565,177.207792449865));
#20361=CARTESIAN_POINT('Ctrl Pts',(-55.3221452554809,-106.312092014488,
175.985484945604));
#20362=CARTESIAN_POINT('Ctrl Pts',(-55.3122072434207,-106.218870244411,
174.763177441344));
#20363=CARTESIAN_POINT('Ctrl Pts',(-56.1617012232874,-106.034027282221,
173.89887555255));
#20364=CARTESIAN_POINT('Ctrl Pts',(-57.0111952031541,-105.84918432003,173.034573663757));
#20365=CARTESIAN_POINT('Ctrl Pts',(-58.2166775402229,-105.626390620641,
173.034573714903));
#20366=CARTESIAN_POINT('Ctrl Pts',(-59.4221598772917,-105.403596921252,
173.034573766048));
#20367=CARTESIAN_POINT('Ctrl Pts',(-60.2716537852359,-105.218753966728,
173.898875727171));
#20368=CARTESIAN_POINT('Ctrl Pts',(-61.1211476931802,-105.033911012205,
174.763177688294));
#20369=CARTESIAN_POINT('Ctrl Pts',(-61.1112095794063,-104.940689252971,
175.985485192554));
#20370=CARTESIAN_POINT('Ctrl Pts',(-61.1012714656324,-104.847467493738,
177.207792696815));
#20371=CARTESIAN_POINT('Ctrl Pts',(-60.2319013599317,-104.845866926618,
178.072094585608));
#20372=CARTESIAN_POINT('Ctrl Pts',(-59.362531254231,-104.844266359498,178.936396474401));
#20373=CARTESIAN_POINT('Ctrl Pts',(-58.1371727913281,-104.880616529576,
178.936396423256));
#20374=CARTESIAN_POINT('Ctrl Pts',(-56.9118143284253,-104.916966699654,
178.936396372111));
#20375=CARTESIAN_POINT('Ctrl Pts',(-56.042444294647,-104.915366124867,178.072094410988));
#20376=CARTESIAN_POINT('Ctrl Pts',(-55.1730742608688,-104.91376555008,177.207792449865));
#20377=CARTESIAN_POINT('Ctrl Pts',(-55.1631362488087,-104.820543780003,
175.985484945604));
#20378=CARTESIAN_POINT('Ctrl Pts',(-55.1531982367485,-104.727322009926,
174.763177441344));
#20379=CARTESIAN_POINT('Ctrl Pts',(-56.0026922166152,-104.542479047735,
173.89887555255));
#20380=CARTESIAN_POINT('Ctrl Pts',(-56.8521861964818,-104.357636085544,
173.034573663757));
#20381=CARTESIAN_POINT('Ctrl Pts',(-58.0576685335507,-104.134842386155,
173.034573714903));
#20382=CARTESIAN_POINT('Ctrl Pts',(-59.2631508706195,-103.912048686766,
173.034573766048));
#20383=CARTESIAN_POINT('Ctrl Pts',(-60.1126447785637,-103.727205732243,
173.898875727171));
#20384=CARTESIAN_POINT('Ctrl Pts',(-60.9621386865079,-103.54236277772,174.763177688294));
#20385=CARTESIAN_POINT('Ctrl Pts',(-60.952200572734,-103.449141018486,175.985485192554));
#20386=CARTESIAN_POINT('Ctrl Pts',(-60.9422624589602,-103.355919259252,
177.207792696815));
#20387=CARTESIAN_POINT('Ctrl Pts',(-60.0728923532595,-103.354318692132,
178.072094585608));
#20388=CARTESIAN_POINT('Ctrl Pts',(-59.2035222475588,-103.352718125012,
178.936396474401));
#20389=CARTESIAN_POINT('Ctrl Pts',(-57.9781637846559,-103.389068295091,
178.936396423256));
#20390=CARTESIAN_POINT('Ctrl Pts',(-56.7528053217531,-103.425418465169,
178.936396372111));
#20391=CARTESIAN_POINT('Ctrl Pts',(-55.8834352879748,-103.423817890381,
178.072094410988));
#20392=CARTESIAN_POINT('Ctrl Pts',(-55.0140652541966,-103.422217315594,
177.207792449865));
#20393=CARTESIAN_POINT('Ctrl Pts',(-55.0041272421364,-103.328995545517,
175.985484945604));
#20394=CARTESIAN_POINT('Ctrl Pts',(-54.9941892300763,-103.23577377544,174.763177441344));
#20395=CARTESIAN_POINT('Ctrl Pts',(-55.8436832099429,-103.050930813249,
173.89887555255));
#20396=CARTESIAN_POINT('Ctrl Pts',(-56.6931771898096,-102.866087851059,
173.034573663757));
#20397=CARTESIAN_POINT('Ctrl Pts',(-57.8986595268784,-102.64329415167,173.034573714903));
#20398=CARTESIAN_POINT('Ctrl Pts',(-59.1041418639473,-102.420500452281,
173.034573766048));
#20399=CARTESIAN_POINT('Ctrl Pts',(-59.9536357718915,-102.235657497757,
173.898875727171));
#20400=CARTESIAN_POINT('Ctrl Pts',(-60.8031296798357,-102.050814543234,
174.763177688294));
#20401=CARTESIAN_POINT('Ctrl Pts',(-60.7931915660618,-101.957592784,175.985485192554));
#20402=CARTESIAN_POINT('Ctrl Pts',(-60.783253452288,-101.864371024767,177.207792696815));
#20403=CARTESIAN_POINT('Ctrl Pts',(-59.9138833465873,-101.862770457647,
178.072094585608));
#20404=CARTESIAN_POINT('Ctrl Pts',(-59.0445132408866,-101.861169890527,
178.936396474401));
#20405=CARTESIAN_POINT('Ctrl Pts',(-57.8191547779837,-101.897520060605,
178.936396423256));
#20406=CARTESIAN_POINT('Ctrl Pts',(-56.5937963150808,-101.933870230683,
178.936396372111));
#20407=CARTESIAN_POINT('Ctrl Pts',(-55.7244262813026,-101.932269655896,
178.072094410988));
#20408=CARTESIAN_POINT('Ctrl Pts',(-54.8550562475244,-101.930669081108,
177.207792449865));
#20409=CARTESIAN_POINT('Ctrl Pts',(-54.8451182354642,-101.837447311031,
175.985484945604));
#20410=CARTESIAN_POINT('Ctrl Pts',(-54.8351802234041,-101.744225540954,
174.763177441344));
#20411=CARTESIAN_POINT('Ctrl Pts',(-55.6846742032707,-101.559382578764,
173.89887555255));
#20412=CARTESIAN_POINT('Ctrl Pts',(-56.5341681831374,-101.374539616573,
173.034573663757));
#20413=CARTESIAN_POINT('Ctrl Pts',(-57.7396505202062,-101.151745917184,
173.034573714903));
#20414=CARTESIAN_POINT('Ctrl Pts',(-58.9451328572751,-100.928952217795,
173.034573766048));
#20415=CARTESIAN_POINT('Ctrl Pts',(-59.7946267652193,-100.744109263272,
173.898875727171));
#20416=CARTESIAN_POINT('Ctrl Pts',(-60.6441206731635,-100.559266308748,
174.763177688294));
#20417=CARTESIAN_POINT('Ctrl Pts',(-60.6341825593896,-100.466044549515,
175.985485192554));
#20418=CARTESIAN_POINT('Ctrl Pts',(-60.6242444456157,-100.372822790281,
177.207792696815));
#20419=CARTESIAN_POINT('Ctrl Pts',(-59.754874339915,-100.371222223161,178.072094585608));
#20420=CARTESIAN_POINT('Ctrl Pts',(-58.8855042342143,-100.369621656041,
178.936396474401));
#20421=CARTESIAN_POINT('Ctrl Pts',(-57.6601457713115,-100.405971826119,
178.936396423256));
#20422=CARTESIAN_POINT('Ctrl Pts',(-56.4347873084086,-100.442321996198,
178.936396372111));
#20423=CARTESIAN_POINT('Ctrl Pts',(-55.5654172746304,-100.44072142141,178.072094410988));
#20424=CARTESIAN_POINT('Ctrl Pts',(-54.6960472408521,-100.439120846623,
177.207792449865));
#20425=CARTESIAN_POINT('Ctrl Pts',(-54.686109228792,-100.345899076546,175.985484945604));
#20426=CARTESIAN_POINT('Ctrl Pts',(-54.6761712167318,-100.252677306469,
174.763177441344));
#20427=CARTESIAN_POINT('Ctrl Pts',(-55.5256651965985,-100.067834344278,
173.89887555255));
#20428=CARTESIAN_POINT('Ctrl Pts',(-56.3751591764652,-99.8829913820874,
173.034573663757));
#20429=CARTESIAN_POINT('Ctrl Pts',(-57.580641513534,-99.6601976826983,173.034573714903));
#20430=CARTESIAN_POINT('Ctrl Pts',(-58.7861238506028,-99.4374039833093,
173.034573766048));
#20431=CARTESIAN_POINT('Ctrl Pts',(-59.635617758547,-99.252561028786,173.898875727171));
#20432=CARTESIAN_POINT('Ctrl Pts',(-60.4851116664912,-99.0677180742627,
174.763177688294));
#20433=CARTESIAN_POINT('Ctrl Pts',(-60.4751735527174,-98.9744963150291,
175.985485192554));
#20434=CARTESIAN_POINT('Ctrl Pts',(-60.4652354389435,-98.8812745557954,
177.207792696815));
#20435=CARTESIAN_POINT('Ctrl Pts',(-59.5958653332428,-98.8796739886754,
178.072094585608));
#20436=CARTESIAN_POINT('Ctrl Pts',(-58.7264952275421,-98.8780734215554,
178.936396474401));
#20437=CARTESIAN_POINT('Ctrl Pts',(-57.5011367646392,-98.9144235916337,
178.936396423256));
#20438=CARTESIAN_POINT('Ctrl Pts',(-56.2757783017364,-98.9507737617121,
178.936396372111));
#20439=CARTESIAN_POINT('Ctrl Pts',(-55.4064082679581,-98.9491731869247,
178.072094410988));
#20440=CARTESIAN_POINT('Ctrl Pts',(-61.0705815801248,-102.940927762808,
178.485485069079));
#20441=CARTESIAN_POINT('Ctrl Pts',(-60.9320093757681,-102.942642280685,
178.657813499464));
#20442=CARTESIAN_POINT('Ctrl Pts',(-60.7754659560919,-102.946768948967,
178.813912312176));
#20443=CARTESIAN_POINT('Ctrl Pts',(-59.6005562086583,-102.977740948934,
179.985485138407));
#20444=CARTESIAN_POINT('Ctrl Pts',(-57.9430994586544,-103.06015568322,179.985485069079));
#20445=CARTESIAN_POINT('Ctrl Pts',(-56.2856427086505,-103.142570417507,
179.985484999752));
#20446=CARTESIAN_POINT('Ctrl Pts',(-55.1107330587087,-103.17354240708,178.813912075476));
#20447=CARTESIAN_POINT('Ctrl Pts',(-53.935823408767,-103.204514396654,177.6423391512));
#20448=CARTESIAN_POINT('Ctrl Pts',(-53.9258854147871,-103.111292624649,
175.985484901707));
#20449=CARTESIAN_POINT('Ctrl Pts',(-53.9159474208072,-103.018070852645,
174.328630652215));
#20450=CARTESIAN_POINT('Ctrl Pts',(-55.0709810424069,-102.800655323367,
173.157057825983));
#20451=CARTESIAN_POINT('Ctrl Pts',(-56.2260146640065,-102.58323979409,171.985484999752));
#20452=CARTESIAN_POINT('Ctrl Pts',(-57.8635952881763,-102.314381530493,
171.985485069079));
#20453=CARTESIAN_POINT('Ctrl Pts',(-58.9165917619278,-102.141500391495,
171.985485113659));
#20454=CARTESIAN_POINT('Ctrl Pts',(-59.8287670060529,-101.979172801565,
172.515418850865));
#20455=CARTESIAN_POINT('Ctrl Pts',(-56.8733667677527,-112.709647553905,
178.072094410988));
#20456=CARTESIAN_POINT('Ctrl Pts',(-56.0039967339745,-112.708046979118,
177.207792449865));
#20457=CARTESIAN_POINT('Ctrl Pts',(-55.9940587219143,-112.614825209041,
175.985484945604));
#20458=CARTESIAN_POINT('Ctrl Pts',(-55.9841207098542,-112.521603438964,
174.763177441344));
#20459=CARTESIAN_POINT('Ctrl Pts',(-56.8336146897208,-112.336760476773,
173.89887555255));
#20460=CARTESIAN_POINT('Ctrl Pts',(-57.6831086695875,-112.151917514582,
173.034573663757));
#20461=CARTESIAN_POINT('Ctrl Pts',(-58.8885910066563,-111.929123815193,
173.034573714903));
#20462=CARTESIAN_POINT('Ctrl Pts',(-60.0940733437252,-111.706330115804,
173.034573766048));
#20463=CARTESIAN_POINT('Ctrl Pts',(-60.9435672516694,-111.521487161281,
173.898875727171));
#20464=CARTESIAN_POINT('Ctrl Pts',(-61.7930611596136,-111.336644206758,
174.763177688294));
#20465=CARTESIAN_POINT('Ctrl Pts',(-61.7831230458397,-111.243422447524,
175.985485192554));
#20466=CARTESIAN_POINT('Ctrl Pts',(-61.7731849320658,-111.15020068829,177.207792696815));
#20467=CARTESIAN_POINT('Ctrl Pts',(-60.9038148263651,-111.14860012117,178.072094585608));
#20468=CARTESIAN_POINT('Ctrl Pts',(-60.0344447206644,-111.14699955405,178.936396474401));
#20469=CARTESIAN_POINT('Ctrl Pts',(-58.8090862577616,-111.183349724129,
178.936396423256));
#20470=CARTESIAN_POINT('Ctrl Pts',(-57.5837277948587,-111.219699894207,
178.936396372111));
#20471=CARTESIAN_POINT('Ctrl Pts',(-56.7143577610805,-111.21809931942,178.072094410988));
#20472=CARTESIAN_POINT('Ctrl Pts',(-55.8449877273022,-111.216498744632,
177.207792449865));
#20473=CARTESIAN_POINT('Ctrl Pts',(-55.8350497152421,-111.123276974555,
175.985484945604));
#20474=CARTESIAN_POINT('Ctrl Pts',(-55.8251117031819,-111.030055204478,
174.763177441344));
#20475=CARTESIAN_POINT('Ctrl Pts',(-56.6746056830486,-110.845212242287,
173.89887555255));
#20476=CARTESIAN_POINT('Ctrl Pts',(-57.5240996629153,-110.660369280097,
173.034573663757));
#20477=CARTESIAN_POINT('Ctrl Pts',(-58.7295819999841,-110.437575580708,
173.034573714903));
#20478=CARTESIAN_POINT('Ctrl Pts',(-59.9350643370529,-110.214781881319,
173.034573766048));
#20479=CARTESIAN_POINT('Ctrl Pts',(-60.7845582449971,-110.029938926795,
173.898875727171));
#20480=CARTESIAN_POINT('Ctrl Pts',(-61.6340521529414,-109.845095972272,
174.763177688294));
#20481=CARTESIAN_POINT('Ctrl Pts',(-61.6241140391675,-109.751874213038,
175.985485192554));
#20482=CARTESIAN_POINT('Ctrl Pts',(-61.6141759253936,-109.658652453805,
177.207792696815));
#20483=CARTESIAN_POINT('Ctrl Pts',(-60.7448058196929,-109.657051886685,
178.072094585608));
#20484=CARTESIAN_POINT('Ctrl Pts',(-59.8754357139922,-109.655451319565,
178.936396474401));
#20485=CARTESIAN_POINT('Ctrl Pts',(-58.6500772510893,-109.691801489643,
178.936396423256));
#20486=CARTESIAN_POINT('Ctrl Pts',(-57.4247187881865,-109.728151659721,
178.936396372111));
#20487=CARTESIAN_POINT('Ctrl Pts',(-56.5553487544082,-109.726551084934,
178.072094410988));
#20488=CARTESIAN_POINT('Ctrl Pts',(-55.68597872063,-109.724950510147,177.207792449865));
#20489=CARTESIAN_POINT('Ctrl Pts',(-55.6760407085698,-109.63172874007,175.985484945604));
#20490=CARTESIAN_POINT('Ctrl Pts',(-55.6661026965097,-109.538506969993,
174.763177441344));
#20491=CARTESIAN_POINT('Ctrl Pts',(-56.5155966763764,-109.353664007802,
173.89887555255));
#20492=CARTESIAN_POINT('Ctrl Pts',(-57.365090656243,-109.168821045611,173.034573663757));
#20493=CARTESIAN_POINT('Ctrl Pts',(-58.5705729933119,-108.946027346222,
173.034573714903));
#20494=CARTESIAN_POINT('Ctrl Pts',(-59.7760553303807,-108.723233646833,
173.034573766048));
#20495=CARTESIAN_POINT('Ctrl Pts',(-60.6255492383249,-108.53839069231,173.898875727171));
#20496=CARTESIAN_POINT('Ctrl Pts',(-61.4750431462691,-108.353547737786,
174.763177688294));
#20497=CARTESIAN_POINT('Ctrl Pts',(-61.4651050324952,-108.260325978553,
175.985485192554));
#20498=CARTESIAN_POINT('Ctrl Pts',(-61.4551669187214,-108.167104219319,
177.207792696815));
#20499=CARTESIAN_POINT('Ctrl Pts',(-60.5857968130207,-108.165503652199,
178.072094585608));
#20500=CARTESIAN_POINT('Ctrl Pts',(-59.71642670732,-108.163903085079,178.936396474401));
#20501=CARTESIAN_POINT('Ctrl Pts',(-58.4910682444171,-108.200253255158,
178.936396423256));
#20502=CARTESIAN_POINT('Ctrl Pts',(-57.2657097815143,-108.236603425236,
178.936396372111));
#20503=CARTESIAN_POINT('Ctrl Pts',(-56.396339747736,-108.235002850448,178.072094410988));
#20504=CARTESIAN_POINT('Ctrl Pts',(-55.5269697139578,-108.233402275661,
177.207792449865));
#20505=CARTESIAN_POINT('Ctrl Pts',(-55.5170317018976,-108.140180505584,
175.985484945604));
#20506=CARTESIAN_POINT('Ctrl Pts',(-55.5070936898375,-108.046958735507,
174.763177441344));
#20507=CARTESIAN_POINT('Ctrl Pts',(-56.3565876697041,-107.862115773316,
173.89887555255));
#20508=CARTESIAN_POINT('Ctrl Pts',(-57.2060816495708,-107.677272811126,
173.034573663757));
#20509=CARTESIAN_POINT('Ctrl Pts',(-58.4115639866396,-107.454479111736,
173.034573714903));
#20510=CARTESIAN_POINT('Ctrl Pts',(-59.6170463237085,-107.231685412347,
173.034573766048));
#20511=CARTESIAN_POINT('Ctrl Pts',(-60.4665402316527,-107.046842457824,
173.898875727171));
#20512=CARTESIAN_POINT('Ctrl Pts',(-61.3160341395969,-106.861999503301,
174.763177688294));
#20513=CARTESIAN_POINT('Ctrl Pts',(-61.306096025823,-106.768777744067,175.985485192554));
#20514=CARTESIAN_POINT('Ctrl Pts',(-61.2961579120492,-106.675555984834,
177.207792696815));
#20515=CARTESIAN_POINT('Ctrl Pts',(-60.4267878063484,-106.673955417714,
178.072094585608));
#20516=CARTESIAN_POINT('Ctrl Pts',(-59.5574177006478,-106.672354850594,
178.936396474401));
#20517=CARTESIAN_POINT('Ctrl Pts',(-58.3320592377449,-106.708705020672,
178.936396423256));
#20518=CARTESIAN_POINT('Ctrl Pts',(-57.106700774842,-106.74505519075,178.936396372111));
#20519=CARTESIAN_POINT('Ctrl Pts',(-56.2373307410638,-106.743454615963,
178.072094410988));
#20520=CARTESIAN_POINT('Ctrl Pts',(-55.3679607072856,-106.741854041175,
177.207792449865));
#20521=CARTESIAN_POINT('Ctrl Pts',(-55.3580226952254,-106.648632271098,
175.985484945604));
#20522=CARTESIAN_POINT('Ctrl Pts',(-55.3480846831652,-106.555410501021,
174.763177441344));
#20523=CARTESIAN_POINT('Ctrl Pts',(-56.1975786630319,-106.370567538831,
173.89887555255));
#20524=CARTESIAN_POINT('Ctrl Pts',(-57.0470726428986,-106.18572457664,173.034573663757));
#20525=CARTESIAN_POINT('Ctrl Pts',(-58.2525549799674,-105.962930877251,
173.034573714903));
#20526=CARTESIAN_POINT('Ctrl Pts',(-59.4580373170363,-105.740137177862,
173.034573766048));
#20527=CARTESIAN_POINT('Ctrl Pts',(-60.3075312249805,-105.555294223339,
173.898875727171));
#20528=CARTESIAN_POINT('Ctrl Pts',(-61.1570251329247,-105.370451268815,
174.763177688294));
#20529=CARTESIAN_POINT('Ctrl Pts',(-61.1470870191508,-105.277229509582,
175.985485192554));
#20530=CARTESIAN_POINT('Ctrl Pts',(-61.1371489053769,-105.184007750348,
177.207792696815));
#20531=CARTESIAN_POINT('Ctrl Pts',(-60.2677787996762,-105.182407183228,
178.072094585608));
#20532=CARTESIAN_POINT('Ctrl Pts',(-59.3984086939755,-105.180806616108,
178.936396474401));
#20533=CARTESIAN_POINT('Ctrl Pts',(-58.1730502310727,-105.217156786186,
178.936396423256));
#20534=CARTESIAN_POINT('Ctrl Pts',(-56.9476917681698,-105.253506956265,
178.936396372111));
#20535=CARTESIAN_POINT('Ctrl Pts',(-56.0783217343916,-105.251906381477,
178.072094410988));
#20536=CARTESIAN_POINT('Ctrl Pts',(-55.2089517006133,-105.25030580669,177.207792449865));
#20537=CARTESIAN_POINT('Ctrl Pts',(-55.1990136885532,-105.157084036613,
175.985484945604));
#20538=CARTESIAN_POINT('Ctrl Pts',(-55.189075676493,-105.063862266536,174.763177441344));
#20539=CARTESIAN_POINT('Ctrl Pts',(-56.0385696563597,-104.879019304345,
173.89887555255));
#20540=CARTESIAN_POINT('Ctrl Pts',(-56.8880636362264,-104.694176342154,
173.034573663757));
#20541=CARTESIAN_POINT('Ctrl Pts',(-58.0935459732952,-104.471382642765,
173.034573714903));
#20542=CARTESIAN_POINT('Ctrl Pts',(-59.299028310364,-104.248588943376,173.034573766048));
#20543=CARTESIAN_POINT('Ctrl Pts',(-60.1485222183082,-104.063745988853,
173.898875727171));
#20544=CARTESIAN_POINT('Ctrl Pts',(-60.9980161262524,-103.87890303433,174.763177688294));
#20545=CARTESIAN_POINT('Ctrl Pts',(-60.9880780124786,-103.785681275096,
175.985485192554));
#20546=CARTESIAN_POINT('Ctrl Pts',(-60.9781398987047,-103.692459515862,
177.207792696815));
#20547=CARTESIAN_POINT('Ctrl Pts',(-60.108769793004,-103.690858948742,178.072094585608));
#20548=CARTESIAN_POINT('Ctrl Pts',(-59.2393996873033,-103.689258381622,
178.936396474401));
#20549=CARTESIAN_POINT('Ctrl Pts',(-58.0140412244004,-103.725608551701,
178.936396423256));
#20550=CARTESIAN_POINT('Ctrl Pts',(-56.7886827614976,-103.761958721779,
178.936396372111));
#20551=CARTESIAN_POINT('Ctrl Pts',(-55.9193127277193,-103.760358146992,
178.072094410988));
#20552=CARTESIAN_POINT('Ctrl Pts',(-55.0499426939411,-103.758757572204,
177.207792449865));
#20553=CARTESIAN_POINT('Ctrl Pts',(-55.0400046818809,-103.665535802127,
175.985484945604));
#20554=CARTESIAN_POINT('Ctrl Pts',(-55.0300666698208,-103.57231403205,174.763177441344));
#20555=CARTESIAN_POINT('Ctrl Pts',(-55.8795606496874,-103.387471069859,
173.89887555255));
#20556=CARTESIAN_POINT('Ctrl Pts',(-56.7290546295541,-103.202628107669,
173.034573663757));
#20557=CARTESIAN_POINT('Ctrl Pts',(-57.934536966623,-102.97983440828,173.034573714903));
#20558=CARTESIAN_POINT('Ctrl Pts',(-59.1400193036918,-102.757040708891,
173.034573766048));
#20559=CARTESIAN_POINT('Ctrl Pts',(-59.989513211636,-102.572197754367,173.898875727171));
#20560=CARTESIAN_POINT('Ctrl Pts',(-60.8390071195802,-102.387354799844,
174.763177688294));
#20561=CARTESIAN_POINT('Ctrl Pts',(-60.8290690058063,-102.29413304061,175.985485192554));
#20562=CARTESIAN_POINT('Ctrl Pts',(-60.8191308920325,-102.200911281377,
177.207792696815));
#20563=CARTESIAN_POINT('Ctrl Pts',(-59.9497607863318,-102.199310714257,
178.072094585608));
#20564=CARTESIAN_POINT('Ctrl Pts',(-59.0803906806311,-102.197710147137,
178.936396474401));
#20565=CARTESIAN_POINT('Ctrl Pts',(-57.8550322177282,-102.234060317215,
178.936396423256));
#20566=CARTESIAN_POINT('Ctrl Pts',(-56.6296737548253,-102.270410487293,
178.936396372111));
#20567=CARTESIAN_POINT('Ctrl Pts',(-55.7603037210471,-102.268809912506,
178.072094410988));
#20568=CARTESIAN_POINT('Ctrl Pts',(-54.8909336872689,-102.267209337719,
177.207792449865));
#20569=CARTESIAN_POINT('Ctrl Pts',(-54.8809956752087,-102.173987567642,
175.985484945604));
#20570=CARTESIAN_POINT('Ctrl Pts',(-54.8710576631486,-102.080765797565,
174.763177441344));
#20571=CARTESIAN_POINT('Ctrl Pts',(-55.7205516430152,-101.895922835374,
173.89887555255));
#20572=CARTESIAN_POINT('Ctrl Pts',(-56.5700456228819,-101.711079873183,
173.034573663757));
#20573=CARTESIAN_POINT('Ctrl Pts',(-57.7755279599507,-101.488286173794,
173.034573714903));
#20574=CARTESIAN_POINT('Ctrl Pts',(-58.9810102970196,-101.265492474405,
173.034573766048));
#20575=CARTESIAN_POINT('Ctrl Pts',(-59.8305042049638,-101.080649519882,
173.898875727171));
#20576=CARTESIAN_POINT('Ctrl Pts',(-60.679998112908,-100.895806565358,174.763177688294));
#20577=CARTESIAN_POINT('Ctrl Pts',(-60.6700599991341,-100.802584806125,
175.985485192554));
#20578=CARTESIAN_POINT('Ctrl Pts',(-60.6601218853602,-100.709363046891,
177.207792696815));
#20579=CARTESIAN_POINT('Ctrl Pts',(-59.7907517796595,-100.707762479771,
178.072094585608));
#20580=CARTESIAN_POINT('Ctrl Pts',(-58.9213816739588,-100.706161912651,
178.936396474401));
#20581=CARTESIAN_POINT('Ctrl Pts',(-57.696023211056,-100.742512082729,178.936396423256));
#20582=CARTESIAN_POINT('Ctrl Pts',(-56.4706647481531,-100.778862252808,
178.936396372111));
#20583=CARTESIAN_POINT('Ctrl Pts',(-55.6012947143749,-100.77726167802,178.072094410988));
#20584=CARTESIAN_POINT('Ctrl Pts',(-54.7319246805966,-100.775661103233,
177.207792449865));
#20585=CARTESIAN_POINT('Ctrl Pts',(-54.7219866685365,-100.682439333156,
175.985484945604));
#20586=CARTESIAN_POINT('Ctrl Pts',(-54.7120486564763,-100.589217563079,
174.763177441344));
#20587=CARTESIAN_POINT('Ctrl Pts',(-55.561542636343,-100.404374600888,173.89887555255));
#20588=CARTESIAN_POINT('Ctrl Pts',(-56.4110366162097,-100.219531638698,
173.034573663757));
#20589=CARTESIAN_POINT('Ctrl Pts',(-57.6165189532785,-99.9967379393085,
173.034573714903));
#20590=CARTESIAN_POINT('Ctrl Pts',(-58.8220012903473,-99.7739442399195,
173.034573766048));
#20591=CARTESIAN_POINT('Ctrl Pts',(-59.6714951982915,-99.5891012853962,
173.898875727171));
#20592=CARTESIAN_POINT('Ctrl Pts',(-60.5209891062358,-99.4042583308729,
174.763177688294));
#20593=CARTESIAN_POINT('Ctrl Pts',(-60.5110509924619,-99.3110365716392,
175.985485192554));
#20594=CARTESIAN_POINT('Ctrl Pts',(-60.501112878688,-99.2178148124055,177.207792696815));
#20595=CARTESIAN_POINT('Ctrl Pts',(-59.6317427729873,-99.2162142452855,
178.072094585608));
#20596=CARTESIAN_POINT('Ctrl Pts',(-58.7623726672866,-99.2146136781656,
178.936396474401));
#20597=CARTESIAN_POINT('Ctrl Pts',(-57.5370142043838,-99.2509638482439,
178.936396423256));
#20598=CARTESIAN_POINT('Ctrl Pts',(-56.3116557414809,-99.2873140183222,
178.936396372111));
#20599=CARTESIAN_POINT('Ctrl Pts',(-55.4422857077027,-99.2857134435348,
178.072094410988));
#20600=CARTESIAN_POINT('Ctrl Pts',(-54.5729156739244,-99.2841128687474,
177.207792449865));
#20601=CARTESIAN_POINT('Ctrl Pts',(-54.5629776618643,-99.1908910986704,
175.985484945604));
#20602=CARTESIAN_POINT('Ctrl Pts',(-54.5530396498041,-99.0976693285933,
174.763177441344));
#20603=CARTESIAN_POINT('Ctrl Pts',(-55.4025336296708,-98.9128263664026,
173.89887555255));
#20604=CARTESIAN_POINT('Ctrl Pts',(-56.2520276095374,-98.727983404212,173.034573663757));
#20605=CARTESIAN_POINT('Ctrl Pts',(-57.4575099466063,-98.5051897048229,
173.034573714903));
#20606=CARTESIAN_POINT('Ctrl Pts',(-58.6629922836751,-98.2823960054338,
173.034573766048));
#20607=CARTESIAN_POINT('Ctrl Pts',(-59.5124861916193,-98.0975530509106,
173.898875727171));
#20608=CARTESIAN_POINT('Ctrl Pts',(-60.3619800995635,-97.9127100963873,
174.763177688294));
#20609=CARTESIAN_POINT('Ctrl Pts',(-60.3520419857897,-97.8194883371536,
175.985485192554));
#20610=CARTESIAN_POINT('Ctrl Pts',(-60.3421038720158,-97.7262665779199,
177.207792696815));
#20611=CARTESIAN_POINT('Ctrl Pts',(-59.4727337663151,-97.7246660108,178.072094585608));
#20612=CARTESIAN_POINT('Ctrl Pts',(-58.6033636606144,-97.72306544368,178.936396474401));
#20613=CARTESIAN_POINT('Ctrl Pts',(-57.3780051977115,-97.7594156137583,
178.936396423256));
#20614=CARTESIAN_POINT('Ctrl Pts',(-56.1526467348087,-97.7957657838366,
178.936396372111));
#20615=CARTESIAN_POINT('Ctrl Pts',(-55.2832767010304,-97.7941652090492,
178.072094410988));
#20616=CARTESIAN_POINT('Ctrl Pts',(-56.1707931031902,-113.117197303651,
178.813912075476));
#20617=CARTESIAN_POINT('Ctrl Pts',(-54.9958834532485,-113.148169293224,
177.6423391512));
#20618=CARTESIAN_POINT('Ctrl Pts',(-54.9859454592686,-113.05494752122,175.985484901707));
#20619=CARTESIAN_POINT('Ctrl Pts',(-54.9760074652888,-112.961725749215,
174.328630652215));
#20620=CARTESIAN_POINT('Ctrl Pts',(-56.1310410868884,-112.744310219938,
173.157057825983));
#20621=CARTESIAN_POINT('Ctrl Pts',(-57.286074708488,-112.52689469066,171.985484999752));
#20622=CARTESIAN_POINT('Ctrl Pts',(-58.9236553326579,-112.258036427063,
171.985485069079));
#20623=CARTESIAN_POINT('Ctrl Pts',(-60.5612359568277,-111.989178163466,
171.985485138407));
#20624=CARTESIAN_POINT('Ctrl Pts',(-61.7162694809355,-111.771762644582,
173.157058062683));
#20625=CARTESIAN_POINT('Ctrl Pts',(-62.8713030050432,-111.554347125698,
174.328630986959));
#20626=CARTESIAN_POINT('Ctrl Pts',(-62.861364873189,-111.461125368392,175.985485236451));
#20627=CARTESIAN_POINT('Ctrl Pts',(-62.8514267413349,-111.367903611086,
177.642339485944));
#20628=CARTESIAN_POINT('Ctrl Pts',(-61.6765169939012,-111.398875611052,
178.813912312176));
#20629=CARTESIAN_POINT('Ctrl Pts',(-60.5016072464676,-111.429847611019,
179.985485138407));
#20630=CARTESIAN_POINT('Ctrl Pts',(-58.8441504964637,-111.512262345305,
179.985485069079));
#20631=CARTESIAN_POINT('Ctrl Pts',(-57.1866937464598,-111.594677079592,
179.985484999752));
#20632=CARTESIAN_POINT('Ctrl Pts',(-56.011784096518,-111.625649069165,178.813912075476));
#20633=CARTESIAN_POINT('Ctrl Pts',(-54.8368744465762,-111.656621058739,
177.6423391512));
#20634=CARTESIAN_POINT('Ctrl Pts',(-54.8269364525964,-111.563399286734,
175.985484901707));
#20635=CARTESIAN_POINT('Ctrl Pts',(-54.8169984586165,-111.47017751473,174.328630652215));
#20636=CARTESIAN_POINT('Ctrl Pts',(-55.9720320802161,-111.252761985452,
173.157057825983));
#20637=CARTESIAN_POINT('Ctrl Pts',(-57.1270657018158,-111.035346456175,
171.985484999752));
#20638=CARTESIAN_POINT('Ctrl Pts',(-58.7646463259856,-110.766488192578,
171.985485069079));
#20639=CARTESIAN_POINT('Ctrl Pts',(-60.4022269501555,-110.497629928981,
171.985485138407));
#20640=CARTESIAN_POINT('Ctrl Pts',(-61.5572604742632,-110.280214410097,
173.157058062683));
#20641=CARTESIAN_POINT('Ctrl Pts',(-62.712293998371,-110.062798891212,174.328630986959));
#20642=CARTESIAN_POINT('Ctrl Pts',(-62.7023558665168,-109.969577133906,
175.985485236451));
#20643=CARTESIAN_POINT('Ctrl Pts',(-62.6924177346626,-109.8763553766,177.642339485944));
#20644=CARTESIAN_POINT('Ctrl Pts',(-61.517507987229,-109.907327376567,178.813912312176));
#20645=CARTESIAN_POINT('Ctrl Pts',(-60.3425982397954,-109.938299376534,
179.985485138407));
#20646=CARTESIAN_POINT('Ctrl Pts',(-58.6851414897915,-110.02071411082,179.985485069079));
#20647=CARTESIAN_POINT('Ctrl Pts',(-57.0276847397876,-110.103128845106,
179.985484999752));
#20648=CARTESIAN_POINT('Ctrl Pts',(-55.8527750898458,-110.13410083468,178.813912075476));
#20649=CARTESIAN_POINT('Ctrl Pts',(-54.677865439904,-110.165072824253,177.6423391512));
#20650=CARTESIAN_POINT('Ctrl Pts',(-54.6679274459242,-110.071851052249,
175.985484901707));
#20651=CARTESIAN_POINT('Ctrl Pts',(-54.6579894519443,-109.978629280244,
174.328630652215));
#20652=CARTESIAN_POINT('Ctrl Pts',(-55.8130230735439,-109.761213750967,
173.157057825983));
#20653=CARTESIAN_POINT('Ctrl Pts',(-56.9680566951435,-109.543798221689,
171.985484999752));
#20654=CARTESIAN_POINT('Ctrl Pts',(-58.6056373193134,-109.274939958092,
171.985485069079));
#20655=CARTESIAN_POINT('Ctrl Pts',(-60.2432179434833,-109.006081694495,
171.985485138407));
#20656=CARTESIAN_POINT('Ctrl Pts',(-61.398251467591,-108.788666175611,173.157058062683));
#20657=CARTESIAN_POINT('Ctrl Pts',(-62.5532849916988,-108.571250656727,
174.328630986959));
#20658=CARTESIAN_POINT('Ctrl Pts',(-62.5433468598446,-108.478028899421,
175.985485236451));
#20659=CARTESIAN_POINT('Ctrl Pts',(-62.5334087279904,-108.384807142114,
177.642339485944));
#20660=CARTESIAN_POINT('Ctrl Pts',(-61.3584989805568,-108.415779142081,
178.813912312176));
#20661=CARTESIAN_POINT('Ctrl Pts',(-60.1835892331231,-108.446751142048,
179.985485138407));
#20662=CARTESIAN_POINT('Ctrl Pts',(-58.5261324831192,-108.529165876334,
179.985485069079));
#20663=CARTESIAN_POINT('Ctrl Pts',(-56.8686757331153,-108.611580610621,
179.985484999752));
#20664=CARTESIAN_POINT('Ctrl Pts',(-55.6937660831736,-108.642552600194,
178.813912075476));
#20665=CARTESIAN_POINT('Ctrl Pts',(-54.5188564332318,-108.673524589768,
177.6423391512));
#20666=CARTESIAN_POINT('Ctrl Pts',(-54.5089184392519,-108.580302817763,
175.985484901707));
#20667=CARTESIAN_POINT('Ctrl Pts',(-54.4989804452721,-108.487081045759,
174.328630652215));
#20668=CARTESIAN_POINT('Ctrl Pts',(-55.6540140668717,-108.269665516481,
173.157057825983));
#20669=CARTESIAN_POINT('Ctrl Pts',(-56.8090476884713,-108.052249987204,
171.985484999752));
#20670=CARTESIAN_POINT('Ctrl Pts',(-58.4466283126412,-107.783391723607,
171.985485069079));
#20671=CARTESIAN_POINT('Ctrl Pts',(-60.084208936811,-107.51453346001,171.985485138407));
#20672=CARTESIAN_POINT('Ctrl Pts',(-61.2392424609188,-107.297117941125,
173.157058062683));
#20673=CARTESIAN_POINT('Ctrl Pts',(-62.3942759850265,-107.079702422241,
174.328630986959));
#20674=CARTESIAN_POINT('Ctrl Pts',(-62.3843378531723,-106.986480664935,
175.985485236451));
#20675=CARTESIAN_POINT('Ctrl Pts',(-62.3743997213182,-106.893258907629,
177.642339485944));
#20676=CARTESIAN_POINT('Ctrl Pts',(-61.1994899738845,-106.924230907596,
178.813912312176));
#20677=CARTESIAN_POINT('Ctrl Pts',(-60.0245802264509,-106.955202907562,
179.985485138407));
#20678=CARTESIAN_POINT('Ctrl Pts',(-58.367123476447,-107.037617641849,179.985485069079));
#20679=CARTESIAN_POINT('Ctrl Pts',(-56.7096667264431,-107.120032376135,
179.985484999752));
#20680=CARTESIAN_POINT('Ctrl Pts',(-55.5347570765013,-107.151004365708,
178.813912075476));
#20681=CARTESIAN_POINT('Ctrl Pts',(-54.3598474265596,-107.181976355282,
177.6423391512));
#20682=CARTESIAN_POINT('Ctrl Pts',(-54.3499094325797,-107.088754583277,
175.985484901707));
#20683=CARTESIAN_POINT('Ctrl Pts',(-54.3399714385998,-106.995532811273,
174.328630652215));
#20684=CARTESIAN_POINT('Ctrl Pts',(-55.4950050601995,-106.778117281995,
173.157057825983));
#20685=CARTESIAN_POINT('Ctrl Pts',(-56.6500386817991,-106.560701752718,
171.985484999752));
#20686=CARTESIAN_POINT('Ctrl Pts',(-58.2876193059689,-106.291843489121,
171.985485069079));
#20687=CARTESIAN_POINT('Ctrl Pts',(-59.9251999301388,-106.022985225524,
171.985485138407));
#20688=CARTESIAN_POINT('Ctrl Pts',(-61.0802334542465,-105.80556970664,173.157058062683));
#20689=CARTESIAN_POINT('Ctrl Pts',(-62.2352669783543,-105.588154187756,
174.328630986959));
#20690=CARTESIAN_POINT('Ctrl Pts',(-62.2253288465001,-105.494932430449,
175.985485236451));
#20691=CARTESIAN_POINT('Ctrl Pts',(-62.2153907146459,-105.401710673143,
177.642339485944));
#20692=CARTESIAN_POINT('Ctrl Pts',(-61.0404809672123,-105.43268267311,178.813912312176));
#20693=CARTESIAN_POINT('Ctrl Pts',(-59.8655712197787,-105.463654673077,
179.985485138407));
#20694=CARTESIAN_POINT('Ctrl Pts',(-58.2081144697748,-105.546069407363,
179.985485069079));
#20695=CARTESIAN_POINT('Ctrl Pts',(-56.5506577197709,-105.628484141649,
179.985484999752));
#20696=CARTESIAN_POINT('Ctrl Pts',(-55.3757480698291,-105.659456131223,
178.813912075476));
#20697=CARTESIAN_POINT('Ctrl Pts',(-54.2008384198873,-105.690428120796,
177.6423391512));
#20698=CARTESIAN_POINT('Ctrl Pts',(-54.1909004259075,-105.597206348792,
175.985484901707));
#20699=CARTESIAN_POINT('Ctrl Pts',(-54.1809624319276,-105.503984576787,
174.328630652215));
#20700=CARTESIAN_POINT('Ctrl Pts',(-55.3359960535272,-105.28656904751,173.157057825983));
#20701=CARTESIAN_POINT('Ctrl Pts',(-56.4910296751268,-105.069153518232,
171.985484999752));
#20702=CARTESIAN_POINT('Ctrl Pts',(-58.1286102992967,-104.800295254635,
171.985485069079));
#20703=CARTESIAN_POINT('Ctrl Pts',(-59.7661909234666,-104.531436991038,
171.985485138407));
#20704=CARTESIAN_POINT('Ctrl Pts',(-60.9212244475743,-104.314021472154,
173.157058062683));
#20705=CARTESIAN_POINT('Ctrl Pts',(-62.0762579716821,-104.09660595327,174.328630986959));
#20706=CARTESIAN_POINT('Ctrl Pts',(-62.0663198398279,-104.003384195964,
175.985485236451));
#20707=CARTESIAN_POINT('Ctrl Pts',(-62.0563817079737,-103.910162438658,
177.642339485944));
#20708=CARTESIAN_POINT('Ctrl Pts',(-60.8814719605401,-103.941134438624,
178.813912312176));
#20709=CARTESIAN_POINT('Ctrl Pts',(-59.7065622131064,-103.972106438591,
179.985485138407));
#20710=CARTESIAN_POINT('Ctrl Pts',(-58.0491054631025,-104.054521172878,
179.985485069079));
#20711=CARTESIAN_POINT('Ctrl Pts',(-56.3916487130987,-104.136935907164,
179.985484999752));
#20712=CARTESIAN_POINT('Ctrl Pts',(-55.2167390631569,-104.167907896737,
178.813912075476));
#20713=CARTESIAN_POINT('Ctrl Pts',(-54.0418294132151,-104.198879886311,
177.6423391512));
#20714=CARTESIAN_POINT('Ctrl Pts',(-54.0318914192353,-104.105658114306,
175.985484901707));
#20715=CARTESIAN_POINT('Ctrl Pts',(-54.0219534252554,-104.012436342302,
174.328630652215));
#20716=CARTESIAN_POINT('Ctrl Pts',(-55.176987046855,-103.795020813024,173.157057825983));
#20717=CARTESIAN_POINT('Ctrl Pts',(-56.3320206684546,-103.577605283747,
171.985484999752));
#20718=CARTESIAN_POINT('Ctrl Pts',(-57.9696012926245,-103.30874702015,171.985485069079));
#20719=CARTESIAN_POINT('Ctrl Pts',(-59.6071819167943,-103.039888756553,
171.985485138407));
#20720=CARTESIAN_POINT('Ctrl Pts',(-60.7622154409021,-102.822473237669,
173.157058062683));
#20721=CARTESIAN_POINT('Ctrl Pts',(-61.9172489650099,-102.605057718784,
174.328630986959));
#20722=CARTESIAN_POINT('Ctrl Pts',(-61.9073108331557,-102.511835961478,
175.985485236451));
#20723=CARTESIAN_POINT('Ctrl Pts',(-61.8973727013015,-102.418614204172,
177.642339485944));
#20724=CARTESIAN_POINT('Ctrl Pts',(-60.7224629538678,-102.449586204139,
178.813912312176));
#20725=CARTESIAN_POINT('Ctrl Pts',(-59.5475532064342,-102.480558204106,
179.985485138407));
#20726=CARTESIAN_POINT('Ctrl Pts',(-57.8900964564303,-102.562972938392,
179.985485069079));
#20727=CARTESIAN_POINT('Ctrl Pts',(-56.2326397064264,-102.645387672678,
179.985484999752));
#20728=CARTESIAN_POINT('Ctrl Pts',(-55.0577300564847,-102.676359662252,
178.813912075476));
#20729=CARTESIAN_POINT('Ctrl Pts',(-53.8828204065429,-102.707331651825,
177.6423391512));
#20730=CARTESIAN_POINT('Ctrl Pts',(-53.872882412563,-102.614109879821,175.985484901707));
#20731=CARTESIAN_POINT('Ctrl Pts',(-53.8629444185832,-102.520888107816,
174.328630652215));
#20732=CARTESIAN_POINT('Ctrl Pts',(-55.0179780401828,-102.303472578539,
173.157057825983));
#20733=CARTESIAN_POINT('Ctrl Pts',(-56.1730116617824,-102.086057049261,
171.985484999752));
#20734=CARTESIAN_POINT('Ctrl Pts',(-57.8105922859523,-101.817198785664,
171.985485069079));
#20735=CARTESIAN_POINT('Ctrl Pts',(-59.4481729101221,-101.548340522067,
171.985485138407));
#20736=CARTESIAN_POINT('Ctrl Pts',(-60.6032064342299,-101.330925003183,
173.157058062683));
#20737=CARTESIAN_POINT('Ctrl Pts',(-61.7582399583376,-101.113509484299,
174.328630986959));
#20738=CARTESIAN_POINT('Ctrl Pts',(-61.7483018264834,-101.020287726993,
175.985485236451));
#20739=CARTESIAN_POINT('Ctrl Pts',(-61.7383636946293,-100.927065969686,
177.642339485944));
#20740=CARTESIAN_POINT('Ctrl Pts',(-60.5634539471956,-100.958037969653,
178.813912312176));
#20741=CARTESIAN_POINT('Ctrl Pts',(-59.388544199762,-100.98900996962,179.985485138407));
#20742=CARTESIAN_POINT('Ctrl Pts',(-57.7310874497581,-101.071424703906,
179.985485069079));
#20743=CARTESIAN_POINT('Ctrl Pts',(-56.0736306997542,-101.153839438193,
179.985484999752));
#20744=CARTESIAN_POINT('Ctrl Pts',(-54.8987210498124,-101.184811427766,
178.813912075476));
#20745=CARTESIAN_POINT('Ctrl Pts',(-53.7238113998707,-101.21578341734,177.6423391512));
#20746=CARTESIAN_POINT('Ctrl Pts',(-53.7138734058908,-101.122561645335,
175.985484901707));
#20747=CARTESIAN_POINT('Ctrl Pts',(-53.7039354119109,-101.029339873331,
174.328630652215));
#20748=CARTESIAN_POINT('Ctrl Pts',(-54.8589690335105,-100.811924344053,
173.157057825983));
#20749=CARTESIAN_POINT('Ctrl Pts',(-56.0140026551102,-100.594508814776,
171.985484999752));
#20750=CARTESIAN_POINT('Ctrl Pts',(-57.65158327928,-100.325650551179,171.985485069079));
#20751=CARTESIAN_POINT('Ctrl Pts',(-59.2891639034499,-100.056792287582,
171.985485138407));
#20752=CARTESIAN_POINT('Ctrl Pts',(-60.4441974275576,-99.8393767686974,
173.157058062683));
#20753=CARTESIAN_POINT('Ctrl Pts',(-61.5992309516654,-99.6219612498133,
174.328630986959));
#20754=CARTESIAN_POINT('Ctrl Pts',(-61.5892928198112,-99.528739492507,175.985485236451));
#20755=CARTESIAN_POINT('Ctrl Pts',(-61.579354687957,-99.4355177352008,177.642339485944));
#20756=CARTESIAN_POINT('Ctrl Pts',(-60.4044449405234,-99.4664897351676,
178.813912312176));
#20757=CARTESIAN_POINT('Ctrl Pts',(-59.2295351930898,-99.4974617351344,
179.985485138407));
#20758=CARTESIAN_POINT('Ctrl Pts',(-57.5720784430859,-99.5798764694207,
179.985485069079));
#20759=CARTESIAN_POINT('Ctrl Pts',(-55.914621693082,-99.662291203707,179.985484999752));
#20760=CARTESIAN_POINT('Ctrl Pts',(-54.7397120431402,-99.6932631932805,
178.813912075476));
#20761=CARTESIAN_POINT('Ctrl Pts',(-53.5648023931984,-99.724235182854,177.6423391512));
#20762=CARTESIAN_POINT('Ctrl Pts',(-53.5548643992186,-99.6310134108495,
175.985484901707));
#20763=CARTESIAN_POINT('Ctrl Pts',(-53.5449264052387,-99.5377916388449,
174.328630652215));
#20764=CARTESIAN_POINT('Ctrl Pts',(-54.6999600268383,-99.3203761095675,
173.157057825983));
#20765=CARTESIAN_POINT('Ctrl Pts',(-55.8549936484379,-99.10296058029,171.985484999752));
#20766=CARTESIAN_POINT('Ctrl Pts',(-57.4925742726078,-98.834102316693,171.985485069079));
#20767=CARTESIAN_POINT('Ctrl Pts',(-59.1301548967777,-98.565244053096,171.985485138407));
#20768=CARTESIAN_POINT('Ctrl Pts',(-60.2851884208854,-98.3478285342118,
173.157058062683));
#20769=CARTESIAN_POINT('Ctrl Pts',(-61.4402219449932,-98.1304130153276,
174.328630986959));
#20770=CARTESIAN_POINT('Ctrl Pts',(-61.430283813139,-98.0371912580215,175.985485236451));
#20771=CARTESIAN_POINT('Ctrl Pts',(-61.4203456812848,-97.9439695007152,
177.642339485944));
#20772=CARTESIAN_POINT('Ctrl Pts',(-60.2454359338512,-97.974941500682,178.813912312176));
#20773=CARTESIAN_POINT('Ctrl Pts',(-59.0705261864175,-98.0059135006488,
179.985485138407));
#20774=CARTESIAN_POINT('Ctrl Pts',(-57.4130694364136,-98.0883282349351,
179.985485069079));
#20775=CARTESIAN_POINT('Ctrl Pts',(-55.7556126864097,-98.1707429692214,
179.985484999752));
#20776=CARTESIAN_POINT('Ctrl Pts',(-54.580703036468,-98.2017149587949,178.813912075476));
#20777=CARTESIAN_POINT('Ctrl Pts',(-61.0175785779007,-102.443745017979,
178.485485069079));
#20778=CARTESIAN_POINT('Ctrl Pts',(-60.879006373544,-102.445459535857,178.657813499464));
#20779=CARTESIAN_POINT('Ctrl Pts',(-60.7224629538678,-102.449586204139,
178.813912312176));
#20780=CARTESIAN_POINT('Ctrl Pts',(-59.5475532064342,-102.480558204106,
179.985485138407));
#20781=CARTESIAN_POINT('Ctrl Pts',(-57.8900964564303,-102.562972938392,
179.985485069079));
#20782=CARTESIAN_POINT('Ctrl Pts',(-56.2326397064264,-102.645387672678,
179.985484999752));
#20783=CARTESIAN_POINT('Ctrl Pts',(-55.0577300564847,-102.676359662252,
178.813912075476));
#20784=CARTESIAN_POINT('Ctrl Pts',(-53.8828204798772,-102.707331649892,
177.642339224326));
#20785=CARTESIAN_POINT('Ctrl Pts',(-53.8728824136219,-102.614109889754,
175.985485078249));
#20786=CARTESIAN_POINT('Ctrl Pts',(-56.1707931031902,-113.117197303651,
178.813912075476));
#20787=CARTESIAN_POINT('Ctrl Pts',(-54.9958834532485,-113.148169293224,
177.6423391512));
#20788=CARTESIAN_POINT('Ctrl Pts',(-54.9859454592686,-113.05494752122,175.985484901707));
#20789=CARTESIAN_POINT('Ctrl Pts',(-54.9760074652888,-112.961725749215,
174.328630652215));
#20790=CARTESIAN_POINT('Ctrl Pts',(-56.1310410868884,-112.744310219938,
173.157057825983));
#20791=CARTESIAN_POINT('Ctrl Pts',(-57.286074708488,-112.52689469066,171.985484999752));
#20792=CARTESIAN_POINT('Ctrl Pts',(-58.9236553326578,-112.258036427063,
171.985485069079));
#20793=CARTESIAN_POINT('Ctrl Pts',(-60.5612359568277,-111.989178163466,
171.985485138407));
#20794=CARTESIAN_POINT('Ctrl Pts',(-61.7162694809355,-111.771762644582,
173.157058062683));
#20795=CARTESIAN_POINT('Ctrl Pts',(-62.8713030050432,-111.554347125698,
174.328630986959));
#20796=CARTESIAN_POINT('Ctrl Pts',(-62.861364873189,-111.461125368392,175.985485236451));
#20797=CARTESIAN_POINT('Ctrl Pts',(-62.8514267413349,-111.367903611086,
177.642339485944));
#20798=CARTESIAN_POINT('Ctrl Pts',(-61.6765169939012,-111.398875611052,
178.813912312176));
#20799=CARTESIAN_POINT('Ctrl Pts',(-60.5016072464676,-111.429847611019,
179.985485138407));
#20800=CARTESIAN_POINT('Ctrl Pts',(-58.8441504964637,-111.512262345305,
179.985485069079));
#20801=CARTESIAN_POINT('Ctrl Pts',(-57.1866937464598,-111.594677079592,
179.985484999752));
#20802=CARTESIAN_POINT('Ctrl Pts',(-56.011784096518,-111.625649069165,178.813912075476));
#20803=CARTESIAN_POINT('Ctrl Pts',(-54.8368744465763,-111.656621058739,
177.6423391512));
#20804=CARTESIAN_POINT('Ctrl Pts',(-54.8269364525964,-111.563399286734,
175.985484901707));
#20805=CARTESIAN_POINT('Ctrl Pts',(-54.8169984586165,-111.47017751473,174.328630652215));
#20806=CARTESIAN_POINT('Ctrl Pts',(-55.9720320802161,-111.252761985452,
173.157057825983));
#20807=CARTESIAN_POINT('Ctrl Pts',(-57.1270657018158,-111.035346456175,
171.985484999752));
#20808=CARTESIAN_POINT('Ctrl Pts',(-58.7646463259856,-110.766488192578,
171.985485069079));
#20809=CARTESIAN_POINT('Ctrl Pts',(-60.4022269501555,-110.497629928981,
171.985485138407));
#20810=CARTESIAN_POINT('Ctrl Pts',(-61.5572604742632,-110.280214410097,
173.157058062683));
#20811=CARTESIAN_POINT('Ctrl Pts',(-62.712293998371,-110.062798891212,174.328630986959));
#20812=CARTESIAN_POINT('Ctrl Pts',(-62.7023558665168,-109.969577133906,
175.985485236451));
#20813=CARTESIAN_POINT('Ctrl Pts',(-62.6924177346626,-109.8763553766,177.642339485944));
#20814=CARTESIAN_POINT('Ctrl Pts',(-61.517507987229,-109.907327376567,178.813912312176));
#20815=CARTESIAN_POINT('Ctrl Pts',(-60.3425982397954,-109.938299376534,
179.985485138407));
#20816=CARTESIAN_POINT('Ctrl Pts',(-58.6851414897915,-110.02071411082,179.985485069079));
#20817=CARTESIAN_POINT('Ctrl Pts',(-57.0276847397876,-110.103128845106,
179.985484999752));
#20818=CARTESIAN_POINT('Ctrl Pts',(-55.8527750898458,-110.13410083468,178.813912075476));
#20819=CARTESIAN_POINT('Ctrl Pts',(-54.677865439904,-110.165072824253,177.6423391512));
#20820=CARTESIAN_POINT('Ctrl Pts',(-54.6679274459242,-110.071851052249,
175.985484901707));
#20821=CARTESIAN_POINT('Ctrl Pts',(-54.6579894519443,-109.978629280244,
174.328630652215));
#20822=CARTESIAN_POINT('Ctrl Pts',(-55.8130230735439,-109.761213750967,
173.157057825983));
#20823=CARTESIAN_POINT('Ctrl Pts',(-56.9680566951435,-109.543798221689,
171.985484999752));
#20824=CARTESIAN_POINT('Ctrl Pts',(-58.6056373193134,-109.274939958092,
171.985485069079));
#20825=CARTESIAN_POINT('Ctrl Pts',(-60.2432179434833,-109.006081694495,
171.985485138407));
#20826=CARTESIAN_POINT('Ctrl Pts',(-61.398251467591,-108.788666175611,173.157058062683));
#20827=CARTESIAN_POINT('Ctrl Pts',(-62.5532849916988,-108.571250656727,
174.328630986959));
#20828=CARTESIAN_POINT('Ctrl Pts',(-62.5433468598446,-108.478028899421,
175.985485236451));
#20829=CARTESIAN_POINT('Ctrl Pts',(-62.5334087279904,-108.384807142114,
177.642339485944));
#20830=CARTESIAN_POINT('Ctrl Pts',(-61.3584989805568,-108.415779142081,
178.813912312176));
#20831=CARTESIAN_POINT('Ctrl Pts',(-60.1835892331231,-108.446751142048,
179.985485138407));
#20832=CARTESIAN_POINT('Ctrl Pts',(-58.5261324831192,-108.529165876334,
179.985485069079));
#20833=CARTESIAN_POINT('Ctrl Pts',(-56.8686757331153,-108.611580610621,
179.985484999752));
#20834=CARTESIAN_POINT('Ctrl Pts',(-55.6937660831736,-108.642552600194,
178.813912075476));
#20835=CARTESIAN_POINT('Ctrl Pts',(-54.5188564332318,-108.673524589768,
177.6423391512));
#20836=CARTESIAN_POINT('Ctrl Pts',(-54.5089184392519,-108.580302817763,
175.985484901707));
#20837=CARTESIAN_POINT('Ctrl Pts',(-54.4989804452721,-108.487081045759,
174.328630652215));
#20838=CARTESIAN_POINT('Ctrl Pts',(-55.6540140668717,-108.269665516481,
173.157057825983));
#20839=CARTESIAN_POINT('Ctrl Pts',(-56.8090476884713,-108.052249987204,
171.985484999752));
#20840=CARTESIAN_POINT('Ctrl Pts',(-58.4466283126412,-107.783391723607,
171.985485069079));
#20841=CARTESIAN_POINT('Ctrl Pts',(-60.084208936811,-107.51453346001,171.985485138407));
#20842=CARTESIAN_POINT('Ctrl Pts',(-61.2392424609188,-107.297117941125,
173.157058062683));
#20843=CARTESIAN_POINT('Ctrl Pts',(-62.3942759850265,-107.079702422241,
174.328630986959));
#20844=CARTESIAN_POINT('Ctrl Pts',(-62.3843378531723,-106.986480664935,
175.985485236451));
#20845=CARTESIAN_POINT('Ctrl Pts',(-62.3743997213182,-106.893258907629,
177.642339485944));
#20846=CARTESIAN_POINT('Ctrl Pts',(-61.1994899738845,-106.924230907596,
178.813912312176));
#20847=CARTESIAN_POINT('Ctrl Pts',(-60.0245802264509,-106.955202907562,
179.985485138407));
#20848=CARTESIAN_POINT('Ctrl Pts',(-58.367123476447,-107.037617641849,179.985485069079));
#20849=CARTESIAN_POINT('Ctrl Pts',(-56.7096667264431,-107.120032376135,
179.985484999752));
#20850=CARTESIAN_POINT('Ctrl Pts',(-55.5347570765013,-107.151004365708,
178.813912075476));
#20851=CARTESIAN_POINT('Ctrl Pts',(-54.3598474265596,-107.181976355282,
177.6423391512));
#20852=CARTESIAN_POINT('Ctrl Pts',(-54.3499094325797,-107.088754583277,
175.985484901707));
#20853=CARTESIAN_POINT('Ctrl Pts',(-54.3399714385998,-106.995532811273,
174.328630652215));
#20854=CARTESIAN_POINT('Ctrl Pts',(-55.4950050601995,-106.778117281995,
173.157057825983));
#20855=CARTESIAN_POINT('Ctrl Pts',(-56.6500386817991,-106.560701752718,
171.985484999752));
#20856=CARTESIAN_POINT('Ctrl Pts',(-58.2876193059689,-106.291843489121,
171.985485069079));
#20857=CARTESIAN_POINT('Ctrl Pts',(-59.9251999301388,-106.022985225524,
171.985485138407));
#20858=CARTESIAN_POINT('Ctrl Pts',(-61.0802334542465,-105.80556970664,173.157058062683));
#20859=CARTESIAN_POINT('Ctrl Pts',(-62.2352669783543,-105.588154187756,
174.328630986959));
#20860=CARTESIAN_POINT('Ctrl Pts',(-62.2253288465001,-105.494932430449,
175.985485236451));
#20861=CARTESIAN_POINT('Ctrl Pts',(-62.2153907146459,-105.401710673143,
177.642339485944));
#20862=CARTESIAN_POINT('Ctrl Pts',(-61.0404809672123,-105.43268267311,178.813912312176));
#20863=CARTESIAN_POINT('Ctrl Pts',(-59.8655712197787,-105.463654673077,
179.985485138407));
#20864=CARTESIAN_POINT('Ctrl Pts',(-58.2081144697748,-105.546069407363,
179.985485069079));
#20865=CARTESIAN_POINT('Ctrl Pts',(-56.5506577197709,-105.628484141649,
179.985484999752));
#20866=CARTESIAN_POINT('Ctrl Pts',(-55.3757480698291,-105.659456131223,
178.813912075476));
#20867=CARTESIAN_POINT('Ctrl Pts',(-54.2008384198873,-105.690428120796,
177.6423391512));
#20868=CARTESIAN_POINT('Ctrl Pts',(-54.1909004259075,-105.597206348792,
175.985484901707));
#20869=CARTESIAN_POINT('Ctrl Pts',(-54.1809624319276,-105.503984576787,
174.328630652215));
#20870=CARTESIAN_POINT('Ctrl Pts',(-55.3359960535272,-105.28656904751,173.157057825983));
#20871=CARTESIAN_POINT('Ctrl Pts',(-56.4910296751268,-105.069153518232,
171.985484999752));
#20872=CARTESIAN_POINT('Ctrl Pts',(-58.1286102992967,-104.800295254635,
171.985485069079));
#20873=CARTESIAN_POINT('Ctrl Pts',(-59.7661909234666,-104.531436991038,
171.985485138407));
#20874=CARTESIAN_POINT('Ctrl Pts',(-60.9212244475743,-104.314021472154,
173.157058062683));
#20875=CARTESIAN_POINT('Ctrl Pts',(-62.0762579716821,-104.09660595327,174.328630986959));
#20876=CARTESIAN_POINT('Ctrl Pts',(-62.0663198398279,-104.003384195964,
175.985485236451));
#20877=CARTESIAN_POINT('Ctrl Pts',(-62.0563817079737,-103.910162438658,
177.642339485944));
#20878=CARTESIAN_POINT('Ctrl Pts',(-60.8814719605401,-103.941134438624,
178.813912312176));
#20879=CARTESIAN_POINT('Ctrl Pts',(-59.7065622131064,-103.972106438591,
179.985485138407));
#20880=CARTESIAN_POINT('Ctrl Pts',(-58.0491054631025,-104.054521172878,
179.985485069079));
#20881=CARTESIAN_POINT('Ctrl Pts',(-56.3916487130987,-104.136935907164,
179.985484999752));
#20882=CARTESIAN_POINT('Ctrl Pts',(-55.2167390631569,-104.167907896737,
178.813912075476));
#20883=CARTESIAN_POINT('Ctrl Pts',(-54.0418294132151,-104.198879886311,
177.6423391512));
#20884=CARTESIAN_POINT('Ctrl Pts',(-54.0318914192353,-104.105658114306,
175.985484901707));
#20885=CARTESIAN_POINT('Ctrl Pts',(-54.0219534252554,-104.012436342302,
174.328630652215));
#20886=CARTESIAN_POINT('Ctrl Pts',(-55.176987046855,-103.795020813024,173.157057825983));
#20887=CARTESIAN_POINT('Ctrl Pts',(-56.3320206684546,-103.577605283747,
171.985484999752));
#20888=CARTESIAN_POINT('Ctrl Pts',(-57.9696012926245,-103.30874702015,171.985485069079));
#20889=CARTESIAN_POINT('Ctrl Pts',(-59.6071819167943,-103.039888756553,
171.985485138407));
#20890=CARTESIAN_POINT('Ctrl Pts',(-60.7622154409021,-102.822473237669,
173.157058062683));
#20891=CARTESIAN_POINT('Ctrl Pts',(-61.9172489650099,-102.605057718784,
174.328630986959));
#20892=CARTESIAN_POINT('Ctrl Pts',(-61.9073108331557,-102.511835961478,
175.985485236451));
#20893=CARTESIAN_POINT('Ctrl Pts',(-61.8973727013015,-102.418614204172,
177.642339485944));
#20894=CARTESIAN_POINT('Ctrl Pts',(-60.7224629538678,-102.449586204139,
178.813912312176));
#20895=CARTESIAN_POINT('Ctrl Pts',(-59.5475532064342,-102.480558204106,
179.985485138407));
#20896=CARTESIAN_POINT('Ctrl Pts',(-57.8900964564303,-102.562972938392,
179.985485069079));
#20897=CARTESIAN_POINT('Ctrl Pts',(-56.2326397064264,-102.645387672678,
179.985484999752));
#20898=CARTESIAN_POINT('Ctrl Pts',(-55.0577300564847,-102.676359662252,
178.813912075476));
#20899=CARTESIAN_POINT('Ctrl Pts',(-53.8828204065429,-102.707331651825,
177.6423391512));
#20900=CARTESIAN_POINT('Ctrl Pts',(-53.872882412563,-102.614109879821,175.985484901707));
#20901=CARTESIAN_POINT('Ctrl Pts',(-53.8629444185832,-102.520888107816,
174.328630652215));
#20902=CARTESIAN_POINT('Ctrl Pts',(-55.0179780401828,-102.303472578539,
173.157057825983));
#20903=CARTESIAN_POINT('Ctrl Pts',(-56.1730116617824,-102.086057049261,
171.985484999752));
#20904=CARTESIAN_POINT('Ctrl Pts',(-57.8105922859523,-101.817198785664,
171.985485069079));
#20905=CARTESIAN_POINT('Ctrl Pts',(-59.4481729101221,-101.548340522067,
171.985485138407));
#20906=CARTESIAN_POINT('Ctrl Pts',(-60.6032064342299,-101.330925003183,
173.157058062683));
#20907=CARTESIAN_POINT('Ctrl Pts',(-61.7582399583376,-101.113509484299,
174.328630986959));
#20908=CARTESIAN_POINT('Ctrl Pts',(-61.7483018264834,-101.020287726993,
175.985485236451));
#20909=CARTESIAN_POINT('Ctrl Pts',(-61.7383636946293,-100.927065969686,
177.642339485944));
#20910=CARTESIAN_POINT('Ctrl Pts',(-60.5634539471956,-100.958037969653,
178.813912312176));
#20911=CARTESIAN_POINT('Ctrl Pts',(-59.388544199762,-100.98900996962,179.985485138407));
#20912=CARTESIAN_POINT('Ctrl Pts',(-57.7310874497581,-101.071424703906,
179.985485069079));
#20913=CARTESIAN_POINT('Ctrl Pts',(-56.0736306997542,-101.153839438193,
179.985484999752));
#20914=CARTESIAN_POINT('Ctrl Pts',(-54.8987210498124,-101.184811427766,
178.813912075476));
#20915=CARTESIAN_POINT('Ctrl Pts',(-53.7238113998707,-101.21578341734,177.6423391512));
#20916=CARTESIAN_POINT('Ctrl Pts',(-53.7138734058908,-101.122561645335,
175.985484901707));
#20917=CARTESIAN_POINT('Ctrl Pts',(-53.7039354119109,-101.029339873331,
174.328630652215));
#20918=CARTESIAN_POINT('Ctrl Pts',(-54.8589690335105,-100.811924344053,
173.157057825983));
#20919=CARTESIAN_POINT('Ctrl Pts',(-56.0140026551102,-100.594508814776,
171.985484999752));
#20920=CARTESIAN_POINT('Ctrl Pts',(-57.65158327928,-100.325650551179,171.985485069079));
#20921=CARTESIAN_POINT('Ctrl Pts',(-59.2891639034499,-100.056792287582,
171.985485138407));
#20922=CARTESIAN_POINT('Ctrl Pts',(-60.4441974275576,-99.8393767686974,
173.157058062683));
#20923=CARTESIAN_POINT('Ctrl Pts',(-61.5992309516654,-99.6219612498133,
174.328630986959));
#20924=CARTESIAN_POINT('Ctrl Pts',(-61.5892928198112,-99.528739492507,175.985485236451));
#20925=CARTESIAN_POINT('Ctrl Pts',(-61.579354687957,-99.4355177352008,177.642339485944));
#20926=CARTESIAN_POINT('Ctrl Pts',(-60.4044449405234,-99.4664897351676,
178.813912312176));
#20927=CARTESIAN_POINT('Ctrl Pts',(-59.2295351930898,-99.4974617351344,
179.985485138407));
#20928=CARTESIAN_POINT('Ctrl Pts',(-57.5720784430859,-99.5798764694207,
179.985485069079));
#20929=CARTESIAN_POINT('Ctrl Pts',(-55.914621693082,-99.662291203707,179.985484999752));
#20930=CARTESIAN_POINT('Ctrl Pts',(-54.7397120431402,-99.6932631932805,
178.813912075476));
#20931=CARTESIAN_POINT('Ctrl Pts',(-53.5648023931984,-99.724235182854,177.6423391512));
#20932=CARTESIAN_POINT('Ctrl Pts',(-53.5548643992186,-99.6310134108495,
175.985484901707));
#20933=CARTESIAN_POINT('Ctrl Pts',(-53.5449264052387,-99.5377916388449,
174.328630652215));
#20934=CARTESIAN_POINT('Ctrl Pts',(-54.6999600268383,-99.3203761095675,
173.157057825983));
#20935=CARTESIAN_POINT('Ctrl Pts',(-55.8549936484379,-99.10296058029,171.985484999752));
#20936=CARTESIAN_POINT('Ctrl Pts',(-57.4925742726078,-98.834102316693,171.985485069079));
#20937=CARTESIAN_POINT('Ctrl Pts',(-59.1301548967777,-98.5652440530961,
171.985485138407));
#20938=CARTESIAN_POINT('Ctrl Pts',(-60.2851884208854,-98.3478285342118,
173.157058062683));
#20939=CARTESIAN_POINT('Ctrl Pts',(-61.4402219449932,-98.1304130153276,
174.328630986959));
#20940=CARTESIAN_POINT('Ctrl Pts',(-61.430283813139,-98.0371912580215,175.985485236451));
#20941=CARTESIAN_POINT('Ctrl Pts',(-61.4203456812848,-97.9439695007152,
177.642339485944));
#20942=CARTESIAN_POINT('Ctrl Pts',(-60.2454359338512,-97.974941500682,178.813912312176));
#20943=CARTESIAN_POINT('Ctrl Pts',(-59.0705261864175,-98.0059135006488,
179.985485138407));
#20944=CARTESIAN_POINT('Ctrl Pts',(-57.4130694364136,-98.0883282349351,
179.985485069079));
#20945=CARTESIAN_POINT('Ctrl Pts',(-55.7556126864097,-98.1707429692214,
179.985484999752));
#20946=CARTESIAN_POINT('Ctrl Pts',(-54.580703036468,-98.2017149587949,178.813912075476));
#20947=CARTESIAN_POINT('Ctrl Pts',(-56.181115489574,-113.283598570176,178.821287383467));
#20948=CARTESIAN_POINT('Ctrl Pts',(-55.0031681001975,-113.314894403068,
177.646659506339));
#20949=CARTESIAN_POINT('Ctrl Pts',(-54.9932301063974,-113.221672631044,
175.985484901271));
#20950=CARTESIAN_POINT('Ctrl Pts',(-54.9832921125973,-113.12845085902,174.324310296203));
#20951=CARTESIAN_POINT('Ctrl Pts',(-56.1413634738858,-112.910711486397,
173.149682517375));
#20952=CARTESIAN_POINT('Ctrl Pts',(-57.2994348351743,-112.692972113774,
171.975054738546));
#20953=CARTESIAN_POINT('Ctrl Pts',(-58.9413114718314,-112.423655866545,
171.975054808055));
#20954=CARTESIAN_POINT('Ctrl Pts',(-60.5831881084886,-112.154339619316,
171.975054877564));
#20955=CARTESIAN_POINT('Ctrl Pts',(-61.741259372031,-111.936600257113,173.149682754692));
#20956=CARTESIAN_POINT('Ctrl Pts',(-62.8993306355734,-111.71886089491,174.32431063182));
#20957=CARTESIAN_POINT('Ctrl Pts',(-62.8893925035395,-111.625639137623,
175.985485236888));
#20958=CARTESIAN_POINT('Ctrl Pts',(-62.8794543715055,-111.532417380336,
177.646659841956));
#20959=CARTESIAN_POINT('Ctrl Pts',(-61.701506884383,-111.563713223648,178.821287620784));
#20960=CARTESIAN_POINT('Ctrl Pts',(-60.5235593972605,-111.595009066961,
179.995915399612));
#20961=CARTESIAN_POINT('Ctrl Pts',(-58.8618066347693,-111.677881784879,
179.995915330104));
#20962=CARTESIAN_POINT('Ctrl Pts',(-57.2000538722782,-111.760754502798,
179.995915260595));
#20963=CARTESIAN_POINT('Ctrl Pts',(-56.0221064829017,-111.79205033569,178.821287383467));
#20964=CARTESIAN_POINT('Ctrl Pts',(-54.8441590935253,-111.823346168582,
177.646659506339));
#20965=CARTESIAN_POINT('Ctrl Pts',(-54.8342210997252,-111.730124396559,
175.985484901271));
#20966=CARTESIAN_POINT('Ctrl Pts',(-54.8242831059251,-111.636902624535,
174.324310296203));
#20967=CARTESIAN_POINT('Ctrl Pts',(-55.9823544672136,-111.419163251912,
173.149682517375));
#20968=CARTESIAN_POINT('Ctrl Pts',(-57.1404258285021,-111.201423879289,
171.975054738546));
#20969=CARTESIAN_POINT('Ctrl Pts',(-58.7823024651592,-110.932107632059,
171.975054808055));
#20970=CARTESIAN_POINT('Ctrl Pts',(-60.4241791018163,-110.66279138483,171.975054877564));
#20971=CARTESIAN_POINT('Ctrl Pts',(-61.5822503653587,-110.445052022627,
173.149682754692));
#20972=CARTESIAN_POINT('Ctrl Pts',(-62.7403216289012,-110.227312660424,
174.32431063182));
#20973=CARTESIAN_POINT('Ctrl Pts',(-62.7303834968672,-110.134090903137,
175.985485236888));
#20974=CARTESIAN_POINT('Ctrl Pts',(-62.7204453648333,-110.04086914585,177.646659841956));
#20975=CARTESIAN_POINT('Ctrl Pts',(-61.5424978777108,-110.072164989163,
178.821287620784));
#20976=CARTESIAN_POINT('Ctrl Pts',(-60.3645503905882,-110.103460832475,
179.995915399612));
#20977=CARTESIAN_POINT('Ctrl Pts',(-58.7027976280971,-110.186333550394,
179.995915330104));
#20978=CARTESIAN_POINT('Ctrl Pts',(-57.041044865606,-110.269206268313,179.995915260595));
#20979=CARTESIAN_POINT('Ctrl Pts',(-55.8630974762295,-110.300502101205,
178.821287383467));
#20980=CARTESIAN_POINT('Ctrl Pts',(-54.6851500868531,-110.331797934097,
177.646659506339));
#20981=CARTESIAN_POINT('Ctrl Pts',(-54.675212093053,-110.238576162073,175.985484901271));
#20982=CARTESIAN_POINT('Ctrl Pts',(-54.6652740992529,-110.145354390049,
174.324310296203));
#20983=CARTESIAN_POINT('Ctrl Pts',(-55.8233454605414,-109.927615017426,
173.149682517375));
#20984=CARTESIAN_POINT('Ctrl Pts',(-56.9814168218299,-109.709875644803,
171.975054738546));
#20985=CARTESIAN_POINT('Ctrl Pts',(-58.623293458487,-109.440559397574,171.975054808055));
#20986=CARTESIAN_POINT('Ctrl Pts',(-60.2651700951441,-109.171243150344,
171.975054877564));
#20987=CARTESIAN_POINT('Ctrl Pts',(-61.4232413586865,-108.953503788142,
173.149682754692));
#20988=CARTESIAN_POINT('Ctrl Pts',(-62.581312622229,-108.735764425939,174.32431063182));
#20989=CARTESIAN_POINT('Ctrl Pts',(-62.571374490195,-108.642542668652,175.985485236888));
#20990=CARTESIAN_POINT('Ctrl Pts',(-62.5614363581611,-108.549320911365,
177.646659841956));
#20991=CARTESIAN_POINT('Ctrl Pts',(-61.3834888710385,-108.580616754677,
178.821287620784));
#20992=CARTESIAN_POINT('Ctrl Pts',(-60.205541383916,-108.61191259799,179.995915399612));
#20993=CARTESIAN_POINT('Ctrl Pts',(-58.5437886214249,-108.694785315908,
179.995915330104));
#20994=CARTESIAN_POINT('Ctrl Pts',(-56.8820358589338,-108.777658033827,
179.995915260595));
#20995=CARTESIAN_POINT('Ctrl Pts',(-55.7040884695573,-108.808953866719,
178.821287383467));
#20996=CARTESIAN_POINT('Ctrl Pts',(-54.5261410801808,-108.840249699611,
177.646659506339));
#20997=CARTESIAN_POINT('Ctrl Pts',(-54.5162030863807,-108.747027927587,
175.985484901271));
#20998=CARTESIAN_POINT('Ctrl Pts',(-54.5062650925806,-108.653806155564,
174.324310296203));
#20999=CARTESIAN_POINT('Ctrl Pts',(-55.6643364538691,-108.436066782941,
173.149682517375));
#21000=CARTESIAN_POINT('Ctrl Pts',(-56.8224078151577,-108.218327410317,
171.975054738546));
#21001=CARTESIAN_POINT('Ctrl Pts',(-58.4642844518147,-107.949011163088,
171.975054808055));
#21002=CARTESIAN_POINT('Ctrl Pts',(-60.1061610884719,-107.679694915859,
171.975054877564));
#21003=CARTESIAN_POINT('Ctrl Pts',(-61.2642323520143,-107.461955553656,
173.149682754692));
#21004=CARTESIAN_POINT('Ctrl Pts',(-62.4223036155567,-107.244216191453,
174.32431063182));
#21005=CARTESIAN_POINT('Ctrl Pts',(-62.4123654835228,-107.150994434166,
175.985485236888));
#21006=CARTESIAN_POINT('Ctrl Pts',(-62.4024273514889,-107.057772676879,
177.646659841956));
#21007=CARTESIAN_POINT('Ctrl Pts',(-61.2244798643663,-107.089068520192,
178.821287620784));
#21008=CARTESIAN_POINT('Ctrl Pts',(-60.0465323772438,-107.120364363504,
179.995915399612));
#21009=CARTESIAN_POINT('Ctrl Pts',(-58.3847796147526,-107.203237081423,
179.995915330104));
#21010=CARTESIAN_POINT('Ctrl Pts',(-56.7230268522615,-107.286109799341,
179.995915260595));
#21011=CARTESIAN_POINT('Ctrl Pts',(-55.5450794628851,-107.317405632233,
178.821287383467));
#21012=CARTESIAN_POINT('Ctrl Pts',(-54.3671320735086,-107.348701465125,
177.646659506339));
#21013=CARTESIAN_POINT('Ctrl Pts',(-54.3571940797085,-107.255479693102,
175.985484901271));
#21014=CARTESIAN_POINT('Ctrl Pts',(-54.3472560859084,-107.162257921078,
174.324310296203));
#21015=CARTESIAN_POINT('Ctrl Pts',(-55.5053274471969,-106.944518548455,
173.149682517375));
#21016=CARTESIAN_POINT('Ctrl Pts',(-56.6633988084854,-106.726779175832,
171.975054738546));
#21017=CARTESIAN_POINT('Ctrl Pts',(-58.3052754451425,-106.457462928602,
171.975054808055));
#21018=CARTESIAN_POINT('Ctrl Pts',(-59.9471520817997,-106.188146681373,
171.975054877564));
#21019=CARTESIAN_POINT('Ctrl Pts',(-61.1052233453421,-105.97040731917,173.149682754692));
#21020=CARTESIAN_POINT('Ctrl Pts',(-62.2632946088845,-105.752667956968,
174.32431063182));
#21021=CARTESIAN_POINT('Ctrl Pts',(-62.2533564768505,-105.659446199681,
175.985485236888));
#21022=CARTESIAN_POINT('Ctrl Pts',(-62.2434183448166,-105.566224442394,
177.646659841956));
#21023=CARTESIAN_POINT('Ctrl Pts',(-61.0654708576941,-105.597520285706,
178.821287620784));
#21024=CARTESIAN_POINT('Ctrl Pts',(-59.8875233705716,-105.628816129018,
179.995915399612));
#21025=CARTESIAN_POINT('Ctrl Pts',(-58.2257706080804,-105.711688846937,
179.995915330104));
#21026=CARTESIAN_POINT('Ctrl Pts',(-56.5640178455893,-105.794561564856,
179.995915260595));
#21027=CARTESIAN_POINT('Ctrl Pts',(-55.3860704562128,-105.825857397748,
178.821287383467));
#21028=CARTESIAN_POINT('Ctrl Pts',(-54.2081230668364,-105.85715323064,177.646659506339));
#21029=CARTESIAN_POINT('Ctrl Pts',(-54.1981850730363,-105.763931458616,
175.985484901271));
#21030=CARTESIAN_POINT('Ctrl Pts',(-54.1882470792362,-105.670709686593,
174.324310296203));
#21031=CARTESIAN_POINT('Ctrl Pts',(-55.3463184405247,-105.452970313969,
173.149682517375));
#21032=CARTESIAN_POINT('Ctrl Pts',(-56.5043898018132,-105.235230941346,
171.975054738546));
#21033=CARTESIAN_POINT('Ctrl Pts',(-58.1462664384703,-104.965914694117,
171.975054808055));
#21034=CARTESIAN_POINT('Ctrl Pts',(-59.7881430751274,-104.696598446888,
171.975054877564));
#21035=CARTESIAN_POINT('Ctrl Pts',(-60.9462143386698,-104.478859084685,
173.149682754692));
#21036=CARTESIAN_POINT('Ctrl Pts',(-62.1042856022123,-104.261119722482,
174.32431063182));
#21037=CARTESIAN_POINT('Ctrl Pts',(-62.0943474701783,-104.167897965195,
175.985485236888));
#21038=CARTESIAN_POINT('Ctrl Pts',(-62.0844093381444,-104.074676207908,
177.646659841956));
#21039=CARTESIAN_POINT('Ctrl Pts',(-60.9064618510219,-104.10597205122,178.821287620784));
#21040=CARTESIAN_POINT('Ctrl Pts',(-59.7285143638993,-104.137267894533,
179.995915399612));
#21041=CARTESIAN_POINT('Ctrl Pts',(-58.0667616014082,-104.220140612451,
179.995915330104));
#21042=CARTESIAN_POINT('Ctrl Pts',(-56.4050088389171,-104.30301333037,179.995915260595));
#21043=CARTESIAN_POINT('Ctrl Pts',(-55.2270614495406,-104.334309163262,
178.821287383467));
#21044=CARTESIAN_POINT('Ctrl Pts',(-54.0491140601642,-104.365604996154,
177.646659506339));
#21045=CARTESIAN_POINT('Ctrl Pts',(-54.039176066364,-104.272383224131,175.985484901271));
#21046=CARTESIAN_POINT('Ctrl Pts',(-54.029238072564,-104.179161452107,174.324310296203));
#21047=CARTESIAN_POINT('Ctrl Pts',(-55.1873094338524,-103.961422079484,
173.149682517375));
#21048=CARTESIAN_POINT('Ctrl Pts',(-56.345380795141,-103.743682706861,171.975054738546));
#21049=CARTESIAN_POINT('Ctrl Pts',(-57.9872574317981,-103.474366459631,
171.975054808055));
#21050=CARTESIAN_POINT('Ctrl Pts',(-59.6291340684552,-103.205050212402,
171.975054877564));
#21051=CARTESIAN_POINT('Ctrl Pts',(-60.7872053319976,-102.987310850199,
173.149682754692));
#21052=CARTESIAN_POINT('Ctrl Pts',(-61.94527659554,-102.769571487996,174.32431063182));
#21053=CARTESIAN_POINT('Ctrl Pts',(-61.9353384635061,-102.676349730709,
175.985485236888));
#21054=CARTESIAN_POINT('Ctrl Pts',(-61.9254003314722,-102.583127973422,
177.646659841956));
#21055=CARTESIAN_POINT('Ctrl Pts',(-60.7474528443496,-102.614423816735,
178.821287620784));
#21056=CARTESIAN_POINT('Ctrl Pts',(-59.5695053572271,-102.645719660047,
179.995915399612));
#21057=CARTESIAN_POINT('Ctrl Pts',(-57.907752594736,-102.728592377966,179.995915330104));
#21058=CARTESIAN_POINT('Ctrl Pts',(-56.2459998322448,-102.811465095885,
179.995915260595));
#21059=CARTESIAN_POINT('Ctrl Pts',(-55.0680524428684,-102.842760928777,
178.821287383467));
#21060=CARTESIAN_POINT('Ctrl Pts',(-53.8901050534919,-102.874056761669,
177.646659506339));
#21061=CARTESIAN_POINT('Ctrl Pts',(-53.8801670596918,-102.780834989645,
175.985484901271));
#21062=CARTESIAN_POINT('Ctrl Pts',(-53.8702290658917,-102.687613217621,
174.324310296203));
#21063=CARTESIAN_POINT('Ctrl Pts',(-55.0283004271802,-102.469873844998,
173.149682517375));
#21064=CARTESIAN_POINT('Ctrl Pts',(-56.1863717884687,-102.252134472375,
171.975054738546));
#21065=CARTESIAN_POINT('Ctrl Pts',(-57.8282484251258,-101.982818225146,
171.975054808055));
#21066=CARTESIAN_POINT('Ctrl Pts',(-59.470125061783,-101.713501977916,171.975054877564));
#21067=CARTESIAN_POINT('Ctrl Pts',(-60.6281963253254,-101.495762615714,
173.149682754692));
#21068=CARTESIAN_POINT('Ctrl Pts',(-61.7862675888678,-101.278023253511,
174.32431063182));
#21069=CARTESIAN_POINT('Ctrl Pts',(-61.7763294568339,-101.184801496224,
175.985485236888));
#21070=CARTESIAN_POINT('Ctrl Pts',(-61.7663913247999,-101.091579738937,
177.646659841956));
#21071=CARTESIAN_POINT('Ctrl Pts',(-60.5884438376774,-101.122875582249,
178.821287620784));
#21072=CARTESIAN_POINT('Ctrl Pts',(-59.4104963505549,-101.154171425562,
179.995915399612));
#21073=CARTESIAN_POINT('Ctrl Pts',(-57.7487435880637,-101.23704414348,179.995915330104));
#21074=CARTESIAN_POINT('Ctrl Pts',(-56.0869908255726,-101.319916861399,
179.995915260595));
#21075=CARTESIAN_POINT('Ctrl Pts',(-54.9090434361961,-101.351212694291,
178.821287383467));
#21076=CARTESIAN_POINT('Ctrl Pts',(-53.7310960468197,-101.382508527183,
177.646659506339));
#21077=CARTESIAN_POINT('Ctrl Pts',(-53.7211580530196,-101.289286755159,
175.985484901271));
#21078=CARTESIAN_POINT('Ctrl Pts',(-53.7112200592195,-101.196064983136,
174.324310296203));
#21079=CARTESIAN_POINT('Ctrl Pts',(-54.869291420508,-100.978325610513,173.149682517375));
#21080=CARTESIAN_POINT('Ctrl Pts',(-56.0273627817965,-100.760586237889,
171.975054738546));
#21081=CARTESIAN_POINT('Ctrl Pts',(-57.6692394184536,-100.49126999066,171.975054808055));
#21082=CARTESIAN_POINT('Ctrl Pts',(-59.3111160551107,-100.221953743431,
171.975054877564));
#21083=CARTESIAN_POINT('Ctrl Pts',(-60.4691873186531,-100.004214381228,
173.149682754692));
#21084=CARTESIAN_POINT('Ctrl Pts',(-61.6272585821956,-99.7864750190253,
174.32431063182));
#21085=CARTESIAN_POINT('Ctrl Pts',(-61.6173204501616,-99.6932532617382,
175.985485236888));
#21086=CARTESIAN_POINT('Ctrl Pts',(-61.6073823181277,-99.6000315044512,
177.646659841956));
#21087=CARTESIAN_POINT('Ctrl Pts',(-60.4294348310052,-99.6313273477637,
178.821287620784));
#21088=CARTESIAN_POINT('Ctrl Pts',(-59.2514873438827,-99.6626231910761,
179.995915399612));
#21089=CARTESIAN_POINT('Ctrl Pts',(-57.5897345813915,-99.7454959089947,
179.995915330104));
#21090=CARTESIAN_POINT('Ctrl Pts',(-55.9279818189004,-99.8283686269133,
179.995915260595));
#21091=CARTESIAN_POINT('Ctrl Pts',(-54.7500344295239,-99.8596644598054,
178.821287383467));
#21092=CARTESIAN_POINT('Ctrl Pts',(-53.5720870401475,-99.8909602926975,
177.646659506339));
#21093=CARTESIAN_POINT('Ctrl Pts',(-53.5621490463474,-99.7977385206737,
175.985484901271));
#21094=CARTESIAN_POINT('Ctrl Pts',(-53.5522110525473,-99.7045167486501,
174.324310296203));
#21095=CARTESIAN_POINT('Ctrl Pts',(-54.7102824138358,-99.4867773760269,
173.149682517375));
#21096=CARTESIAN_POINT('Ctrl Pts',(-55.8683537751243,-99.2690380034038,
171.975054738546));
#21097=CARTESIAN_POINT('Ctrl Pts',(-57.5102304117814,-98.9997217561745,
171.975054808055));
#21098=CARTESIAN_POINT('Ctrl Pts',(-59.1521070484385,-98.7304055089452,
171.975054877564));
#21099=CARTESIAN_POINT('Ctrl Pts',(-60.3101783119809,-98.5126661467424,
173.149682754692));
#21100=CARTESIAN_POINT('Ctrl Pts',(-61.4682495755234,-98.2949267845397,
174.32431063182));
#21101=CARTESIAN_POINT('Ctrl Pts',(-61.4583114434894,-98.2017050272526,
175.985485236888));
#21102=CARTESIAN_POINT('Ctrl Pts',(-61.4483733114555,-98.1084832699656,
177.646659841956));
#21103=CARTESIAN_POINT('Ctrl Pts',(-60.2704258243329,-98.139779113278,178.821287620784));
#21104=CARTESIAN_POINT('Ctrl Pts',(-59.0924783372104,-98.1710749565905,
179.995915399612));
#21105=CARTESIAN_POINT('Ctrl Pts',(-57.4307255747193,-98.2539476745091,
179.995915330104));
#21106=CARTESIAN_POINT('Ctrl Pts',(-55.7689728122282,-98.3368203924277,
179.995915260595));
#21107=CARTESIAN_POINT('Ctrl Pts',(-54.5910254228517,-98.3681162253198,
178.821287383467));
#21108=CARTESIAN_POINT('Ctrl Pts',(-56.1988062143188,-113.449542435949,
178.821287383467));
#21109=CARTESIAN_POINT('Ctrl Pts',(-55.0208588249424,-113.480838268841,
177.646659506339));
#21110=CARTESIAN_POINT('Ctrl Pts',(-55.0109208311422,-113.387616496817,
175.985484901271));
#21111=CARTESIAN_POINT('Ctrl Pts',(-55.0009828373422,-113.294394724794,
174.324310296203));
#21112=CARTESIAN_POINT('Ctrl Pts',(-56.1590541986307,-113.07665535217,173.149682517375));
#21113=CARTESIAN_POINT('Ctrl Pts',(-57.3171255599192,-112.858915979547,
171.975054738546));
#21114=CARTESIAN_POINT('Ctrl Pts',(-58.9590021965763,-112.589599732318,
171.975054808055));
#21115=CARTESIAN_POINT('Ctrl Pts',(-60.6008788332334,-112.320283485089,
171.975054877564));
#21116=CARTESIAN_POINT('Ctrl Pts',(-61.7589500967758,-112.102544122886,
173.149682754692));
#21117=CARTESIAN_POINT('Ctrl Pts',(-62.9170213603182,-111.884804760683,
174.32431063182));
#21118=CARTESIAN_POINT('Ctrl Pts',(-62.9070832282843,-111.791583003396,
175.985485236888));
#21119=CARTESIAN_POINT('Ctrl Pts',(-62.8971450962504,-111.698361246109,
177.646659841956));
#21120=CARTESIAN_POINT('Ctrl Pts',(-61.7191976091278,-111.729657089422,
178.821287620784));
#21121=CARTESIAN_POINT('Ctrl Pts',(-60.5412501220053,-111.760952932734,
179.995915399612));
#21122=CARTESIAN_POINT('Ctrl Pts',(-58.8794973595142,-111.843825650653,
179.995915330104));
#21123=CARTESIAN_POINT('Ctrl Pts',(-57.217744597023,-111.926698368571,179.995915260595));
#21124=CARTESIAN_POINT('Ctrl Pts',(-56.0397972076466,-111.957994201463,
178.821287383467));
#21125=CARTESIAN_POINT('Ctrl Pts',(-54.8618498182701,-111.989290034355,
177.646659506339));
#21126=CARTESIAN_POINT('Ctrl Pts',(-54.85191182447,-111.896068262332,175.985484901271));
#21127=CARTESIAN_POINT('Ctrl Pts',(-54.8419738306699,-111.802846490308,
174.324310296203));
#21128=CARTESIAN_POINT('Ctrl Pts',(-56.0000451919584,-111.585107117685,
173.149682517375));
#21129=CARTESIAN_POINT('Ctrl Pts',(-57.158116553247,-111.367367745062,171.975054738546));
#21130=CARTESIAN_POINT('Ctrl Pts',(-58.799993189904,-111.098051497832,171.975054808055));
#21131=CARTESIAN_POINT('Ctrl Pts',(-60.4418698265612,-110.828735250603,
171.975054877564));
#21132=CARTESIAN_POINT('Ctrl Pts',(-61.5999410901036,-110.6109958884,173.149682754692));
#21133=CARTESIAN_POINT('Ctrl Pts',(-62.758012353646,-110.393256526198,174.32431063182));
#21134=CARTESIAN_POINT('Ctrl Pts',(-62.7480742216121,-110.30003476891,175.985485236888));
#21135=CARTESIAN_POINT('Ctrl Pts',(-62.7381360895782,-110.206813011623,
177.646659841956));
#21136=CARTESIAN_POINT('Ctrl Pts',(-61.5601886024556,-110.238108854936,
178.821287620784));
#21137=CARTESIAN_POINT('Ctrl Pts',(-60.3822411153331,-110.269404698248,
179.995915399612));
#21138=CARTESIAN_POINT('Ctrl Pts',(-58.7204883528419,-110.352277416167,
179.995915330104));
#21139=CARTESIAN_POINT('Ctrl Pts',(-57.0587355903508,-110.435150134086,
179.995915260595));
#21140=CARTESIAN_POINT('Ctrl Pts',(-55.8807882009743,-110.466445966978,
178.821287383467));
#21141=CARTESIAN_POINT('Ctrl Pts',(-54.7028408115979,-110.49774179987,177.646659506339));
#21142=CARTESIAN_POINT('Ctrl Pts',(-54.6929028177978,-110.404520027846,
175.985484901271));
#21143=CARTESIAN_POINT('Ctrl Pts',(-54.6829648239977,-110.311298255822,
174.324310296203));
#21144=CARTESIAN_POINT('Ctrl Pts',(-55.8410361852862,-110.093558883199,
173.149682517375));
#21145=CARTESIAN_POINT('Ctrl Pts',(-56.9991075465747,-109.875819510576,
171.975054738546));
#21146=CARTESIAN_POINT('Ctrl Pts',(-58.6409841832318,-109.606503263347,
171.975054808055));
#21147=CARTESIAN_POINT('Ctrl Pts',(-60.2828608198889,-109.337187016117,
171.975054877564));
#21148=CARTESIAN_POINT('Ctrl Pts',(-61.4409320834313,-109.119447653915,
173.149682754692));
#21149=CARTESIAN_POINT('Ctrl Pts',(-62.5990033469738,-108.901708291712,
174.32431063182));
#21150=CARTESIAN_POINT('Ctrl Pts',(-62.5890652149398,-108.808486534425,
175.985485236888));
#21151=CARTESIAN_POINT('Ctrl Pts',(-62.5791270829059,-108.715264777138,
177.646659841956));
#21152=CARTESIAN_POINT('Ctrl Pts',(-61.4011795957834,-108.74656062045,178.821287620784));
#21153=CARTESIAN_POINT('Ctrl Pts',(-60.2232321086609,-108.777856463763,
179.995915399612));
#21154=CARTESIAN_POINT('Ctrl Pts',(-58.5614793461697,-108.860729181681,
179.995915330104));
#21155=CARTESIAN_POINT('Ctrl Pts',(-56.8997265836786,-108.9436018996,179.995915260595));
#21156=CARTESIAN_POINT('Ctrl Pts',(-55.7217791943021,-108.974897732492,
178.821287383467));
#21157=CARTESIAN_POINT('Ctrl Pts',(-54.5438318049257,-109.006193565384,
177.646659506339));
#21158=CARTESIAN_POINT('Ctrl Pts',(-54.5338938111256,-108.91297179336,175.985484901271));
#21159=CARTESIAN_POINT('Ctrl Pts',(-54.5239558173255,-108.819750021337,
174.324310296203));
#21160=CARTESIAN_POINT('Ctrl Pts',(-55.682027178614,-108.602010648714,173.149682517375));
#21161=CARTESIAN_POINT('Ctrl Pts',(-56.8400985399025,-108.384271276091,
171.975054738546));
#21162=CARTESIAN_POINT('Ctrl Pts',(-58.4819751765596,-108.114955028861,
171.975054808055));
#21163=CARTESIAN_POINT('Ctrl Pts',(-60.1238518132167,-107.845638781632,
171.975054877564));
#21164=CARTESIAN_POINT('Ctrl Pts',(-61.2819230767591,-107.627899419429,
173.149682754692));
#21165=CARTESIAN_POINT('Ctrl Pts',(-62.4399943403016,-107.410160057226,
174.32431063182));
#21166=CARTESIAN_POINT('Ctrl Pts',(-62.4300562082676,-107.316938299939,
175.985485236888));
#21167=CARTESIAN_POINT('Ctrl Pts',(-62.4201180762337,-107.223716542652,
177.646659841956));
#21168=CARTESIAN_POINT('Ctrl Pts',(-61.2421705891111,-107.255012385965,
178.821287620784));
#21169=CARTESIAN_POINT('Ctrl Pts',(-60.0642231019886,-107.286308229277,
179.995915399612));
#21170=CARTESIAN_POINT('Ctrl Pts',(-58.4024703394975,-107.369180947196,
179.995915330104));
#21171=CARTESIAN_POINT('Ctrl Pts',(-56.7407175770064,-107.452053665114,
179.995915260595));
#21172=CARTESIAN_POINT('Ctrl Pts',(-55.5627701876299,-107.483349498006,
178.821287383467));
#21173=CARTESIAN_POINT('Ctrl Pts',(-54.3848227982534,-107.514645330899,
177.646659506339));
#21174=CARTESIAN_POINT('Ctrl Pts',(-54.3748848044533,-107.421423558875,
175.985484901271));
#21175=CARTESIAN_POINT('Ctrl Pts',(-54.3649468106533,-107.328201786851,
174.324310296203));
#21176=CARTESIAN_POINT('Ctrl Pts',(-55.5230181719417,-107.110462414228,
173.149682517375));
#21177=CARTESIAN_POINT('Ctrl Pts',(-56.6810895332303,-106.892723041605,
171.975054738546));
#21178=CARTESIAN_POINT('Ctrl Pts',(-58.3229661698874,-106.623406794376,
171.975054808055));
#21179=CARTESIAN_POINT('Ctrl Pts',(-59.9648428065445,-106.354090547146,
171.975054877564));
#21180=CARTESIAN_POINT('Ctrl Pts',(-61.1229140700869,-106.136351184943,
173.149682754692));
#21181=CARTESIAN_POINT('Ctrl Pts',(-62.2809853336293,-105.918611822741,
174.32431063182));
#21182=CARTESIAN_POINT('Ctrl Pts',(-62.2710472015954,-105.825390065454,
175.985485236888));
#21183=CARTESIAN_POINT('Ctrl Pts',(-62.2611090695615,-105.732168308167,
177.646659841956));
#21184=CARTESIAN_POINT('Ctrl Pts',(-61.0831615824389,-105.763464151479,
178.821287620784));
#21185=CARTESIAN_POINT('Ctrl Pts',(-59.9052140953164,-105.794759994792,
179.995915399612));
#21186=CARTESIAN_POINT('Ctrl Pts',(-58.2434613328252,-105.87763271271,179.995915330104));
#21187=CARTESIAN_POINT('Ctrl Pts',(-56.5817085703341,-105.960505430629,
179.995915260595));
#21188=CARTESIAN_POINT('Ctrl Pts',(-55.4037611809577,-105.991801263521,
178.821287383467));
#21189=CARTESIAN_POINT('Ctrl Pts',(-54.2258137915812,-106.023097096413,
177.646659506339));
#21190=CARTESIAN_POINT('Ctrl Pts',(-54.2158757977811,-105.929875324389,
175.985484901271));
#21191=CARTESIAN_POINT('Ctrl Pts',(-54.205937803981,-105.836653552366,174.324310296203));
#21192=CARTESIAN_POINT('Ctrl Pts',(-55.3640091652695,-105.618914179742,
173.149682517375));
#21193=CARTESIAN_POINT('Ctrl Pts',(-56.522080526558,-105.401174807119,171.975054738546));
#21194=CARTESIAN_POINT('Ctrl Pts',(-58.1639571632151,-105.13185855989,171.975054808055));
#21195=CARTESIAN_POINT('Ctrl Pts',(-59.8058337998722,-104.862542312661,
171.975054877564));
#21196=CARTESIAN_POINT('Ctrl Pts',(-60.9639050634147,-104.644802950458,
173.149682754692));
#21197=CARTESIAN_POINT('Ctrl Pts',(-62.1219763269571,-104.427063588255,
174.32431063182));
#21198=CARTESIAN_POINT('Ctrl Pts',(-62.1120381949232,-104.333841830968,
175.985485236888));
#21199=CARTESIAN_POINT('Ctrl Pts',(-62.1021000628892,-104.240620073681,
177.646659841956));
#21200=CARTESIAN_POINT('Ctrl Pts',(-60.9241525757667,-104.271915916993,
178.821287620784));
#21201=CARTESIAN_POINT('Ctrl Pts',(-59.7462050886442,-104.303211760306,
179.995915399612));
#21202=CARTESIAN_POINT('Ctrl Pts',(-58.084452326153,-104.386084478225,179.995915330104));
#21203=CARTESIAN_POINT('Ctrl Pts',(-56.4226995636619,-104.468957196143,
179.995915260595));
#21204=CARTESIAN_POINT('Ctrl Pts',(-55.2447521742854,-104.500253029035,
178.821287383467));
#21205=CARTESIAN_POINT('Ctrl Pts',(-54.066804784909,-104.531548861927,177.646659506339));
#21206=CARTESIAN_POINT('Ctrl Pts',(-54.0568667911089,-104.438327089904,
175.985484901271));
#21207=CARTESIAN_POINT('Ctrl Pts',(-54.0469287973088,-104.34510531788,174.324310296203));
#21208=CARTESIAN_POINT('Ctrl Pts',(-55.2050001585973,-104.127365945257,
173.149682517375));
#21209=CARTESIAN_POINT('Ctrl Pts',(-56.3630715198858,-103.909626572634,
171.975054738546));
#21210=CARTESIAN_POINT('Ctrl Pts',(-58.0049481565429,-103.640310325404,
171.975054808055));
#21211=CARTESIAN_POINT('Ctrl Pts',(-59.6468247932,-103.370994078175,171.975054877564));
#21212=CARTESIAN_POINT('Ctrl Pts',(-60.8048960567424,-103.153254715972,
173.149682754692));
#21213=CARTESIAN_POINT('Ctrl Pts',(-61.9629673202849,-102.93551535377,174.32431063182));
#21214=CARTESIAN_POINT('Ctrl Pts',(-61.9530291882509,-102.842293596483,
175.985485236888));
#21215=CARTESIAN_POINT('Ctrl Pts',(-61.943091056217,-102.749071839196,177.646659841956));
#21216=CARTESIAN_POINT('Ctrl Pts',(-60.7651435690945,-102.780367682508,
178.821287620784));
#21217=CARTESIAN_POINT('Ctrl Pts',(-59.587196081972,-102.81166352582,179.995915399612));
#21218=CARTESIAN_POINT('Ctrl Pts',(-57.9254433194808,-102.894536243739,
179.995915330104));
#21219=CARTESIAN_POINT('Ctrl Pts',(-56.2636905569897,-102.977408961658,
179.995915260595));
#21220=CARTESIAN_POINT('Ctrl Pts',(-55.0857431676132,-103.00870479455,178.821287383467));
#21221=CARTESIAN_POINT('Ctrl Pts',(-53.9077957782368,-103.040000627442,
177.646659506339));
#21222=CARTESIAN_POINT('Ctrl Pts',(-53.8978577844367,-102.946778855418,
175.985484901271));
#21223=CARTESIAN_POINT('Ctrl Pts',(-53.8879197906366,-102.853557083394,
174.324310296203));
#21224=CARTESIAN_POINT('Ctrl Pts',(-55.0459911519251,-102.635817710771,
173.149682517375));
#21225=CARTESIAN_POINT('Ctrl Pts',(-56.2040625132136,-102.418078338148,
171.975054738546));
#21226=CARTESIAN_POINT('Ctrl Pts',(-57.8459391498707,-102.148762090919,
171.975054808055));
#21227=CARTESIAN_POINT('Ctrl Pts',(-59.4878157865278,-101.879445843689,
171.975054877564));
#21228=CARTESIAN_POINT('Ctrl Pts',(-60.6458870500702,-101.661706481487,
173.149682754692));
#21229=CARTESIAN_POINT('Ctrl Pts',(-61.8039583136126,-101.443967119284,
174.32431063182));
#21230=CARTESIAN_POINT('Ctrl Pts',(-61.7940201815787,-101.350745361997,
175.985485236888));
#21231=CARTESIAN_POINT('Ctrl Pts',(-61.7840820495448,-101.25752360471,177.646659841956));
#21232=CARTESIAN_POINT('Ctrl Pts',(-60.6061345624222,-101.288819448022,
178.821287620784));
#21233=CARTESIAN_POINT('Ctrl Pts',(-59.4281870752997,-101.320115291335,
179.995915399612));
#21234=CARTESIAN_POINT('Ctrl Pts',(-57.7664343128086,-101.402988009253,
179.995915330104));
#21235=CARTESIAN_POINT('Ctrl Pts',(-56.1046815503175,-101.485860727172,
179.995915260595));
#21236=CARTESIAN_POINT('Ctrl Pts',(-54.926734160941,-101.517156560064,178.821287383467));
#21237=CARTESIAN_POINT('Ctrl Pts',(-53.7487867715645,-101.548452392956,
177.646659506339));
#21238=CARTESIAN_POINT('Ctrl Pts',(-53.7388487777644,-101.455230620932,
175.985484901271));
#21239=CARTESIAN_POINT('Ctrl Pts',(-53.7289107839643,-101.362008848909,
174.324310296203));
#21240=CARTESIAN_POINT('Ctrl Pts',(-54.8869821452528,-101.144269476286,
173.149682517375));
#21241=CARTESIAN_POINT('Ctrl Pts',(-56.0450535065414,-100.926530103662,
171.975054738546));
#21242=CARTESIAN_POINT('Ctrl Pts',(-57.6869301431984,-100.657213856433,
171.975054808055));
#21243=CARTESIAN_POINT('Ctrl Pts',(-59.3288067798556,-100.387897609204,
171.975054877564));
#21244=CARTESIAN_POINT('Ctrl Pts',(-60.486878043398,-100.170158247001,173.149682754692));
#21245=CARTESIAN_POINT('Ctrl Pts',(-61.6449493069404,-99.9524188847983,
174.32431063182));
#21246=CARTESIAN_POINT('Ctrl Pts',(-61.6350111749065,-99.8591971275113,
175.985485236888));
#21247=CARTESIAN_POINT('Ctrl Pts',(-61.6250730428726,-99.7659753702243,
177.646659841956));
#21248=CARTESIAN_POINT('Ctrl Pts',(-60.44712555575,-99.7972712135367,178.821287620784));
#21249=CARTESIAN_POINT('Ctrl Pts',(-59.2691780686275,-99.8285670568492,
179.995915399612));
#21250=CARTESIAN_POINT('Ctrl Pts',(-57.6074253061363,-99.9114397747677,
179.995915330104));
#21251=CARTESIAN_POINT('Ctrl Pts',(-55.9456725436452,-99.9943124926864,
179.995915260595));
#21252=CARTESIAN_POINT('Ctrl Pts',(-54.7677251542687,-100.025608325578,
178.821287383467));
#21253=CARTESIAN_POINT('Ctrl Pts',(-53.5897777648923,-100.05690415847,177.646659506339));
#21254=CARTESIAN_POINT('Ctrl Pts',(-53.5798397710922,-99.9636823864468,
175.985484901271));
#21255=CARTESIAN_POINT('Ctrl Pts',(-53.5699017772921,-99.8704606144232,
174.324310296203));
#21256=CARTESIAN_POINT('Ctrl Pts',(-54.7279731385806,-99.6527212418,173.149682517375));
#21257=CARTESIAN_POINT('Ctrl Pts',(-55.8860444998691,-99.4349818691769,
171.975054738546));
#21258=CARTESIAN_POINT('Ctrl Pts',(-57.5279211365262,-99.1656656219475,
171.975054808055));
#21259=CARTESIAN_POINT('Ctrl Pts',(-59.1697977731833,-98.8963493747183,
171.975054877564));
#21260=CARTESIAN_POINT('Ctrl Pts',(-60.3278690367257,-98.6786100125155,
173.149682754692));
#21261=CARTESIAN_POINT('Ctrl Pts',(-61.4859403002682,-98.4608706503128,
174.32431063182));
#21262=CARTESIAN_POINT('Ctrl Pts',(-61.4760021682342,-98.3676488930257,
175.985485236888));
#21263=CARTESIAN_POINT('Ctrl Pts',(-61.4660640362003,-98.2744271357387,
177.646659841956));
#21264=CARTESIAN_POINT('Ctrl Pts',(-60.2881165490778,-98.3057229790511,
178.821287620784));
#21265=CARTESIAN_POINT('Ctrl Pts',(-59.1101690619552,-98.3370188223636,
179.995915399612));
#21266=CARTESIAN_POINT('Ctrl Pts',(-57.4484162994641,-98.4198915402821,
179.995915330104));
#21267=CARTESIAN_POINT('Ctrl Pts',(-55.786663536973,-98.5027642582008,179.995915260595));
#21268=CARTESIAN_POINT('Ctrl Pts',(-54.6087161475965,-98.5340600910929,
178.821287383467));
#21269=CARTESIAN_POINT('Ctrl Pts',(-56.2237961054143,-113.614380048479,
178.813912075476));
#21270=CARTESIAN_POINT('Ctrl Pts',(-55.0488864554725,-113.645352038053,
177.6423391512));
#21271=CARTESIAN_POINT('Ctrl Pts',(-55.0389484614927,-113.552130266048,
175.985484901707));
#21272=CARTESIAN_POINT('Ctrl Pts',(-55.0290104675128,-113.458908494044,
174.328630652215));
#21273=CARTESIAN_POINT('Ctrl Pts',(-56.1840440891124,-113.241492964766,
173.157057825983));
#21274=CARTESIAN_POINT('Ctrl Pts',(-57.3390777107121,-113.024077435489,
171.985484999752));
#21275=CARTESIAN_POINT('Ctrl Pts',(-58.9766583348819,-112.755219171892,
171.985485069079));
#21276=CARTESIAN_POINT('Ctrl Pts',(-60.6142389590518,-112.486360908295,
171.985485138407));
#21277=CARTESIAN_POINT('Ctrl Pts',(-61.7692724831595,-112.268945389411,
173.157058062683));
#21278=CARTESIAN_POINT('Ctrl Pts',(-62.9243060072673,-112.051529870527,
174.328630986959));
#21279=CARTESIAN_POINT('Ctrl Pts',(-62.9143678754131,-111.95830811322,175.985485236451));
#21280=CARTESIAN_POINT('Ctrl Pts',(-62.9044297435589,-111.865086355914,
177.642339485944));
#21281=CARTESIAN_POINT('Ctrl Pts',(-61.7295199961253,-111.896058355881,
178.813912312176));
#21282=CARTESIAN_POINT('Ctrl Pts',(-60.5546102486917,-111.927030355848,
179.985485138407));
#21283=CARTESIAN_POINT('Ctrl Pts',(-58.8971534986878,-112.009445090134,
179.985485069079));
#21284=CARTESIAN_POINT('Ctrl Pts',(-57.2396967486839,-112.09185982442,179.985484999752));
#21285=CARTESIAN_POINT('Ctrl Pts',(-56.0647870987421,-112.122831813994,
178.813912075476));
#21286=CARTESIAN_POINT('Ctrl Pts',(-54.8898774488003,-112.153803803567,
177.6423391512));
#21287=CARTESIAN_POINT('Ctrl Pts',(-54.8799394548205,-112.060582031563,
175.985484901707));
#21288=CARTESIAN_POINT('Ctrl Pts',(-54.8700014608406,-111.967360259558,
174.328630652215));
#21289=CARTESIAN_POINT('Ctrl Pts',(-56.0250350824402,-111.749944730281,
173.157057825983));
#21290=CARTESIAN_POINT('Ctrl Pts',(-57.1800687040398,-111.532529201003,
171.985484999752));
#21291=CARTESIAN_POINT('Ctrl Pts',(-58.8176493282097,-111.263670937406,
171.985485069079));
#21292=CARTESIAN_POINT('Ctrl Pts',(-60.4552299523796,-110.994812673809,
171.985485138407));
#21293=CARTESIAN_POINT('Ctrl Pts',(-61.6102634764873,-110.777397154925,
173.157058062683));
#21294=CARTESIAN_POINT('Ctrl Pts',(-62.7652970005951,-110.559981636041,
174.328630986959));
#21295=CARTESIAN_POINT('Ctrl Pts',(-62.7553588687409,-110.466759878735,
175.985485236451));
#21296=CARTESIAN_POINT('Ctrl Pts',(-62.7454207368867,-110.373538121429,
177.642339485944));
#21297=CARTESIAN_POINT('Ctrl Pts',(-61.5705109894531,-110.404510121395,
178.813912312176));
#21298=CARTESIAN_POINT('Ctrl Pts',(-60.3956012420194,-110.435482121362,
179.985485138407));
#21299=CARTESIAN_POINT('Ctrl Pts',(-58.7381444920155,-110.517896855648,
179.985485069079));
#21300=CARTESIAN_POINT('Ctrl Pts',(-57.0806877420116,-110.600311589935,
179.985484999752));
#21301=CARTESIAN_POINT('Ctrl Pts',(-55.9057780920699,-110.631283579508,
178.813912075476));
#21302=CARTESIAN_POINT('Ctrl Pts',(-54.7308684421281,-110.662255569082,
177.6423391512));
#21303=CARTESIAN_POINT('Ctrl Pts',(-54.7209304481482,-110.569033797077,
175.985484901707));
#21304=CARTESIAN_POINT('Ctrl Pts',(-54.7109924541684,-110.475812025073,
174.328630652215));
#21305=CARTESIAN_POINT('Ctrl Pts',(-55.866026075768,-110.258396495795,173.157057825983));
#21306=CARTESIAN_POINT('Ctrl Pts',(-57.0210596973676,-110.040980966518,
171.985484999752));
#21307=CARTESIAN_POINT('Ctrl Pts',(-58.6586403215375,-109.772122702921,
171.985485069079));
#21308=CARTESIAN_POINT('Ctrl Pts',(-60.2962209457073,-109.503264439324,
171.985485138407));
#21309=CARTESIAN_POINT('Ctrl Pts',(-61.4512544698151,-109.28584892044,173.157058062683));
#21310=CARTESIAN_POINT('Ctrl Pts',(-62.6062879939228,-109.068433401555,
174.328630986959));
#21311=CARTESIAN_POINT('Ctrl Pts',(-62.5963498620687,-108.975211644249,
175.985485236451));
#21312=CARTESIAN_POINT('Ctrl Pts',(-62.5864117302145,-108.881989886943,
177.642339485944));
#21313=CARTESIAN_POINT('Ctrl Pts',(-61.4115019827808,-108.91296188691,178.813912312176));
#21314=CARTESIAN_POINT('Ctrl Pts',(-60.2365922353472,-108.943933886877,
179.985485138407));
#21315=CARTESIAN_POINT('Ctrl Pts',(-58.5791354853433,-109.026348621163,
179.985485069079));
#21316=CARTESIAN_POINT('Ctrl Pts',(-56.9216787353394,-109.108763355449,
179.985484999752));
#21317=CARTESIAN_POINT('Ctrl Pts',(-55.7467690853976,-109.139735345023,
178.813912075476));
#21318=CARTESIAN_POINT('Ctrl Pts',(-54.5718594354559,-109.170707334596,
177.6423391512));
#21319=CARTESIAN_POINT('Ctrl Pts',(-54.561921441476,-109.077485562592,175.985484901707));
#21320=CARTESIAN_POINT('Ctrl Pts',(-54.5519834474962,-108.984263790587,
174.328630652215));
#21321=CARTESIAN_POINT('Ctrl Pts',(-55.7070170690958,-108.76684826131,173.157057825983));
#21322=CARTESIAN_POINT('Ctrl Pts',(-56.8620506906954,-108.549432732032,
171.985484999752));
#21323=CARTESIAN_POINT('Ctrl Pts',(-58.4996313148652,-108.280574468435,
171.985485069079));
#21324=CARTESIAN_POINT('Ctrl Pts',(-60.1372119390351,-108.011716204838,
171.985485138407));
#21325=CARTESIAN_POINT('Ctrl Pts',(-61.2922454631428,-107.794300685954,
173.157058062683));
#21326=CARTESIAN_POINT('Ctrl Pts',(-62.4472789872506,-107.57688516707,174.328630986959));
#21327=CARTESIAN_POINT('Ctrl Pts',(-62.4373408553964,-107.483663409764,
175.985485236451));
#21328=CARTESIAN_POINT('Ctrl Pts',(-62.4274027235423,-107.390441652457,
177.642339485944));
#21329=CARTESIAN_POINT('Ctrl Pts',(-61.2524929761086,-107.421413652424,
178.813912312176));
#21330=CARTESIAN_POINT('Ctrl Pts',(-60.077583228675,-107.452385652391,179.985485138407));
#21331=CARTESIAN_POINT('Ctrl Pts',(-58.4201264786711,-107.534800386677,
179.985485069079));
#21332=CARTESIAN_POINT('Ctrl Pts',(-56.7626697286672,-107.617215120964,
179.985484999752));
#21333=CARTESIAN_POINT('Ctrl Pts',(-55.5877600787254,-107.648187110537,
178.813912075476));
#21334=CARTESIAN_POINT('Ctrl Pts',(-54.4128504287836,-107.67915910011,177.6423391512));
#21335=CARTESIAN_POINT('Ctrl Pts',(-54.4029124348038,-107.585937328106,
175.985484901707));
#21336=CARTESIAN_POINT('Ctrl Pts',(-54.3929744408239,-107.492715556102,
174.328630652215));
#21337=CARTESIAN_POINT('Ctrl Pts',(-55.5480080624235,-107.275300026824,
173.157057825983));
#21338=CARTESIAN_POINT('Ctrl Pts',(-56.7030416840231,-107.057884497547,
171.985484999752));
#21339=CARTESIAN_POINT('Ctrl Pts',(-58.340622308193,-106.78902623395,171.985485069079));
#21340=CARTESIAN_POINT('Ctrl Pts',(-59.9782029323629,-106.520167970353,
171.985485138407));
#21341=CARTESIAN_POINT('Ctrl Pts',(-61.1332364564706,-106.302752451468,
173.157058062683));
#21342=CARTESIAN_POINT('Ctrl Pts',(-62.2882699805784,-106.085336932584,
174.328630986959));
#21343=CARTESIAN_POINT('Ctrl Pts',(-62.2783318487242,-105.992115175278,
175.985485236451));
#21344=CARTESIAN_POINT('Ctrl Pts',(-62.26839371687,-105.898893417972,177.642339485944));
#21345=CARTESIAN_POINT('Ctrl Pts',(-61.0934839694364,-105.929865417939,
178.813912312176));
#21346=CARTESIAN_POINT('Ctrl Pts',(-59.9185742220028,-105.960837417905,
179.985485138407));
#21347=CARTESIAN_POINT('Ctrl Pts',(-58.2611174719989,-106.043252152192,
179.985485069079));
#21348=CARTESIAN_POINT('Ctrl Pts',(-56.603660721995,-106.125666886478,179.985484999752));
#21349=CARTESIAN_POINT('Ctrl Pts',(-55.4287510720532,-106.156638876051,
178.813912075476));
#21350=CARTESIAN_POINT('Ctrl Pts',(-54.2538414221114,-106.187610865625,
177.6423391512));
#21351=CARTESIAN_POINT('Ctrl Pts',(-54.2439034281315,-106.09438909362,175.985484901707));
#21352=CARTESIAN_POINT('Ctrl Pts',(-54.2339654341517,-106.001167321616,
174.328630652215));
#21353=CARTESIAN_POINT('Ctrl Pts',(-55.3889990557513,-105.783751792338,
173.157057825983));
#21354=CARTESIAN_POINT('Ctrl Pts',(-56.5440326773509,-105.566336263061,
171.985484999752));
#21355=CARTESIAN_POINT('Ctrl Pts',(-58.1816133015208,-105.297477999464,
171.985485069079));
#21356=CARTESIAN_POINT('Ctrl Pts',(-59.8191939256906,-105.028619735867,
171.985485138407));
#21357=CARTESIAN_POINT('Ctrl Pts',(-60.9742274497984,-104.811204216983,
173.157058062683));
#21358=CARTESIAN_POINT('Ctrl Pts',(-62.1292609739061,-104.593788698099,
174.328630986959));
#21359=CARTESIAN_POINT('Ctrl Pts',(-62.119322842052,-104.500566940792,175.985485236451));
#21360=CARTESIAN_POINT('Ctrl Pts',(-62.1093847101978,-104.407345183486,
177.642339485944));
#21361=CARTESIAN_POINT('Ctrl Pts',(-60.9344749627642,-104.438317183453,
178.813912312176));
#21362=CARTESIAN_POINT('Ctrl Pts',(-59.7595652153305,-104.46928918342,179.985485138407));
#21363=CARTESIAN_POINT('Ctrl Pts',(-58.1021084653266,-104.551703917706,
179.985485069079));
#21364=CARTESIAN_POINT('Ctrl Pts',(-56.4446517153227,-104.634118651992,
179.985484999752));
#21365=CARTESIAN_POINT('Ctrl Pts',(-55.269742065381,-104.665090641566,178.813912075476));
#21366=CARTESIAN_POINT('Ctrl Pts',(-54.0948324154392,-104.696062631139,
177.6423391512));
#21367=CARTESIAN_POINT('Ctrl Pts',(-54.0848944214593,-104.602840859135,
175.985484901707));
#21368=CARTESIAN_POINT('Ctrl Pts',(-54.0749564274795,-104.50961908713,174.328630652215));
#21369=CARTESIAN_POINT('Ctrl Pts',(-55.2299900490791,-104.292203557853,
173.157057825983));
#21370=CARTESIAN_POINT('Ctrl Pts',(-56.3850236706787,-104.074788028575,
171.985484999752));
#21371=CARTESIAN_POINT('Ctrl Pts',(-58.0226042948486,-103.805929764978,
171.985485069079));
#21372=CARTESIAN_POINT('Ctrl Pts',(-59.6601849190184,-103.537071501381,
171.985485138407));
#21373=CARTESIAN_POINT('Ctrl Pts',(-60.8152184431262,-103.319655982497,
173.157058062683));
#21374=CARTESIAN_POINT('Ctrl Pts',(-61.9702519672339,-103.102240463613,
174.328630986959));
#21375=CARTESIAN_POINT('Ctrl Pts',(-61.9603138353797,-103.009018706307,
175.985485236451));
#21376=CARTESIAN_POINT('Ctrl Pts',(-61.9503757035256,-102.915796949001,
177.642339485944));
#21377=CARTESIAN_POINT('Ctrl Pts',(-60.7754659560919,-102.946768948967,
178.813912312176));
#21378=CARTESIAN_POINT('Ctrl Pts',(-59.6005562086583,-102.977740948934,
179.985485138407));
#21379=CARTESIAN_POINT('Ctrl Pts',(-57.9430994586544,-103.06015568322,179.985485069079));
#21380=CARTESIAN_POINT('Ctrl Pts',(-56.2856427086505,-103.142570417507,
179.985484999752));
#21381=CARTESIAN_POINT('Ctrl Pts',(-55.1107330587087,-103.17354240708,178.813912075476));
#21382=CARTESIAN_POINT('Ctrl Pts',(-53.935823408767,-103.204514396654,177.6423391512));
#21383=CARTESIAN_POINT('Ctrl Pts',(-53.9258854147871,-103.111292624649,
175.985484901707));
#21384=CARTESIAN_POINT('Ctrl Pts',(-53.9159474208072,-103.018070852645,
174.328630652215));
#21385=CARTESIAN_POINT('Ctrl Pts',(-55.0709810424069,-102.800655323367,
173.157057825983));
#21386=CARTESIAN_POINT('Ctrl Pts',(-56.2260146640065,-102.58323979409,171.985484999752));
#21387=CARTESIAN_POINT('Ctrl Pts',(-57.8635952881763,-102.314381530493,
171.985485069079));
#21388=CARTESIAN_POINT('Ctrl Pts',(-59.5011759123462,-102.045523266896,
171.985485138407));
#21389=CARTESIAN_POINT('Ctrl Pts',(-60.6562094364539,-101.828107748012,
173.157058062683));
#21390=CARTESIAN_POINT('Ctrl Pts',(-61.8112429605617,-101.610692229127,
174.328630986959));
#21391=CARTESIAN_POINT('Ctrl Pts',(-61.8013048287075,-101.517470471821,
175.985485236451));
#21392=CARTESIAN_POINT('Ctrl Pts',(-61.7913666968533,-101.424248714515,
177.642339485944));
#21393=CARTESIAN_POINT('Ctrl Pts',(-60.6164569494197,-101.455220714482,
178.813912312176));
#21394=CARTESIAN_POINT('Ctrl Pts',(-59.4415472019861,-101.486192714449,
179.985485138407));
#21395=CARTESIAN_POINT('Ctrl Pts',(-57.7840904519822,-101.568607448735,
179.985485069079));
#21396=CARTESIAN_POINT('Ctrl Pts',(-56.1266337019783,-101.651022183021,
179.985484999752));
#21397=CARTESIAN_POINT('Ctrl Pts',(-54.9517240520365,-101.681994172595,
178.813912075476));
#21398=CARTESIAN_POINT('Ctrl Pts',(-53.7768144020947,-101.712966162168,
177.6423391512));
#21399=CARTESIAN_POINT('Ctrl Pts',(-53.7668764081149,-101.619744390164,
175.985484901707));
#21400=CARTESIAN_POINT('Ctrl Pts',(-53.756938414135,-101.526522618159,174.328630652215));
#21401=CARTESIAN_POINT('Ctrl Pts',(-54.9119720357346,-101.309107088882,
173.157057825983));
#21402=CARTESIAN_POINT('Ctrl Pts',(-56.0670056573342,-101.091691559604,
171.985484999752));
#21403=CARTESIAN_POINT('Ctrl Pts',(-57.7045862815041,-100.822833296007,
171.985485069079));
#21404=CARTESIAN_POINT('Ctrl Pts',(-59.342166905674,-100.55397503241,171.985485138407));
#21405=CARTESIAN_POINT('Ctrl Pts',(-60.4972004297817,-100.336559513526,
173.157058062683));
#21406=CARTESIAN_POINT('Ctrl Pts',(-61.6522339538895,-100.119143994642,
174.328630986959));
#21407=CARTESIAN_POINT('Ctrl Pts',(-61.6422958220353,-100.025922237336,
175.985485236451));
#21408=CARTESIAN_POINT('Ctrl Pts',(-61.6323576901811,-99.9327004800294,
177.642339485944));
#21409=CARTESIAN_POINT('Ctrl Pts',(-60.4574479427475,-99.9636724799962,
178.813912312176));
#21410=CARTESIAN_POINT('Ctrl Pts',(-59.2825381953138,-99.994644479963,179.985485138407));
#21411=CARTESIAN_POINT('Ctrl Pts',(-57.6250814453099,-100.077059214249,
179.985485069079));
#21412=CARTESIAN_POINT('Ctrl Pts',(-55.9676246953061,-100.159473948536,
179.985484999752));
#21413=CARTESIAN_POINT('Ctrl Pts',(-54.7927150453643,-100.190445938109,
178.813912075476));
#21414=CARTESIAN_POINT('Ctrl Pts',(-53.6178053954225,-100.221417927683,
177.6423391512));
#21415=CARTESIAN_POINT('Ctrl Pts',(-53.6078674014426,-100.128196155678,
175.985484901707));
#21416=CARTESIAN_POINT('Ctrl Pts',(-53.5979294074628,-100.034974383673,
174.328630652215));
#21417=CARTESIAN_POINT('Ctrl Pts',(-54.7529630290624,-99.817558854396,173.157057825983));
#21418=CARTESIAN_POINT('Ctrl Pts',(-55.907996650662,-99.6001433251185,171.985484999752));
#21419=CARTESIAN_POINT('Ctrl Pts',(-57.5455772748319,-99.3312850615215,
171.985485069079));
#21420=CARTESIAN_POINT('Ctrl Pts',(-59.1831578990017,-99.0624267979246,
171.985485138407));
#21421=CARTESIAN_POINT('Ctrl Pts',(-60.3381914231095,-98.8450112790404,
173.157058062683));
#21422=CARTESIAN_POINT('Ctrl Pts',(-61.4932249472172,-98.6275957601562,
174.328630986959));
#21423=CARTESIAN_POINT('Ctrl Pts',(-61.4832868153631,-98.53437400285,175.985485236451));
#21424=CARTESIAN_POINT('Ctrl Pts',(-61.4733486835089,-98.4411522455438,
177.642339485944));
#21425=CARTESIAN_POINT('Ctrl Pts',(-60.2984389360752,-98.4721242455106,
178.813912312176));
#21426=CARTESIAN_POINT('Ctrl Pts',(-59.1235291886416,-98.5030962454774,
179.985485138407));
#21427=CARTESIAN_POINT('Ctrl Pts',(-57.4660724386377,-98.5855109797636,
179.985485069079));
#21428=CARTESIAN_POINT('Ctrl Pts',(-55.8086156886338,-98.6679257140499,
179.985484999752));
#21429=CARTESIAN_POINT('Ctrl Pts',(-54.633706038692,-98.6988977036234,178.813912075476));
#21430=CARTESIAN_POINT('Ctrl Pts',(-56.1707931031902,-113.117197303651,
178.813912075476));
#21431=CARTESIAN_POINT('Ctrl Pts',(-54.9958834532485,-113.148169293224,
177.6423391512));
#21432=CARTESIAN_POINT('Ctrl Pts',(-54.9859454592686,-113.05494752122,175.985484901707));
#21433=CARTESIAN_POINT('Ctrl Pts',(-54.9760074652888,-112.961725749215,
174.328630652215));
#21434=CARTESIAN_POINT('Ctrl Pts',(-56.1310410868884,-112.744310219938,
173.157057825983));
#21435=CARTESIAN_POINT('Ctrl Pts',(-57.286074708488,-112.52689469066,171.985484999752));
#21436=CARTESIAN_POINT('Ctrl Pts',(-58.9236553326578,-112.258036427063,
171.985485069079));
#21437=CARTESIAN_POINT('Ctrl Pts',(-60.5612359568277,-111.989178163466,
171.985485138407));
#21438=CARTESIAN_POINT('Ctrl Pts',(-61.7162694809355,-111.771762644582,
173.157058062683));
#21439=CARTESIAN_POINT('Ctrl Pts',(-62.8713030050432,-111.554347125698,
174.328630986959));
#21440=CARTESIAN_POINT('Ctrl Pts',(-62.861364873189,-111.461125368392,175.985485236451));
#21441=CARTESIAN_POINT('Ctrl Pts',(-62.8514267413349,-111.367903611086,
177.642339485944));
#21442=CARTESIAN_POINT('Ctrl Pts',(-61.6765169939012,-111.398875611052,
178.813912312176));
#21443=CARTESIAN_POINT('Ctrl Pts',(-60.5016072464676,-111.429847611019,
179.985485138407));
#21444=CARTESIAN_POINT('Ctrl Pts',(-58.8441504964637,-111.512262345305,
179.985485069079));
#21445=CARTESIAN_POINT('Ctrl Pts',(-57.1866937464598,-111.594677079592,
179.985484999752));
#21446=CARTESIAN_POINT('Ctrl Pts',(-56.011784096518,-111.625649069165,178.813912075476));
#21447=CARTESIAN_POINT('Ctrl Pts',(-54.8368744465763,-111.656621058739,
177.6423391512));
#21448=CARTESIAN_POINT('Ctrl Pts',(-54.8269364525964,-111.563399286734,
175.985484901707));
#21449=CARTESIAN_POINT('Ctrl Pts',(-54.8169984586165,-111.47017751473,174.328630652215));
#21450=CARTESIAN_POINT('Ctrl Pts',(-55.9720320802161,-111.252761985452,
173.157057825983));
#21451=CARTESIAN_POINT('Ctrl Pts',(-57.1270657018158,-111.035346456175,
171.985484999752));
#21452=CARTESIAN_POINT('Ctrl Pts',(-58.7646463259856,-110.766488192578,
171.985485069079));
#21453=CARTESIAN_POINT('Ctrl Pts',(-60.4022269501555,-110.497629928981,
171.985485138407));
#21454=CARTESIAN_POINT('Ctrl Pts',(-61.5572604742632,-110.280214410097,
173.157058062683));
#21455=CARTESIAN_POINT('Ctrl Pts',(-62.712293998371,-110.062798891212,174.328630986959));
#21456=CARTESIAN_POINT('Ctrl Pts',(-62.7023558665168,-109.969577133906,
175.985485236451));
#21457=CARTESIAN_POINT('Ctrl Pts',(-62.6924177346626,-109.8763553766,177.642339485944));
#21458=CARTESIAN_POINT('Ctrl Pts',(-61.517507987229,-109.907327376567,178.813912312176));
#21459=CARTESIAN_POINT('Ctrl Pts',(-60.3425982397954,-109.938299376534,
179.985485138407));
#21460=CARTESIAN_POINT('Ctrl Pts',(-58.6851414897915,-110.02071411082,179.985485069079));
#21461=CARTESIAN_POINT('Ctrl Pts',(-57.0276847397876,-110.103128845106,
179.985484999752));
#21462=CARTESIAN_POINT('Ctrl Pts',(-55.8527750898458,-110.13410083468,178.813912075476));
#21463=CARTESIAN_POINT('Ctrl Pts',(-54.677865439904,-110.165072824253,177.6423391512));
#21464=CARTESIAN_POINT('Ctrl Pts',(-54.6679274459242,-110.071851052249,
175.985484901707));
#21465=CARTESIAN_POINT('Ctrl Pts',(-54.6579894519443,-109.978629280244,
174.328630652215));
#21466=CARTESIAN_POINT('Ctrl Pts',(-55.8130230735439,-109.761213750967,
173.157057825983));
#21467=CARTESIAN_POINT('Ctrl Pts',(-56.9680566951435,-109.543798221689,
171.985484999752));
#21468=CARTESIAN_POINT('Ctrl Pts',(-58.6056373193134,-109.274939958092,
171.985485069079));
#21469=CARTESIAN_POINT('Ctrl Pts',(-60.2432179434833,-109.006081694495,
171.985485138407));
#21470=CARTESIAN_POINT('Ctrl Pts',(-61.398251467591,-108.788666175611,173.157058062683));
#21471=CARTESIAN_POINT('Ctrl Pts',(-62.5532849916988,-108.571250656727,
174.328630986959));
#21472=CARTESIAN_POINT('Ctrl Pts',(-62.5433468598446,-108.478028899421,
175.985485236451));
#21473=CARTESIAN_POINT('Ctrl Pts',(-62.5334087279904,-108.384807142114,
177.642339485944));
#21474=CARTESIAN_POINT('Ctrl Pts',(-61.3584989805568,-108.415779142081,
178.813912312176));
#21475=CARTESIAN_POINT('Ctrl Pts',(-60.1835892331231,-108.446751142048,
179.985485138407));
#21476=CARTESIAN_POINT('Ctrl Pts',(-58.5261324831192,-108.529165876334,
179.985485069079));
#21477=CARTESIAN_POINT('Ctrl Pts',(-56.8686757331153,-108.611580610621,
179.985484999752));
#21478=CARTESIAN_POINT('Ctrl Pts',(-55.6937660831736,-108.642552600194,
178.813912075476));
#21479=CARTESIAN_POINT('Ctrl Pts',(-54.5188564332318,-108.673524589768,
177.6423391512));
#21480=CARTESIAN_POINT('Ctrl Pts',(-54.5089184392519,-108.580302817763,
175.985484901707));
#21481=CARTESIAN_POINT('Ctrl Pts',(-54.4989804452721,-108.487081045759,
174.328630652215));
#21482=CARTESIAN_POINT('Ctrl Pts',(-55.6540140668717,-108.269665516481,
173.157057825983));
#21483=CARTESIAN_POINT('Ctrl Pts',(-56.8090476884713,-108.052249987204,
171.985484999752));
#21484=CARTESIAN_POINT('Ctrl Pts',(-58.4466283126412,-107.783391723607,
171.985485069079));
#21485=CARTESIAN_POINT('Ctrl Pts',(-60.084208936811,-107.51453346001,171.985485138407));
#21486=CARTESIAN_POINT('Ctrl Pts',(-61.2392424609188,-107.297117941125,
173.157058062683));
#21487=CARTESIAN_POINT('Ctrl Pts',(-62.3942759850265,-107.079702422241,
174.328630986959));
#21488=CARTESIAN_POINT('Ctrl Pts',(-62.3843378531723,-106.986480664935,
175.985485236451));
#21489=CARTESIAN_POINT('Ctrl Pts',(-62.3743997213182,-106.893258907629,
177.642339485944));
#21490=CARTESIAN_POINT('Ctrl Pts',(-61.1994899738845,-106.924230907596,
178.813912312176));
#21491=CARTESIAN_POINT('Ctrl Pts',(-60.0245802264509,-106.955202907562,
179.985485138407));
#21492=CARTESIAN_POINT('Ctrl Pts',(-58.367123476447,-107.037617641849,179.985485069079));
#21493=CARTESIAN_POINT('Ctrl Pts',(-56.7096667264431,-107.120032376135,
179.985484999752));
#21494=CARTESIAN_POINT('Ctrl Pts',(-55.5347570765013,-107.151004365708,
178.813912075476));
#21495=CARTESIAN_POINT('Ctrl Pts',(-54.3598474265596,-107.181976355282,
177.6423391512));
#21496=CARTESIAN_POINT('Ctrl Pts',(-54.3499094325797,-107.088754583277,
175.985484901707));
#21497=CARTESIAN_POINT('Ctrl Pts',(-54.3399714385999,-106.995532811273,
174.328630652215));
#21498=CARTESIAN_POINT('Ctrl Pts',(-55.4950050601995,-106.778117281995,
173.157057825983));
#21499=CARTESIAN_POINT('Ctrl Pts',(-56.6500386817991,-106.560701752718,
171.985484999752));
#21500=CARTESIAN_POINT('Ctrl Pts',(-58.2876193059689,-106.291843489121,
171.985485069079));
#21501=CARTESIAN_POINT('Ctrl Pts',(-59.9251999301388,-106.022985225524,
171.985485138407));
#21502=CARTESIAN_POINT('Ctrl Pts',(-61.0802334542465,-105.80556970664,173.157058062683));
#21503=CARTESIAN_POINT('Ctrl Pts',(-62.2352669783543,-105.588154187756,
174.328630986959));
#21504=CARTESIAN_POINT('Ctrl Pts',(-62.2253288465001,-105.494932430449,
175.985485236451));
#21505=CARTESIAN_POINT('Ctrl Pts',(-62.2153907146459,-105.401710673143,
177.642339485944));
#21506=CARTESIAN_POINT('Ctrl Pts',(-61.0404809672123,-105.43268267311,178.813912312176));
#21507=CARTESIAN_POINT('Ctrl Pts',(-59.8655712197787,-105.463654673077,
179.985485138407));
#21508=CARTESIAN_POINT('Ctrl Pts',(-58.2081144697748,-105.546069407363,
179.985485069079));
#21509=CARTESIAN_POINT('Ctrl Pts',(-56.5506577197709,-105.628484141649,
179.985484999752));
#21510=CARTESIAN_POINT('Ctrl Pts',(-55.3757480698291,-105.659456131223,
178.813912075476));
#21511=CARTESIAN_POINT('Ctrl Pts',(-54.2008384198873,-105.690428120796,
177.6423391512));
#21512=CARTESIAN_POINT('Ctrl Pts',(-54.1909004259075,-105.597206348792,
175.985484901707));
#21513=CARTESIAN_POINT('Ctrl Pts',(-54.1809624319276,-105.503984576787,
174.328630652215));
#21514=CARTESIAN_POINT('Ctrl Pts',(-55.3359960535272,-105.28656904751,173.157057825983));
#21515=CARTESIAN_POINT('Ctrl Pts',(-56.4910296751268,-105.069153518232,
171.985484999752));
#21516=CARTESIAN_POINT('Ctrl Pts',(-58.1286102992967,-104.800295254635,
171.985485069079));
#21517=CARTESIAN_POINT('Ctrl Pts',(-59.7661909234666,-104.531436991038,
171.985485138407));
#21518=CARTESIAN_POINT('Ctrl Pts',(-60.9212244475743,-104.314021472154,
173.157058062683));
#21519=CARTESIAN_POINT('Ctrl Pts',(-62.0762579716821,-104.09660595327,174.328630986959));
#21520=CARTESIAN_POINT('Ctrl Pts',(-62.0663198398279,-104.003384195964,
175.985485236451));
#21521=CARTESIAN_POINT('Ctrl Pts',(-62.0563817079737,-103.910162438658,
177.642339485944));
#21522=CARTESIAN_POINT('Ctrl Pts',(-60.8814719605401,-103.941134438624,
178.813912312176));
#21523=CARTESIAN_POINT('Ctrl Pts',(-59.7065622131064,-103.972106438591,
179.985485138407));
#21524=CARTESIAN_POINT('Ctrl Pts',(-58.0491054631025,-104.054521172878,
179.985485069079));
#21525=CARTESIAN_POINT('Ctrl Pts',(-56.3916487130987,-104.136935907164,
179.985484999752));
#21526=CARTESIAN_POINT('Ctrl Pts',(-55.2167390631569,-104.167907896737,
178.813912075476));
#21527=CARTESIAN_POINT('Ctrl Pts',(-54.0418294132151,-104.198879886311,
177.6423391512));
#21528=CARTESIAN_POINT('Ctrl Pts',(-54.0318914192353,-104.105658114306,
175.985484901707));
#21529=CARTESIAN_POINT('Ctrl Pts',(-54.0219534252554,-104.012436342302,
174.328630652215));
#21530=CARTESIAN_POINT('Ctrl Pts',(-55.176987046855,-103.795020813024,173.157057825983));
#21531=CARTESIAN_POINT('Ctrl Pts',(-56.3320206684546,-103.577605283747,
171.985484999752));
#21532=CARTESIAN_POINT('Ctrl Pts',(-57.9696012926245,-103.30874702015,171.985485069079));
#21533=CARTESIAN_POINT('Ctrl Pts',(-59.6071819167943,-103.039888756553,
171.985485138407));
#21534=CARTESIAN_POINT('Ctrl Pts',(-60.7622154409021,-102.822473237669,
173.157058062683));
#21535=CARTESIAN_POINT('Ctrl Pts',(-61.9172489650099,-102.605057718784,
174.328630986959));
#21536=CARTESIAN_POINT('Ctrl Pts',(-61.9073108331557,-102.511835961478,
175.985485236451));
#21537=CARTESIAN_POINT('Ctrl Pts',(-61.8973727013015,-102.418614204172,
177.642339485944));
#21538=CARTESIAN_POINT('Ctrl Pts',(-60.7224629538678,-102.449586204139,
178.813912312176));
#21539=CARTESIAN_POINT('Ctrl Pts',(-59.5475532064342,-102.480558204106,
179.985485138407));
#21540=CARTESIAN_POINT('Ctrl Pts',(-57.8900964564303,-102.562972938392,
179.985485069079));
#21541=CARTESIAN_POINT('Ctrl Pts',(-56.2326397064264,-102.645387672678,
179.985484999752));
#21542=CARTESIAN_POINT('Ctrl Pts',(-55.0577300564847,-102.676359662252,
178.813912075476));
#21543=CARTESIAN_POINT('Ctrl Pts',(-53.8828204065429,-102.707331651825,
177.6423391512));
#21544=CARTESIAN_POINT('Ctrl Pts',(-53.872882412563,-102.614109879821,175.985484901707));
#21545=CARTESIAN_POINT('Ctrl Pts',(-53.8629444185832,-102.520888107816,
174.328630652215));
#21546=CARTESIAN_POINT('Ctrl Pts',(-55.0179780401828,-102.303472578539,
173.157057825983));
#21547=CARTESIAN_POINT('Ctrl Pts',(-56.1730116617824,-102.086057049261,
171.985484999752));
#21548=CARTESIAN_POINT('Ctrl Pts',(-57.8105922859523,-101.817198785664,
171.985485069079));
#21549=CARTESIAN_POINT('Ctrl Pts',(-59.4481729101221,-101.548340522067,
171.985485138407));
#21550=CARTESIAN_POINT('Ctrl Pts',(-60.6032064342299,-101.330925003183,
173.157058062683));
#21551=CARTESIAN_POINT('Ctrl Pts',(-61.7582399583376,-101.113509484299,
174.328630986959));
#21552=CARTESIAN_POINT('Ctrl Pts',(-61.7483018264834,-101.020287726993,
175.985485236451));
#21553=CARTESIAN_POINT('Ctrl Pts',(-61.7383636946293,-100.927065969686,
177.642339485944));
#21554=CARTESIAN_POINT('Ctrl Pts',(-60.5634539471956,-100.958037969653,
178.813912312176));
#21555=CARTESIAN_POINT('Ctrl Pts',(-59.388544199762,-100.98900996962,179.985485138407));
#21556=CARTESIAN_POINT('Ctrl Pts',(-57.7310874497581,-101.071424703906,
179.985485069079));
#21557=CARTESIAN_POINT('Ctrl Pts',(-56.0736306997542,-101.153839438193,
179.985484999752));
#21558=CARTESIAN_POINT('Ctrl Pts',(-54.8987210498124,-101.184811427766,
178.813912075476));
#21559=CARTESIAN_POINT('Ctrl Pts',(-53.7238113998707,-101.21578341734,177.6423391512));
#21560=CARTESIAN_POINT('Ctrl Pts',(-53.7138734058908,-101.122561645335,
175.985484901707));
#21561=CARTESIAN_POINT('Ctrl Pts',(-53.7039354119109,-101.029339873331,
174.328630652215));
#21562=CARTESIAN_POINT('Ctrl Pts',(-54.8589690335105,-100.811924344053,
173.157057825983));
#21563=CARTESIAN_POINT('Ctrl Pts',(-56.0140026551102,-100.594508814776,
171.985484999752));
#21564=CARTESIAN_POINT('Ctrl Pts',(-57.65158327928,-100.325650551179,171.985485069079));
#21565=CARTESIAN_POINT('Ctrl Pts',(-59.2891639034499,-100.056792287582,
171.985485138407));
#21566=CARTESIAN_POINT('Ctrl Pts',(-60.4441974275576,-99.8393767686974,
173.157058062683));
#21567=CARTESIAN_POINT('Ctrl Pts',(-61.5992309516654,-99.6219612498133,
174.328630986959));
#21568=CARTESIAN_POINT('Ctrl Pts',(-61.5892928198112,-99.528739492507,175.985485236451));
#21569=CARTESIAN_POINT('Ctrl Pts',(-61.579354687957,-99.4355177352008,177.642339485944));
#21570=CARTESIAN_POINT('Ctrl Pts',(-60.4044449405234,-99.4664897351676,
178.813912312176));
#21571=CARTESIAN_POINT('Ctrl Pts',(-59.2295351930898,-99.4974617351344,
179.985485138407));
#21572=CARTESIAN_POINT('Ctrl Pts',(-57.5720784430859,-99.5798764694207,
179.985485069079));
#21573=CARTESIAN_POINT('Ctrl Pts',(-55.914621693082,-99.662291203707,179.985484999752));
#21574=CARTESIAN_POINT('Ctrl Pts',(-54.7397120431402,-99.6932631932805,
178.813912075476));
#21575=CARTESIAN_POINT('Ctrl Pts',(-53.5648023931984,-99.724235182854,177.6423391512));
#21576=CARTESIAN_POINT('Ctrl Pts',(-53.5548643992186,-99.6310134108495,
175.985484901707));
#21577=CARTESIAN_POINT('Ctrl Pts',(-53.5449264052387,-99.5377916388449,
174.328630652215));
#21578=CARTESIAN_POINT('Ctrl Pts',(-54.6999600268383,-99.3203761095675,
173.157057825983));
#21579=CARTESIAN_POINT('Ctrl Pts',(-55.8549936484379,-99.10296058029,171.985484999752));
#21580=CARTESIAN_POINT('Ctrl Pts',(-57.4925742726078,-98.834102316693,171.985485069079));
#21581=CARTESIAN_POINT('Ctrl Pts',(-59.1301548967777,-98.5652440530961,
171.985485138407));
#21582=CARTESIAN_POINT('Ctrl Pts',(-60.2851884208854,-98.3478285342118,
173.157058062683));
#21583=CARTESIAN_POINT('Ctrl Pts',(-61.4402219449932,-98.1304130153276,
174.328630986959));
#21584=CARTESIAN_POINT('Ctrl Pts',(-61.430283813139,-98.0371912580215,175.985485236451));
#21585=CARTESIAN_POINT('Ctrl Pts',(-61.4203456812848,-97.9439695007152,
177.642339485944));
#21586=CARTESIAN_POINT('Ctrl Pts',(-60.2454359338512,-97.974941500682,178.813912312176));
#21587=CARTESIAN_POINT('Ctrl Pts',(-59.0705261864175,-98.0059135006488,
179.985485138407));
#21588=CARTESIAN_POINT('Ctrl Pts',(-57.4130694364136,-98.0883282349351,
179.985485069079));
#21589=CARTESIAN_POINT('Ctrl Pts',(-55.3334083509023,-98.1917364932607,
179.985484982092));
#21590=CARTESIAN_POINT('Ctrl Pts',(-54.1340831983237,-98.2115101422526,
178.284125180033));
#21591=CARTESIAN_POINT('Ctrl Pts',(-56.1811453168472,-113.284079398529,
178.821308694947));
#21592=CARTESIAN_POINT('Ctrl Pts',(-55.0031891497056,-113.315376167189,
177.646671990314));
#21593=CARTESIAN_POINT('Ctrl Pts',(-54.993251155906,-113.222154395166,175.98548490127));
#21594=CARTESIAN_POINT('Ctrl Pts',(-54.9833131621064,-113.128932623142,
174.324297812226));
#21595=CARTESIAN_POINT('Ctrl Pts',(-56.1413933011608,-112.91119231475,173.149661205893));
#21596=CARTESIAN_POINT('Ctrl Pts',(-57.2994734402153,-112.693452006359,
171.975024599561));
#21597=CARTESIAN_POINT('Ctrl Pts',(-58.9413624905075,-112.424134435753,
171.97502466907));
#21598=CARTESIAN_POINT('Ctrl Pts',(-60.5832515407998,-112.154816865147,
171.975024738579));
#21599=CARTESIAN_POINT('Ctrl Pts',(-61.7413315821074,-111.937076567176,
173.149661443212));
#21600=CARTESIAN_POINT('Ctrl Pts',(-62.8994116234151,-111.719336269205,
174.324298147845));
#21601=CARTESIAN_POINT('Ctrl Pts',(-62.8894734913806,-111.626114511918,
175.985485236889));
#21602=CARTESIAN_POINT('Ctrl Pts',(-62.8795353593462,-111.532892754631,
177.646672325933));
#21603=CARTESIAN_POINT('Ctrl Pts',(-61.7015790944577,-111.564189533712,
178.821308932265));
#21604=CARTESIAN_POINT('Ctrl Pts',(-60.5236228295692,-111.595486312793,
179.995945538598));
#21605=CARTESIAN_POINT('Ctrl Pts',(-58.8618576534429,-111.678360354088,
179.995945469089));
#21606=CARTESIAN_POINT('Ctrl Pts',(-57.2000924773167,-111.761234395383,
179.99594539958));
#21607=CARTESIAN_POINT('Ctrl Pts',(-56.022136310175,-111.792531164043,178.821308694947));
#21608=CARTESIAN_POINT('Ctrl Pts',(-54.8441801430333,-111.823827932704,
177.646671990314));
#21609=CARTESIAN_POINT('Ctrl Pts',(-54.8342421492337,-111.73060616068,175.98548490127));
#21610=CARTESIAN_POINT('Ctrl Pts',(-54.8243041554342,-111.637384388656,
174.324297812226));
#21611=CARTESIAN_POINT('Ctrl Pts',(-55.9823842944886,-111.419644080265,
173.149661205893));
#21612=CARTESIAN_POINT('Ctrl Pts',(-57.1404644335431,-111.201903771873,
171.975024599561));
#21613=CARTESIAN_POINT('Ctrl Pts',(-58.7823534838353,-110.932586201267,
171.97502466907));
#21614=CARTESIAN_POINT('Ctrl Pts',(-60.4242425341276,-110.663268630661,
171.975024738579));
#21615=CARTESIAN_POINT('Ctrl Pts',(-61.5823225754352,-110.44552833269,173.149661443212));
#21616=CARTESIAN_POINT('Ctrl Pts',(-62.7404026167429,-110.227788034719,
174.324298147845));
#21617=CARTESIAN_POINT('Ctrl Pts',(-62.7304644847084,-110.134566277432,
175.985485236889));
#21618=CARTESIAN_POINT('Ctrl Pts',(-62.720526352674,-110.041344520145,177.646672325933));
#21619=CARTESIAN_POINT('Ctrl Pts',(-61.5425700877854,-110.072641299226,
178.821308932265));
#21620=CARTESIAN_POINT('Ctrl Pts',(-60.364613822897,-110.103938078307,179.995945538598));
#21621=CARTESIAN_POINT('Ctrl Pts',(-58.7028486467707,-110.186812119602,
179.995945469089));
#21622=CARTESIAN_POINT('Ctrl Pts',(-57.0410834706445,-110.269686160897,
179.99594539958));
#21623=CARTESIAN_POINT('Ctrl Pts',(-55.8631273035028,-110.300982929558,
178.821308694947));
#21624=CARTESIAN_POINT('Ctrl Pts',(-54.6851711363611,-110.332279698218,
177.646671990314));
#21625=CARTESIAN_POINT('Ctrl Pts',(-54.6752331425615,-110.239057926194,
175.98548490127));
#21626=CARTESIAN_POINT('Ctrl Pts',(-54.665295148762,-110.145836154171,174.324297812226));
#21627=CARTESIAN_POINT('Ctrl Pts',(-55.8233752878164,-109.928095845779,
173.149661205893));
#21628=CARTESIAN_POINT('Ctrl Pts',(-56.9814554268709,-109.710355537387,
171.975024599561));
#21629=CARTESIAN_POINT('Ctrl Pts',(-58.6233444771631,-109.441037966782,
171.97502466907));
#21630=CARTESIAN_POINT('Ctrl Pts',(-60.2652335274553,-109.171720396176,
171.975024738579));
#21631=CARTESIAN_POINT('Ctrl Pts',(-61.423313568763,-108.953980098205,173.149661443212));
#21632=CARTESIAN_POINT('Ctrl Pts',(-62.5813936100706,-108.736239800234,
174.324298147845));
#21633=CARTESIAN_POINT('Ctrl Pts',(-62.5714554780362,-108.643018042946,
175.985485236889));
#21634=CARTESIAN_POINT('Ctrl Pts',(-62.5615173460017,-108.54979628566,177.646672325933));
#21635=CARTESIAN_POINT('Ctrl Pts',(-61.3835610811132,-108.58109306474,178.821308932265));
#21636=CARTESIAN_POINT('Ctrl Pts',(-60.2056048162248,-108.612389843821,
179.995945538598));
#21637=CARTESIAN_POINT('Ctrl Pts',(-58.5438396400985,-108.695263885116,
179.995945469089));
#21638=CARTESIAN_POINT('Ctrl Pts',(-56.8820744639722,-108.778137926412,
179.99594539958));
#21639=CARTESIAN_POINT('Ctrl Pts',(-55.7041182968305,-108.809434695072,
178.821308694947));
#21640=CARTESIAN_POINT('Ctrl Pts',(-54.5261621296889,-108.840731463732,
177.646671990314));
#21641=CARTESIAN_POINT('Ctrl Pts',(-54.5162241358893,-108.747509691709,
175.98548490127));
#21642=CARTESIAN_POINT('Ctrl Pts',(-54.5062861420897,-108.654287919685,
174.324297812226));
#21643=CARTESIAN_POINT('Ctrl Pts',(-55.6643662811442,-108.436547611293,
173.149661205893));
#21644=CARTESIAN_POINT('Ctrl Pts',(-56.8224464201986,-108.218807302902,
171.975024599561));
#21645=CARTESIAN_POINT('Ctrl Pts',(-58.4643354704908,-107.949489732296,
171.97502466907));
#21646=CARTESIAN_POINT('Ctrl Pts',(-60.1062245207831,-107.68017216169,171.975024738579));
#21647=CARTESIAN_POINT('Ctrl Pts',(-61.2643045620907,-107.462431863719,
173.149661443212));
#21648=CARTESIAN_POINT('Ctrl Pts',(-62.4223846033984,-107.244691565748,
174.324298147845));
#21649=CARTESIAN_POINT('Ctrl Pts',(-62.4124464713639,-107.151469808461,
175.985485236889));
#21650=CARTESIAN_POINT('Ctrl Pts',(-62.4025083393295,-107.058248051174,
177.646672325933));
#21651=CARTESIAN_POINT('Ctrl Pts',(-61.224552074441,-107.089544830255,178.821308932265));
#21652=CARTESIAN_POINT('Ctrl Pts',(-60.0465958095525,-107.120841609336,
179.995945538598));
#21653=CARTESIAN_POINT('Ctrl Pts',(-58.3848306334262,-107.203715650631,
179.995945469089));
#21654=CARTESIAN_POINT('Ctrl Pts',(-56.7230654573,-107.286589691926,179.99594539958));
#21655=CARTESIAN_POINT('Ctrl Pts',(-55.5451092901583,-107.317886460586,
178.821308694947));
#21656=CARTESIAN_POINT('Ctrl Pts',(-54.3671531230166,-107.349183229247,
177.646671990314));
#21657=CARTESIAN_POINT('Ctrl Pts',(-54.357215129217,-107.255961457223,175.98548490127));
#21658=CARTESIAN_POINT('Ctrl Pts',(-54.3472771354175,-107.162739685199,
174.324297812226));
#21659=CARTESIAN_POINT('Ctrl Pts',(-55.5053572744719,-106.944999376808,
173.149661205893));
#21660=CARTESIAN_POINT('Ctrl Pts',(-56.6634374135264,-106.727259068416,
171.975024599561));
#21661=CARTESIAN_POINT('Ctrl Pts',(-58.3053264638186,-106.45794149781,171.97502466907));
#21662=CARTESIAN_POINT('Ctrl Pts',(-59.9472155141109,-106.188623927205,
171.975024738579));
#21663=CARTESIAN_POINT('Ctrl Pts',(-61.1052955554185,-105.970883629233,
173.149661443212));
#21664=CARTESIAN_POINT('Ctrl Pts',(-62.2633755967262,-105.753143331262,
174.324298147845));
#21665=CARTESIAN_POINT('Ctrl Pts',(-62.2534374646917,-105.659921573975,
175.985485236889));
#21666=CARTESIAN_POINT('Ctrl Pts',(-62.2434993326573,-105.566699816688,
177.646672325933));
#21667=CARTESIAN_POINT('Ctrl Pts',(-61.0655430677688,-105.597996595769,
178.821308932265));
#21668=CARTESIAN_POINT('Ctrl Pts',(-59.8875868028803,-105.62929337485,179.995945538598));
#21669=CARTESIAN_POINT('Ctrl Pts',(-58.225821626754,-105.712167416145,179.995945469089));
#21670=CARTESIAN_POINT('Ctrl Pts',(-56.5640564506278,-105.79504145744,179.99594539958));
#21671=CARTESIAN_POINT('Ctrl Pts',(-55.3861002834861,-105.826338226101,
178.821308694947));
#21672=CARTESIAN_POINT('Ctrl Pts',(-54.2081441163444,-105.857634994761,
177.646671990314));
#21673=CARTESIAN_POINT('Ctrl Pts',(-54.1982061225448,-105.764413222738,
175.98548490127));
#21674=CARTESIAN_POINT('Ctrl Pts',(-54.1882681287453,-105.671191450714,
174.324297812226));
#21675=CARTESIAN_POINT('Ctrl Pts',(-55.3463482677997,-105.453451142322,
173.149661205893));
#21676=CARTESIAN_POINT('Ctrl Pts',(-56.5044284068542,-105.235710833931,
171.975024599561));
#21677=CARTESIAN_POINT('Ctrl Pts',(-58.1463174571464,-104.966393263325,
171.97502466907));
#21678=CARTESIAN_POINT('Ctrl Pts',(-59.7882065074387,-104.697075692719,
171.975024738579));
#21679=CARTESIAN_POINT('Ctrl Pts',(-60.9462865487463,-104.479335394748,
173.149661443212));
#21680=CARTESIAN_POINT('Ctrl Pts',(-62.104366590054,-104.261595096777,174.324298147845));
#21681=CARTESIAN_POINT('Ctrl Pts',(-62.0944284580195,-104.16837333949,175.985485236889));
#21682=CARTESIAN_POINT('Ctrl Pts',(-62.0844903259851,-104.075151582203,
177.646672325933));
#21683=CARTESIAN_POINT('Ctrl Pts',(-60.9065340610965,-104.106448361284,
178.821308932265));
#21684=CARTESIAN_POINT('Ctrl Pts',(-59.7285777962081,-104.137745140365,
179.995945538598));
#21685=CARTESIAN_POINT('Ctrl Pts',(-58.0668126200818,-104.22061918166,179.995945469089));
#21686=CARTESIAN_POINT('Ctrl Pts',(-56.4050474439555,-104.303493222955,
179.99594539958));
#21687=CARTESIAN_POINT('Ctrl Pts',(-55.2270912768138,-104.334789991615,
178.821308694947));
#21688=CARTESIAN_POINT('Ctrl Pts',(-54.0491351096722,-104.366086760276,
177.646671990314));
#21689=CARTESIAN_POINT('Ctrl Pts',(-54.0391971158726,-104.272864988252,
175.98548490127));
#21690=CARTESIAN_POINT('Ctrl Pts',(-54.029259122073,-104.179643216228,174.324297812226));
#21691=CARTESIAN_POINT('Ctrl Pts',(-55.1873392611275,-103.961902907837,
173.149661205893));
#21692=CARTESIAN_POINT('Ctrl Pts',(-56.3454194001819,-103.744162599445,
171.975024599561));
#21693=CARTESIAN_POINT('Ctrl Pts',(-57.9873084504742,-103.474845028839,
171.97502466907));
#21694=CARTESIAN_POINT('Ctrl Pts',(-59.6291975007664,-103.205527458233,
171.975024738579));
#21695=CARTESIAN_POINT('Ctrl Pts',(-60.7872775420741,-102.987787160262,
173.149661443212));
#21696=CARTESIAN_POINT('Ctrl Pts',(-61.9453575833817,-102.770046862291,
174.324298147845));
#21697=CARTESIAN_POINT('Ctrl Pts',(-61.9354194513472,-102.676825105004,
175.985485236889));
#21698=CARTESIAN_POINT('Ctrl Pts',(-61.9254813193128,-102.583603347717,
177.646672325933));
#21699=CARTESIAN_POINT('Ctrl Pts',(-60.7475250544243,-102.614900126798,
178.821308932265));
#21700=CARTESIAN_POINT('Ctrl Pts',(-59.5695687895358,-102.646196905879,
179.995945538598));
#21701=CARTESIAN_POINT('Ctrl Pts',(-57.9078036134095,-102.729070947174,
179.995945469089));
#21702=CARTESIAN_POINT('Ctrl Pts',(-56.2460384372833,-102.811944988469,
179.99594539958));
#21703=CARTESIAN_POINT('Ctrl Pts',(-55.0680822701416,-102.84324175713,178.821308694947));
#21704=CARTESIAN_POINT('Ctrl Pts',(-53.890126103,-102.87453852579,177.646671990314));
#21705=CARTESIAN_POINT('Ctrl Pts',(-53.8801881092004,-102.781316753766,
175.98548490127));
#21706=CARTESIAN_POINT('Ctrl Pts',(-53.8702501154008,-102.688094981743,
174.324297812226));
#21707=CARTESIAN_POINT('Ctrl Pts',(-55.0283302544552,-102.470354673351,
173.149661205893));
#21708=CARTESIAN_POINT('Ctrl Pts',(-56.1864103935097,-102.252614364959,
171.975024599561));
#21709=CARTESIAN_POINT('Ctrl Pts',(-57.8282994438019,-101.983296794354,
171.97502466907));
#21710=CARTESIAN_POINT('Ctrl Pts',(-59.4701884940942,-101.713979223748,
171.975024738579));
#21711=CARTESIAN_POINT('Ctrl Pts',(-60.6282685354018,-101.496238925777,
173.149661443212));
#21712=CARTESIAN_POINT('Ctrl Pts',(-61.7863485767095,-101.278498627806,
174.324298147845));
#21713=CARTESIAN_POINT('Ctrl Pts',(-61.776410444675,-101.185276870519,175.985485236889));
#21714=CARTESIAN_POINT('Ctrl Pts',(-61.7664723126406,-101.092055113232,
177.646672325933));
#21715=CARTESIAN_POINT('Ctrl Pts',(-60.5885160477521,-101.123351892312,
178.821308932265));
#21716=CARTESIAN_POINT('Ctrl Pts',(-59.4105597828636,-101.154648671393,
179.995945538598));
#21717=CARTESIAN_POINT('Ctrl Pts',(-57.7487946067373,-101.237522712688,
179.995945469089));
#21718=CARTESIAN_POINT('Ctrl Pts',(-56.0870294306111,-101.320396753984,
179.99594539958));
#21719=CARTESIAN_POINT('Ctrl Pts',(-54.9090732634694,-101.351693522644,
178.821308694947));
#21720=CARTESIAN_POINT('Ctrl Pts',(-53.7311170963277,-101.382990291305,
177.646671990314));
#21721=CARTESIAN_POINT('Ctrl Pts',(-53.7211791025281,-101.289768519281,
175.98548490127));
#21722=CARTESIAN_POINT('Ctrl Pts',(-53.7112411087286,-101.196546747257,
174.324297812226));
#21723=CARTESIAN_POINT('Ctrl Pts',(-54.869321247783,-100.978806438865,173.149661205893));
#21724=CARTESIAN_POINT('Ctrl Pts',(-56.0274013868375,-100.761066130474,
171.975024599561));
#21725=CARTESIAN_POINT('Ctrl Pts',(-57.6692904371297,-100.491748559868,
171.97502466907));
#21726=CARTESIAN_POINT('Ctrl Pts',(-59.311179487422,-100.222430989262,171.975024738579));
#21727=CARTESIAN_POINT('Ctrl Pts',(-60.4692595287296,-100.004690691291,
173.149661443212));
#21728=CARTESIAN_POINT('Ctrl Pts',(-61.6273395700373,-99.7869503933199,
174.324298147845));
#21729=CARTESIAN_POINT('Ctrl Pts',(-61.6174014380028,-99.6937286360329,
175.985485236889));
#21730=CARTESIAN_POINT('Ctrl Pts',(-61.6074633059684,-99.6005068787459,
177.646672325933));
#21731=CARTESIAN_POINT('Ctrl Pts',(-60.4295070410798,-99.6318036578269,
178.821308932265));
#21732=CARTESIAN_POINT('Ctrl Pts',(-59.2515507761914,-99.6631004369078,
179.995945538598));
#21733=CARTESIAN_POINT('Ctrl Pts',(-57.5897856000651,-99.7459744782029,
179.995945469089));
#21734=CARTESIAN_POINT('Ctrl Pts',(-55.9280204239389,-99.828848519498,179.99594539958));
#21735=CARTESIAN_POINT('Ctrl Pts',(-54.7500642567972,-99.8601452881584,
178.821308694947));
#21736=CARTESIAN_POINT('Ctrl Pts',(-53.5721080896555,-99.8914420568189,
177.646671990314));
#21737=CARTESIAN_POINT('Ctrl Pts',(-53.5621700958559,-99.7982202847951,
175.98548490127));
#21738=CARTESIAN_POINT('Ctrl Pts',(-53.5522321020564,-99.7049985127714,
174.324297812226));
#21739=CARTESIAN_POINT('Ctrl Pts',(-54.7103122411108,-99.4872582043798,
173.149661205893));
#21740=CARTESIAN_POINT('Ctrl Pts',(-55.8683923801653,-99.2695178959882,
171.975024599561));
#21741=CARTESIAN_POINT('Ctrl Pts',(-57.5102814304575,-99.0002003253824,
171.97502466907));
#21742=CARTESIAN_POINT('Ctrl Pts',(-59.1521704807498,-98.7308827547766,
171.975024738579));
#21743=CARTESIAN_POINT('Ctrl Pts',(-60.3102505220574,-98.5131424568055,
173.149661443212));
#21744=CARTESIAN_POINT('Ctrl Pts',(-61.468330563365,-98.2954021588343,174.324298147845));
#21745=CARTESIAN_POINT('Ctrl Pts',(-61.4583924313306,-98.2021804015473,
175.985485236889));
#21746=CARTESIAN_POINT('Ctrl Pts',(-61.4484542992961,-98.1089586442604,
177.646672325933));
#21747=CARTESIAN_POINT('Ctrl Pts',(-60.2704980344076,-98.1402554233413,
178.821308932265));
#21748=CARTESIAN_POINT('Ctrl Pts',(-59.0925417695192,-98.1715522024222,
179.995945538598));
#21749=CARTESIAN_POINT('Ctrl Pts',(-57.4307765933929,-98.2544262437173,
179.995945469089));
#21750=CARTESIAN_POINT('Ctrl Pts',(-55.3457095953916,-98.3584108084307,
179.995945381874));
#21751=CARTESIAN_POINT('Ctrl Pts',(-54.1432778809914,-98.3785156376673,
178.290136353792));
#21752=CARTESIAN_POINT('Ctrl Pts',(-56.1989083789663,-113.450500188295,
178.821287321967));
#21753=CARTESIAN_POINT('Ctrl Pts',(-55.0209610149206,-113.481796018486,
177.646659470313));
#21754=CARTESIAN_POINT('Ctrl Pts',(-55.0110230211205,-113.388574246463,
175.985484901271));
#21755=CARTESIAN_POINT('Ctrl Pts',(-55.0010850273204,-113.295352474439,
174.324310332229));
#21756=CARTESIAN_POINT('Ctrl Pts',(-56.1591563632782,-113.077613104516,
173.149682578875));
#21757=CARTESIAN_POINT('Ctrl Pts',(-57.317227699236,-112.859873734594,171.975054825521));
#21758=CARTESIAN_POINT('Ctrl Pts',(-58.95910430007,-112.590557491183,171.97505489503));
#21759=CARTESIAN_POINT('Ctrl Pts',(-60.600980900904,-112.321241247773,171.975054964538));
#21760=CARTESIAN_POINT('Ctrl Pts',(-61.7590521391157,-112.103501888271,
173.149682816192));
#21761=CARTESIAN_POINT('Ctrl Pts',(-62.9171233773274,-111.885762528768,
174.324310667846));
#21762=CARTESIAN_POINT('Ctrl Pts',(-62.9071852452935,-111.792540771481,
175.985485236888));
#21763=CARTESIAN_POINT('Ctrl Pts',(-62.8972471132596,-111.699319014194,
177.64665980593));
#21764=CARTESIAN_POINT('Ctrl Pts',(-61.7192996514678,-111.730614854806,
178.821287559284));
#21765=CARTESIAN_POINT('Ctrl Pts',(-60.541352189676,-111.761910695418,179.995915312638));
#21766=CARTESIAN_POINT('Ctrl Pts',(-58.8795994630079,-111.844783409518,
179.995915243129));
#21767=CARTESIAN_POINT('Ctrl Pts',(-57.2178467363399,-111.927656123618,
179.995915173621));
#21768=CARTESIAN_POINT('Ctrl Pts',(-56.0398993722941,-111.958951953809,
178.821287321967));
#21769=CARTESIAN_POINT('Ctrl Pts',(-54.8619520082484,-111.990247784001,
177.646659470313));
#21770=CARTESIAN_POINT('Ctrl Pts',(-54.8520140144483,-111.897026011977,
175.985484901271));
#21771=CARTESIAN_POINT('Ctrl Pts',(-54.8420760206482,-111.803804239954,
174.324310332229));
#21772=CARTESIAN_POINT('Ctrl Pts',(-56.000147356606,-111.586064870031,173.149682578875));
#21773=CARTESIAN_POINT('Ctrl Pts',(-57.1582186925638,-111.368325500108,
171.975054825521));
#21774=CARTESIAN_POINT('Ctrl Pts',(-58.8000952933978,-111.099009256698,
171.97505489503));
#21775=CARTESIAN_POINT('Ctrl Pts',(-60.4419718942318,-110.829693013287,
171.975054964538));
#21776=CARTESIAN_POINT('Ctrl Pts',(-61.6000431324435,-110.611953653785,
173.149682816192));
#21777=CARTESIAN_POINT('Ctrl Pts',(-62.7581143706552,-110.394214294283,
174.324310667846));
#21778=CARTESIAN_POINT('Ctrl Pts',(-62.7481762386213,-110.300992536996,
175.985485236888));
#21779=CARTESIAN_POINT('Ctrl Pts',(-62.7382381065874,-110.207770779709,
177.64665980593));
#21780=CARTESIAN_POINT('Ctrl Pts',(-61.5602906447956,-110.239066620321,
178.821287559284));
#21781=CARTESIAN_POINT('Ctrl Pts',(-60.3823431830037,-110.270362460933,
179.995915312638));
#21782=CARTESIAN_POINT('Ctrl Pts',(-58.7205904563357,-110.353235175032,
179.995915243129));
#21783=CARTESIAN_POINT('Ctrl Pts',(-57.0588377296676,-110.436107889132,
179.995915173621));
#21784=CARTESIAN_POINT('Ctrl Pts',(-55.8808903656219,-110.467403719324,
178.821287321967));
#21785=CARTESIAN_POINT('Ctrl Pts',(-54.7029430015762,-110.498699549515,
177.646659470313));
#21786=CARTESIAN_POINT('Ctrl Pts',(-54.6930050077761,-110.405477777492,
175.985484901271));
#21787=CARTESIAN_POINT('Ctrl Pts',(-54.683067013976,-110.312256005468,174.324310332229));
#21788=CARTESIAN_POINT('Ctrl Pts',(-55.8411383499337,-110.094516635545,
173.149682578875));
#21789=CARTESIAN_POINT('Ctrl Pts',(-56.9992096858915,-109.876777265623,
171.975054825521));
#21790=CARTESIAN_POINT('Ctrl Pts',(-58.6410862867255,-109.607461022212,
171.97505489503));
#21791=CARTESIAN_POINT('Ctrl Pts',(-60.2829628875596,-109.338144778802,
171.975054964538));
#21792=CARTESIAN_POINT('Ctrl Pts',(-61.4410341257713,-109.120405419299,
173.149682816192));
#21793=CARTESIAN_POINT('Ctrl Pts',(-62.599105363983,-108.902666059797,174.324310667846));
#21794=CARTESIAN_POINT('Ctrl Pts',(-62.589167231949,-108.80944430251,175.985485236888));
#21795=CARTESIAN_POINT('Ctrl Pts',(-62.5792290999151,-108.716222545223,
177.64665980593));
#21796=CARTESIAN_POINT('Ctrl Pts',(-61.4012816381233,-108.747518385835,
178.821287559284));
#21797=CARTESIAN_POINT('Ctrl Pts',(-60.2233341763315,-108.778814226447,
179.995915312638));
#21798=CARTESIAN_POINT('Ctrl Pts',(-58.5615814496634,-108.861686940547,
179.995915243129));
#21799=CARTESIAN_POINT('Ctrl Pts',(-56.8998287229954,-108.944559654646,
179.995915173621));
#21800=CARTESIAN_POINT('Ctrl Pts',(-55.7218813589497,-108.975855484838,
178.821287321967));
#21801=CARTESIAN_POINT('Ctrl Pts',(-54.543933994904,-109.00715131503,177.646659470313));
#21802=CARTESIAN_POINT('Ctrl Pts',(-54.5339960011038,-108.913929543006,
175.985484901271));
#21803=CARTESIAN_POINT('Ctrl Pts',(-54.5240580073037,-108.820707770982,
174.324310332229));
#21804=CARTESIAN_POINT('Ctrl Pts',(-55.6821293432615,-108.60296840106,173.149682578875));
#21805=CARTESIAN_POINT('Ctrl Pts',(-56.8402006792193,-108.385229031137,
171.975054825521));
#21806=CARTESIAN_POINT('Ctrl Pts',(-58.4820772800533,-108.115912787727,
171.97505489503));
#21807=CARTESIAN_POINT('Ctrl Pts',(-60.1239538808874,-107.846596544316,
171.975054964538));
#21808=CARTESIAN_POINT('Ctrl Pts',(-61.2820251190991,-107.628857184814,
173.149682816192));
#21809=CARTESIAN_POINT('Ctrl Pts',(-62.4400963573108,-107.411117825312,
174.324310667846));
#21810=CARTESIAN_POINT('Ctrl Pts',(-62.4301582252768,-107.317896068025,
175.985485236888));
#21811=CARTESIAN_POINT('Ctrl Pts',(-62.4202200932429,-107.224674310738,
177.64665980593));
#21812=CARTESIAN_POINT('Ctrl Pts',(-61.2422726314511,-107.25597015135,178.821287559284));
#21813=CARTESIAN_POINT('Ctrl Pts',(-60.0643251696593,-107.287265991962,
179.995915312638));
#21814=CARTESIAN_POINT('Ctrl Pts',(-58.4025724429912,-107.370138706061,
179.995915243129));
#21815=CARTESIAN_POINT('Ctrl Pts',(-56.7408197163232,-107.453011420161,
179.995915173621));
#21816=CARTESIAN_POINT('Ctrl Pts',(-55.5628723522774,-107.484307250352,
178.821287321967));
#21817=CARTESIAN_POINT('Ctrl Pts',(-54.3849249882317,-107.515603080544,
177.646659470313));
#21818=CARTESIAN_POINT('Ctrl Pts',(-54.3749869944316,-107.42238130852,175.985484901271));
#21819=CARTESIAN_POINT('Ctrl Pts',(-54.3650490006315,-107.329159536497,
174.324310332229));
#21820=CARTESIAN_POINT('Ctrl Pts',(-55.5231203365893,-107.111420166574,
173.149682578875));
#21821=CARTESIAN_POINT('Ctrl Pts',(-56.6811916725471,-106.893680796651,
171.975054825521));
#21822=CARTESIAN_POINT('Ctrl Pts',(-58.3230682733811,-106.624364553241,
171.97505489503));
#21823=CARTESIAN_POINT('Ctrl Pts',(-59.9649448742151,-106.355048309831,
171.975054964538));
#21824=CARTESIAN_POINT('Ctrl Pts',(-61.1230161124268,-106.137308950328,
173.149682816192));
#21825=CARTESIAN_POINT('Ctrl Pts',(-62.2810873506385,-105.919569590826,
174.324310667846));
#21826=CARTESIAN_POINT('Ctrl Pts',(-62.2711492186046,-105.826347833539,
175.985485236888));
#21827=CARTESIAN_POINT('Ctrl Pts',(-62.2612110865707,-105.733126076252,
177.64665980593));
#21828=CARTESIAN_POINT('Ctrl Pts',(-61.0832636247789,-105.764421916864,
178.821287559284));
#21829=CARTESIAN_POINT('Ctrl Pts',(-59.9053161629871,-105.795717757476,
179.995915312638));
#21830=CARTESIAN_POINT('Ctrl Pts',(-58.243563436319,-105.878590471576,179.995915243129));
#21831=CARTESIAN_POINT('Ctrl Pts',(-56.5818107096509,-105.961463185675,
179.995915173621));
#21832=CARTESIAN_POINT('Ctrl Pts',(-55.4038633456052,-105.992759015867,
178.821287321967));
#21833=CARTESIAN_POINT('Ctrl Pts',(-54.2259159815595,-106.024054846058,
177.646659470313));
#21834=CARTESIAN_POINT('Ctrl Pts',(-54.2159779877594,-105.930833074035,
175.985484901271));
#21835=CARTESIAN_POINT('Ctrl Pts',(-54.2060399939593,-105.837611302011,
174.324310332229));
#21836=CARTESIAN_POINT('Ctrl Pts',(-55.364111329917,-105.619871932088,173.149682578875));
#21837=CARTESIAN_POINT('Ctrl Pts',(-56.5221826658748,-105.402132562166,
171.975054825521));
#21838=CARTESIAN_POINT('Ctrl Pts',(-58.1640592667089,-105.132816318755,
171.97505489503));
#21839=CARTESIAN_POINT('Ctrl Pts',(-59.8059358675429,-104.863500075345,
171.975054964538));
#21840=CARTESIAN_POINT('Ctrl Pts',(-60.9640071057546,-104.645760715843,
173.149682816192));
#21841=CARTESIAN_POINT('Ctrl Pts',(-62.1220783439663,-104.42802135634,174.324310667846));
#21842=CARTESIAN_POINT('Ctrl Pts',(-62.1121402119324,-104.334799599053,
175.985485236888));
#21843=CARTESIAN_POINT('Ctrl Pts',(-62.1022020798985,-104.241577841766,
177.64665980593));
#21844=CARTESIAN_POINT('Ctrl Pts',(-60.9242546181066,-104.272873682378,
178.821287559284));
#21845=CARTESIAN_POINT('Ctrl Pts',(-59.7463071563148,-104.30416952299,179.995915312638));
#21846=CARTESIAN_POINT('Ctrl Pts',(-58.0845544296468,-104.38704223709,179.995915243129));
#21847=CARTESIAN_POINT('Ctrl Pts',(-56.4228017029787,-104.46991495119,179.995915173621));
#21848=CARTESIAN_POINT('Ctrl Pts',(-55.244854338933,-104.501210781381,178.821287321967));
#21849=CARTESIAN_POINT('Ctrl Pts',(-54.0669069748872,-104.532506611573,
177.646659470313));
#21850=CARTESIAN_POINT('Ctrl Pts',(-54.0569689810871,-104.439284839549,
175.985484901271));
#21851=CARTESIAN_POINT('Ctrl Pts',(-54.0470309872871,-104.346063067526,
174.324310332229));
#21852=CARTESIAN_POINT('Ctrl Pts',(-55.2051023232448,-104.128323697603,
173.149682578875));
#21853=CARTESIAN_POINT('Ctrl Pts',(-56.3631736592026,-103.91058432768,171.975054825521));
#21854=CARTESIAN_POINT('Ctrl Pts',(-58.0050502600366,-103.64126808427,171.97505489503));
#21855=CARTESIAN_POINT('Ctrl Pts',(-59.6469268608707,-103.371951840859,
171.975054964538));
#21856=CARTESIAN_POINT('Ctrl Pts',(-60.8049980990824,-103.154212481357,
173.149682816192));
#21857=CARTESIAN_POINT('Ctrl Pts',(-61.9630693372941,-102.936473121855,
174.324310667846));
#21858=CARTESIAN_POINT('Ctrl Pts',(-61.9531312052601,-102.843251364568,
175.985485236888));
#21859=CARTESIAN_POINT('Ctrl Pts',(-61.9431930732262,-102.750029607281,
177.64665980593));
#21860=CARTESIAN_POINT('Ctrl Pts',(-60.7652456114344,-102.781325447893,
178.821287559284));
#21861=CARTESIAN_POINT('Ctrl Pts',(-59.5872981496426,-102.812621288505,
179.995915312638));
#21862=CARTESIAN_POINT('Ctrl Pts',(-57.9255454229745,-102.895494002604,
179.995915243129));
#21863=CARTESIAN_POINT('Ctrl Pts',(-56.2637926963065,-102.978366716704,
179.995915173621));
#21864=CARTESIAN_POINT('Ctrl Pts',(-55.0858453322607,-103.009662546896,
178.821287321967));
#21865=CARTESIAN_POINT('Ctrl Pts',(-53.907897968215,-103.040958377087,177.646659470313));
#21866=CARTESIAN_POINT('Ctrl Pts',(-53.8979599744149,-102.947736605064,
175.985484901271));
#21867=CARTESIAN_POINT('Ctrl Pts',(-53.8880219806148,-102.85451483304,174.324310332229));
#21868=CARTESIAN_POINT('Ctrl Pts',(-55.0460933165726,-102.636775463117,
173.149682578875));
#21869=CARTESIAN_POINT('Ctrl Pts',(-56.2041646525304,-102.419036093195,
171.975054825521));
#21870=CARTESIAN_POINT('Ctrl Pts',(-57.8460412533644,-102.149719849784,
171.97505489503));
#21871=CARTESIAN_POINT('Ctrl Pts',(-59.4879178541985,-101.880403606374,
171.975054964538));
#21872=CARTESIAN_POINT('Ctrl Pts',(-60.6459890924101,-101.662664246871,
173.149682816192));
#21873=CARTESIAN_POINT('Ctrl Pts',(-61.8040603306218,-101.444924887369,
174.324310667846));
#21874=CARTESIAN_POINT('Ctrl Pts',(-61.7941221985879,-101.351703130082,
175.985485236888));
#21875=CARTESIAN_POINT('Ctrl Pts',(-61.784184066554,-101.258481372795,177.64665980593));
#21876=CARTESIAN_POINT('Ctrl Pts',(-60.6062366047622,-101.289777213407,
178.821287559284));
#21877=CARTESIAN_POINT('Ctrl Pts',(-59.4282891429704,-101.321073054019,
179.995915312638));
#21878=CARTESIAN_POINT('Ctrl Pts',(-57.7665364163023,-101.403945768119,
179.995915243129));
#21879=CARTESIAN_POINT('Ctrl Pts',(-56.1047836896342,-101.486818482218,
179.995915173621));
#21880=CARTESIAN_POINT('Ctrl Pts',(-54.9268363255885,-101.51811431241,178.821287321967));
#21881=CARTESIAN_POINT('Ctrl Pts',(-53.7488889615428,-101.549410142602,
177.646659470313));
#21882=CARTESIAN_POINT('Ctrl Pts',(-53.7389509677427,-101.456188370578,
175.985484901271));
#21883=CARTESIAN_POINT('Ctrl Pts',(-53.7290129739426,-101.362966598554,
174.324310332229));
#21884=CARTESIAN_POINT('Ctrl Pts',(-54.8870843099004,-101.145227228632,
173.149682578875));
#21885=CARTESIAN_POINT('Ctrl Pts',(-56.0451556458581,-100.927487858709,
171.975054825521));
#21886=CARTESIAN_POINT('Ctrl Pts',(-57.6870322466922,-100.658171615299,
171.97505489503));
#21887=CARTESIAN_POINT('Ctrl Pts',(-59.3289088475262,-100.388855371888,
171.975054964538));
#21888=CARTESIAN_POINT('Ctrl Pts',(-60.4869800857379,-100.171116012386,
173.149682816192));
#21889=CARTESIAN_POINT('Ctrl Pts',(-61.6450513239496,-99.9533766528836,
174.324310667846));
#21890=CARTESIAN_POINT('Ctrl Pts',(-61.6351131919157,-99.8601548955965,
175.985485236888));
#21891=CARTESIAN_POINT('Ctrl Pts',(-61.6251750598818,-99.7669331383095,
177.64665980593));
#21892=CARTESIAN_POINT('Ctrl Pts',(-60.44722759809,-99.7982289789215,178.821287559284));
#21893=CARTESIAN_POINT('Ctrl Pts',(-59.2692801362982,-99.8295248195335,
179.995915312638));
#21894=CARTESIAN_POINT('Ctrl Pts',(-57.6075274096301,-99.9123975336331,
179.995915243129));
#21895=CARTESIAN_POINT('Ctrl Pts',(-55.945774682962,-99.9952702477328,179.995915173621));
#21896=CARTESIAN_POINT('Ctrl Pts',(-54.7678273189163,-100.026566077924,
178.821287321967));
#21897=CARTESIAN_POINT('Ctrl Pts',(-53.5898799548706,-100.057861908116,
177.646659470313));
#21898=CARTESIAN_POINT('Ctrl Pts',(-53.5799419610705,-99.9646401360924,
175.985484901271));
#21899=CARTESIAN_POINT('Ctrl Pts',(-53.5700039672704,-99.8714183640688,
174.324310332229));
#21900=CARTESIAN_POINT('Ctrl Pts',(-54.7280753032281,-99.653678994146,173.149682578875));
#21901=CARTESIAN_POINT('Ctrl Pts',(-55.8861466391859,-99.4359396242233,
171.975054825521));
#21902=CARTESIAN_POINT('Ctrl Pts',(-57.5280232400199,-99.1666233808129,
171.97505489503));
#21903=CARTESIAN_POINT('Ctrl Pts',(-59.169899840854,-98.8973071374026,171.975054964538));
#21904=CARTESIAN_POINT('Ctrl Pts',(-60.3279710790657,-98.6795677779003,
173.149682816192));
#21905=CARTESIAN_POINT('Ctrl Pts',(-61.4860423172774,-98.461828418398,174.324310667846));
#21906=CARTESIAN_POINT('Ctrl Pts',(-61.4761041852435,-98.3686066611109,
175.985485236888));
#21907=CARTESIAN_POINT('Ctrl Pts',(-61.4661660532095,-98.2753849038239,
177.64665980593));
#21908=CARTESIAN_POINT('Ctrl Pts',(-60.2882185914177,-98.3066807444359,
178.821287559284));
#21909=CARTESIAN_POINT('Ctrl Pts',(-59.1102711296259,-98.3379765850479,
179.995915312638));
#21910=CARTESIAN_POINT('Ctrl Pts',(-57.4485184029579,-98.4208492991475,
179.995915243129));
#21911=CARTESIAN_POINT('Ctrl Pts',(-55.363467025668,-98.5248321985888,179.995915155915));
#21912=CARTESIAN_POINT('Ctrl Pts',(-54.1610442878665,-98.5449360708601,
178.290118984142));
#21913=CARTESIAN_POINT('Ctrl Pts',(-56.2240123501782,-113.615805207186,
178.813848124531));
#21914=CARTESIAN_POINT('Ctrl Pts',(-55.0491290403307,-113.646774388729,
177.642301689606));
#21915=CARTESIAN_POINT('Ctrl Pts',(-55.0391910463492,-113.553552616725,
175.985484901711));
#21916=CARTESIAN_POINT('Ctrl Pts',(-55.0292530523678,-113.46033084472,174.328668113817));
#21917=CARTESIAN_POINT('Ctrl Pts',(-56.184260333871,-113.242918123473,173.157121776934));
#21918=CARTESIAN_POINT('Ctrl Pts',(-57.3392676153741,-113.025505402226,
171.985575440051));
#21919=CARTESIAN_POINT('Ctrl Pts',(-58.976810989024,-112.756651109783,171.985575509377));
#21920=CARTESIAN_POINT('Ctrl Pts',(-60.6143543626737,-112.487796817341,
171.985575578703));
#21921=CARTESIAN_POINT('Ctrl Pts',(-61.7693615466873,-112.270384106486,
173.157122013628));
#21922=CARTESIAN_POINT('Ctrl Pts',(-62.9243687307007,-112.052971395632,
174.328668448553));
#21923=CARTESIAN_POINT('Ctrl Pts',(-62.9144305988482,-111.959749638326,
175.985485236448));
#21924=CARTESIAN_POINT('Ctrl Pts',(-62.9044924669955,-111.86652788102,177.642302024342));
#21925=CARTESIAN_POINT('Ctrl Pts',(-61.7296090596583,-111.897497072956,
178.813848361225));
#21926=CARTESIAN_POINT('Ctrl Pts',(-60.5547256523212,-111.928466264893,
179.985394698108));
#21927=CARTESIAN_POINT('Ctrl Pts',(-58.8973061528373,-112.010877028025,
179.985394628782));
#21928=CARTESIAN_POINT('Ctrl Pts',(-57.2398866533535,-112.093287791156,
179.985394559456));
#21929=CARTESIAN_POINT('Ctrl Pts',(-56.0650033435059,-112.1242569727,178.813848124531));
#21930=CARTESIAN_POINT('Ctrl Pts',(-54.8901200336584,-112.155226154243,
177.642301689606));
#21931=CARTESIAN_POINT('Ctrl Pts',(-54.880182039677,-112.062004382239,175.985484901711));
#21932=CARTESIAN_POINT('Ctrl Pts',(-54.8702440456956,-111.968782610235,
174.328668113817));
#21933=CARTESIAN_POINT('Ctrl Pts',(-56.0252513271988,-111.751369888988,
173.157121776934));
#21934=CARTESIAN_POINT('Ctrl Pts',(-57.1802586087019,-111.53395716774,171.985575440051));
#21935=CARTESIAN_POINT('Ctrl Pts',(-58.8178019823517,-111.265102875298,
171.985575509377));
#21936=CARTESIAN_POINT('Ctrl Pts',(-60.4553453560015,-110.996248582855,
171.985575578703));
#21937=CARTESIAN_POINT('Ctrl Pts',(-61.610352540015,-110.778835872001,173.157122013628));
#21938=CARTESIAN_POINT('Ctrl Pts',(-62.7653597240285,-110.561423161147,
174.328668448553));
#21939=CARTESIAN_POINT('Ctrl Pts',(-62.7554215921759,-110.46820140384,175.985485236448));
#21940=CARTESIAN_POINT('Ctrl Pts',(-62.7454834603233,-110.374979646534,
177.642302024342));
#21941=CARTESIAN_POINT('Ctrl Pts',(-61.5706000529861,-110.40594883847,178.813848361225));
#21942=CARTESIAN_POINT('Ctrl Pts',(-60.3957166456489,-110.436918030407,
179.985394698108));
#21943=CARTESIAN_POINT('Ctrl Pts',(-58.7382971461651,-110.519328793539,
179.985394628782));
#21944=CARTESIAN_POINT('Ctrl Pts',(-57.0808776466813,-110.601739556671,
179.985394559456));
#21945=CARTESIAN_POINT('Ctrl Pts',(-55.9059943368337,-110.632708738214,
178.813848124531));
#21946=CARTESIAN_POINT('Ctrl Pts',(-54.7311110269862,-110.663677919758,
177.642301689606));
#21947=CARTESIAN_POINT('Ctrl Pts',(-54.7211730330048,-110.570456147754,
175.985484901711));
#21948=CARTESIAN_POINT('Ctrl Pts',(-54.7112350390234,-110.477234375749,
174.328668113817));
#21949=CARTESIAN_POINT('Ctrl Pts',(-55.8662423205265,-110.259821654502,
173.157121776934));
#21950=CARTESIAN_POINT('Ctrl Pts',(-57.0212496020297,-110.042408933255,
171.985575440051));
#21951=CARTESIAN_POINT('Ctrl Pts',(-58.6587929756795,-109.773554640812,
171.985575509377));
#21952=CARTESIAN_POINT('Ctrl Pts',(-60.2963363493293,-109.504700348369,
171.985575578703));
#21953=CARTESIAN_POINT('Ctrl Pts',(-61.4513435333428,-109.287287637515,
173.157122013628));
#21954=CARTESIAN_POINT('Ctrl Pts',(-62.6063507173563,-109.069874926661,
174.328668448553));
#21955=CARTESIAN_POINT('Ctrl Pts',(-62.5964125855037,-108.976653169355,
175.985485236448));
#21956=CARTESIAN_POINT('Ctrl Pts',(-62.5864744536511,-108.883431412048,
177.642302024342));
#21957=CARTESIAN_POINT('Ctrl Pts',(-61.4115910463139,-108.914400603985,
178.813848361225));
#21958=CARTESIAN_POINT('Ctrl Pts',(-60.2367076389767,-108.945369795921,
179.985394698108));
#21959=CARTESIAN_POINT('Ctrl Pts',(-58.5792881394929,-109.027780559053,
179.985394628782));
#21960=CARTESIAN_POINT('Ctrl Pts',(-56.921868640009,-109.110191322185,179.985394559456));
#21961=CARTESIAN_POINT('Ctrl Pts',(-55.7469853301615,-109.141160503729,
178.813848124531));
#21962=CARTESIAN_POINT('Ctrl Pts',(-54.572102020314,-109.172129685272,177.642301689606));
#21963=CARTESIAN_POINT('Ctrl Pts',(-54.5621640263326,-109.078907913268,
175.985484901711));
#21964=CARTESIAN_POINT('Ctrl Pts',(-54.5522260323511,-108.985686141264,
174.328668113817));
#21965=CARTESIAN_POINT('Ctrl Pts',(-55.7072333138543,-108.768273420016,
173.157121776934));
#21966=CARTESIAN_POINT('Ctrl Pts',(-56.8622405953575,-108.550860698769,
171.985575440051));
#21967=CARTESIAN_POINT('Ctrl Pts',(-58.4997839690073,-108.282006406326,
171.985575509377));
#21968=CARTESIAN_POINT('Ctrl Pts',(-60.1373273426571,-108.013152113884,
171.985575578703));
#21969=CARTESIAN_POINT('Ctrl Pts',(-61.2923345266706,-107.79573940303,173.157122013628));
#21970=CARTESIAN_POINT('Ctrl Pts',(-62.4473417106841,-107.578326692175,
174.328668448553));
#21971=CARTESIAN_POINT('Ctrl Pts',(-62.4374035788315,-107.485104934869,
175.985485236448));
#21972=CARTESIAN_POINT('Ctrl Pts',(-62.4274654469789,-107.391883177563,
177.642302024342));
#21973=CARTESIAN_POINT('Ctrl Pts',(-61.2525820396417,-107.422852369499,
178.813848361225));
#21974=CARTESIAN_POINT('Ctrl Pts',(-60.0776986323045,-107.453821561436,
179.985394698108));
#21975=CARTESIAN_POINT('Ctrl Pts',(-58.4202791328206,-107.536232324568,
179.985394628782));
#21976=CARTESIAN_POINT('Ctrl Pts',(-56.7628596333368,-107.6186430877,179.985394559456));
#21977=CARTESIAN_POINT('Ctrl Pts',(-55.5879763234893,-107.649612269243,
178.813848124531));
#21978=CARTESIAN_POINT('Ctrl Pts',(-54.4130930136417,-107.680581450787,
177.642301689606));
#21979=CARTESIAN_POINT('Ctrl Pts',(-54.4031550196603,-107.587359678782,
175.985484901711));
#21980=CARTESIAN_POINT('Ctrl Pts',(-54.3932170256789,-107.494137906778,
174.328668113817));
#21981=CARTESIAN_POINT('Ctrl Pts',(-55.5482243071821,-107.276725185531,
173.157121776934));
#21982=CARTESIAN_POINT('Ctrl Pts',(-56.7032315886852,-107.059312464284,
171.985575440051));
#21983=CARTESIAN_POINT('Ctrl Pts',(-58.340774962335,-106.790458171841,171.985575509377));
#21984=CARTESIAN_POINT('Ctrl Pts',(-59.9783183359848,-106.521603879398,
171.985575578703));
#21985=CARTESIAN_POINT('Ctrl Pts',(-61.1333255199984,-106.304191168544,
173.157122013628));
#21986=CARTESIAN_POINT('Ctrl Pts',(-62.2883327040119,-106.08677845769,174.328668448553));
#21987=CARTESIAN_POINT('Ctrl Pts',(-62.2783945721593,-105.993556700383,
175.985485236448));
#21988=CARTESIAN_POINT('Ctrl Pts',(-62.2684564403066,-105.900334943077,
177.642302024342));
#21989=CARTESIAN_POINT('Ctrl Pts',(-61.0935730329694,-105.931304135014,
178.813848361225));
#21990=CARTESIAN_POINT('Ctrl Pts',(-59.9186896256322,-105.96227332695,179.985394698108));
#21991=CARTESIAN_POINT('Ctrl Pts',(-58.2612701261484,-106.044684090082,
179.985394628782));
#21992=CARTESIAN_POINT('Ctrl Pts',(-56.6038506266646,-106.127094853214,
179.985394559456));
#21993=CARTESIAN_POINT('Ctrl Pts',(-55.4289673168171,-106.158064034758,
178.813848124531));
#21994=CARTESIAN_POINT('Ctrl Pts',(-54.2540840069695,-106.189033216301,
177.642301689606));
#21995=CARTESIAN_POINT('Ctrl Pts',(-54.2441460129881,-106.095811444297,
175.985484901711));
#21996=CARTESIAN_POINT('Ctrl Pts',(-54.2342080190067,-106.002589672292,
174.328668113817));
#21997=CARTESIAN_POINT('Ctrl Pts',(-55.3892153005098,-105.785176951045,
173.157121776934));
#21998=CARTESIAN_POINT('Ctrl Pts',(-56.544222582013,-105.567764229798,171.985575440051));
#21999=CARTESIAN_POINT('Ctrl Pts',(-58.1817659556628,-105.298909937355,
171.985575509377));
#22000=CARTESIAN_POINT('Ctrl Pts',(-59.8193093293126,-105.030055644913,
171.985575578703));
#22001=CARTESIAN_POINT('Ctrl Pts',(-60.9743165133261,-104.812642934058,
173.157122013628));
#22002=CARTESIAN_POINT('Ctrl Pts',(-62.1293236973396,-104.595230223204,
174.328668448553));
#22003=CARTESIAN_POINT('Ctrl Pts',(-62.119385565487,-104.502008465898,175.985485236448));
#22004=CARTESIAN_POINT('Ctrl Pts',(-62.1094474336344,-104.408786708592,
177.642302024342));
#22005=CARTESIAN_POINT('Ctrl Pts',(-60.9345640262972,-104.439755900528,
178.813848361225));
#22006=CARTESIAN_POINT('Ctrl Pts',(-59.75968061896,-104.470725092465,179.985394698108));
#22007=CARTESIAN_POINT('Ctrl Pts',(-58.1022611194762,-104.553135855597,
179.985394628782));
#22008=CARTESIAN_POINT('Ctrl Pts',(-56.4448416199923,-104.635546618729,
179.985394559456));
#22009=CARTESIAN_POINT('Ctrl Pts',(-55.2699583101448,-104.666515800272,
178.813848124531));
#22010=CARTESIAN_POINT('Ctrl Pts',(-54.0950750002973,-104.697484981815,
177.642301689606));
#22011=CARTESIAN_POINT('Ctrl Pts',(-54.0851370063159,-104.604263209811,
175.985484901711));
#22012=CARTESIAN_POINT('Ctrl Pts',(-54.0751990123344,-104.511041437807,
174.328668113817));
#22013=CARTESIAN_POINT('Ctrl Pts',(-55.2302062938376,-104.29362871656,173.157121776934));
#22014=CARTESIAN_POINT('Ctrl Pts',(-56.3852135753408,-104.076215995312,
171.985575440051));
#22015=CARTESIAN_POINT('Ctrl Pts',(-58.0227569489906,-103.80736170287,171.985575509377));
#22016=CARTESIAN_POINT('Ctrl Pts',(-59.6603003226404,-103.538507410427,
171.985575578703));
#22017=CARTESIAN_POINT('Ctrl Pts',(-60.8153075066539,-103.321094699573,
173.157122013628));
#22018=CARTESIAN_POINT('Ctrl Pts',(-61.9703146906674,-103.103681988719,
174.328668448553));
#22019=CARTESIAN_POINT('Ctrl Pts',(-61.9603765588148,-103.010460231412,
175.985485236448));
#22020=CARTESIAN_POINT('Ctrl Pts',(-61.9504384269622,-102.917238474106,
177.642302024342));
#22021=CARTESIAN_POINT('Ctrl Pts',(-60.775555019625,-102.948207666042,178.813848361225));
#22022=CARTESIAN_POINT('Ctrl Pts',(-59.6006716122878,-102.979176857979,
179.985394698108));
#22023=CARTESIAN_POINT('Ctrl Pts',(-57.943252112804,-103.061587621111,179.985394628782));
#22024=CARTESIAN_POINT('Ctrl Pts',(-56.2858326133201,-103.143998384243,
179.985394559456));
#22025=CARTESIAN_POINT('Ctrl Pts',(-55.1109493034726,-103.174967565786,
178.813848124531));
#22026=CARTESIAN_POINT('Ctrl Pts',(-53.936065993625,-103.20593674733,177.642301689606));
#22027=CARTESIAN_POINT('Ctrl Pts',(-53.9261279996436,-103.112714975326,
175.985484901711));
#22028=CARTESIAN_POINT('Ctrl Pts',(-53.9161900056622,-103.019493203321,
174.328668113817));
#22029=CARTESIAN_POINT('Ctrl Pts',(-55.0711972871654,-102.802080482074,
173.157121776934));
#22030=CARTESIAN_POINT('Ctrl Pts',(-56.2262045686686,-102.584667760827,
171.985575440051));
#22031=CARTESIAN_POINT('Ctrl Pts',(-57.8637479423184,-102.315813468384,
171.985575509377));
#22032=CARTESIAN_POINT('Ctrl Pts',(-59.5012913159682,-102.046959175941,
171.985575578703));
#22033=CARTESIAN_POINT('Ctrl Pts',(-60.6562984999817,-101.829546465087,
173.157122013628));
#22034=CARTESIAN_POINT('Ctrl Pts',(-61.8113056839952,-101.612133754233,
174.328668448553));
#22035=CARTESIAN_POINT('Ctrl Pts',(-61.8013675521426,-101.518911996927,
175.985485236448));
#22036=CARTESIAN_POINT('Ctrl Pts',(-61.79142942029,-101.42569023962,177.642302024342));
#22037=CARTESIAN_POINT('Ctrl Pts',(-60.6165460129528,-101.456659431557,
178.813848361225));
#22038=CARTESIAN_POINT('Ctrl Pts',(-59.4416626056156,-101.487628623493,
179.985394698108));
#22039=CARTESIAN_POINT('Ctrl Pts',(-57.7842431061317,-101.570039386625,
179.985394628782));
#22040=CARTESIAN_POINT('Ctrl Pts',(-56.1268236066479,-101.652450149757,
179.985394559456));
#22041=CARTESIAN_POINT('Ctrl Pts',(-54.9519402968004,-101.683419331301,
178.813848124531));
#22042=CARTESIAN_POINT('Ctrl Pts',(-53.7770569869528,-101.714388512844,
177.642301689606));
#22043=CARTESIAN_POINT('Ctrl Pts',(-53.7671189929714,-101.62116674084,175.985484901711));
#22044=CARTESIAN_POINT('Ctrl Pts',(-53.75718099899,-101.527944968836,174.328668113817));
#22045=CARTESIAN_POINT('Ctrl Pts',(-54.9121882804932,-101.310532247588,
173.157121776934));
#22046=CARTESIAN_POINT('Ctrl Pts',(-56.0671955619963,-101.093119526341,
171.985575440051));
#22047=CARTESIAN_POINT('Ctrl Pts',(-57.7047389356461,-100.824265233898,
171.985575509377));
#22048=CARTESIAN_POINT('Ctrl Pts',(-59.3422823092959,-100.555410941456,
171.985575578703));
#22049=CARTESIAN_POINT('Ctrl Pts',(-60.4972894933094,-100.337998230602,
173.157122013628));
#22050=CARTESIAN_POINT('Ctrl Pts',(-61.652296677323,-100.120585519747,174.328668448553));
#22051=CARTESIAN_POINT('Ctrl Pts',(-61.6423585454703,-100.027363762441,
175.985485236448));
#22052=CARTESIAN_POINT('Ctrl Pts',(-61.6324204136177,-99.9341420051347,
177.642302024342));
#22053=CARTESIAN_POINT('Ctrl Pts',(-60.4575370062805,-99.9651111970713,
178.813848361225));
#22054=CARTESIAN_POINT('Ctrl Pts',(-59.2826535989433,-99.9960803890078,
179.985394698108));
#22055=CARTESIAN_POINT('Ctrl Pts',(-57.6252340994595,-100.07849115214,179.985394628782));
#22056=CARTESIAN_POINT('Ctrl Pts',(-55.9678145999757,-100.160901915272,
179.985394559456));
#22057=CARTESIAN_POINT('Ctrl Pts',(-54.7929312901281,-100.191871096815,
178.813848124531));
#22058=CARTESIAN_POINT('Ctrl Pts',(-53.6180479802806,-100.222840278359,
177.642301689606));
#22059=CARTESIAN_POINT('Ctrl Pts',(-53.6081099862992,-100.129618506354,
175.985484901711));
#22060=CARTESIAN_POINT('Ctrl Pts',(-53.5981719923178,-100.03639673435,174.328668113817));
#22061=CARTESIAN_POINT('Ctrl Pts',(-54.7531792738209,-99.8189840131027,
173.157121776934));
#22062=CARTESIAN_POINT('Ctrl Pts',(-55.9081865553241,-99.6015712918555,
171.985575440051));
#22063=CARTESIAN_POINT('Ctrl Pts',(-57.5457299289739,-99.3327169994129,
171.985575509377));
#22064=CARTESIAN_POINT('Ctrl Pts',(-59.1832733026237,-99.0638627069702,
171.985575578703));
#22065=CARTESIAN_POINT('Ctrl Pts',(-60.3382804866372,-98.846449996116,173.157122013628));
#22066=CARTESIAN_POINT('Ctrl Pts',(-61.4932876706507,-98.6290372852619,
174.328668448553));
#22067=CARTESIAN_POINT('Ctrl Pts',(-61.4833495387981,-98.5358155279555,
175.985485236448));
#22068=CARTESIAN_POINT('Ctrl Pts',(-61.4734114069455,-98.4425937706491,
177.642302024342));
#22069=CARTESIAN_POINT('Ctrl Pts',(-60.2985279996083,-98.4735629625857,
178.813848361225));
#22070=CARTESIAN_POINT('Ctrl Pts',(-59.1236445922711,-98.5045321545222,
179.985394698108));
#22071=CARTESIAN_POINT('Ctrl Pts',(-57.4662250927873,-98.5869429176541,
179.985394628782));
#22072=CARTESIAN_POINT('Ctrl Pts',(-55.3866107466295,-98.6903461932525,
179.985394541796));
#22073=CARTESIAN_POINT('Ctrl Pts',(-54.187312453289,-98.7101169788701,178.284073207609));
#22074=CARTESIAN_POINT('Origin',(-57.4141964578263,-98.1510622392946,175.991014745935));
#22075=CARTESIAN_POINT('Origin',(-54.6017060172855,-98.4508925102076,178.819441752331));
#22076=CARTESIAN_POINT('Ctrl Pts',(-56.1707931031902,-113.117197303651,
178.813912075476));
#22077=CARTESIAN_POINT('Ctrl Pts',(-54.9958834532485,-113.148169293224,
177.6423391512));
#22078=CARTESIAN_POINT('Ctrl Pts',(-54.9859454592686,-113.05494752122,175.985484901707));
#22079=CARTESIAN_POINT('Ctrl Pts',(-54.9760074652888,-112.961725749215,
174.328630652215));
#22080=CARTESIAN_POINT('Ctrl Pts',(-56.1310410868884,-112.744310219938,
173.157057825983));
#22081=CARTESIAN_POINT('Ctrl Pts',(-57.286074708488,-112.52689469066,171.985484999752));
#22082=CARTESIAN_POINT('Ctrl Pts',(-58.9236553326578,-112.258036427063,
171.985485069079));
#22083=CARTESIAN_POINT('Ctrl Pts',(-60.5612359568277,-111.989178163466,
171.985485138407));
#22084=CARTESIAN_POINT('Ctrl Pts',(-61.7162694809355,-111.771762644582,
173.157058062683));
#22085=CARTESIAN_POINT('Ctrl Pts',(-62.8713030050432,-111.554347125698,
174.328630986959));
#22086=CARTESIAN_POINT('Ctrl Pts',(-62.861364873189,-111.461125368392,175.985485236451));
#22087=CARTESIAN_POINT('Ctrl Pts',(-62.8514267413349,-111.367903611086,
177.642339485944));
#22088=CARTESIAN_POINT('Ctrl Pts',(-61.6765169939012,-111.398875611052,
178.813912312176));
#22089=CARTESIAN_POINT('Ctrl Pts',(-60.5016072464676,-111.429847611019,
179.985485138407));
#22090=CARTESIAN_POINT('Ctrl Pts',(-58.8441504964637,-111.512262345305,
179.985485069079));
#22091=CARTESIAN_POINT('Ctrl Pts',(-57.1866937464598,-111.594677079592,
179.985484999752));
#22092=CARTESIAN_POINT('Ctrl Pts',(-56.011784096518,-111.625649069165,178.813912075476));
#22093=CARTESIAN_POINT('Ctrl Pts',(-54.8368744465763,-111.656621058739,
177.6423391512));
#22094=CARTESIAN_POINT('Ctrl Pts',(-54.8269364525964,-111.563399286734,
175.985484901707));
#22095=CARTESIAN_POINT('Ctrl Pts',(-54.8169984586165,-111.47017751473,174.328630652215));
#22096=CARTESIAN_POINT('Ctrl Pts',(-55.9720320802161,-111.252761985452,
173.157057825983));
#22097=CARTESIAN_POINT('Ctrl Pts',(-57.1270657018158,-111.035346456175,
171.985484999752));
#22098=CARTESIAN_POINT('Ctrl Pts',(-58.7646463259856,-110.766488192578,
171.985485069079));
#22099=CARTESIAN_POINT('Ctrl Pts',(-60.4022269501555,-110.497629928981,
171.985485138407));
#22100=CARTESIAN_POINT('Ctrl Pts',(-61.5572604742632,-110.280214410097,
173.157058062683));
#22101=CARTESIAN_POINT('Ctrl Pts',(-62.712293998371,-110.062798891212,174.328630986959));
#22102=CARTESIAN_POINT('Ctrl Pts',(-62.7023558665168,-109.969577133906,
175.985485236451));
#22103=CARTESIAN_POINT('Ctrl Pts',(-62.6924177346626,-109.8763553766,177.642339485944));
#22104=CARTESIAN_POINT('Ctrl Pts',(-61.517507987229,-109.907327376567,178.813912312176));
#22105=CARTESIAN_POINT('Ctrl Pts',(-60.3425982397954,-109.938299376534,
179.985485138407));
#22106=CARTESIAN_POINT('Ctrl Pts',(-58.6851414897915,-110.02071411082,179.985485069079));
#22107=CARTESIAN_POINT('Ctrl Pts',(-57.0276847397876,-110.103128845106,
179.985484999752));
#22108=CARTESIAN_POINT('Ctrl Pts',(-55.8527750898458,-110.13410083468,178.813912075476));
#22109=CARTESIAN_POINT('Ctrl Pts',(-54.677865439904,-110.165072824253,177.6423391512));
#22110=CARTESIAN_POINT('Ctrl Pts',(-54.6679274459242,-110.071851052249,
175.985484901707));
#22111=CARTESIAN_POINT('Ctrl Pts',(-54.6579894519443,-109.978629280244,
174.328630652215));
#22112=CARTESIAN_POINT('Ctrl Pts',(-55.8130230735439,-109.761213750967,
173.157057825983));
#22113=CARTESIAN_POINT('Ctrl Pts',(-56.9680566951435,-109.543798221689,
171.985484999752));
#22114=CARTESIAN_POINT('Ctrl Pts',(-58.6056373193134,-109.274939958092,
171.985485069079));
#22115=CARTESIAN_POINT('Ctrl Pts',(-60.2432179434833,-109.006081694495,
171.985485138407));
#22116=CARTESIAN_POINT('Ctrl Pts',(-61.398251467591,-108.788666175611,173.157058062683));
#22117=CARTESIAN_POINT('Ctrl Pts',(-62.5532849916988,-108.571250656727,
174.328630986959));
#22118=CARTESIAN_POINT('Ctrl Pts',(-62.5433468598446,-108.478028899421,
175.985485236451));
#22119=CARTESIAN_POINT('Ctrl Pts',(-62.5334087279904,-108.384807142114,
177.642339485944));
#22120=CARTESIAN_POINT('Ctrl Pts',(-61.3584989805568,-108.415779142081,
178.813912312176));
#22121=CARTESIAN_POINT('Ctrl Pts',(-60.1835892331231,-108.446751142048,
179.985485138407));
#22122=CARTESIAN_POINT('Ctrl Pts',(-58.5261324831192,-108.529165876334,
179.985485069079));
#22123=CARTESIAN_POINT('Ctrl Pts',(-56.8686757331153,-108.611580610621,
179.985484999752));
#22124=CARTESIAN_POINT('Ctrl Pts',(-55.6937660831736,-108.642552600194,
178.813912075476));
#22125=CARTESIAN_POINT('Ctrl Pts',(-54.5188564332318,-108.673524589768,
177.6423391512));
#22126=CARTESIAN_POINT('Ctrl Pts',(-54.5089184392519,-108.580302817763,
175.985484901707));
#22127=CARTESIAN_POINT('Ctrl Pts',(-54.4989804452721,-108.487081045759,
174.328630652215));
#22128=CARTESIAN_POINT('Ctrl Pts',(-55.6540140668717,-108.269665516481,
173.157057825983));
#22129=CARTESIAN_POINT('Ctrl Pts',(-56.8090476884713,-108.052249987204,
171.985484999752));
#22130=CARTESIAN_POINT('Ctrl Pts',(-58.4466283126412,-107.783391723607,
171.985485069079));
#22131=CARTESIAN_POINT('Ctrl Pts',(-60.084208936811,-107.51453346001,171.985485138407));
#22132=CARTESIAN_POINT('Ctrl Pts',(-61.2392424609188,-107.297117941125,
173.157058062683));
#22133=CARTESIAN_POINT('Ctrl Pts',(-62.3942759850265,-107.079702422241,
174.328630986959));
#22134=CARTESIAN_POINT('Ctrl Pts',(-62.3843378531723,-106.986480664935,
175.985485236451));
#22135=CARTESIAN_POINT('Ctrl Pts',(-62.3743997213182,-106.893258907629,
177.642339485944));
#22136=CARTESIAN_POINT('Ctrl Pts',(-61.1994899738845,-106.924230907596,
178.813912312176));
#22137=CARTESIAN_POINT('Ctrl Pts',(-60.0245802264509,-106.955202907562,
179.985485138407));
#22138=CARTESIAN_POINT('Ctrl Pts',(-58.367123476447,-107.037617641849,179.985485069079));
#22139=CARTESIAN_POINT('Ctrl Pts',(-56.7096667264431,-107.120032376135,
179.985484999752));
#22140=CARTESIAN_POINT('Ctrl Pts',(-55.5347570765013,-107.151004365708,
178.813912075476));
#22141=CARTESIAN_POINT('Ctrl Pts',(-54.3598474265596,-107.181976355282,
177.6423391512));
#22142=CARTESIAN_POINT('Ctrl Pts',(-54.3499094325797,-107.088754583277,
175.985484901707));
#22143=CARTESIAN_POINT('Ctrl Pts',(-54.3399714385998,-106.995532811273,
174.328630652215));
#22144=CARTESIAN_POINT('Ctrl Pts',(-55.4950050601995,-106.778117281995,
173.157057825983));
#22145=CARTESIAN_POINT('Ctrl Pts',(-56.6500386817991,-106.560701752718,
171.985484999752));
#22146=CARTESIAN_POINT('Ctrl Pts',(-58.2876193059689,-106.291843489121,
171.985485069079));
#22147=CARTESIAN_POINT('Ctrl Pts',(-59.9251999301388,-106.022985225524,
171.985485138407));
#22148=CARTESIAN_POINT('Ctrl Pts',(-61.0802334542465,-105.80556970664,173.157058062683));
#22149=CARTESIAN_POINT('Ctrl Pts',(-62.2352669783543,-105.588154187756,
174.328630986959));
#22150=CARTESIAN_POINT('Ctrl Pts',(-62.2253288465001,-105.494932430449,
175.985485236451));
#22151=CARTESIAN_POINT('Ctrl Pts',(-62.2153907146459,-105.401710673143,
177.642339485944));
#22152=CARTESIAN_POINT('Ctrl Pts',(-61.0404809672123,-105.43268267311,178.813912312176));
#22153=CARTESIAN_POINT('Ctrl Pts',(-59.8655712197787,-105.463654673077,
179.985485138407));
#22154=CARTESIAN_POINT('Ctrl Pts',(-58.2081144697748,-105.546069407363,
179.985485069079));
#22155=CARTESIAN_POINT('Ctrl Pts',(-56.5506577197709,-105.628484141649,
179.985484999752));
#22156=CARTESIAN_POINT('Ctrl Pts',(-55.3757480698291,-105.659456131223,
178.813912075476));
#22157=CARTESIAN_POINT('Ctrl Pts',(-54.2008384198873,-105.690428120796,
177.6423391512));
#22158=CARTESIAN_POINT('Ctrl Pts',(-54.1909004259075,-105.597206348792,
175.985484901707));
#22159=CARTESIAN_POINT('Ctrl Pts',(-54.1809624319276,-105.503984576787,
174.328630652215));
#22160=CARTESIAN_POINT('Ctrl Pts',(-55.3359960535272,-105.28656904751,173.157057825983));
#22161=CARTESIAN_POINT('Ctrl Pts',(-56.4910296751268,-105.069153518232,
171.985484999752));
#22162=CARTESIAN_POINT('Ctrl Pts',(-58.1286102992967,-104.800295254635,
171.985485069079));
#22163=CARTESIAN_POINT('Ctrl Pts',(-59.7661909234666,-104.531436991038,
171.985485138407));
#22164=CARTESIAN_POINT('Ctrl Pts',(-60.9212244475743,-104.314021472154,
173.157058062683));
#22165=CARTESIAN_POINT('Ctrl Pts',(-62.0762579716821,-104.09660595327,174.328630986959));
#22166=CARTESIAN_POINT('Ctrl Pts',(-62.0663198398279,-104.003384195964,
175.985485236451));
#22167=CARTESIAN_POINT('Ctrl Pts',(-62.0563817079737,-103.910162438658,
177.642339485944));
#22168=CARTESIAN_POINT('Ctrl Pts',(-60.8814719605401,-103.941134438624,
178.813912312176));
#22169=CARTESIAN_POINT('Ctrl Pts',(-59.7065622131064,-103.972106438591,
179.985485138407));
#22170=CARTESIAN_POINT('Ctrl Pts',(-58.0491054631025,-104.054521172878,
179.985485069079));
#22171=CARTESIAN_POINT('Ctrl Pts',(-56.3916487130987,-104.136935907164,
179.985484999752));
#22172=CARTESIAN_POINT('Ctrl Pts',(-55.2167390631569,-104.167907896737,
178.813912075476));
#22173=CARTESIAN_POINT('Ctrl Pts',(-54.0418294132151,-104.198879886311,
177.6423391512));
#22174=CARTESIAN_POINT('Ctrl Pts',(-54.0318914192353,-104.105658114306,
175.985484901707));
#22175=CARTESIAN_POINT('Ctrl Pts',(-54.0219534252554,-104.012436342302,
174.328630652215));
#22176=CARTESIAN_POINT('Ctrl Pts',(-55.176987046855,-103.795020813024,173.157057825983));
#22177=CARTESIAN_POINT('Ctrl Pts',(-56.3320206684546,-103.577605283747,
171.985484999752));
#22178=CARTESIAN_POINT('Ctrl Pts',(-57.9696012926245,-103.30874702015,171.985485069079));
#22179=CARTESIAN_POINT('Ctrl Pts',(-59.6071819167943,-103.039888756553,
171.985485138407));
#22180=CARTESIAN_POINT('Ctrl Pts',(-60.7622154409021,-102.822473237669,
173.157058062683));
#22181=CARTESIAN_POINT('Ctrl Pts',(-61.9172489650099,-102.605057718784,
174.328630986959));
#22182=CARTESIAN_POINT('Ctrl Pts',(-61.9073108331557,-102.511835961478,
175.985485236451));
#22183=CARTESIAN_POINT('Ctrl Pts',(-61.8973727013015,-102.418614204172,
177.642339485944));
#22184=CARTESIAN_POINT('Ctrl Pts',(-60.7224629538678,-102.449586204139,
178.813912312176));
#22185=CARTESIAN_POINT('Ctrl Pts',(-59.5475532064342,-102.480558204106,
179.985485138407));
#22186=CARTESIAN_POINT('Ctrl Pts',(-57.8900964564303,-102.562972938392,
179.985485069079));
#22187=CARTESIAN_POINT('Ctrl Pts',(-56.2326397064264,-102.645387672678,
179.985484999752));
#22188=CARTESIAN_POINT('Ctrl Pts',(-55.0577300564847,-102.676359662252,
178.813912075476));
#22189=CARTESIAN_POINT('Ctrl Pts',(-53.8828204065429,-102.707331651825,
177.6423391512));
#22190=CARTESIAN_POINT('Ctrl Pts',(-53.872882412563,-102.614109879821,175.985484901707));
#22191=CARTESIAN_POINT('Ctrl Pts',(-53.8629444185832,-102.520888107816,
174.328630652215));
#22192=CARTESIAN_POINT('Ctrl Pts',(-55.0179780401828,-102.303472578539,
173.157057825983));
#22193=CARTESIAN_POINT('Ctrl Pts',(-56.1730116617824,-102.086057049261,
171.985484999752));
#22194=CARTESIAN_POINT('Ctrl Pts',(-57.8105922859523,-101.817198785664,
171.985485069079));
#22195=CARTESIAN_POINT('Ctrl Pts',(-59.4481729101221,-101.548340522067,
171.985485138407));
#22196=CARTESIAN_POINT('Ctrl Pts',(-60.6032064342299,-101.330925003183,
173.157058062683));
#22197=CARTESIAN_POINT('Ctrl Pts',(-61.7582399583376,-101.113509484299,
174.328630986959));
#22198=CARTESIAN_POINT('Ctrl Pts',(-61.7483018264834,-101.020287726993,
175.985485236451));
#22199=CARTESIAN_POINT('Ctrl Pts',(-61.7383636946293,-100.927065969686,
177.642339485944));
#22200=CARTESIAN_POINT('Ctrl Pts',(-60.5634539471956,-100.958037969653,
178.813912312176));
#22201=CARTESIAN_POINT('Ctrl Pts',(-59.388544199762,-100.98900996962,179.985485138407));
#22202=CARTESIAN_POINT('Ctrl Pts',(-57.7310874497581,-101.071424703906,
179.985485069079));
#22203=CARTESIAN_POINT('Ctrl Pts',(-56.0736306997542,-101.153839438193,
179.985484999752));
#22204=CARTESIAN_POINT('Ctrl Pts',(-54.8987210498124,-101.184811427766,
178.813912075476));
#22205=CARTESIAN_POINT('Ctrl Pts',(-53.7238113998707,-101.21578341734,177.6423391512));
#22206=CARTESIAN_POINT('Ctrl Pts',(-53.7138734058908,-101.122561645335,
175.985484901707));
#22207=CARTESIAN_POINT('Ctrl Pts',(-53.7039354119109,-101.029339873331,
174.328630652215));
#22208=CARTESIAN_POINT('Ctrl Pts',(-54.8589690335105,-100.811924344053,
173.157057825983));
#22209=CARTESIAN_POINT('Ctrl Pts',(-56.0140026551102,-100.594508814776,
171.985484999752));
#22210=CARTESIAN_POINT('Ctrl Pts',(-57.65158327928,-100.325650551179,171.985485069079));
#22211=CARTESIAN_POINT('Ctrl Pts',(-59.2891639034499,-100.056792287582,
171.985485138407));
#22212=CARTESIAN_POINT('Ctrl Pts',(-60.4441974275576,-99.8393767686974,
173.157058062683));
#22213=CARTESIAN_POINT('Ctrl Pts',(-61.5992309516654,-99.6219612498133,
174.328630986959));
#22214=CARTESIAN_POINT('Ctrl Pts',(-61.5892928198112,-99.528739492507,175.985485236451));
#22215=CARTESIAN_POINT('Ctrl Pts',(-61.579354687957,-99.4355177352008,177.642339485944));
#22216=CARTESIAN_POINT('Ctrl Pts',(-60.4044449405234,-99.4664897351676,
178.813912312176));
#22217=CARTESIAN_POINT('Ctrl Pts',(-59.2295351930898,-99.4974617351344,
179.985485138407));
#22218=CARTESIAN_POINT('Ctrl Pts',(-57.5720784430859,-99.5798764694207,
179.985485069079));
#22219=CARTESIAN_POINT('Ctrl Pts',(-55.914621693082,-99.662291203707,179.985484999752));
#22220=CARTESIAN_POINT('Ctrl Pts',(-54.7397120431402,-99.6932631932805,
178.813912075476));
#22221=CARTESIAN_POINT('Ctrl Pts',(-53.5648023931984,-99.724235182854,177.6423391512));
#22222=CARTESIAN_POINT('Ctrl Pts',(-53.5548643992186,-99.6310134108495,
175.985484901707));
#22223=CARTESIAN_POINT('Ctrl Pts',(-53.5449264052387,-99.5377916388449,
174.328630652215));
#22224=CARTESIAN_POINT('Ctrl Pts',(-54.6999600268383,-99.3203761095675,
173.157057825983));
#22225=CARTESIAN_POINT('Ctrl Pts',(-55.8549936484379,-99.10296058029,171.985484999752));
#22226=CARTESIAN_POINT('Ctrl Pts',(-57.4925742726078,-98.834102316693,171.985485069079));
#22227=CARTESIAN_POINT('Ctrl Pts',(-59.1301548967777,-98.5652440530961,
171.985485138407));
#22228=CARTESIAN_POINT('Ctrl Pts',(-60.2851884208854,-98.3478285342118,
173.157058062683));
#22229=CARTESIAN_POINT('Ctrl Pts',(-61.4402219449932,-98.1304130153276,
174.328630986959));
#22230=CARTESIAN_POINT('Ctrl Pts',(-61.430283813139,-98.0371912580215,175.985485236451));
#22231=CARTESIAN_POINT('Ctrl Pts',(-61.4203456812848,-97.9439695007152,
177.642339485944));
#22232=CARTESIAN_POINT('Ctrl Pts',(-60.2454359338512,-97.974941500682,178.813912312176));
#22233=CARTESIAN_POINT('Ctrl Pts',(-59.0705261864175,-98.0059135006488,
179.985485138407));
#22234=CARTESIAN_POINT('Ctrl Pts',(-57.4130694364136,-98.0883282349351,
179.985485069079));
#22235=CARTESIAN_POINT('Ctrl Pts',(-55.7556126864097,-98.1707429692214,
179.985484999752));
#22236=CARTESIAN_POINT('Ctrl Pts',(-54.580703036468,-98.2017149587949,178.813912075476));
#22237=CARTESIAN_POINT('Ctrl Pts',(-56.181115489574,-113.283598570176,178.821287383467));
#22238=CARTESIAN_POINT('Ctrl Pts',(-55.0031681001975,-113.314894403068,
177.646659506339));
#22239=CARTESIAN_POINT('Ctrl Pts',(-54.9932301063974,-113.221672631044,
175.985484901271));
#22240=CARTESIAN_POINT('Ctrl Pts',(-54.9832921125973,-113.12845085902,174.324310296203));
#22241=CARTESIAN_POINT('Ctrl Pts',(-56.1413634738858,-112.910711486397,
173.149682517375));
#22242=CARTESIAN_POINT('Ctrl Pts',(-57.2994348351743,-112.692972113774,
171.975054738546));
#22243=CARTESIAN_POINT('Ctrl Pts',(-58.9413114718314,-112.423655866545,
171.975054808055));
#22244=CARTESIAN_POINT('Ctrl Pts',(-60.5831881084886,-112.154339619316,
171.975054877564));
#22245=CARTESIAN_POINT('Ctrl Pts',(-61.741259372031,-111.936600257113,173.149682754692));
#22246=CARTESIAN_POINT('Ctrl Pts',(-62.8993306355734,-111.71886089491,174.32431063182));
#22247=CARTESIAN_POINT('Ctrl Pts',(-62.8893925035395,-111.625639137623,
175.985485236888));
#22248=CARTESIAN_POINT('Ctrl Pts',(-62.8794543715055,-111.532417380336,
177.646659841956));
#22249=CARTESIAN_POINT('Ctrl Pts',(-61.701506884383,-111.563713223648,178.821287620784));
#22250=CARTESIAN_POINT('Ctrl Pts',(-60.5235593972605,-111.595009066961,
179.995915399612));
#22251=CARTESIAN_POINT('Ctrl Pts',(-58.8618066347693,-111.677881784879,
179.995915330104));
#22252=CARTESIAN_POINT('Ctrl Pts',(-57.2000538722782,-111.760754502798,
179.995915260595));
#22253=CARTESIAN_POINT('Ctrl Pts',(-56.0221064829017,-111.79205033569,178.821287383467));
#22254=CARTESIAN_POINT('Ctrl Pts',(-54.8441590935253,-111.823346168582,
177.646659506339));
#22255=CARTESIAN_POINT('Ctrl Pts',(-54.8342210997252,-111.730124396559,
175.985484901271));
#22256=CARTESIAN_POINT('Ctrl Pts',(-54.8242831059251,-111.636902624535,
174.324310296203));
#22257=CARTESIAN_POINT('Ctrl Pts',(-55.9823544672136,-111.419163251912,
173.149682517375));
#22258=CARTESIAN_POINT('Ctrl Pts',(-57.1404258285021,-111.201423879289,
171.975054738546));
#22259=CARTESIAN_POINT('Ctrl Pts',(-58.7823024651592,-110.932107632059,
171.975054808055));
#22260=CARTESIAN_POINT('Ctrl Pts',(-60.4241791018163,-110.66279138483,171.975054877564));
#22261=CARTESIAN_POINT('Ctrl Pts',(-61.5822503653587,-110.445052022627,
173.149682754692));
#22262=CARTESIAN_POINT('Ctrl Pts',(-62.7403216289012,-110.227312660424,
174.32431063182));
#22263=CARTESIAN_POINT('Ctrl Pts',(-62.7303834968672,-110.134090903137,
175.985485236888));
#22264=CARTESIAN_POINT('Ctrl Pts',(-62.7204453648333,-110.04086914585,177.646659841956));
#22265=CARTESIAN_POINT('Ctrl Pts',(-61.5424978777108,-110.072164989163,
178.821287620784));
#22266=CARTESIAN_POINT('Ctrl Pts',(-60.3645503905882,-110.103460832475,
179.995915399612));
#22267=CARTESIAN_POINT('Ctrl Pts',(-58.7027976280971,-110.186333550394,
179.995915330104));
#22268=CARTESIAN_POINT('Ctrl Pts',(-57.041044865606,-110.269206268313,179.995915260595));
#22269=CARTESIAN_POINT('Ctrl Pts',(-55.8630974762295,-110.300502101205,
178.821287383467));
#22270=CARTESIAN_POINT('Ctrl Pts',(-54.6851500868531,-110.331797934097,
177.646659506339));
#22271=CARTESIAN_POINT('Ctrl Pts',(-54.675212093053,-110.238576162073,175.985484901271));
#22272=CARTESIAN_POINT('Ctrl Pts',(-54.6652740992529,-110.145354390049,
174.324310296203));
#22273=CARTESIAN_POINT('Ctrl Pts',(-55.8233454605414,-109.927615017426,
173.149682517375));
#22274=CARTESIAN_POINT('Ctrl Pts',(-56.9814168218299,-109.709875644803,
171.975054738546));
#22275=CARTESIAN_POINT('Ctrl Pts',(-58.623293458487,-109.440559397574,171.975054808055));
#22276=CARTESIAN_POINT('Ctrl Pts',(-60.2651700951441,-109.171243150344,
171.975054877564));
#22277=CARTESIAN_POINT('Ctrl Pts',(-61.4232413586865,-108.953503788142,
173.149682754692));
#22278=CARTESIAN_POINT('Ctrl Pts',(-62.581312622229,-108.735764425939,174.32431063182));
#22279=CARTESIAN_POINT('Ctrl Pts',(-62.571374490195,-108.642542668652,175.985485236888));
#22280=CARTESIAN_POINT('Ctrl Pts',(-62.5614363581611,-108.549320911365,
177.646659841956));
#22281=CARTESIAN_POINT('Ctrl Pts',(-61.3834888710385,-108.580616754677,
178.821287620784));
#22282=CARTESIAN_POINT('Ctrl Pts',(-60.205541383916,-108.61191259799,179.995915399612));
#22283=CARTESIAN_POINT('Ctrl Pts',(-58.5437886214249,-108.694785315908,
179.995915330104));
#22284=CARTESIAN_POINT('Ctrl Pts',(-56.8820358589338,-108.777658033827,
179.995915260595));
#22285=CARTESIAN_POINT('Ctrl Pts',(-55.7040884695573,-108.808953866719,
178.821287383467));
#22286=CARTESIAN_POINT('Ctrl Pts',(-54.5261410801808,-108.840249699611,
177.646659506339));
#22287=CARTESIAN_POINT('Ctrl Pts',(-54.5162030863807,-108.747027927587,
175.985484901271));
#22288=CARTESIAN_POINT('Ctrl Pts',(-54.5062650925806,-108.653806155564,
174.324310296203));
#22289=CARTESIAN_POINT('Ctrl Pts',(-55.6643364538691,-108.436066782941,
173.149682517375));
#22290=CARTESIAN_POINT('Ctrl Pts',(-56.8224078151577,-108.218327410317,
171.975054738546));
#22291=CARTESIAN_POINT('Ctrl Pts',(-58.4642844518147,-107.949011163088,
171.975054808055));
#22292=CARTESIAN_POINT('Ctrl Pts',(-60.1061610884719,-107.679694915859,
171.975054877564));
#22293=CARTESIAN_POINT('Ctrl Pts',(-61.2642323520143,-107.461955553656,
173.149682754692));
#22294=CARTESIAN_POINT('Ctrl Pts',(-62.4223036155567,-107.244216191453,
174.32431063182));
#22295=CARTESIAN_POINT('Ctrl Pts',(-62.4123654835228,-107.150994434166,
175.985485236888));
#22296=CARTESIAN_POINT('Ctrl Pts',(-62.4024273514889,-107.057772676879,
177.646659841956));
#22297=CARTESIAN_POINT('Ctrl Pts',(-61.2244798643663,-107.089068520192,
178.821287620784));
#22298=CARTESIAN_POINT('Ctrl Pts',(-60.0465323772438,-107.120364363504,
179.995915399612));
#22299=CARTESIAN_POINT('Ctrl Pts',(-58.3847796147526,-107.203237081423,
179.995915330104));
#22300=CARTESIAN_POINT('Ctrl Pts',(-56.7230268522615,-107.286109799341,
179.995915260595));
#22301=CARTESIAN_POINT('Ctrl Pts',(-55.5450794628851,-107.317405632233,
178.821287383467));
#22302=CARTESIAN_POINT('Ctrl Pts',(-54.3671320735086,-107.348701465125,
177.646659506339));
#22303=CARTESIAN_POINT('Ctrl Pts',(-54.3571940797085,-107.255479693102,
175.985484901271));
#22304=CARTESIAN_POINT('Ctrl Pts',(-54.3472560859084,-107.162257921078,
174.324310296203));
#22305=CARTESIAN_POINT('Ctrl Pts',(-55.5053274471969,-106.944518548455,
173.149682517375));
#22306=CARTESIAN_POINT('Ctrl Pts',(-56.6633988084854,-106.726779175832,
171.975054738546));
#22307=CARTESIAN_POINT('Ctrl Pts',(-58.3052754451425,-106.457462928602,
171.975054808055));
#22308=CARTESIAN_POINT('Ctrl Pts',(-59.9471520817997,-106.188146681373,
171.975054877564));
#22309=CARTESIAN_POINT('Ctrl Pts',(-61.1052233453421,-105.97040731917,173.149682754692));
#22310=CARTESIAN_POINT('Ctrl Pts',(-62.2632946088845,-105.752667956968,
174.32431063182));
#22311=CARTESIAN_POINT('Ctrl Pts',(-62.2533564768505,-105.659446199681,
175.985485236888));
#22312=CARTESIAN_POINT('Ctrl Pts',(-62.2434183448166,-105.566224442394,
177.646659841956));
#22313=CARTESIAN_POINT('Ctrl Pts',(-61.0654708576941,-105.597520285706,
178.821287620784));
#22314=CARTESIAN_POINT('Ctrl Pts',(-59.8875233705716,-105.628816129018,
179.995915399612));
#22315=CARTESIAN_POINT('Ctrl Pts',(-58.2257706080804,-105.711688846937,
179.995915330104));
#22316=CARTESIAN_POINT('Ctrl Pts',(-56.5640178455893,-105.794561564856,
179.995915260595));
#22317=CARTESIAN_POINT('Ctrl Pts',(-55.3860704562128,-105.825857397748,
178.821287383467));
#22318=CARTESIAN_POINT('Ctrl Pts',(-54.2081230668364,-105.85715323064,177.646659506339));
#22319=CARTESIAN_POINT('Ctrl Pts',(-54.1981850730363,-105.763931458616,
175.985484901271));
#22320=CARTESIAN_POINT('Ctrl Pts',(-54.1882470792362,-105.670709686593,
174.324310296203));
#22321=CARTESIAN_POINT('Ctrl Pts',(-55.3463184405247,-105.452970313969,
173.149682517375));
#22322=CARTESIAN_POINT('Ctrl Pts',(-56.5043898018132,-105.235230941346,
171.975054738546));
#22323=CARTESIAN_POINT('Ctrl Pts',(-58.1462664384703,-104.965914694117,
171.975054808055));
#22324=CARTESIAN_POINT('Ctrl Pts',(-59.7881430751274,-104.696598446888,
171.975054877564));
#22325=CARTESIAN_POINT('Ctrl Pts',(-60.9462143386698,-104.478859084685,
173.149682754692));
#22326=CARTESIAN_POINT('Ctrl Pts',(-62.1042856022123,-104.261119722482,
174.32431063182));
#22327=CARTESIAN_POINT('Ctrl Pts',(-62.0943474701783,-104.167897965195,
175.985485236888));
#22328=CARTESIAN_POINT('Ctrl Pts',(-62.0844093381444,-104.074676207908,
177.646659841956));
#22329=CARTESIAN_POINT('Ctrl Pts',(-60.9064618510219,-104.10597205122,178.821287620784));
#22330=CARTESIAN_POINT('Ctrl Pts',(-59.7285143638993,-104.137267894533,
179.995915399612));
#22331=CARTESIAN_POINT('Ctrl Pts',(-58.0667616014082,-104.220140612451,
179.995915330104));
#22332=CARTESIAN_POINT('Ctrl Pts',(-56.4050088389171,-104.30301333037,179.995915260595));
#22333=CARTESIAN_POINT('Ctrl Pts',(-55.2270614495406,-104.334309163262,
178.821287383467));
#22334=CARTESIAN_POINT('Ctrl Pts',(-54.0491140601642,-104.365604996154,
177.646659506339));
#22335=CARTESIAN_POINT('Ctrl Pts',(-54.039176066364,-104.272383224131,175.985484901271));
#22336=CARTESIAN_POINT('Ctrl Pts',(-54.029238072564,-104.179161452107,174.324310296203));
#22337=CARTESIAN_POINT('Ctrl Pts',(-55.1873094338524,-103.961422079484,
173.149682517375));
#22338=CARTESIAN_POINT('Ctrl Pts',(-56.345380795141,-103.743682706861,171.975054738546));
#22339=CARTESIAN_POINT('Ctrl Pts',(-57.9872574317981,-103.474366459631,
171.975054808055));
#22340=CARTESIAN_POINT('Ctrl Pts',(-59.6291340684552,-103.205050212402,
171.975054877564));
#22341=CARTESIAN_POINT('Ctrl Pts',(-60.7872053319976,-102.987310850199,
173.149682754692));
#22342=CARTESIAN_POINT('Ctrl Pts',(-61.94527659554,-102.769571487996,174.32431063182));
#22343=CARTESIAN_POINT('Ctrl Pts',(-61.9353384635061,-102.676349730709,
175.985485236888));
#22344=CARTESIAN_POINT('Ctrl Pts',(-61.9254003314722,-102.583127973422,
177.646659841956));
#22345=CARTESIAN_POINT('Ctrl Pts',(-60.7474528443496,-102.614423816735,
178.821287620784));
#22346=CARTESIAN_POINT('Ctrl Pts',(-59.5695053572271,-102.645719660047,
179.995915399612));
#22347=CARTESIAN_POINT('Ctrl Pts',(-57.907752594736,-102.728592377966,179.995915330104));
#22348=CARTESIAN_POINT('Ctrl Pts',(-56.2459998322448,-102.811465095885,
179.995915260595));
#22349=CARTESIAN_POINT('Ctrl Pts',(-55.0680524428684,-102.842760928777,
178.821287383467));
#22350=CARTESIAN_POINT('Ctrl Pts',(-53.8901050534919,-102.874056761669,
177.646659506339));
#22351=CARTESIAN_POINT('Ctrl Pts',(-53.8801670596918,-102.780834989645,
175.985484901271));
#22352=CARTESIAN_POINT('Ctrl Pts',(-53.8702290658917,-102.687613217621,
174.324310296203));
#22353=CARTESIAN_POINT('Ctrl Pts',(-55.0283004271802,-102.469873844998,
173.149682517375));
#22354=CARTESIAN_POINT('Ctrl Pts',(-56.1863717884687,-102.252134472375,
171.975054738546));
#22355=CARTESIAN_POINT('Ctrl Pts',(-57.8282484251258,-101.982818225146,
171.975054808055));
#22356=CARTESIAN_POINT('Ctrl Pts',(-59.470125061783,-101.713501977916,171.975054877564));
#22357=CARTESIAN_POINT('Ctrl Pts',(-60.6281963253254,-101.495762615714,
173.149682754692));
#22358=CARTESIAN_POINT('Ctrl Pts',(-61.7862675888678,-101.278023253511,
174.32431063182));
#22359=CARTESIAN_POINT('Ctrl Pts',(-61.7763294568339,-101.184801496224,
175.985485236888));
#22360=CARTESIAN_POINT('Ctrl Pts',(-61.7663913247999,-101.091579738937,
177.646659841956));
#22361=CARTESIAN_POINT('Ctrl Pts',(-60.5884438376774,-101.122875582249,
178.821287620784));
#22362=CARTESIAN_POINT('Ctrl Pts',(-59.4104963505549,-101.154171425562,
179.995915399612));
#22363=CARTESIAN_POINT('Ctrl Pts',(-57.7487435880637,-101.23704414348,179.995915330104));
#22364=CARTESIAN_POINT('Ctrl Pts',(-56.0869908255726,-101.319916861399,
179.995915260595));
#22365=CARTESIAN_POINT('Ctrl Pts',(-54.9090434361961,-101.351212694291,
178.821287383467));
#22366=CARTESIAN_POINT('Ctrl Pts',(-53.7310960468197,-101.382508527183,
177.646659506339));
#22367=CARTESIAN_POINT('Ctrl Pts',(-53.7211580530196,-101.289286755159,
175.985484901271));
#22368=CARTESIAN_POINT('Ctrl Pts',(-53.7112200592195,-101.196064983136,
174.324310296203));
#22369=CARTESIAN_POINT('Ctrl Pts',(-54.869291420508,-100.978325610513,173.149682517375));
#22370=CARTESIAN_POINT('Ctrl Pts',(-56.0273627817965,-100.760586237889,
171.975054738546));
#22371=CARTESIAN_POINT('Ctrl Pts',(-57.6692394184536,-100.49126999066,171.975054808055));
#22372=CARTESIAN_POINT('Ctrl Pts',(-59.3111160551107,-100.221953743431,
171.975054877564));
#22373=CARTESIAN_POINT('Ctrl Pts',(-60.4691873186531,-100.004214381228,
173.149682754692));
#22374=CARTESIAN_POINT('Ctrl Pts',(-61.6272585821956,-99.7864750190253,
174.32431063182));
#22375=CARTESIAN_POINT('Ctrl Pts',(-61.6173204501616,-99.6932532617382,
175.985485236888));
#22376=CARTESIAN_POINT('Ctrl Pts',(-61.6073823181277,-99.6000315044512,
177.646659841956));
#22377=CARTESIAN_POINT('Ctrl Pts',(-60.4294348310052,-99.6313273477637,
178.821287620784));
#22378=CARTESIAN_POINT('Ctrl Pts',(-59.2514873438827,-99.6626231910761,
179.995915399612));
#22379=CARTESIAN_POINT('Ctrl Pts',(-57.5897345813915,-99.7454959089947,
179.995915330104));
#22380=CARTESIAN_POINT('Ctrl Pts',(-55.9279818189004,-99.8283686269133,
179.995915260595));
#22381=CARTESIAN_POINT('Ctrl Pts',(-54.7500344295239,-99.8596644598054,
178.821287383467));
#22382=CARTESIAN_POINT('Ctrl Pts',(-53.5720870401475,-99.8909602926975,
177.646659506339));
#22383=CARTESIAN_POINT('Ctrl Pts',(-53.5621490463474,-99.7977385206737,
175.985484901271));
#22384=CARTESIAN_POINT('Ctrl Pts',(-53.5522110525473,-99.7045167486501,
174.324310296203));
#22385=CARTESIAN_POINT('Ctrl Pts',(-54.7102824138358,-99.4867773760269,
173.149682517375));
#22386=CARTESIAN_POINT('Ctrl Pts',(-55.8683537751243,-99.2690380034038,
171.975054738546));
#22387=CARTESIAN_POINT('Ctrl Pts',(-57.5102304117814,-98.9997217561745,
171.975054808055));
#22388=CARTESIAN_POINT('Ctrl Pts',(-59.1521070484385,-98.7304055089452,
171.975054877564));
#22389=CARTESIAN_POINT('Ctrl Pts',(-60.3101783119809,-98.5126661467424,
173.149682754692));
#22390=CARTESIAN_POINT('Ctrl Pts',(-61.4682495755234,-98.2949267845397,
174.32431063182));
#22391=CARTESIAN_POINT('Ctrl Pts',(-61.4583114434894,-98.2017050272526,
175.985485236888));
#22392=CARTESIAN_POINT('Ctrl Pts',(-61.4483733114555,-98.1084832699656,
177.646659841956));
#22393=CARTESIAN_POINT('Ctrl Pts',(-60.2704258243329,-98.139779113278,178.821287620784));
#22394=CARTESIAN_POINT('Ctrl Pts',(-59.0924783372104,-98.1710749565905,
179.995915399612));
#22395=CARTESIAN_POINT('Ctrl Pts',(-57.4307255747193,-98.2539476745091,
179.995915330104));
#22396=CARTESIAN_POINT('Ctrl Pts',(-55.7689728122282,-98.3368203924277,
179.995915260595));
#22397=CARTESIAN_POINT('Ctrl Pts',(-54.5910254228517,-98.3681162253198,
178.821287383467));
#22398=CARTESIAN_POINT('Ctrl Pts',(-56.1988062143188,-113.449542435949,
178.821287383467));
#22399=CARTESIAN_POINT('Ctrl Pts',(-55.0208588249424,-113.480838268841,
177.646659506339));
#22400=CARTESIAN_POINT('Ctrl Pts',(-55.0109208311422,-113.387616496817,
175.985484901271));
#22401=CARTESIAN_POINT('Ctrl Pts',(-55.0009828373422,-113.294394724794,
174.324310296203));
#22402=CARTESIAN_POINT('Ctrl Pts',(-56.1590541986307,-113.07665535217,173.149682517375));
#22403=CARTESIAN_POINT('Ctrl Pts',(-57.3171255599192,-112.858915979547,
171.975054738546));
#22404=CARTESIAN_POINT('Ctrl Pts',(-58.9590021965763,-112.589599732318,
171.975054808055));
#22405=CARTESIAN_POINT('Ctrl Pts',(-60.6008788332334,-112.320283485089,
171.975054877564));
#22406=CARTESIAN_POINT('Ctrl Pts',(-61.7589500967758,-112.102544122886,
173.149682754692));
#22407=CARTESIAN_POINT('Ctrl Pts',(-62.9170213603182,-111.884804760683,
174.32431063182));
#22408=CARTESIAN_POINT('Ctrl Pts',(-62.9070832282843,-111.791583003396,
175.985485236888));
#22409=CARTESIAN_POINT('Ctrl Pts',(-62.8971450962504,-111.698361246109,
177.646659841956));
#22410=CARTESIAN_POINT('Ctrl Pts',(-61.7191976091278,-111.729657089422,
178.821287620784));
#22411=CARTESIAN_POINT('Ctrl Pts',(-60.5412501220053,-111.760952932734,
179.995915399612));
#22412=CARTESIAN_POINT('Ctrl Pts',(-58.8794973595142,-111.843825650653,
179.995915330104));
#22413=CARTESIAN_POINT('Ctrl Pts',(-57.217744597023,-111.926698368571,179.995915260595));
#22414=CARTESIAN_POINT('Ctrl Pts',(-56.0397972076466,-111.957994201463,
178.821287383467));
#22415=CARTESIAN_POINT('Ctrl Pts',(-54.8618498182701,-111.989290034355,
177.646659506339));
#22416=CARTESIAN_POINT('Ctrl Pts',(-54.85191182447,-111.896068262332,175.985484901271));
#22417=CARTESIAN_POINT('Ctrl Pts',(-54.8419738306699,-111.802846490308,
174.324310296203));
#22418=CARTESIAN_POINT('Ctrl Pts',(-56.0000451919584,-111.585107117685,
173.149682517375));
#22419=CARTESIAN_POINT('Ctrl Pts',(-57.158116553247,-111.367367745062,171.975054738546));
#22420=CARTESIAN_POINT('Ctrl Pts',(-58.799993189904,-111.098051497832,171.975054808055));
#22421=CARTESIAN_POINT('Ctrl Pts',(-60.4418698265612,-110.828735250603,
171.975054877564));
#22422=CARTESIAN_POINT('Ctrl Pts',(-61.5999410901036,-110.6109958884,173.149682754692));
#22423=CARTESIAN_POINT('Ctrl Pts',(-62.758012353646,-110.393256526198,174.32431063182));
#22424=CARTESIAN_POINT('Ctrl Pts',(-62.7480742216121,-110.30003476891,175.985485236888));
#22425=CARTESIAN_POINT('Ctrl Pts',(-62.7381360895782,-110.206813011623,
177.646659841956));
#22426=CARTESIAN_POINT('Ctrl Pts',(-61.5601886024556,-110.238108854936,
178.821287620784));
#22427=CARTESIAN_POINT('Ctrl Pts',(-60.3822411153331,-110.269404698248,
179.995915399612));
#22428=CARTESIAN_POINT('Ctrl Pts',(-58.7204883528419,-110.352277416167,
179.995915330104));
#22429=CARTESIAN_POINT('Ctrl Pts',(-57.0587355903508,-110.435150134086,
179.995915260595));
#22430=CARTESIAN_POINT('Ctrl Pts',(-55.8807882009743,-110.466445966978,
178.821287383467));
#22431=CARTESIAN_POINT('Ctrl Pts',(-54.7028408115979,-110.49774179987,177.646659506339));
#22432=CARTESIAN_POINT('Ctrl Pts',(-54.6929028177978,-110.404520027846,
175.985484901271));
#22433=CARTESIAN_POINT('Ctrl Pts',(-54.6829648239977,-110.311298255822,
174.324310296203));
#22434=CARTESIAN_POINT('Ctrl Pts',(-55.8410361852862,-110.093558883199,
173.149682517375));
#22435=CARTESIAN_POINT('Ctrl Pts',(-56.9991075465747,-109.875819510576,
171.975054738546));
#22436=CARTESIAN_POINT('Ctrl Pts',(-58.6409841832318,-109.606503263347,
171.975054808055));
#22437=CARTESIAN_POINT('Ctrl Pts',(-60.2828608198889,-109.337187016117,
171.975054877564));
#22438=CARTESIAN_POINT('Ctrl Pts',(-61.4409320834313,-109.119447653915,
173.149682754692));
#22439=CARTESIAN_POINT('Ctrl Pts',(-62.5990033469738,-108.901708291712,
174.32431063182));
#22440=CARTESIAN_POINT('Ctrl Pts',(-62.5890652149398,-108.808486534425,
175.985485236888));
#22441=CARTESIAN_POINT('Ctrl Pts',(-62.5791270829059,-108.715264777138,
177.646659841956));
#22442=CARTESIAN_POINT('Ctrl Pts',(-61.4011795957834,-108.74656062045,178.821287620784));
#22443=CARTESIAN_POINT('Ctrl Pts',(-60.2232321086609,-108.777856463763,
179.995915399612));
#22444=CARTESIAN_POINT('Ctrl Pts',(-58.5614793461697,-108.860729181681,
179.995915330104));
#22445=CARTESIAN_POINT('Ctrl Pts',(-56.8997265836786,-108.9436018996,179.995915260595));
#22446=CARTESIAN_POINT('Ctrl Pts',(-55.7217791943021,-108.974897732492,
178.821287383467));
#22447=CARTESIAN_POINT('Ctrl Pts',(-54.5438318049257,-109.006193565384,
177.646659506339));
#22448=CARTESIAN_POINT('Ctrl Pts',(-54.5338938111256,-108.91297179336,175.985484901271));
#22449=CARTESIAN_POINT('Ctrl Pts',(-54.5239558173255,-108.819750021337,
174.324310296203));
#22450=CARTESIAN_POINT('Ctrl Pts',(-55.682027178614,-108.602010648714,173.149682517375));
#22451=CARTESIAN_POINT('Ctrl Pts',(-56.8400985399025,-108.384271276091,
171.975054738546));
#22452=CARTESIAN_POINT('Ctrl Pts',(-58.4819751765596,-108.114955028861,
171.975054808055));
#22453=CARTESIAN_POINT('Ctrl Pts',(-60.1238518132167,-107.845638781632,
171.975054877564));
#22454=CARTESIAN_POINT('Ctrl Pts',(-61.2819230767591,-107.627899419429,
173.149682754692));
#22455=CARTESIAN_POINT('Ctrl Pts',(-62.4399943403016,-107.410160057226,
174.32431063182));
#22456=CARTESIAN_POINT('Ctrl Pts',(-62.4300562082676,-107.316938299939,
175.985485236888));
#22457=CARTESIAN_POINT('Ctrl Pts',(-62.4201180762337,-107.223716542652,
177.646659841956));
#22458=CARTESIAN_POINT('Ctrl Pts',(-61.2421705891111,-107.255012385965,
178.821287620784));
#22459=CARTESIAN_POINT('Ctrl Pts',(-60.0642231019886,-107.286308229277,
179.995915399612));
#22460=CARTESIAN_POINT('Ctrl Pts',(-58.4024703394975,-107.369180947196,
179.995915330104));
#22461=CARTESIAN_POINT('Ctrl Pts',(-56.7407175770064,-107.452053665114,
179.995915260595));
#22462=CARTESIAN_POINT('Ctrl Pts',(-55.5627701876299,-107.483349498006,
178.821287383467));
#22463=CARTESIAN_POINT('Ctrl Pts',(-54.3848227982534,-107.514645330899,
177.646659506339));
#22464=CARTESIAN_POINT('Ctrl Pts',(-54.3748848044533,-107.421423558875,
175.985484901271));
#22465=CARTESIAN_POINT('Ctrl Pts',(-54.3649468106533,-107.328201786851,
174.324310296203));
#22466=CARTESIAN_POINT('Ctrl Pts',(-55.5230181719417,-107.110462414228,
173.149682517375));
#22467=CARTESIAN_POINT('Ctrl Pts',(-56.6810895332303,-106.892723041605,
171.975054738546));
#22468=CARTESIAN_POINT('Ctrl Pts',(-58.3229661698874,-106.623406794376,
171.975054808055));
#22469=CARTESIAN_POINT('Ctrl Pts',(-59.9648428065445,-106.354090547146,
171.975054877564));
#22470=CARTESIAN_POINT('Ctrl Pts',(-61.1229140700869,-106.136351184943,
173.149682754692));
#22471=CARTESIAN_POINT('Ctrl Pts',(-62.2809853336293,-105.918611822741,
174.32431063182));
#22472=CARTESIAN_POINT('Ctrl Pts',(-62.2710472015954,-105.825390065454,
175.985485236888));
#22473=CARTESIAN_POINT('Ctrl Pts',(-62.2611090695615,-105.732168308167,
177.646659841956));
#22474=CARTESIAN_POINT('Ctrl Pts',(-61.0831615824389,-105.763464151479,
178.821287620784));
#22475=CARTESIAN_POINT('Ctrl Pts',(-59.9052140953164,-105.794759994792,
179.995915399612));
#22476=CARTESIAN_POINT('Ctrl Pts',(-58.2434613328252,-105.87763271271,179.995915330104));
#22477=CARTESIAN_POINT('Ctrl Pts',(-56.5817085703341,-105.960505430629,
179.995915260595));
#22478=CARTESIAN_POINT('Ctrl Pts',(-55.4037611809577,-105.991801263521,
178.821287383467));
#22479=CARTESIAN_POINT('Ctrl Pts',(-54.2258137915812,-106.023097096413,
177.646659506339));
#22480=CARTESIAN_POINT('Ctrl Pts',(-54.2158757977811,-105.929875324389,
175.985484901271));
#22481=CARTESIAN_POINT('Ctrl Pts',(-54.205937803981,-105.836653552366,174.324310296203));
#22482=CARTESIAN_POINT('Ctrl Pts',(-55.3640091652695,-105.618914179742,
173.149682517375));
#22483=CARTESIAN_POINT('Ctrl Pts',(-56.522080526558,-105.401174807119,171.975054738546));
#22484=CARTESIAN_POINT('Ctrl Pts',(-58.1639571632151,-105.13185855989,171.975054808055));
#22485=CARTESIAN_POINT('Ctrl Pts',(-59.8058337998722,-104.862542312661,
171.975054877564));
#22486=CARTESIAN_POINT('Ctrl Pts',(-60.9639050634147,-104.644802950458,
173.149682754692));
#22487=CARTESIAN_POINT('Ctrl Pts',(-62.1219763269571,-104.427063588255,
174.32431063182));
#22488=CARTESIAN_POINT('Ctrl Pts',(-62.1120381949232,-104.333841830968,
175.985485236888));
#22489=CARTESIAN_POINT('Ctrl Pts',(-62.1021000628892,-104.240620073681,
177.646659841956));
#22490=CARTESIAN_POINT('Ctrl Pts',(-60.9241525757667,-104.271915916993,
178.821287620784));
#22491=CARTESIAN_POINT('Ctrl Pts',(-59.7462050886442,-104.303211760306,
179.995915399612));
#22492=CARTESIAN_POINT('Ctrl Pts',(-58.084452326153,-104.386084478225,179.995915330104));
#22493=CARTESIAN_POINT('Ctrl Pts',(-56.4226995636619,-104.468957196143,
179.995915260595));
#22494=CARTESIAN_POINT('Ctrl Pts',(-55.2447521742854,-104.500253029035,
178.821287383467));
#22495=CARTESIAN_POINT('Ctrl Pts',(-54.066804784909,-104.531548861927,177.646659506339));
#22496=CARTESIAN_POINT('Ctrl Pts',(-54.0568667911089,-104.438327089904,
175.985484901271));
#22497=CARTESIAN_POINT('Ctrl Pts',(-54.0469287973088,-104.34510531788,174.324310296203));
#22498=CARTESIAN_POINT('Ctrl Pts',(-55.2050001585973,-104.127365945257,
173.149682517375));
#22499=CARTESIAN_POINT('Ctrl Pts',(-56.3630715198858,-103.909626572634,
171.975054738546));
#22500=CARTESIAN_POINT('Ctrl Pts',(-58.0049481565429,-103.640310325404,
171.975054808055));
#22501=CARTESIAN_POINT('Ctrl Pts',(-59.6468247932,-103.370994078175,171.975054877564));
#22502=CARTESIAN_POINT('Ctrl Pts',(-60.8048960567424,-103.153254715972,
173.149682754692));
#22503=CARTESIAN_POINT('Ctrl Pts',(-61.9629673202849,-102.93551535377,174.32431063182));
#22504=CARTESIAN_POINT('Ctrl Pts',(-61.9530291882509,-102.842293596483,
175.985485236888));
#22505=CARTESIAN_POINT('Ctrl Pts',(-61.943091056217,-102.749071839196,177.646659841956));
#22506=CARTESIAN_POINT('Ctrl Pts',(-60.7651435690945,-102.780367682508,
178.821287620784));
#22507=CARTESIAN_POINT('Ctrl Pts',(-59.587196081972,-102.81166352582,179.995915399612));
#22508=CARTESIAN_POINT('Ctrl Pts',(-57.9254433194808,-102.894536243739,
179.995915330104));
#22509=CARTESIAN_POINT('Ctrl Pts',(-56.2636905569897,-102.977408961658,
179.995915260595));
#22510=CARTESIAN_POINT('Ctrl Pts',(-55.0857431676132,-103.00870479455,178.821287383467));
#22511=CARTESIAN_POINT('Ctrl Pts',(-53.9077957782368,-103.040000627442,
177.646659506339));
#22512=CARTESIAN_POINT('Ctrl Pts',(-53.8978577844367,-102.946778855418,
175.985484901271));
#22513=CARTESIAN_POINT('Ctrl Pts',(-53.8879197906366,-102.853557083394,
174.324310296203));
#22514=CARTESIAN_POINT('Ctrl Pts',(-55.0459911519251,-102.635817710771,
173.149682517375));
#22515=CARTESIAN_POINT('Ctrl Pts',(-56.2040625132136,-102.418078338148,
171.975054738546));
#22516=CARTESIAN_POINT('Ctrl Pts',(-57.8459391498707,-102.148762090919,
171.975054808055));
#22517=CARTESIAN_POINT('Ctrl Pts',(-59.4878157865278,-101.879445843689,
171.975054877564));
#22518=CARTESIAN_POINT('Ctrl Pts',(-60.6458870500702,-101.661706481487,
173.149682754692));
#22519=CARTESIAN_POINT('Ctrl Pts',(-61.8039583136126,-101.443967119284,
174.32431063182));
#22520=CARTESIAN_POINT('Ctrl Pts',(-61.7940201815787,-101.350745361997,
175.985485236888));
#22521=CARTESIAN_POINT('Ctrl Pts',(-61.7840820495448,-101.25752360471,177.646659841956));
#22522=CARTESIAN_POINT('Ctrl Pts',(-60.6061345624222,-101.288819448022,
178.821287620784));
#22523=CARTESIAN_POINT('Ctrl Pts',(-59.4281870752997,-101.320115291335,
179.995915399612));
#22524=CARTESIAN_POINT('Ctrl Pts',(-57.7664343128086,-101.402988009253,
179.995915330104));
#22525=CARTESIAN_POINT('Ctrl Pts',(-56.1046815503175,-101.485860727172,
179.995915260595));
#22526=CARTESIAN_POINT('Ctrl Pts',(-54.926734160941,-101.517156560064,178.821287383467));
#22527=CARTESIAN_POINT('Ctrl Pts',(-53.7487867715645,-101.548452392956,
177.646659506339));
#22528=CARTESIAN_POINT('Ctrl Pts',(-53.7388487777644,-101.455230620932,
175.985484901271));
#22529=CARTESIAN_POINT('Ctrl Pts',(-53.7289107839643,-101.362008848909,
174.324310296203));
#22530=CARTESIAN_POINT('Ctrl Pts',(-54.8869821452528,-101.144269476286,
173.149682517375));
#22531=CARTESIAN_POINT('Ctrl Pts',(-56.0450535065414,-100.926530103662,
171.975054738546));
#22532=CARTESIAN_POINT('Ctrl Pts',(-57.6869301431984,-100.657213856433,
171.975054808055));
#22533=CARTESIAN_POINT('Ctrl Pts',(-59.3288067798556,-100.387897609204,
171.975054877564));
#22534=CARTESIAN_POINT('Ctrl Pts',(-60.486878043398,-100.170158247001,173.149682754692));
#22535=CARTESIAN_POINT('Ctrl Pts',(-61.6449493069404,-99.9524188847983,
174.32431063182));
#22536=CARTESIAN_POINT('Ctrl Pts',(-61.6350111749065,-99.8591971275113,
175.985485236888));
#22537=CARTESIAN_POINT('Ctrl Pts',(-61.6250730428726,-99.7659753702243,
177.646659841956));
#22538=CARTESIAN_POINT('Ctrl Pts',(-60.44712555575,-99.7972712135367,178.821287620784));
#22539=CARTESIAN_POINT('Ctrl Pts',(-59.2691780686275,-99.8285670568492,
179.995915399612));
#22540=CARTESIAN_POINT('Ctrl Pts',(-57.6074253061363,-99.9114397747677,
179.995915330104));
#22541=CARTESIAN_POINT('Ctrl Pts',(-55.9456725436452,-99.9943124926864,
179.995915260595));
#22542=CARTESIAN_POINT('Ctrl Pts',(-54.7677251542687,-100.025608325578,
178.821287383467));
#22543=CARTESIAN_POINT('Ctrl Pts',(-53.5897777648923,-100.05690415847,177.646659506339));
#22544=CARTESIAN_POINT('Ctrl Pts',(-53.5798397710922,-99.9636823864468,
175.985484901271));
#22545=CARTESIAN_POINT('Ctrl Pts',(-53.5699017772921,-99.8704606144232,
174.324310296203));
#22546=CARTESIAN_POINT('Ctrl Pts',(-54.7279731385806,-99.6527212418,173.149682517375));
#22547=CARTESIAN_POINT('Ctrl Pts',(-55.8860444998691,-99.4349818691769,
171.975054738546));
#22548=CARTESIAN_POINT('Ctrl Pts',(-57.5279211365262,-99.1656656219475,
171.975054808055));
#22549=CARTESIAN_POINT('Ctrl Pts',(-59.1697977731833,-98.8963493747183,
171.975054877564));
#22550=CARTESIAN_POINT('Ctrl Pts',(-60.3278690367257,-98.6786100125155,
173.149682754692));
#22551=CARTESIAN_POINT('Ctrl Pts',(-61.4859403002682,-98.4608706503128,
174.32431063182));
#22552=CARTESIAN_POINT('Ctrl Pts',(-61.4760021682342,-98.3676488930257,
175.985485236888));
#22553=CARTESIAN_POINT('Ctrl Pts',(-61.4660640362003,-98.2744271357387,
177.646659841956));
#22554=CARTESIAN_POINT('Ctrl Pts',(-60.2881165490778,-98.3057229790511,
178.821287620784));
#22555=CARTESIAN_POINT('Ctrl Pts',(-59.1101690619552,-98.3370188223636,
179.995915399612));
#22556=CARTESIAN_POINT('Ctrl Pts',(-57.4484162994641,-98.4198915402821,
179.995915330104));
#22557=CARTESIAN_POINT('Ctrl Pts',(-55.786663536973,-98.5027642582008,179.995915260595));
#22558=CARTESIAN_POINT('Ctrl Pts',(-54.6087161475965,-98.5340600910929,
178.821287383467));
#22559=CARTESIAN_POINT('Ctrl Pts',(-56.2237961054143,-113.614380048479,
178.813912075476));
#22560=CARTESIAN_POINT('Ctrl Pts',(-55.0488864554725,-113.645352038053,
177.6423391512));
#22561=CARTESIAN_POINT('Ctrl Pts',(-55.0389484614927,-113.552130266048,
175.985484901707));
#22562=CARTESIAN_POINT('Ctrl Pts',(-55.0290104675128,-113.458908494044,
174.328630652215));
#22563=CARTESIAN_POINT('Ctrl Pts',(-56.1840440891124,-113.241492964766,
173.157057825983));
#22564=CARTESIAN_POINT('Ctrl Pts',(-57.3390777107121,-113.024077435489,
171.985484999752));
#22565=CARTESIAN_POINT('Ctrl Pts',(-58.9766583348819,-112.755219171892,
171.985485069079));
#22566=CARTESIAN_POINT('Ctrl Pts',(-60.6142389590518,-112.486360908295,
171.985485138407));
#22567=CARTESIAN_POINT('Ctrl Pts',(-61.7692724831595,-112.268945389411,
173.157058062683));
#22568=CARTESIAN_POINT('Ctrl Pts',(-62.9243060072673,-112.051529870527,
174.328630986959));
#22569=CARTESIAN_POINT('Ctrl Pts',(-62.9143678754131,-111.95830811322,175.985485236451));
#22570=CARTESIAN_POINT('Ctrl Pts',(-62.9044297435589,-111.865086355914,
177.642339485944));
#22571=CARTESIAN_POINT('Ctrl Pts',(-61.7295199961253,-111.896058355881,
178.813912312176));
#22572=CARTESIAN_POINT('Ctrl Pts',(-60.5546102486917,-111.927030355848,
179.985485138407));
#22573=CARTESIAN_POINT('Ctrl Pts',(-58.8971534986878,-112.009445090134,
179.985485069079));
#22574=CARTESIAN_POINT('Ctrl Pts',(-57.2396967486839,-112.09185982442,179.985484999752));
#22575=CARTESIAN_POINT('Ctrl Pts',(-56.0647870987421,-112.122831813994,
178.813912075476));
#22576=CARTESIAN_POINT('Ctrl Pts',(-54.8898774488003,-112.153803803567,
177.6423391512));
#22577=CARTESIAN_POINT('Ctrl Pts',(-54.8799394548205,-112.060582031563,
175.985484901707));
#22578=CARTESIAN_POINT('Ctrl Pts',(-54.8700014608406,-111.967360259558,
174.328630652215));
#22579=CARTESIAN_POINT('Ctrl Pts',(-56.0250350824402,-111.749944730281,
173.157057825983));
#22580=CARTESIAN_POINT('Ctrl Pts',(-57.1800687040398,-111.532529201003,
171.985484999752));
#22581=CARTESIAN_POINT('Ctrl Pts',(-58.8176493282097,-111.263670937406,
171.985485069079));
#22582=CARTESIAN_POINT('Ctrl Pts',(-60.4552299523796,-110.994812673809,
171.985485138407));
#22583=CARTESIAN_POINT('Ctrl Pts',(-61.6102634764873,-110.777397154925,
173.157058062683));
#22584=CARTESIAN_POINT('Ctrl Pts',(-62.7652970005951,-110.559981636041,
174.328630986959));
#22585=CARTESIAN_POINT('Ctrl Pts',(-62.7553588687409,-110.466759878735,
175.985485236451));
#22586=CARTESIAN_POINT('Ctrl Pts',(-62.7454207368867,-110.373538121429,
177.642339485944));
#22587=CARTESIAN_POINT('Ctrl Pts',(-61.5705109894531,-110.404510121395,
178.813912312176));
#22588=CARTESIAN_POINT('Ctrl Pts',(-60.3956012420194,-110.435482121362,
179.985485138407));
#22589=CARTESIAN_POINT('Ctrl Pts',(-58.7381444920155,-110.517896855648,
179.985485069079));
#22590=CARTESIAN_POINT('Ctrl Pts',(-57.0806877420116,-110.600311589935,
179.985484999752));
#22591=CARTESIAN_POINT('Ctrl Pts',(-55.9057780920699,-110.631283579508,
178.813912075476));
#22592=CARTESIAN_POINT('Ctrl Pts',(-54.7308684421281,-110.662255569082,
177.6423391512));
#22593=CARTESIAN_POINT('Ctrl Pts',(-54.7209304481482,-110.569033797077,
175.985484901707));
#22594=CARTESIAN_POINT('Ctrl Pts',(-54.7109924541684,-110.475812025073,
174.328630652215));
#22595=CARTESIAN_POINT('Ctrl Pts',(-55.866026075768,-110.258396495795,173.157057825983));
#22596=CARTESIAN_POINT('Ctrl Pts',(-57.0210596973676,-110.040980966518,
171.985484999752));
#22597=CARTESIAN_POINT('Ctrl Pts',(-58.6586403215375,-109.772122702921,
171.985485069079));
#22598=CARTESIAN_POINT('Ctrl Pts',(-60.2962209457073,-109.503264439324,
171.985485138407));
#22599=CARTESIAN_POINT('Ctrl Pts',(-61.4512544698151,-109.28584892044,173.157058062683));
#22600=CARTESIAN_POINT('Ctrl Pts',(-62.6062879939228,-109.068433401555,
174.328630986959));
#22601=CARTESIAN_POINT('Ctrl Pts',(-62.5963498620687,-108.975211644249,
175.985485236451));
#22602=CARTESIAN_POINT('Ctrl Pts',(-62.5864117302145,-108.881989886943,
177.642339485944));
#22603=CARTESIAN_POINT('Ctrl Pts',(-61.4115019827808,-108.91296188691,178.813912312176));
#22604=CARTESIAN_POINT('Ctrl Pts',(-60.2365922353472,-108.943933886877,
179.985485138407));
#22605=CARTESIAN_POINT('Ctrl Pts',(-58.5791354853433,-109.026348621163,
179.985485069079));
#22606=CARTESIAN_POINT('Ctrl Pts',(-56.9216787353394,-109.108763355449,
179.985484999752));
#22607=CARTESIAN_POINT('Ctrl Pts',(-55.7467690853976,-109.139735345023,
178.813912075476));
#22608=CARTESIAN_POINT('Ctrl Pts',(-54.5718594354559,-109.170707334596,
177.6423391512));
#22609=CARTESIAN_POINT('Ctrl Pts',(-54.561921441476,-109.077485562592,175.985484901707));
#22610=CARTESIAN_POINT('Ctrl Pts',(-54.5519834474962,-108.984263790587,
174.328630652215));
#22611=CARTESIAN_POINT('Ctrl Pts',(-55.7070170690958,-108.76684826131,173.157057825983));
#22612=CARTESIAN_POINT('Ctrl Pts',(-56.8620506906954,-108.549432732032,
171.985484999752));
#22613=CARTESIAN_POINT('Ctrl Pts',(-58.4996313148652,-108.280574468435,
171.985485069079));
#22614=CARTESIAN_POINT('Ctrl Pts',(-60.1372119390351,-108.011716204838,
171.985485138407));
#22615=CARTESIAN_POINT('Ctrl Pts',(-61.2922454631428,-107.794300685954,
173.157058062683));
#22616=CARTESIAN_POINT('Ctrl Pts',(-62.4472789872506,-107.57688516707,174.328630986959));
#22617=CARTESIAN_POINT('Ctrl Pts',(-62.4373408553964,-107.483663409764,
175.985485236451));
#22618=CARTESIAN_POINT('Ctrl Pts',(-62.4274027235423,-107.390441652457,
177.642339485944));
#22619=CARTESIAN_POINT('Ctrl Pts',(-61.2524929761086,-107.421413652424,
178.813912312176));
#22620=CARTESIAN_POINT('Ctrl Pts',(-60.077583228675,-107.452385652391,179.985485138407));
#22621=CARTESIAN_POINT('Ctrl Pts',(-58.4201264786711,-107.534800386677,
179.985485069079));
#22622=CARTESIAN_POINT('Ctrl Pts',(-56.7626697286672,-107.617215120964,
179.985484999752));
#22623=CARTESIAN_POINT('Ctrl Pts',(-55.5877600787254,-107.648187110537,
178.813912075476));
#22624=CARTESIAN_POINT('Ctrl Pts',(-54.4128504287836,-107.67915910011,177.6423391512));
#22625=CARTESIAN_POINT('Ctrl Pts',(-54.4029124348038,-107.585937328106,
175.985484901707));
#22626=CARTESIAN_POINT('Ctrl Pts',(-54.3929744408239,-107.492715556102,
174.328630652215));
#22627=CARTESIAN_POINT('Ctrl Pts',(-55.5480080624235,-107.275300026824,
173.157057825983));
#22628=CARTESIAN_POINT('Ctrl Pts',(-56.7030416840231,-107.057884497547,
171.985484999752));
#22629=CARTESIAN_POINT('Ctrl Pts',(-58.340622308193,-106.78902623395,171.985485069079));
#22630=CARTESIAN_POINT('Ctrl Pts',(-59.9782029323629,-106.520167970353,
171.985485138407));
#22631=CARTESIAN_POINT('Ctrl Pts',(-61.1332364564706,-106.302752451468,
173.157058062683));
#22632=CARTESIAN_POINT('Ctrl Pts',(-62.2882699805784,-106.085336932584,
174.328630986959));
#22633=CARTESIAN_POINT('Ctrl Pts',(-62.2783318487242,-105.992115175278,
175.985485236451));
#22634=CARTESIAN_POINT('Ctrl Pts',(-62.26839371687,-105.898893417972,177.642339485944));
#22635=CARTESIAN_POINT('Ctrl Pts',(-61.0934839694364,-105.929865417939,
178.813912312176));
#22636=CARTESIAN_POINT('Ctrl Pts',(-59.9185742220028,-105.960837417905,
179.985485138407));
#22637=CARTESIAN_POINT('Ctrl Pts',(-58.2611174719989,-106.043252152192,
179.985485069079));
#22638=CARTESIAN_POINT('Ctrl Pts',(-56.603660721995,-106.125666886478,179.985484999752));
#22639=CARTESIAN_POINT('Ctrl Pts',(-55.4287510720532,-106.156638876051,
178.813912075476));
#22640=CARTESIAN_POINT('Ctrl Pts',(-54.2538414221114,-106.187610865625,
177.6423391512));
#22641=CARTESIAN_POINT('Ctrl Pts',(-54.2439034281315,-106.09438909362,175.985484901707));
#22642=CARTESIAN_POINT('Ctrl Pts',(-54.2339654341517,-106.001167321616,
174.328630652215));
#22643=CARTESIAN_POINT('Ctrl Pts',(-55.3889990557513,-105.783751792338,
173.157057825983));
#22644=CARTESIAN_POINT('Ctrl Pts',(-56.5440326773509,-105.566336263061,
171.985484999752));
#22645=CARTESIAN_POINT('Ctrl Pts',(-58.1816133015208,-105.297477999464,
171.985485069079));
#22646=CARTESIAN_POINT('Ctrl Pts',(-59.8191939256906,-105.028619735867,
171.985485138407));
#22647=CARTESIAN_POINT('Ctrl Pts',(-60.9742274497984,-104.811204216983,
173.157058062683));
#22648=CARTESIAN_POINT('Ctrl Pts',(-62.1292609739061,-104.593788698099,
174.328630986959));
#22649=CARTESIAN_POINT('Ctrl Pts',(-62.119322842052,-104.500566940792,175.985485236451));
#22650=CARTESIAN_POINT('Ctrl Pts',(-62.1093847101978,-104.407345183486,
177.642339485944));
#22651=CARTESIAN_POINT('Ctrl Pts',(-60.9344749627642,-104.438317183453,
178.813912312176));
#22652=CARTESIAN_POINT('Ctrl Pts',(-59.7595652153305,-104.46928918342,179.985485138407));
#22653=CARTESIAN_POINT('Ctrl Pts',(-58.1021084653266,-104.551703917706,
179.985485069079));
#22654=CARTESIAN_POINT('Ctrl Pts',(-56.4446517153227,-104.634118651992,
179.985484999752));
#22655=CARTESIAN_POINT('Ctrl Pts',(-55.269742065381,-104.665090641566,178.813912075476));
#22656=CARTESIAN_POINT('Ctrl Pts',(-54.0948324154392,-104.696062631139,
177.6423391512));
#22657=CARTESIAN_POINT('Ctrl Pts',(-54.0848944214593,-104.602840859135,
175.985484901707));
#22658=CARTESIAN_POINT('Ctrl Pts',(-54.0749564274795,-104.50961908713,174.328630652215));
#22659=CARTESIAN_POINT('Ctrl Pts',(-55.2299900490791,-104.292203557853,
173.157057825983));
#22660=CARTESIAN_POINT('Ctrl Pts',(-56.3850236706787,-104.074788028575,
171.985484999752));
#22661=CARTESIAN_POINT('Ctrl Pts',(-58.0226042948486,-103.805929764978,
171.985485069079));
#22662=CARTESIAN_POINT('Ctrl Pts',(-59.6601849190184,-103.537071501381,
171.985485138407));
#22663=CARTESIAN_POINT('Ctrl Pts',(-60.8152184431262,-103.319655982497,
173.157058062683));
#22664=CARTESIAN_POINT('Ctrl Pts',(-61.9702519672339,-103.102240463613,
174.328630986959));
#22665=CARTESIAN_POINT('Ctrl Pts',(-61.9603138353797,-103.009018706307,
175.985485236451));
#22666=CARTESIAN_POINT('Ctrl Pts',(-61.9503757035256,-102.915796949001,
177.642339485944));
#22667=CARTESIAN_POINT('Ctrl Pts',(-60.7754659560919,-102.946768948967,
178.813912312176));
#22668=CARTESIAN_POINT('Ctrl Pts',(-59.6005562086583,-102.977740948934,
179.985485138407));
#22669=CARTESIAN_POINT('Ctrl Pts',(-57.9430994586544,-103.06015568322,179.985485069079));
#22670=CARTESIAN_POINT('Ctrl Pts',(-56.2856427086505,-103.142570417507,
179.985484999752));
#22671=CARTESIAN_POINT('Ctrl Pts',(-55.1107330587087,-103.17354240708,178.813912075476));
#22672=CARTESIAN_POINT('Ctrl Pts',(-53.935823408767,-103.204514396654,177.6423391512));
#22673=CARTESIAN_POINT('Ctrl Pts',(-53.9258854147871,-103.111292624649,
175.985484901707));
#22674=CARTESIAN_POINT('Ctrl Pts',(-53.9159474208072,-103.018070852645,
174.328630652215));
#22675=CARTESIAN_POINT('Ctrl Pts',(-55.0709810424069,-102.800655323367,
173.157057825983));
#22676=CARTESIAN_POINT('Ctrl Pts',(-56.2260146640065,-102.58323979409,171.985484999752));
#22677=CARTESIAN_POINT('Ctrl Pts',(-57.8635952881763,-102.314381530493,
171.985485069079));
#22678=CARTESIAN_POINT('Ctrl Pts',(-59.5011759123462,-102.045523266896,
171.985485138407));
#22679=CARTESIAN_POINT('Ctrl Pts',(-60.6562094364539,-101.828107748012,
173.157058062683));
#22680=CARTESIAN_POINT('Ctrl Pts',(-61.8112429605617,-101.610692229127,
174.328630986959));
#22681=CARTESIAN_POINT('Ctrl Pts',(-61.8013048287075,-101.517470471821,
175.985485236451));
#22682=CARTESIAN_POINT('Ctrl Pts',(-61.7913666968533,-101.424248714515,
177.642339485944));
#22683=CARTESIAN_POINT('Ctrl Pts',(-60.6164569494197,-101.455220714482,
178.813912312176));
#22684=CARTESIAN_POINT('Ctrl Pts',(-59.4415472019861,-101.486192714449,
179.985485138407));
#22685=CARTESIAN_POINT('Ctrl Pts',(-57.7840904519822,-101.568607448735,
179.985485069079));
#22686=CARTESIAN_POINT('Ctrl Pts',(-56.1266337019783,-101.651022183021,
179.985484999752));
#22687=CARTESIAN_POINT('Ctrl Pts',(-54.9517240520365,-101.681994172595,
178.813912075476));
#22688=CARTESIAN_POINT('Ctrl Pts',(-53.7768144020947,-101.712966162168,
177.6423391512));
#22689=CARTESIAN_POINT('Ctrl Pts',(-53.7668764081149,-101.619744390164,
175.985484901707));
#22690=CARTESIAN_POINT('Ctrl Pts',(-53.756938414135,-101.526522618159,174.328630652215));
#22691=CARTESIAN_POINT('Ctrl Pts',(-54.9119720357346,-101.309107088882,
173.157057825983));
#22692=CARTESIAN_POINT('Ctrl Pts',(-56.0670056573342,-101.091691559604,
171.985484999752));
#22693=CARTESIAN_POINT('Ctrl Pts',(-57.7045862815041,-100.822833296007,
171.985485069079));
#22694=CARTESIAN_POINT('Ctrl Pts',(-59.342166905674,-100.55397503241,171.985485138407));
#22695=CARTESIAN_POINT('Ctrl Pts',(-60.4972004297817,-100.336559513526,
173.157058062683));
#22696=CARTESIAN_POINT('Ctrl Pts',(-61.6522339538895,-100.119143994642,
174.328630986959));
#22697=CARTESIAN_POINT('Ctrl Pts',(-61.6422958220353,-100.025922237336,
175.985485236451));
#22698=CARTESIAN_POINT('Ctrl Pts',(-61.6323576901811,-99.9327004800294,
177.642339485944));
#22699=CARTESIAN_POINT('Ctrl Pts',(-60.4574479427475,-99.9636724799962,
178.813912312176));
#22700=CARTESIAN_POINT('Ctrl Pts',(-59.2825381953138,-99.994644479963,179.985485138407));
#22701=CARTESIAN_POINT('Ctrl Pts',(-57.6250814453099,-100.077059214249,
179.985485069079));
#22702=CARTESIAN_POINT('Ctrl Pts',(-55.9676246953061,-100.159473948536,
179.985484999752));
#22703=CARTESIAN_POINT('Ctrl Pts',(-54.7927150453643,-100.190445938109,
178.813912075476));
#22704=CARTESIAN_POINT('Ctrl Pts',(-53.6178053954225,-100.221417927683,
177.6423391512));
#22705=CARTESIAN_POINT('Ctrl Pts',(-53.6078674014426,-100.128196155678,
175.985484901707));
#22706=CARTESIAN_POINT('Ctrl Pts',(-53.5979294074628,-100.034974383673,
174.328630652215));
#22707=CARTESIAN_POINT('Ctrl Pts',(-54.7529630290624,-99.817558854396,173.157057825983));
#22708=CARTESIAN_POINT('Ctrl Pts',(-55.907996650662,-99.6001433251185,171.985484999752));
#22709=CARTESIAN_POINT('Ctrl Pts',(-57.5455772748319,-99.3312850615215,
171.985485069079));
#22710=CARTESIAN_POINT('Ctrl Pts',(-59.1831578990017,-99.0624267979246,
171.985485138407));
#22711=CARTESIAN_POINT('Ctrl Pts',(-60.3381914231095,-98.8450112790404,
173.157058062683));
#22712=CARTESIAN_POINT('Ctrl Pts',(-61.4932249472172,-98.6275957601562,
174.328630986959));
#22713=CARTESIAN_POINT('Ctrl Pts',(-61.4832868153631,-98.53437400285,175.985485236451));
#22714=CARTESIAN_POINT('Ctrl Pts',(-61.4733486835089,-98.4411522455438,
177.642339485944));
#22715=CARTESIAN_POINT('Ctrl Pts',(-60.2984389360752,-98.4721242455106,
178.813912312176));
#22716=CARTESIAN_POINT('Ctrl Pts',(-59.1235291886416,-98.5030962454774,
179.985485138407));
#22717=CARTESIAN_POINT('Ctrl Pts',(-57.4660724386377,-98.5855109797636,
179.985485069079));
#22718=CARTESIAN_POINT('Ctrl Pts',(-55.8086156886338,-98.6679257140499,
179.985484999752));
#22719=CARTESIAN_POINT('Ctrl Pts',(-54.633706038692,-98.6988977036234,178.813912075476));
#22720=CARTESIAN_POINT('Ctrl Pts',(-56.1707931031902,-113.117197303651,
178.813912075476));
#22721=CARTESIAN_POINT('Ctrl Pts',(-54.9958834532485,-113.148169293224,
177.6423391512));
#22722=CARTESIAN_POINT('Ctrl Pts',(-54.9859454592686,-113.05494752122,175.985484901707));
#22723=CARTESIAN_POINT('Ctrl Pts',(-54.9760074652888,-112.961725749215,
174.328630652215));
#22724=CARTESIAN_POINT('Ctrl Pts',(-56.1310410868884,-112.744310219938,
173.157057825983));
#22725=CARTESIAN_POINT('Ctrl Pts',(-57.286074708488,-112.52689469066,171.985484999752));
#22726=CARTESIAN_POINT('Ctrl Pts',(-58.9236553326578,-112.258036427063,
171.985485069079));
#22727=CARTESIAN_POINT('Ctrl Pts',(-60.5612359568277,-111.989178163466,
171.985485138407));
#22728=CARTESIAN_POINT('Ctrl Pts',(-61.7162694809355,-111.771762644582,
173.157058062683));
#22729=CARTESIAN_POINT('Ctrl Pts',(-62.8713030050432,-111.554347125698,
174.328630986959));
#22730=CARTESIAN_POINT('Ctrl Pts',(-62.861364873189,-111.461125368392,175.985485236451));
#22731=CARTESIAN_POINT('Ctrl Pts',(-62.8514267413349,-111.367903611086,
177.642339485944));
#22732=CARTESIAN_POINT('Ctrl Pts',(-61.6765169939012,-111.398875611052,
178.813912312176));
#22733=CARTESIAN_POINT('Ctrl Pts',(-60.5016072464676,-111.429847611019,
179.985485138407));
#22734=CARTESIAN_POINT('Ctrl Pts',(-58.8441504964637,-111.512262345305,
179.985485069079));
#22735=CARTESIAN_POINT('Ctrl Pts',(-57.1866937464598,-111.594677079592,
179.985484999752));
#22736=CARTESIAN_POINT('Ctrl Pts',(-56.011784096518,-111.625649069165,178.813912075476));
#22737=CARTESIAN_POINT('Ctrl Pts',(-54.8368744465763,-111.656621058739,
177.6423391512));
#22738=CARTESIAN_POINT('Ctrl Pts',(-54.8269364525964,-111.563399286734,
175.985484901707));
#22739=CARTESIAN_POINT('Ctrl Pts',(-54.8169984586165,-111.47017751473,174.328630652215));
#22740=CARTESIAN_POINT('Ctrl Pts',(-55.9720320802161,-111.252761985452,
173.157057825983));
#22741=CARTESIAN_POINT('Ctrl Pts',(-57.1270657018158,-111.035346456175,
171.985484999752));
#22742=CARTESIAN_POINT('Ctrl Pts',(-58.7646463259856,-110.766488192578,
171.985485069079));
#22743=CARTESIAN_POINT('Ctrl Pts',(-60.4022269501555,-110.497629928981,
171.985485138407));
#22744=CARTESIAN_POINT('Ctrl Pts',(-61.5572604742632,-110.280214410097,
173.157058062683));
#22745=CARTESIAN_POINT('Ctrl Pts',(-62.712293998371,-110.062798891212,174.328630986959));
#22746=CARTESIAN_POINT('Ctrl Pts',(-62.7023558665168,-109.969577133906,
175.985485236451));
#22747=CARTESIAN_POINT('Ctrl Pts',(-62.6924177346626,-109.8763553766,177.642339485944));
#22748=CARTESIAN_POINT('Ctrl Pts',(-61.517507987229,-109.907327376567,178.813912312176));
#22749=CARTESIAN_POINT('Ctrl Pts',(-60.3425982397954,-109.938299376534,
179.985485138407));
#22750=CARTESIAN_POINT('Ctrl Pts',(-58.6851414897915,-110.02071411082,179.985485069079));
#22751=CARTESIAN_POINT('Ctrl Pts',(-57.0276847397876,-110.103128845106,
179.985484999752));
#22752=CARTESIAN_POINT('Ctrl Pts',(-55.8527750898458,-110.13410083468,178.813912075476));
#22753=CARTESIAN_POINT('Ctrl Pts',(-54.677865439904,-110.165072824253,177.6423391512));
#22754=CARTESIAN_POINT('Ctrl Pts',(-54.6679274459242,-110.071851052249,
175.985484901707));
#22755=CARTESIAN_POINT('Ctrl Pts',(-54.6579894519443,-109.978629280244,
174.328630652215));
#22756=CARTESIAN_POINT('Ctrl Pts',(-55.8130230735439,-109.761213750967,
173.157057825983));
#22757=CARTESIAN_POINT('Ctrl Pts',(-56.9680566951435,-109.543798221689,
171.985484999752));
#22758=CARTESIAN_POINT('Ctrl Pts',(-58.6056373193134,-109.274939958092,
171.985485069079));
#22759=CARTESIAN_POINT('Ctrl Pts',(-60.2432179434833,-109.006081694495,
171.985485138407));
#22760=CARTESIAN_POINT('Ctrl Pts',(-61.398251467591,-108.788666175611,173.157058062683));
#22761=CARTESIAN_POINT('Ctrl Pts',(-62.5532849916988,-108.571250656727,
174.328630986959));
#22762=CARTESIAN_POINT('Ctrl Pts',(-62.5433468598446,-108.478028899421,
175.985485236451));
#22763=CARTESIAN_POINT('Ctrl Pts',(-62.5334087279904,-108.384807142114,
177.642339485944));
#22764=CARTESIAN_POINT('Ctrl Pts',(-61.3584989805568,-108.415779142081,
178.813912312176));
#22765=CARTESIAN_POINT('Ctrl Pts',(-60.1835892331231,-108.446751142048,
179.985485138407));
#22766=CARTESIAN_POINT('Ctrl Pts',(-58.5261324831192,-108.529165876334,
179.985485069079));
#22767=CARTESIAN_POINT('Ctrl Pts',(-56.8686757331153,-108.611580610621,
179.985484999752));
#22768=CARTESIAN_POINT('Ctrl Pts',(-55.6937660831736,-108.642552600194,
178.813912075476));
#22769=CARTESIAN_POINT('Ctrl Pts',(-54.5188564332318,-108.673524589768,
177.6423391512));
#22770=CARTESIAN_POINT('Ctrl Pts',(-54.5089184392519,-108.580302817763,
175.985484901707));
#22771=CARTESIAN_POINT('Ctrl Pts',(-54.4989804452721,-108.487081045759,
174.328630652215));
#22772=CARTESIAN_POINT('Ctrl Pts',(-55.6540140668717,-108.269665516481,
173.157057825983));
#22773=CARTESIAN_POINT('Ctrl Pts',(-56.8090476884713,-108.052249987204,
171.985484999752));
#22774=CARTESIAN_POINT('Ctrl Pts',(-58.4466283126412,-107.783391723607,
171.985485069079));
#22775=CARTESIAN_POINT('Ctrl Pts',(-60.084208936811,-107.51453346001,171.985485138407));
#22776=CARTESIAN_POINT('Ctrl Pts',(-61.2392424609188,-107.297117941125,
173.157058062683));
#22777=CARTESIAN_POINT('Ctrl Pts',(-62.3942759850265,-107.079702422241,
174.328630986959));
#22778=CARTESIAN_POINT('Ctrl Pts',(-62.3843378531723,-106.986480664935,
175.985485236451));
#22779=CARTESIAN_POINT('Ctrl Pts',(-62.3743997213182,-106.893258907629,
177.642339485944));
#22780=CARTESIAN_POINT('Ctrl Pts',(-61.1994899738845,-106.924230907596,
178.813912312176));
#22781=CARTESIAN_POINT('Ctrl Pts',(-60.0245802264509,-106.955202907562,
179.985485138407));
#22782=CARTESIAN_POINT('Ctrl Pts',(-58.367123476447,-107.037617641849,179.985485069079));
#22783=CARTESIAN_POINT('Ctrl Pts',(-56.7096667264431,-107.120032376135,
179.985484999752));
#22784=CARTESIAN_POINT('Ctrl Pts',(-55.5347570765013,-107.151004365708,
178.813912075476));
#22785=CARTESIAN_POINT('Ctrl Pts',(-54.3598474265596,-107.181976355282,
177.6423391512));
#22786=CARTESIAN_POINT('Ctrl Pts',(-54.3499094325797,-107.088754583277,
175.985484901707));
#22787=CARTESIAN_POINT('Ctrl Pts',(-54.3399714385998,-106.995532811273,
174.328630652215));
#22788=CARTESIAN_POINT('Ctrl Pts',(-55.4950050601995,-106.778117281995,
173.157057825983));
#22789=CARTESIAN_POINT('Ctrl Pts',(-56.6500386817991,-106.560701752718,
171.985484999752));
#22790=CARTESIAN_POINT('Ctrl Pts',(-58.2876193059689,-106.291843489121,
171.985485069079));
#22791=CARTESIAN_POINT('Ctrl Pts',(-59.9251999301388,-106.022985225524,
171.985485138407));
#22792=CARTESIAN_POINT('Ctrl Pts',(-61.0802334542465,-105.80556970664,173.157058062683));
#22793=CARTESIAN_POINT('Ctrl Pts',(-62.2352669783543,-105.588154187756,
174.328630986959));
#22794=CARTESIAN_POINT('Ctrl Pts',(-62.2253288465001,-105.494932430449,
175.985485236451));
#22795=CARTESIAN_POINT('Ctrl Pts',(-62.2153907146459,-105.401710673143,
177.642339485944));
#22796=CARTESIAN_POINT('Ctrl Pts',(-61.0404809672123,-105.43268267311,178.813912312176));
#22797=CARTESIAN_POINT('Ctrl Pts',(-59.8655712197787,-105.463654673077,
179.985485138407));
#22798=CARTESIAN_POINT('Ctrl Pts',(-58.2081144697748,-105.546069407363,
179.985485069079));
#22799=CARTESIAN_POINT('Ctrl Pts',(-56.5506577197709,-105.628484141649,
179.985484999752));
#22800=CARTESIAN_POINT('Ctrl Pts',(-55.3757480698291,-105.659456131223,
178.813912075476));
#22801=CARTESIAN_POINT('Ctrl Pts',(-54.2008384198873,-105.690428120796,
177.6423391512));
#22802=CARTESIAN_POINT('Ctrl Pts',(-54.1909004259075,-105.597206348792,
175.985484901707));
#22803=CARTESIAN_POINT('Ctrl Pts',(-54.1809624319276,-105.503984576787,
174.328630652215));
#22804=CARTESIAN_POINT('Ctrl Pts',(-55.3359960535272,-105.28656904751,173.157057825983));
#22805=CARTESIAN_POINT('Ctrl Pts',(-56.4910296751268,-105.069153518232,
171.985484999752));
#22806=CARTESIAN_POINT('Ctrl Pts',(-58.1286102992967,-104.800295254635,
171.985485069079));
#22807=CARTESIAN_POINT('Ctrl Pts',(-59.7661909234666,-104.531436991038,
171.985485138407));
#22808=CARTESIAN_POINT('Ctrl Pts',(-60.9212244475743,-104.314021472154,
173.157058062683));
#22809=CARTESIAN_POINT('Ctrl Pts',(-62.0762579716821,-104.09660595327,174.328630986959));
#22810=CARTESIAN_POINT('Ctrl Pts',(-62.0663198398279,-104.003384195964,
175.985485236451));
#22811=CARTESIAN_POINT('Ctrl Pts',(-62.0563817079737,-103.910162438658,
177.642339485944));
#22812=CARTESIAN_POINT('Ctrl Pts',(-60.8814719605401,-103.941134438624,
178.813912312176));
#22813=CARTESIAN_POINT('Ctrl Pts',(-59.7065622131064,-103.972106438591,
179.985485138407));
#22814=CARTESIAN_POINT('Ctrl Pts',(-58.0491054631025,-104.054521172878,
179.985485069079));
#22815=CARTESIAN_POINT('Ctrl Pts',(-56.3916487130987,-104.136935907164,
179.985484999752));
#22816=CARTESIAN_POINT('Ctrl Pts',(-55.2167390631569,-104.167907896737,
178.813912075476));
#22817=CARTESIAN_POINT('Ctrl Pts',(-54.0418294132151,-104.198879886311,
177.6423391512));
#22818=CARTESIAN_POINT('Ctrl Pts',(-54.0318914192353,-104.105658114306,
175.985484901707));
#22819=CARTESIAN_POINT('Ctrl Pts',(-54.0219534252554,-104.012436342302,
174.328630652215));
#22820=CARTESIAN_POINT('Ctrl Pts',(-55.176987046855,-103.795020813024,173.157057825983));
#22821=CARTESIAN_POINT('Ctrl Pts',(-56.3320206684546,-103.577605283747,
171.985484999752));
#22822=CARTESIAN_POINT('Ctrl Pts',(-57.9696012926245,-103.30874702015,171.985485069079));
#22823=CARTESIAN_POINT('Ctrl Pts',(-59.6071819167943,-103.039888756553,
171.985485138407));
#22824=CARTESIAN_POINT('Ctrl Pts',(-60.7622154409021,-102.822473237669,
173.157058062683));
#22825=CARTESIAN_POINT('Ctrl Pts',(-61.9172489650099,-102.605057718784,
174.328630986959));
#22826=CARTESIAN_POINT('Ctrl Pts',(-61.9073108331557,-102.511835961478,
175.985485236451));
#22827=CARTESIAN_POINT('Ctrl Pts',(-61.8973727013015,-102.418614204172,
177.642339485944));
#22828=CARTESIAN_POINT('Ctrl Pts',(-60.7224629538678,-102.449586204139,
178.813912312176));
#22829=CARTESIAN_POINT('Ctrl Pts',(-59.5475532064342,-102.480558204106,
179.985485138407));
#22830=CARTESIAN_POINT('Ctrl Pts',(-57.8900964564303,-102.562972938392,
179.985485069079));
#22831=CARTESIAN_POINT('Ctrl Pts',(-56.2326397064264,-102.645387672678,
179.985484999752));
#22832=CARTESIAN_POINT('Ctrl Pts',(-55.0577300564847,-102.676359662252,
178.813912075476));
#22833=CARTESIAN_POINT('Ctrl Pts',(-53.8828204065429,-102.707331651825,
177.6423391512));
#22834=CARTESIAN_POINT('Ctrl Pts',(-53.872882412563,-102.614109879821,175.985484901707));
#22835=CARTESIAN_POINT('Ctrl Pts',(-53.8629444185832,-102.520888107816,
174.328630652215));
#22836=CARTESIAN_POINT('Ctrl Pts',(-55.0179780401828,-102.303472578539,
173.157057825983));
#22837=CARTESIAN_POINT('Ctrl Pts',(-56.1730116617824,-102.086057049261,
171.985484999752));
#22838=CARTESIAN_POINT('Ctrl Pts',(-57.8105922859523,-101.817198785664,
171.985485069079));
#22839=CARTESIAN_POINT('Ctrl Pts',(-59.4481729101221,-101.548340522067,
171.985485138407));
#22840=CARTESIAN_POINT('Ctrl Pts',(-60.6032064342299,-101.330925003183,
173.157058062683));
#22841=CARTESIAN_POINT('Ctrl Pts',(-61.7582399583376,-101.113509484299,
174.328630986959));
#22842=CARTESIAN_POINT('Ctrl Pts',(-61.7483018264834,-101.020287726993,
175.985485236451));
#22843=CARTESIAN_POINT('Ctrl Pts',(-61.7383636946293,-100.927065969686,
177.642339485944));
#22844=CARTESIAN_POINT('Ctrl Pts',(-60.5634539471956,-100.958037969653,
178.813912312176));
#22845=CARTESIAN_POINT('Ctrl Pts',(-59.388544199762,-100.98900996962,179.985485138407));
#22846=CARTESIAN_POINT('Ctrl Pts',(-57.7310874497581,-101.071424703906,
179.985485069079));
#22847=CARTESIAN_POINT('Ctrl Pts',(-56.0736306997542,-101.153839438193,
179.985484999752));
#22848=CARTESIAN_POINT('Ctrl Pts',(-54.8987210498124,-101.184811427766,
178.813912075476));
#22849=CARTESIAN_POINT('Ctrl Pts',(-53.7238113998707,-101.21578341734,177.6423391512));
#22850=CARTESIAN_POINT('Ctrl Pts',(-53.7138734058908,-101.122561645335,
175.985484901707));
#22851=CARTESIAN_POINT('Ctrl Pts',(-53.7039354119109,-101.029339873331,
174.328630652215));
#22852=CARTESIAN_POINT('Ctrl Pts',(-54.8589690335105,-100.811924344053,
173.157057825983));
#22853=CARTESIAN_POINT('Ctrl Pts',(-56.0140026551102,-100.594508814776,
171.985484999752));
#22854=CARTESIAN_POINT('Ctrl Pts',(-57.65158327928,-100.325650551179,171.985485069079));
#22855=CARTESIAN_POINT('Ctrl Pts',(-59.2891639034499,-100.056792287582,
171.985485138407));
#22856=CARTESIAN_POINT('Ctrl Pts',(-60.4441974275576,-99.8393767686974,
173.157058062683));
#22857=CARTESIAN_POINT('Ctrl Pts',(-61.5992309516654,-99.6219612498133,
174.328630986959));
#22858=CARTESIAN_POINT('Ctrl Pts',(-61.5892928198112,-99.528739492507,175.985485236451));
#22859=CARTESIAN_POINT('Ctrl Pts',(-61.579354687957,-99.4355177352008,177.642339485944));
#22860=CARTESIAN_POINT('Ctrl Pts',(-60.4044449405234,-99.4664897351676,
178.813912312176));
#22861=CARTESIAN_POINT('Ctrl Pts',(-59.2295351930898,-99.4974617351344,
179.985485138407));
#22862=CARTESIAN_POINT('Ctrl Pts',(-57.5720784430859,-99.5798764694207,
179.985485069079));
#22863=CARTESIAN_POINT('Ctrl Pts',(-55.914621693082,-99.662291203707,179.985484999752));
#22864=CARTESIAN_POINT('Ctrl Pts',(-54.7397120431402,-99.6932631932805,
178.813912075476));
#22865=CARTESIAN_POINT('Ctrl Pts',(-53.5648023931984,-99.724235182854,177.6423391512));
#22866=CARTESIAN_POINT('Ctrl Pts',(-53.5548643992186,-99.6310134108495,
175.985484901707));
#22867=CARTESIAN_POINT('Ctrl Pts',(-53.5449264052387,-99.5377916388449,
174.328630652215));
#22868=CARTESIAN_POINT('Ctrl Pts',(-54.6999600268383,-99.3203761095675,
173.157057825983));
#22869=CARTESIAN_POINT('Ctrl Pts',(-55.8549936484379,-99.10296058029,171.985484999752));
#22870=CARTESIAN_POINT('Ctrl Pts',(-57.4925742726078,-98.834102316693,171.985485069079));
#22871=CARTESIAN_POINT('Ctrl Pts',(-59.1301548967777,-98.5652440530961,
171.985485138407));
#22872=CARTESIAN_POINT('Ctrl Pts',(-60.2851884208854,-98.3478285342118,
173.157058062683));
#22873=CARTESIAN_POINT('Ctrl Pts',(-61.4402219449932,-98.1304130153276,
174.328630986959));
#22874=CARTESIAN_POINT('Ctrl Pts',(-61.430283813139,-98.0371912580215,175.985485236451));
#22875=CARTESIAN_POINT('Ctrl Pts',(-61.4203456812848,-97.9439695007152,
177.642339485944));
#22876=CARTESIAN_POINT('Ctrl Pts',(-60.2454359338512,-97.974941500682,178.813912312176));
#22877=CARTESIAN_POINT('Ctrl Pts',(-59.0705261864175,-98.0059135006488,
179.985485138407));
#22878=CARTESIAN_POINT('Ctrl Pts',(-57.4130694364136,-98.0883282349351,
179.985485069079));
#22879=CARTESIAN_POINT('Ctrl Pts',(-55.7556126864097,-98.1707429692214,
179.985484999752));
#22880=CARTESIAN_POINT('Ctrl Pts',(-54.580703036468,-98.2017149587949,178.813912075476));
#22881=CARTESIAN_POINT('Ctrl Pts',(-56.181115489574,-113.283598570176,178.821287383467));
#22882=CARTESIAN_POINT('Ctrl Pts',(-55.0031681001975,-113.314894403068,
177.646659506339));
#22883=CARTESIAN_POINT('Ctrl Pts',(-54.9932301063974,-113.221672631044,
175.985484901271));
#22884=CARTESIAN_POINT('Ctrl Pts',(-54.9832921125973,-113.12845085902,174.324310296203));
#22885=CARTESIAN_POINT('Ctrl Pts',(-56.1413634738858,-112.910711486397,
173.149682517375));
#22886=CARTESIAN_POINT('Ctrl Pts',(-57.2994348351743,-112.692972113774,
171.975054738546));
#22887=CARTESIAN_POINT('Ctrl Pts',(-58.9413114718314,-112.423655866545,
171.975054808055));
#22888=CARTESIAN_POINT('Ctrl Pts',(-60.5831881084886,-112.154339619316,
171.975054877564));
#22889=CARTESIAN_POINT('Ctrl Pts',(-61.741259372031,-111.936600257113,173.149682754692));
#22890=CARTESIAN_POINT('Ctrl Pts',(-62.8993306355734,-111.71886089491,174.32431063182));
#22891=CARTESIAN_POINT('Ctrl Pts',(-62.8893925035395,-111.625639137623,
175.985485236888));
#22892=CARTESIAN_POINT('Ctrl Pts',(-62.8794543715055,-111.532417380336,
177.646659841956));
#22893=CARTESIAN_POINT('Ctrl Pts',(-61.701506884383,-111.563713223648,178.821287620784));
#22894=CARTESIAN_POINT('Ctrl Pts',(-60.5235593972605,-111.595009066961,
179.995915399612));
#22895=CARTESIAN_POINT('Ctrl Pts',(-58.8618066347693,-111.677881784879,
179.995915330104));
#22896=CARTESIAN_POINT('Ctrl Pts',(-57.2000538722782,-111.760754502798,
179.995915260595));
#22897=CARTESIAN_POINT('Ctrl Pts',(-56.0221064829017,-111.79205033569,178.821287383467));
#22898=CARTESIAN_POINT('Ctrl Pts',(-54.8441590935253,-111.823346168582,
177.646659506339));
#22899=CARTESIAN_POINT('Ctrl Pts',(-54.8342210997252,-111.730124396559,
175.985484901271));
#22900=CARTESIAN_POINT('Ctrl Pts',(-54.8242831059251,-111.636902624535,
174.324310296203));
#22901=CARTESIAN_POINT('Ctrl Pts',(-55.9823544672136,-111.419163251912,
173.149682517375));
#22902=CARTESIAN_POINT('Ctrl Pts',(-57.1404258285021,-111.201423879289,
171.975054738546));
#22903=CARTESIAN_POINT('Ctrl Pts',(-58.7823024651592,-110.932107632059,
171.975054808055));
#22904=CARTESIAN_POINT('Ctrl Pts',(-60.4241791018163,-110.66279138483,171.975054877564));
#22905=CARTESIAN_POINT('Ctrl Pts',(-61.5822503653587,-110.445052022627,
173.149682754692));
#22906=CARTESIAN_POINT('Ctrl Pts',(-62.7403216289012,-110.227312660424,
174.32431063182));
#22907=CARTESIAN_POINT('Ctrl Pts',(-62.7303834968672,-110.134090903137,
175.985485236888));
#22908=CARTESIAN_POINT('Ctrl Pts',(-62.7204453648333,-110.04086914585,177.646659841956));
#22909=CARTESIAN_POINT('Ctrl Pts',(-61.5424978777108,-110.072164989163,
178.821287620784));
#22910=CARTESIAN_POINT('Ctrl Pts',(-60.3645503905882,-110.103460832475,
179.995915399612));
#22911=CARTESIAN_POINT('Ctrl Pts',(-58.7027976280971,-110.186333550394,
179.995915330104));
#22912=CARTESIAN_POINT('Ctrl Pts',(-57.041044865606,-110.269206268313,179.995915260595));
#22913=CARTESIAN_POINT('Ctrl Pts',(-55.8630974762295,-110.300502101205,
178.821287383467));
#22914=CARTESIAN_POINT('Ctrl Pts',(-54.6851500868531,-110.331797934097,
177.646659506339));
#22915=CARTESIAN_POINT('Ctrl Pts',(-54.675212093053,-110.238576162073,175.985484901271));
#22916=CARTESIAN_POINT('Ctrl Pts',(-54.6652740992529,-110.145354390049,
174.324310296203));
#22917=CARTESIAN_POINT('Ctrl Pts',(-55.8233454605414,-109.927615017426,
173.149682517375));
#22918=CARTESIAN_POINT('Ctrl Pts',(-56.9814168218299,-109.709875644803,
171.975054738546));
#22919=CARTESIAN_POINT('Ctrl Pts',(-58.623293458487,-109.440559397574,171.975054808055));
#22920=CARTESIAN_POINT('Ctrl Pts',(-60.2651700951441,-109.171243150344,
171.975054877564));
#22921=CARTESIAN_POINT('Ctrl Pts',(-61.4232413586865,-108.953503788142,
173.149682754692));
#22922=CARTESIAN_POINT('Ctrl Pts',(-62.581312622229,-108.735764425939,174.32431063182));
#22923=CARTESIAN_POINT('Ctrl Pts',(-62.571374490195,-108.642542668652,175.985485236888));
#22924=CARTESIAN_POINT('Ctrl Pts',(-62.5614363581611,-108.549320911365,
177.646659841956));
#22925=CARTESIAN_POINT('Ctrl Pts',(-61.3834888710385,-108.580616754677,
178.821287620784));
#22926=CARTESIAN_POINT('Ctrl Pts',(-60.205541383916,-108.61191259799,179.995915399612));
#22927=CARTESIAN_POINT('Ctrl Pts',(-58.5437886214249,-108.694785315908,
179.995915330104));
#22928=CARTESIAN_POINT('Ctrl Pts',(-56.8820358589338,-108.777658033827,
179.995915260595));
#22929=CARTESIAN_POINT('Ctrl Pts',(-55.7040884695573,-108.808953866719,
178.821287383467));
#22930=CARTESIAN_POINT('Ctrl Pts',(-54.5261410801808,-108.840249699611,
177.646659506339));
#22931=CARTESIAN_POINT('Ctrl Pts',(-54.5162030863807,-108.747027927587,
175.985484901271));
#22932=CARTESIAN_POINT('Ctrl Pts',(-54.5062650925806,-108.653806155564,
174.324310296203));
#22933=CARTESIAN_POINT('Ctrl Pts',(-55.6643364538691,-108.436066782941,
173.149682517375));
#22934=CARTESIAN_POINT('Ctrl Pts',(-56.8224078151577,-108.218327410317,
171.975054738546));
#22935=CARTESIAN_POINT('Ctrl Pts',(-58.4642844518147,-107.949011163088,
171.975054808055));
#22936=CARTESIAN_POINT('Ctrl Pts',(-60.1061610884719,-107.679694915859,
171.975054877564));
#22937=CARTESIAN_POINT('Ctrl Pts',(-61.2642323520143,-107.461955553656,
173.149682754692));
#22938=CARTESIAN_POINT('Ctrl Pts',(-62.4223036155567,-107.244216191453,
174.32431063182));
#22939=CARTESIAN_POINT('Ctrl Pts',(-62.4123654835228,-107.150994434166,
175.985485236888));
#22940=CARTESIAN_POINT('Ctrl Pts',(-62.4024273514889,-107.057772676879,
177.646659841956));
#22941=CARTESIAN_POINT('Ctrl Pts',(-61.2244798643663,-107.089068520192,
178.821287620784));
#22942=CARTESIAN_POINT('Ctrl Pts',(-60.0465323772438,-107.120364363504,
179.995915399612));
#22943=CARTESIAN_POINT('Ctrl Pts',(-58.3847796147526,-107.203237081423,
179.995915330104));
#22944=CARTESIAN_POINT('Ctrl Pts',(-56.7230268522615,-107.286109799341,
179.995915260595));
#22945=CARTESIAN_POINT('Ctrl Pts',(-55.5450794628851,-107.317405632233,
178.821287383467));
#22946=CARTESIAN_POINT('Ctrl Pts',(-54.3671320735086,-107.348701465125,
177.646659506339));
#22947=CARTESIAN_POINT('Ctrl Pts',(-54.3571940797085,-107.255479693102,
175.985484901271));
#22948=CARTESIAN_POINT('Ctrl Pts',(-54.3472560859084,-107.162257921078,
174.324310296203));
#22949=CARTESIAN_POINT('Ctrl Pts',(-55.5053274471969,-106.944518548455,
173.149682517375));
#22950=CARTESIAN_POINT('Ctrl Pts',(-56.6633988084854,-106.726779175832,
171.975054738546));
#22951=CARTESIAN_POINT('Ctrl Pts',(-58.3052754451425,-106.457462928602,
171.975054808055));
#22952=CARTESIAN_POINT('Ctrl Pts',(-59.9471520817997,-106.188146681373,
171.975054877564));
#22953=CARTESIAN_POINT('Ctrl Pts',(-61.1052233453421,-105.97040731917,173.149682754692));
#22954=CARTESIAN_POINT('Ctrl Pts',(-62.2632946088845,-105.752667956968,
174.32431063182));
#22955=CARTESIAN_POINT('Ctrl Pts',(-62.2533564768505,-105.659446199681,
175.985485236888));
#22956=CARTESIAN_POINT('Ctrl Pts',(-62.2434183448166,-105.566224442394,
177.646659841956));
#22957=CARTESIAN_POINT('Ctrl Pts',(-61.0654708576941,-105.597520285706,
178.821287620784));
#22958=CARTESIAN_POINT('Ctrl Pts',(-59.8875233705716,-105.628816129018,
179.995915399612));
#22959=CARTESIAN_POINT('Ctrl Pts',(-58.2257706080804,-105.711688846937,
179.995915330104));
#22960=CARTESIAN_POINT('Ctrl Pts',(-56.5640178455893,-105.794561564856,
179.995915260595));
#22961=CARTESIAN_POINT('Ctrl Pts',(-55.3860704562128,-105.825857397748,
178.821287383467));
#22962=CARTESIAN_POINT('Ctrl Pts',(-54.2081230668364,-105.85715323064,177.646659506339));
#22963=CARTESIAN_POINT('Ctrl Pts',(-54.1981850730363,-105.763931458616,
175.985484901271));
#22964=CARTESIAN_POINT('Ctrl Pts',(-54.1882470792362,-105.670709686593,
174.324310296203));
#22965=CARTESIAN_POINT('Ctrl Pts',(-55.3463184405247,-105.452970313969,
173.149682517375));
#22966=CARTESIAN_POINT('Ctrl Pts',(-56.5043898018132,-105.235230941346,
171.975054738546));
#22967=CARTESIAN_POINT('Ctrl Pts',(-58.1462664384703,-104.965914694117,
171.975054808055));
#22968=CARTESIAN_POINT('Ctrl Pts',(-59.7881430751274,-104.696598446888,
171.975054877564));
#22969=CARTESIAN_POINT('Ctrl Pts',(-60.9462143386698,-104.478859084685,
173.149682754692));
#22970=CARTESIAN_POINT('Ctrl Pts',(-62.1042856022123,-104.261119722482,
174.32431063182));
#22971=CARTESIAN_POINT('Ctrl Pts',(-62.0943474701783,-104.167897965195,
175.985485236888));
#22972=CARTESIAN_POINT('Ctrl Pts',(-62.0844093381444,-104.074676207908,
177.646659841956));
#22973=CARTESIAN_POINT('Ctrl Pts',(-60.9064618510219,-104.10597205122,178.821287620784));
#22974=CARTESIAN_POINT('Ctrl Pts',(-59.7285143638993,-104.137267894533,
179.995915399612));
#22975=CARTESIAN_POINT('Ctrl Pts',(-58.0667616014082,-104.220140612451,
179.995915330104));
#22976=CARTESIAN_POINT('Ctrl Pts',(-56.4050088389171,-104.30301333037,179.995915260595));
#22977=CARTESIAN_POINT('Ctrl Pts',(-55.2270614495406,-104.334309163262,
178.821287383467));
#22978=CARTESIAN_POINT('Ctrl Pts',(-54.0491140601642,-104.365604996154,
177.646659506339));
#22979=CARTESIAN_POINT('Ctrl Pts',(-54.039176066364,-104.272383224131,175.985484901271));
#22980=CARTESIAN_POINT('Ctrl Pts',(-54.029238072564,-104.179161452107,174.324310296203));
#22981=CARTESIAN_POINT('Ctrl Pts',(-55.1873094338524,-103.961422079484,
173.149682517375));
#22982=CARTESIAN_POINT('Ctrl Pts',(-56.345380795141,-103.743682706861,171.975054738546));
#22983=CARTESIAN_POINT('Ctrl Pts',(-57.9872574317981,-103.474366459631,
171.975054808055));
#22984=CARTESIAN_POINT('Ctrl Pts',(-59.6291340684552,-103.205050212402,
171.975054877564));
#22985=CARTESIAN_POINT('Ctrl Pts',(-60.7872053319976,-102.987310850199,
173.149682754692));
#22986=CARTESIAN_POINT('Ctrl Pts',(-61.94527659554,-102.769571487996,174.32431063182));
#22987=CARTESIAN_POINT('Ctrl Pts',(-61.9353384635061,-102.676349730709,
175.985485236888));
#22988=CARTESIAN_POINT('Ctrl Pts',(-61.9254003314722,-102.583127973422,
177.646659841956));
#22989=CARTESIAN_POINT('Ctrl Pts',(-60.7474528443496,-102.614423816735,
178.821287620784));
#22990=CARTESIAN_POINT('Ctrl Pts',(-59.5695053572271,-102.645719660047,
179.995915399612));
#22991=CARTESIAN_POINT('Ctrl Pts',(-57.907752594736,-102.728592377966,179.995915330104));
#22992=CARTESIAN_POINT('Ctrl Pts',(-56.2459998322448,-102.811465095885,
179.995915260595));
#22993=CARTESIAN_POINT('Ctrl Pts',(-55.0680524428684,-102.842760928777,
178.821287383467));
#22994=CARTESIAN_POINT('Ctrl Pts',(-53.8901050534919,-102.874056761669,
177.646659506339));
#22995=CARTESIAN_POINT('Ctrl Pts',(-53.8801670596918,-102.780834989645,
175.985484901271));
#22996=CARTESIAN_POINT('Ctrl Pts',(-53.8702290658917,-102.687613217621,
174.324310296203));
#22997=CARTESIAN_POINT('Ctrl Pts',(-55.0283004271802,-102.469873844998,
173.149682517375));
#22998=CARTESIAN_POINT('Ctrl Pts',(-56.1863717884687,-102.252134472375,
171.975054738546));
#22999=CARTESIAN_POINT('Ctrl Pts',(-57.8282484251258,-101.982818225146,
171.975054808055));
#23000=CARTESIAN_POINT('Ctrl Pts',(-59.470125061783,-101.713501977916,171.975054877564));
#23001=CARTESIAN_POINT('Ctrl Pts',(-60.6281963253254,-101.495762615714,
173.149682754692));
#23002=CARTESIAN_POINT('Ctrl Pts',(-61.7862675888678,-101.278023253511,
174.32431063182));
#23003=CARTESIAN_POINT('Ctrl Pts',(-61.7763294568339,-101.184801496224,
175.985485236888));
#23004=CARTESIAN_POINT('Ctrl Pts',(-61.7663913247999,-101.091579738937,
177.646659841956));
#23005=CARTESIAN_POINT('Ctrl Pts',(-60.5884438376774,-101.122875582249,
178.821287620784));
#23006=CARTESIAN_POINT('Ctrl Pts',(-59.4104963505549,-101.154171425562,
179.995915399612));
#23007=CARTESIAN_POINT('Ctrl Pts',(-57.7487435880637,-101.23704414348,179.995915330104));
#23008=CARTESIAN_POINT('Ctrl Pts',(-56.0869908255726,-101.319916861399,
179.995915260595));
#23009=CARTESIAN_POINT('Ctrl Pts',(-54.9090434361961,-101.351212694291,
178.821287383467));
#23010=CARTESIAN_POINT('Ctrl Pts',(-53.7310960468197,-101.382508527183,
177.646659506339));
#23011=CARTESIAN_POINT('Ctrl Pts',(-53.7211580530196,-101.289286755159,
175.985484901271));
#23012=CARTESIAN_POINT('Ctrl Pts',(-53.7112200592195,-101.196064983136,
174.324310296203));
#23013=CARTESIAN_POINT('Ctrl Pts',(-54.869291420508,-100.978325610513,173.149682517375));
#23014=CARTESIAN_POINT('Ctrl Pts',(-56.0273627817965,-100.760586237889,
171.975054738546));
#23015=CARTESIAN_POINT('Ctrl Pts',(-57.6692394184536,-100.49126999066,171.975054808055));
#23016=CARTESIAN_POINT('Ctrl Pts',(-59.3111160551107,-100.221953743431,
171.975054877564));
#23017=CARTESIAN_POINT('Ctrl Pts',(-60.4691873186531,-100.004214381228,
173.149682754692));
#23018=CARTESIAN_POINT('Ctrl Pts',(-61.6272585821956,-99.7864750190253,
174.32431063182));
#23019=CARTESIAN_POINT('Ctrl Pts',(-61.6173204501616,-99.6932532617382,
175.985485236888));
#23020=CARTESIAN_POINT('Ctrl Pts',(-61.6073823181277,-99.6000315044512,
177.646659841956));
#23021=CARTESIAN_POINT('Ctrl Pts',(-60.4294348310052,-99.6313273477637,
178.821287620784));
#23022=CARTESIAN_POINT('Ctrl Pts',(-59.2514873438827,-99.6626231910761,
179.995915399612));
#23023=CARTESIAN_POINT('Ctrl Pts',(-57.5897345813915,-99.7454959089947,
179.995915330104));
#23024=CARTESIAN_POINT('Ctrl Pts',(-55.9279818189004,-99.8283686269133,
179.995915260595));
#23025=CARTESIAN_POINT('Ctrl Pts',(-54.7500344295239,-99.8596644598054,
178.821287383467));
#23026=CARTESIAN_POINT('Ctrl Pts',(-53.5720870401475,-99.8909602926975,
177.646659506339));
#23027=CARTESIAN_POINT('Ctrl Pts',(-53.5621490463474,-99.7977385206737,
175.985484901271));
#23028=CARTESIAN_POINT('Ctrl Pts',(-53.5522110525473,-99.7045167486501,
174.324310296203));
#23029=CARTESIAN_POINT('Ctrl Pts',(-54.7102824138358,-99.4867773760269,
173.149682517375));
#23030=CARTESIAN_POINT('Ctrl Pts',(-55.8683537751243,-99.2690380034038,
171.975054738546));
#23031=CARTESIAN_POINT('Ctrl Pts',(-57.5102304117814,-98.9997217561745,
171.975054808055));
#23032=CARTESIAN_POINT('Ctrl Pts',(-59.1521070484385,-98.7304055089452,
171.975054877564));
#23033=CARTESIAN_POINT('Ctrl Pts',(-60.3101783119809,-98.5126661467424,
173.149682754692));
#23034=CARTESIAN_POINT('Ctrl Pts',(-61.4682495755234,-98.2949267845397,
174.32431063182));
#23035=CARTESIAN_POINT('Ctrl Pts',(-61.4583114434894,-98.2017050272526,
175.985485236888));
#23036=CARTESIAN_POINT('Ctrl Pts',(-61.4483733114555,-98.1084832699656,
177.646659841956));
#23037=CARTESIAN_POINT('Ctrl Pts',(-60.2704258243329,-98.139779113278,178.821287620784));
#23038=CARTESIAN_POINT('Ctrl Pts',(-59.0924783372104,-98.1710749565905,
179.995915399612));
#23039=CARTESIAN_POINT('Ctrl Pts',(-57.4307255747193,-98.2539476745091,
179.995915330104));
#23040=CARTESIAN_POINT('Ctrl Pts',(-55.7689728122282,-98.3368203924277,
179.995915260595));
#23041=CARTESIAN_POINT('Ctrl Pts',(-54.5910254228517,-98.3681162253198,
178.821287383467));
#23042=CARTESIAN_POINT('Ctrl Pts',(-56.1988062143188,-113.449542435949,
178.821287383467));
#23043=CARTESIAN_POINT('Ctrl Pts',(-55.0208588249424,-113.480838268841,
177.646659506339));
#23044=CARTESIAN_POINT('Ctrl Pts',(-55.0109208311422,-113.387616496817,
175.985484901271));
#23045=CARTESIAN_POINT('Ctrl Pts',(-55.0009828373422,-113.294394724794,
174.324310296203));
#23046=CARTESIAN_POINT('Ctrl Pts',(-56.1590541986307,-113.07665535217,173.149682517375));
#23047=CARTESIAN_POINT('Ctrl Pts',(-57.3171255599192,-112.858915979547,
171.975054738546));
#23048=CARTESIAN_POINT('Ctrl Pts',(-58.9590021965763,-112.589599732318,
171.975054808055));
#23049=CARTESIAN_POINT('Ctrl Pts',(-60.6008788332334,-112.320283485089,
171.975054877564));
#23050=CARTESIAN_POINT('Ctrl Pts',(-61.7589500967758,-112.102544122886,
173.149682754692));
#23051=CARTESIAN_POINT('Ctrl Pts',(-62.9170213603182,-111.884804760683,
174.32431063182));
#23052=CARTESIAN_POINT('Ctrl Pts',(-62.9070832282843,-111.791583003396,
175.985485236888));
#23053=CARTESIAN_POINT('Ctrl Pts',(-62.8971450962504,-111.698361246109,
177.646659841956));
#23054=CARTESIAN_POINT('Ctrl Pts',(-61.7191976091278,-111.729657089422,
178.821287620784));
#23055=CARTESIAN_POINT('Ctrl Pts',(-60.5412501220053,-111.760952932734,
179.995915399612));
#23056=CARTESIAN_POINT('Ctrl Pts',(-58.8794973595142,-111.843825650653,
179.995915330104));
#23057=CARTESIAN_POINT('Ctrl Pts',(-57.217744597023,-111.926698368571,179.995915260595));
#23058=CARTESIAN_POINT('Ctrl Pts',(-56.0397972076466,-111.957994201463,
178.821287383467));
#23059=CARTESIAN_POINT('Ctrl Pts',(-54.8618498182701,-111.989290034355,
177.646659506339));
#23060=CARTESIAN_POINT('Ctrl Pts',(-54.85191182447,-111.896068262332,175.985484901271));
#23061=CARTESIAN_POINT('Ctrl Pts',(-54.8419738306699,-111.802846490308,
174.324310296203));
#23062=CARTESIAN_POINT('Ctrl Pts',(-56.0000451919584,-111.585107117685,
173.149682517375));
#23063=CARTESIAN_POINT('Ctrl Pts',(-57.158116553247,-111.367367745062,171.975054738546));
#23064=CARTESIAN_POINT('Ctrl Pts',(-58.799993189904,-111.098051497832,171.975054808055));
#23065=CARTESIAN_POINT('Ctrl Pts',(-60.4418698265612,-110.828735250603,
171.975054877564));
#23066=CARTESIAN_POINT('Ctrl Pts',(-61.5999410901036,-110.6109958884,173.149682754692));
#23067=CARTESIAN_POINT('Ctrl Pts',(-62.758012353646,-110.393256526198,174.32431063182));
#23068=CARTESIAN_POINT('Ctrl Pts',(-62.7480742216121,-110.30003476891,175.985485236888));
#23069=CARTESIAN_POINT('Ctrl Pts',(-62.7381360895782,-110.206813011623,
177.646659841956));
#23070=CARTESIAN_POINT('Ctrl Pts',(-61.5601886024556,-110.238108854936,
178.821287620784));
#23071=CARTESIAN_POINT('Ctrl Pts',(-60.3822411153331,-110.269404698248,
179.995915399612));
#23072=CARTESIAN_POINT('Ctrl Pts',(-58.7204883528419,-110.352277416167,
179.995915330104));
#23073=CARTESIAN_POINT('Ctrl Pts',(-57.0587355903508,-110.435150134086,
179.995915260595));
#23074=CARTESIAN_POINT('Ctrl Pts',(-55.8807882009743,-110.466445966978,
178.821287383467));
#23075=CARTESIAN_POINT('Ctrl Pts',(-54.7028408115979,-110.49774179987,177.646659506339));
#23076=CARTESIAN_POINT('Ctrl Pts',(-54.6929028177978,-110.404520027846,
175.985484901271));
#23077=CARTESIAN_POINT('Ctrl Pts',(-54.6829648239977,-110.311298255822,
174.324310296203));
#23078=CARTESIAN_POINT('Ctrl Pts',(-55.8410361852862,-110.093558883199,
173.149682517375));
#23079=CARTESIAN_POINT('Ctrl Pts',(-56.9991075465747,-109.875819510576,
171.975054738546));
#23080=CARTESIAN_POINT('Ctrl Pts',(-58.6409841832318,-109.606503263347,
171.975054808055));
#23081=CARTESIAN_POINT('Ctrl Pts',(-60.2828608198889,-109.337187016117,
171.975054877564));
#23082=CARTESIAN_POINT('Ctrl Pts',(-61.4409320834313,-109.119447653915,
173.149682754692));
#23083=CARTESIAN_POINT('Ctrl Pts',(-62.5990033469738,-108.901708291712,
174.32431063182));
#23084=CARTESIAN_POINT('Ctrl Pts',(-62.5890652149398,-108.808486534425,
175.985485236888));
#23085=CARTESIAN_POINT('Ctrl Pts',(-62.5791270829059,-108.715264777138,
177.646659841956));
#23086=CARTESIAN_POINT('Ctrl Pts',(-61.4011795957834,-108.74656062045,178.821287620784));
#23087=CARTESIAN_POINT('Ctrl Pts',(-60.2232321086609,-108.777856463763,
179.995915399612));
#23088=CARTESIAN_POINT('Ctrl Pts',(-58.5614793461697,-108.860729181681,
179.995915330104));
#23089=CARTESIAN_POINT('Ctrl Pts',(-56.8997265836786,-108.9436018996,179.995915260595));
#23090=CARTESIAN_POINT('Ctrl Pts',(-55.7217791943021,-108.974897732492,
178.821287383467));
#23091=CARTESIAN_POINT('Ctrl Pts',(-54.5438318049257,-109.006193565384,
177.646659506339));
#23092=CARTESIAN_POINT('Ctrl Pts',(-54.5338938111256,-108.91297179336,175.985484901271));
#23093=CARTESIAN_POINT('Ctrl Pts',(-54.5239558173255,-108.819750021337,
174.324310296203));
#23094=CARTESIAN_POINT('Ctrl Pts',(-55.682027178614,-108.602010648714,173.149682517375));
#23095=CARTESIAN_POINT('Ctrl Pts',(-56.8400985399025,-108.384271276091,
171.975054738546));
#23096=CARTESIAN_POINT('Ctrl Pts',(-58.4819751765596,-108.114955028861,
171.975054808055));
#23097=CARTESIAN_POINT('Ctrl Pts',(-60.1238518132167,-107.845638781632,
171.975054877564));
#23098=CARTESIAN_POINT('Ctrl Pts',(-61.2819230767591,-107.627899419429,
173.149682754692));
#23099=CARTESIAN_POINT('Ctrl Pts',(-62.4399943403016,-107.410160057226,
174.32431063182));
#23100=CARTESIAN_POINT('Ctrl Pts',(-62.4300562082676,-107.316938299939,
175.985485236888));
#23101=CARTESIAN_POINT('Ctrl Pts',(-62.4201180762337,-107.223716542652,
177.646659841956));
#23102=CARTESIAN_POINT('Ctrl Pts',(-61.2421705891111,-107.255012385965,
178.821287620784));
#23103=CARTESIAN_POINT('Ctrl Pts',(-60.0642231019886,-107.286308229277,
179.995915399612));
#23104=CARTESIAN_POINT('Ctrl Pts',(-58.4024703394975,-107.369180947196,
179.995915330104));
#23105=CARTESIAN_POINT('Ctrl Pts',(-56.7407175770064,-107.452053665114,
179.995915260595));
#23106=CARTESIAN_POINT('Ctrl Pts',(-55.5627701876299,-107.483349498006,
178.821287383467));
#23107=CARTESIAN_POINT('Ctrl Pts',(-54.3848227982534,-107.514645330899,
177.646659506339));
#23108=CARTESIAN_POINT('Ctrl Pts',(-54.3748848044533,-107.421423558875,
175.985484901271));
#23109=CARTESIAN_POINT('Ctrl Pts',(-54.3649468106533,-107.328201786851,
174.324310296203));
#23110=CARTESIAN_POINT('Ctrl Pts',(-55.5230181719417,-107.110462414228,
173.149682517375));
#23111=CARTESIAN_POINT('Ctrl Pts',(-56.6810895332303,-106.892723041605,
171.975054738546));
#23112=CARTESIAN_POINT('Ctrl Pts',(-58.3229661698874,-106.623406794376,
171.975054808055));
#23113=CARTESIAN_POINT('Ctrl Pts',(-59.9648428065445,-106.354090547146,
171.975054877564));
#23114=CARTESIAN_POINT('Ctrl Pts',(-61.1229140700869,-106.136351184943,
173.149682754692));
#23115=CARTESIAN_POINT('Ctrl Pts',(-62.2809853336293,-105.918611822741,
174.32431063182));
#23116=CARTESIAN_POINT('Ctrl Pts',(-62.2710472015954,-105.825390065454,
175.985485236888));
#23117=CARTESIAN_POINT('Ctrl Pts',(-62.2611090695615,-105.732168308167,
177.646659841956));
#23118=CARTESIAN_POINT('Ctrl Pts',(-61.0831615824389,-105.763464151479,
178.821287620784));
#23119=CARTESIAN_POINT('Ctrl Pts',(-59.9052140953164,-105.794759994792,
179.995915399612));
#23120=CARTESIAN_POINT('Ctrl Pts',(-58.2434613328252,-105.87763271271,179.995915330104));
#23121=CARTESIAN_POINT('Ctrl Pts',(-56.5817085703341,-105.960505430629,
179.995915260595));
#23122=CARTESIAN_POINT('Ctrl Pts',(-55.4037611809577,-105.991801263521,
178.821287383467));
#23123=CARTESIAN_POINT('Ctrl Pts',(-54.2258137915812,-106.023097096413,
177.646659506339));
#23124=CARTESIAN_POINT('Ctrl Pts',(-54.2158757977811,-105.929875324389,
175.985484901271));
#23125=CARTESIAN_POINT('Ctrl Pts',(-54.205937803981,-105.836653552366,174.324310296203));
#23126=CARTESIAN_POINT('Ctrl Pts',(-55.3640091652695,-105.618914179742,
173.149682517375));
#23127=CARTESIAN_POINT('Ctrl Pts',(-56.522080526558,-105.401174807119,171.975054738546));
#23128=CARTESIAN_POINT('Ctrl Pts',(-58.1639571632151,-105.13185855989,171.975054808055));
#23129=CARTESIAN_POINT('Ctrl Pts',(-59.8058337998722,-104.862542312661,
171.975054877564));
#23130=CARTESIAN_POINT('Ctrl Pts',(-60.9639050634147,-104.644802950458,
173.149682754692));
#23131=CARTESIAN_POINT('Ctrl Pts',(-62.1219763269571,-104.427063588255,
174.32431063182));
#23132=CARTESIAN_POINT('Ctrl Pts',(-62.1120381949232,-104.333841830968,
175.985485236888));
#23133=CARTESIAN_POINT('Ctrl Pts',(-62.1021000628892,-104.240620073681,
177.646659841956));
#23134=CARTESIAN_POINT('Ctrl Pts',(-60.9241525757667,-104.271915916993,
178.821287620784));
#23135=CARTESIAN_POINT('Ctrl Pts',(-59.7462050886442,-104.303211760306,
179.995915399612));
#23136=CARTESIAN_POINT('Ctrl Pts',(-58.084452326153,-104.386084478225,179.995915330104));
#23137=CARTESIAN_POINT('Ctrl Pts',(-56.4226995636619,-104.468957196143,
179.995915260595));
#23138=CARTESIAN_POINT('Ctrl Pts',(-55.2447521742854,-104.500253029035,
178.821287383467));
#23139=CARTESIAN_POINT('Ctrl Pts',(-54.066804784909,-104.531548861927,177.646659506339));
#23140=CARTESIAN_POINT('Ctrl Pts',(-54.0568667911089,-104.438327089904,
175.985484901271));
#23141=CARTESIAN_POINT('Ctrl Pts',(-54.0469287973088,-104.34510531788,174.324310296203));
#23142=CARTESIAN_POINT('Ctrl Pts',(-55.2050001585973,-104.127365945257,
173.149682517375));
#23143=CARTESIAN_POINT('Ctrl Pts',(-56.3630715198858,-103.909626572634,
171.975054738546));
#23144=CARTESIAN_POINT('Ctrl Pts',(-58.0049481565429,-103.640310325404,
171.975054808055));
#23145=CARTESIAN_POINT('Ctrl Pts',(-59.6468247932,-103.370994078175,171.975054877564));
#23146=CARTESIAN_POINT('Ctrl Pts',(-60.8048960567424,-103.153254715972,
173.149682754692));
#23147=CARTESIAN_POINT('Ctrl Pts',(-61.9629673202849,-102.93551535377,174.32431063182));
#23148=CARTESIAN_POINT('Ctrl Pts',(-61.9530291882509,-102.842293596483,
175.985485236888));
#23149=CARTESIAN_POINT('Ctrl Pts',(-61.943091056217,-102.749071839196,177.646659841956));
#23150=CARTESIAN_POINT('Ctrl Pts',(-60.7651435690945,-102.780367682508,
178.821287620784));
#23151=CARTESIAN_POINT('Ctrl Pts',(-59.587196081972,-102.81166352582,179.995915399612));
#23152=CARTESIAN_POINT('Ctrl Pts',(-57.9254433194808,-102.894536243739,
179.995915330104));
#23153=CARTESIAN_POINT('Ctrl Pts',(-56.2636905569897,-102.977408961658,
179.995915260595));
#23154=CARTESIAN_POINT('Ctrl Pts',(-55.0857431676132,-103.00870479455,178.821287383467));
#23155=CARTESIAN_POINT('Ctrl Pts',(-53.9077957782368,-103.040000627442,
177.646659506339));
#23156=CARTESIAN_POINT('Ctrl Pts',(-53.8978577844367,-102.946778855418,
175.985484901271));
#23157=CARTESIAN_POINT('Ctrl Pts',(-53.8879197906366,-102.853557083394,
174.324310296203));
#23158=CARTESIAN_POINT('Ctrl Pts',(-55.0459911519251,-102.635817710771,
173.149682517375));
#23159=CARTESIAN_POINT('Ctrl Pts',(-56.2040625132136,-102.418078338148,
171.975054738546));
#23160=CARTESIAN_POINT('Ctrl Pts',(-57.8459391498707,-102.148762090919,
171.975054808055));
#23161=CARTESIAN_POINT('Ctrl Pts',(-59.4878157865278,-101.879445843689,
171.975054877564));
#23162=CARTESIAN_POINT('Ctrl Pts',(-60.6458870500702,-101.661706481487,
173.149682754692));
#23163=CARTESIAN_POINT('Ctrl Pts',(-61.8039583136126,-101.443967119284,
174.32431063182));
#23164=CARTESIAN_POINT('Ctrl Pts',(-61.7940201815787,-101.350745361997,
175.985485236888));
#23165=CARTESIAN_POINT('Ctrl Pts',(-61.7840820495448,-101.25752360471,177.646659841956));
#23166=CARTESIAN_POINT('Ctrl Pts',(-60.6061345624222,-101.288819448022,
178.821287620784));
#23167=CARTESIAN_POINT('Ctrl Pts',(-59.4281870752997,-101.320115291335,
179.995915399612));
#23168=CARTESIAN_POINT('Ctrl Pts',(-57.7664343128086,-101.402988009253,
179.995915330104));
#23169=CARTESIAN_POINT('Ctrl Pts',(-56.1046815503175,-101.485860727172,
179.995915260595));
#23170=CARTESIAN_POINT('Ctrl Pts',(-54.926734160941,-101.517156560064,178.821287383467));
#23171=CARTESIAN_POINT('Ctrl Pts',(-53.7487867715645,-101.548452392956,
177.646659506339));
#23172=CARTESIAN_POINT('Ctrl Pts',(-53.7388487777644,-101.455230620932,
175.985484901271));
#23173=CARTESIAN_POINT('Ctrl Pts',(-53.7289107839643,-101.362008848909,
174.324310296203));
#23174=CARTESIAN_POINT('Ctrl Pts',(-54.8869821452528,-101.144269476286,
173.149682517375));
#23175=CARTESIAN_POINT('Ctrl Pts',(-56.0450535065414,-100.926530103662,
171.975054738546));
#23176=CARTESIAN_POINT('Ctrl Pts',(-57.6869301431984,-100.657213856433,
171.975054808055));
#23177=CARTESIAN_POINT('Ctrl Pts',(-59.3288067798556,-100.387897609204,
171.975054877564));
#23178=CARTESIAN_POINT('Ctrl Pts',(-60.486878043398,-100.170158247001,173.149682754692));
#23179=CARTESIAN_POINT('Ctrl Pts',(-61.6449493069404,-99.9524188847983,
174.32431063182));
#23180=CARTESIAN_POINT('Ctrl Pts',(-61.6350111749065,-99.8591971275113,
175.985485236888));
#23181=CARTESIAN_POINT('Ctrl Pts',(-61.6250730428726,-99.7659753702243,
177.646659841956));
#23182=CARTESIAN_POINT('Ctrl Pts',(-60.44712555575,-99.7972712135367,178.821287620784));
#23183=CARTESIAN_POINT('Ctrl Pts',(-59.2691780686275,-99.8285670568492,
179.995915399612));
#23184=CARTESIAN_POINT('Ctrl Pts',(-57.6074253061363,-99.9114397747677,
179.995915330104));
#23185=CARTESIAN_POINT('Ctrl Pts',(-55.9456725436452,-99.9943124926864,
179.995915260595));
#23186=CARTESIAN_POINT('Ctrl Pts',(-54.7677251542687,-100.025608325578,
178.821287383467));
#23187=CARTESIAN_POINT('Ctrl Pts',(-53.5897777648923,-100.05690415847,177.646659506339));
#23188=CARTESIAN_POINT('Ctrl Pts',(-53.5798397710922,-99.9636823864468,
175.985484901271));
#23189=CARTESIAN_POINT('Ctrl Pts',(-53.5699017772921,-99.8704606144232,
174.324310296203));
#23190=CARTESIAN_POINT('Ctrl Pts',(-54.7279731385806,-99.6527212418,173.149682517375));
#23191=CARTESIAN_POINT('Ctrl Pts',(-55.8860444998691,-99.4349818691769,
171.975054738546));
#23192=CARTESIAN_POINT('Ctrl Pts',(-57.5279211365262,-99.1656656219475,
171.975054808055));
#23193=CARTESIAN_POINT('Ctrl Pts',(-59.1697977731833,-98.8963493747183,
171.975054877564));
#23194=CARTESIAN_POINT('Ctrl Pts',(-60.3278690367257,-98.6786100125155,
173.149682754692));
#23195=CARTESIAN_POINT('Ctrl Pts',(-61.4859403002682,-98.4608706503128,
174.32431063182));
#23196=CARTESIAN_POINT('Ctrl Pts',(-61.4760021682342,-98.3676488930257,
175.985485236888));
#23197=CARTESIAN_POINT('Ctrl Pts',(-61.4660640362003,-98.2744271357387,
177.646659841956));
#23198=CARTESIAN_POINT('Ctrl Pts',(-60.2881165490778,-98.3057229790511,
178.821287620784));
#23199=CARTESIAN_POINT('Ctrl Pts',(-59.1101690619552,-98.3370188223636,
179.995915399612));
#23200=CARTESIAN_POINT('Ctrl Pts',(-57.4484162994641,-98.4198915402821,
179.995915330104));
#23201=CARTESIAN_POINT('Ctrl Pts',(-55.786663536973,-98.5027642582008,179.995915260595));
#23202=CARTESIAN_POINT('Ctrl Pts',(-54.6087161475965,-98.5340600910929,
178.821287383467));
#23203=CARTESIAN_POINT('Ctrl Pts',(-56.2237961054143,-113.614380048479,
178.813912075476));
#23204=CARTESIAN_POINT('Ctrl Pts',(-55.0488864554725,-113.645352038053,
177.6423391512));
#23205=CARTESIAN_POINT('Ctrl Pts',(-55.0389484614927,-113.552130266048,
175.985484901707));
#23206=CARTESIAN_POINT('Ctrl Pts',(-55.0290104675128,-113.458908494044,
174.328630652215));
#23207=CARTESIAN_POINT('Ctrl Pts',(-56.1840440891124,-113.241492964766,
173.157057825983));
#23208=CARTESIAN_POINT('Ctrl Pts',(-57.3390777107121,-113.024077435489,
171.985484999752));
#23209=CARTESIAN_POINT('Ctrl Pts',(-58.9766583348819,-112.755219171892,
171.985485069079));
#23210=CARTESIAN_POINT('Ctrl Pts',(-60.6142389590518,-112.486360908295,
171.985485138407));
#23211=CARTESIAN_POINT('Ctrl Pts',(-61.7692724831595,-112.268945389411,
173.157058062683));
#23212=CARTESIAN_POINT('Ctrl Pts',(-62.9243060072673,-112.051529870527,
174.328630986959));
#23213=CARTESIAN_POINT('Ctrl Pts',(-62.9143678754131,-111.95830811322,175.985485236451));
#23214=CARTESIAN_POINT('Ctrl Pts',(-62.9044297435589,-111.865086355914,
177.642339485944));
#23215=CARTESIAN_POINT('Ctrl Pts',(-61.7295199961253,-111.896058355881,
178.813912312176));
#23216=CARTESIAN_POINT('Ctrl Pts',(-60.5546102486917,-111.927030355848,
179.985485138407));
#23217=CARTESIAN_POINT('Ctrl Pts',(-58.8971534986878,-112.009445090134,
179.985485069079));
#23218=CARTESIAN_POINT('Ctrl Pts',(-57.2396967486839,-112.09185982442,179.985484999752));
#23219=CARTESIAN_POINT('Ctrl Pts',(-56.0647870987421,-112.122831813994,
178.813912075476));
#23220=CARTESIAN_POINT('Ctrl Pts',(-54.8898774488003,-112.153803803567,
177.6423391512));
#23221=CARTESIAN_POINT('Ctrl Pts',(-54.8799394548205,-112.060582031563,
175.985484901707));
#23222=CARTESIAN_POINT('Ctrl Pts',(-54.8700014608406,-111.967360259558,
174.328630652215));
#23223=CARTESIAN_POINT('Ctrl Pts',(-56.0250350824402,-111.749944730281,
173.157057825983));
#23224=CARTESIAN_POINT('Ctrl Pts',(-57.1800687040398,-111.532529201003,
171.985484999752));
#23225=CARTESIAN_POINT('Ctrl Pts',(-58.8176493282097,-111.263670937406,
171.985485069079));
#23226=CARTESIAN_POINT('Ctrl Pts',(-60.4552299523796,-110.994812673809,
171.985485138407));
#23227=CARTESIAN_POINT('Ctrl Pts',(-61.6102634764873,-110.777397154925,
173.157058062683));
#23228=CARTESIAN_POINT('Ctrl Pts',(-62.7652970005951,-110.559981636041,
174.328630986959));
#23229=CARTESIAN_POINT('Ctrl Pts',(-62.7553588687409,-110.466759878735,
175.985485236451));
#23230=CARTESIAN_POINT('Ctrl Pts',(-62.7454207368867,-110.373538121429,
177.642339485944));
#23231=CARTESIAN_POINT('Ctrl Pts',(-61.5705109894531,-110.404510121395,
178.813912312176));
#23232=CARTESIAN_POINT('Ctrl Pts',(-60.3956012420194,-110.435482121362,
179.985485138407));
#23233=CARTESIAN_POINT('Ctrl Pts',(-58.7381444920155,-110.517896855648,
179.985485069079));
#23234=CARTESIAN_POINT('Ctrl Pts',(-57.0806877420116,-110.600311589935,
179.985484999752));
#23235=CARTESIAN_POINT('Ctrl Pts',(-55.9057780920699,-110.631283579508,
178.813912075476));
#23236=CARTESIAN_POINT('Ctrl Pts',(-54.7308684421281,-110.662255569082,
177.6423391512));
#23237=CARTESIAN_POINT('Ctrl Pts',(-54.7209304481482,-110.569033797077,
175.985484901707));
#23238=CARTESIAN_POINT('Ctrl Pts',(-54.7109924541684,-110.475812025073,
174.328630652215));
#23239=CARTESIAN_POINT('Ctrl Pts',(-55.866026075768,-110.258396495795,173.157057825983));
#23240=CARTESIAN_POINT('Ctrl Pts',(-57.0210596973676,-110.040980966518,
171.985484999752));
#23241=CARTESIAN_POINT('Ctrl Pts',(-58.6586403215375,-109.772122702921,
171.985485069079));
#23242=CARTESIAN_POINT('Ctrl Pts',(-60.2962209457073,-109.503264439324,
171.985485138407));
#23243=CARTESIAN_POINT('Ctrl Pts',(-61.4512544698151,-109.28584892044,173.157058062683));
#23244=CARTESIAN_POINT('Ctrl Pts',(-62.6062879939228,-109.068433401555,
174.328630986959));
#23245=CARTESIAN_POINT('Ctrl Pts',(-62.5963498620687,-108.975211644249,
175.985485236451));
#23246=CARTESIAN_POINT('Ctrl Pts',(-62.5864117302145,-108.881989886943,
177.642339485944));
#23247=CARTESIAN_POINT('Ctrl Pts',(-61.4115019827808,-108.91296188691,178.813912312176));
#23248=CARTESIAN_POINT('Ctrl Pts',(-60.2365922353472,-108.943933886877,
179.985485138407));
#23249=CARTESIAN_POINT('Ctrl Pts',(-58.5791354853433,-109.026348621163,
179.985485069079));
#23250=CARTESIAN_POINT('Ctrl Pts',(-56.9216787353394,-109.108763355449,
179.985484999752));
#23251=CARTESIAN_POINT('Ctrl Pts',(-55.7467690853976,-109.139735345023,
178.813912075476));
#23252=CARTESIAN_POINT('Ctrl Pts',(-54.5718594354559,-109.170707334596,
177.6423391512));
#23253=CARTESIAN_POINT('Ctrl Pts',(-54.561921441476,-109.077485562592,175.985484901707));
#23254=CARTESIAN_POINT('Ctrl Pts',(-54.5519834474962,-108.984263790587,
174.328630652215));
#23255=CARTESIAN_POINT('Ctrl Pts',(-55.7070170690958,-108.76684826131,173.157057825983));
#23256=CARTESIAN_POINT('Ctrl Pts',(-56.8620506906954,-108.549432732032,
171.985484999752));
#23257=CARTESIAN_POINT('Ctrl Pts',(-58.4996313148652,-108.280574468435,
171.985485069079));
#23258=CARTESIAN_POINT('Ctrl Pts',(-60.1372119390351,-108.011716204838,
171.985485138407));
#23259=CARTESIAN_POINT('Ctrl Pts',(-61.2922454631428,-107.794300685954,
173.157058062683));
#23260=CARTESIAN_POINT('Ctrl Pts',(-62.4472789872506,-107.57688516707,174.328630986959));
#23261=CARTESIAN_POINT('Ctrl Pts',(-62.4373408553964,-107.483663409764,
175.985485236451));
#23262=CARTESIAN_POINT('Ctrl Pts',(-62.4274027235423,-107.390441652457,
177.642339485944));
#23263=CARTESIAN_POINT('Ctrl Pts',(-61.2524929761086,-107.421413652424,
178.813912312176));
#23264=CARTESIAN_POINT('Ctrl Pts',(-60.077583228675,-107.452385652391,179.985485138407));
#23265=CARTESIAN_POINT('Ctrl Pts',(-58.4201264786711,-107.534800386677,
179.985485069079));
#23266=CARTESIAN_POINT('Ctrl Pts',(-56.7626697286672,-107.617215120964,
179.985484999752));
#23267=CARTESIAN_POINT('Ctrl Pts',(-55.5877600787254,-107.648187110537,
178.813912075476));
#23268=CARTESIAN_POINT('Ctrl Pts',(-54.4128504287836,-107.67915910011,177.6423391512));
#23269=CARTESIAN_POINT('Ctrl Pts',(-54.4029124348038,-107.585937328106,
175.985484901707));
#23270=CARTESIAN_POINT('Ctrl Pts',(-54.3929744408239,-107.492715556102,
174.328630652215));
#23271=CARTESIAN_POINT('Ctrl Pts',(-55.5480080624235,-107.275300026824,
173.157057825983));
#23272=CARTESIAN_POINT('Ctrl Pts',(-56.7030416840231,-107.057884497547,
171.985484999752));
#23273=CARTESIAN_POINT('Ctrl Pts',(-58.340622308193,-106.78902623395,171.985485069079));
#23274=CARTESIAN_POINT('Ctrl Pts',(-59.9782029323629,-106.520167970353,
171.985485138407));
#23275=CARTESIAN_POINT('Ctrl Pts',(-61.1332364564706,-106.302752451468,
173.157058062683));
#23276=CARTESIAN_POINT('Ctrl Pts',(-62.2882699805784,-106.085336932584,
174.328630986959));
#23277=CARTESIAN_POINT('Ctrl Pts',(-62.2783318487242,-105.992115175278,
175.985485236451));
#23278=CARTESIAN_POINT('Ctrl Pts',(-62.26839371687,-105.898893417972,177.642339485944));
#23279=CARTESIAN_POINT('Ctrl Pts',(-61.0934839694364,-105.929865417939,
178.813912312176));
#23280=CARTESIAN_POINT('Ctrl Pts',(-59.9185742220028,-105.960837417905,
179.985485138407));
#23281=CARTESIAN_POINT('Ctrl Pts',(-58.2611174719989,-106.043252152192,
179.985485069079));
#23282=CARTESIAN_POINT('Ctrl Pts',(-56.603660721995,-106.125666886478,179.985484999752));
#23283=CARTESIAN_POINT('Ctrl Pts',(-55.4287510720532,-106.156638876051,
178.813912075476));
#23284=CARTESIAN_POINT('Ctrl Pts',(-54.2538414221114,-106.187610865625,
177.6423391512));
#23285=CARTESIAN_POINT('Ctrl Pts',(-54.2439034281315,-106.09438909362,175.985484901707));
#23286=CARTESIAN_POINT('Ctrl Pts',(-54.2339654341517,-106.001167321616,
174.328630652215));
#23287=CARTESIAN_POINT('Ctrl Pts',(-55.3889990557513,-105.783751792338,
173.157057825983));
#23288=CARTESIAN_POINT('Ctrl Pts',(-56.5440326773509,-105.566336263061,
171.985484999752));
#23289=CARTESIAN_POINT('Ctrl Pts',(-58.1816133015208,-105.297477999464,
171.985485069079));
#23290=CARTESIAN_POINT('Ctrl Pts',(-59.8191939256906,-105.028619735867,
171.985485138407));
#23291=CARTESIAN_POINT('Ctrl Pts',(-60.9742274497984,-104.811204216983,
173.157058062683));
#23292=CARTESIAN_POINT('Ctrl Pts',(-62.1292609739061,-104.593788698099,
174.328630986959));
#23293=CARTESIAN_POINT('Ctrl Pts',(-62.119322842052,-104.500566940792,175.985485236451));
#23294=CARTESIAN_POINT('Ctrl Pts',(-62.1093847101978,-104.407345183486,
177.642339485944));
#23295=CARTESIAN_POINT('Ctrl Pts',(-60.9344749627642,-104.438317183453,
178.813912312176));
#23296=CARTESIAN_POINT('Ctrl Pts',(-59.7595652153305,-104.46928918342,179.985485138407));
#23297=CARTESIAN_POINT('Ctrl Pts',(-58.1021084653266,-104.551703917706,
179.985485069079));
#23298=CARTESIAN_POINT('Ctrl Pts',(-56.4446517153227,-104.634118651992,
179.985484999752));
#23299=CARTESIAN_POINT('Ctrl Pts',(-55.269742065381,-104.665090641566,178.813912075476));
#23300=CARTESIAN_POINT('Ctrl Pts',(-54.0948324154392,-104.696062631139,
177.6423391512));
#23301=CARTESIAN_POINT('Ctrl Pts',(-54.0848944214593,-104.602840859135,
175.985484901707));
#23302=CARTESIAN_POINT('Ctrl Pts',(-54.0749564274795,-104.50961908713,174.328630652215));
#23303=CARTESIAN_POINT('Ctrl Pts',(-55.2299900490791,-104.292203557853,
173.157057825983));
#23304=CARTESIAN_POINT('Ctrl Pts',(-56.3850236706787,-104.074788028575,
171.985484999752));
#23305=CARTESIAN_POINT('Ctrl Pts',(-58.0226042948486,-103.805929764978,
171.985485069079));
#23306=CARTESIAN_POINT('Ctrl Pts',(-59.6601849190184,-103.537071501381,
171.985485138407));
#23307=CARTESIAN_POINT('Ctrl Pts',(-60.8152184431262,-103.319655982497,
173.157058062683));
#23308=CARTESIAN_POINT('Ctrl Pts',(-61.9702519672339,-103.102240463613,
174.328630986959));
#23309=CARTESIAN_POINT('Ctrl Pts',(-61.9603138353797,-103.009018706307,
175.985485236451));
#23310=CARTESIAN_POINT('Ctrl Pts',(-61.9503757035256,-102.915796949001,
177.642339485944));
#23311=CARTESIAN_POINT('Ctrl Pts',(-60.7754659560919,-102.946768948967,
178.813912312176));
#23312=CARTESIAN_POINT('Ctrl Pts',(-59.6005562086583,-102.977740948934,
179.985485138407));
#23313=CARTESIAN_POINT('Ctrl Pts',(-57.9430994586544,-103.06015568322,179.985485069079));
#23314=CARTESIAN_POINT('Ctrl Pts',(-56.2856427086505,-103.142570417507,
179.985484999752));
#23315=CARTESIAN_POINT('Ctrl Pts',(-55.1107330587087,-103.17354240708,178.813912075476));
#23316=CARTESIAN_POINT('Ctrl Pts',(-53.935823408767,-103.204514396654,177.6423391512));
#23317=CARTESIAN_POINT('Ctrl Pts',(-53.9258854147871,-103.111292624649,
175.985484901707));
#23318=CARTESIAN_POINT('Ctrl Pts',(-53.9159474208072,-103.018070852645,
174.328630652215));
#23319=CARTESIAN_POINT('Ctrl Pts',(-55.0709810424069,-102.800655323367,
173.157057825983));
#23320=CARTESIAN_POINT('Ctrl Pts',(-56.2260146640065,-102.58323979409,171.985484999752));
#23321=CARTESIAN_POINT('Ctrl Pts',(-57.8635952881763,-102.314381530493,
171.985485069079));
#23322=CARTESIAN_POINT('Ctrl Pts',(-59.5011759123462,-102.045523266896,
171.985485138407));
#23323=CARTESIAN_POINT('Ctrl Pts',(-60.6562094364539,-101.828107748012,
173.157058062683));
#23324=CARTESIAN_POINT('Ctrl Pts',(-61.8112429605617,-101.610692229127,
174.328630986959));
#23325=CARTESIAN_POINT('Ctrl Pts',(-61.8013048287075,-101.517470471821,
175.985485236451));
#23326=CARTESIAN_POINT('Ctrl Pts',(-61.7913666968533,-101.424248714515,
177.642339485944));
#23327=CARTESIAN_POINT('Ctrl Pts',(-60.6164569494197,-101.455220714482,
178.813912312176));
#23328=CARTESIAN_POINT('Ctrl Pts',(-59.4415472019861,-101.486192714449,
179.985485138407));
#23329=CARTESIAN_POINT('Ctrl Pts',(-57.7840904519822,-101.568607448735,
179.985485069079));
#23330=CARTESIAN_POINT('Ctrl Pts',(-56.1266337019783,-101.651022183021,
179.985484999752));
#23331=CARTESIAN_POINT('Ctrl Pts',(-54.9517240520365,-101.681994172595,
178.813912075476));
#23332=CARTESIAN_POINT('Ctrl Pts',(-53.7768144020947,-101.712966162168,
177.6423391512));
#23333=CARTESIAN_POINT('Ctrl Pts',(-53.7668764081149,-101.619744390164,
175.985484901707));
#23334=CARTESIAN_POINT('Ctrl Pts',(-53.756938414135,-101.526522618159,174.328630652215));
#23335=CARTESIAN_POINT('Ctrl Pts',(-54.9119720357346,-101.309107088882,
173.157057825983));
#23336=CARTESIAN_POINT('Ctrl Pts',(-56.0670056573342,-101.091691559604,
171.985484999752));
#23337=CARTESIAN_POINT('Ctrl Pts',(-57.7045862815041,-100.822833296007,
171.985485069079));
#23338=CARTESIAN_POINT('Ctrl Pts',(-59.342166905674,-100.55397503241,171.985485138407));
#23339=CARTESIAN_POINT('Ctrl Pts',(-60.4972004297817,-100.336559513526,
173.157058062683));
#23340=CARTESIAN_POINT('Ctrl Pts',(-61.6522339538895,-100.119143994642,
174.328630986959));
#23341=CARTESIAN_POINT('Ctrl Pts',(-61.6422958220353,-100.025922237336,
175.985485236451));
#23342=CARTESIAN_POINT('Ctrl Pts',(-61.6323576901811,-99.9327004800294,
177.642339485944));
#23343=CARTESIAN_POINT('Ctrl Pts',(-60.4574479427475,-99.9636724799962,
178.813912312176));
#23344=CARTESIAN_POINT('Ctrl Pts',(-59.2825381953138,-99.994644479963,179.985485138407));
#23345=CARTESIAN_POINT('Ctrl Pts',(-57.6250814453099,-100.077059214249,
179.985485069079));
#23346=CARTESIAN_POINT('Ctrl Pts',(-55.9676246953061,-100.159473948536,
179.985484999752));
#23347=CARTESIAN_POINT('Ctrl Pts',(-54.7927150453643,-100.190445938109,
178.813912075476));
#23348=CARTESIAN_POINT('Ctrl Pts',(-53.6178053954225,-100.221417927683,
177.6423391512));
#23349=CARTESIAN_POINT('Ctrl Pts',(-53.6078674014426,-100.128196155678,
175.985484901707));
#23350=CARTESIAN_POINT('Ctrl Pts',(-53.5979294074628,-100.034974383673,
174.328630652215));
#23351=CARTESIAN_POINT('Ctrl Pts',(-54.7529630290624,-99.817558854396,173.157057825983));
#23352=CARTESIAN_POINT('Ctrl Pts',(-55.907996650662,-99.6001433251185,171.985484999752));
#23353=CARTESIAN_POINT('Ctrl Pts',(-57.5455772748319,-99.3312850615215,
171.985485069079));
#23354=CARTESIAN_POINT('Ctrl Pts',(-59.1831578990017,-99.0624267979246,
171.985485138407));
#23355=CARTESIAN_POINT('Ctrl Pts',(-60.3381914231095,-98.8450112790404,
173.157058062683));
#23356=CARTESIAN_POINT('Ctrl Pts',(-61.4932249472172,-98.6275957601562,
174.328630986959));
#23357=CARTESIAN_POINT('Ctrl Pts',(-61.4832868153631,-98.53437400285,175.985485236451));
#23358=CARTESIAN_POINT('Ctrl Pts',(-61.4733486835089,-98.4411522455438,
177.642339485944));
#23359=CARTESIAN_POINT('Ctrl Pts',(-60.2984389360752,-98.4721242455106,
178.813912312176));
#23360=CARTESIAN_POINT('Ctrl Pts',(-59.1235291886416,-98.5030962454774,
179.985485138407));
#23361=CARTESIAN_POINT('Ctrl Pts',(-57.4660724386377,-98.5855109797636,
179.985485069079));
#23362=CARTESIAN_POINT('Ctrl Pts',(-55.8086156886338,-98.6679257140499,
179.985484999752));
#23363=CARTESIAN_POINT('Ctrl Pts',(-54.633706038692,-98.6988977036234,178.813912075476));
#23364=CARTESIAN_POINT('Ctrl Pts',(-56.8733667677527,-112.709647553905,
178.072094410988));
#23365=CARTESIAN_POINT('Ctrl Pts',(-56.0039967339745,-112.708046979118,
177.207792449865));
#23366=CARTESIAN_POINT('Ctrl Pts',(-55.9940587219143,-112.614825209041,
175.985484945604));
#23367=CARTESIAN_POINT('Ctrl Pts',(-55.9841207098542,-112.521603438964,
174.763177441344));
#23368=CARTESIAN_POINT('Ctrl Pts',(-56.8336146897208,-112.336760476773,
173.89887555255));
#23369=CARTESIAN_POINT('Ctrl Pts',(-57.6831086695875,-112.151917514582,
173.034573663757));
#23370=CARTESIAN_POINT('Ctrl Pts',(-58.8885910066563,-111.929123815193,
173.034573714903));
#23371=CARTESIAN_POINT('Ctrl Pts',(-60.0940733437252,-111.706330115804,
173.034573766048));
#23372=CARTESIAN_POINT('Ctrl Pts',(-60.9435672516694,-111.521487161281,
173.898875727171));
#23373=CARTESIAN_POINT('Ctrl Pts',(-61.7930611596136,-111.336644206758,
174.763177688294));
#23374=CARTESIAN_POINT('Ctrl Pts',(-61.7831230458397,-111.243422447524,
175.985485192554));
#23375=CARTESIAN_POINT('Ctrl Pts',(-61.7731849320658,-111.15020068829,177.207792696815));
#23376=CARTESIAN_POINT('Ctrl Pts',(-60.9038148263651,-111.14860012117,178.072094585608));
#23377=CARTESIAN_POINT('Ctrl Pts',(-60.0344447206644,-111.14699955405,178.936396474401));
#23378=CARTESIAN_POINT('Ctrl Pts',(-58.8090862577616,-111.183349724129,
178.936396423256));
#23379=CARTESIAN_POINT('Ctrl Pts',(-57.5837277948587,-111.219699894207,
178.936396372111));
#23380=CARTESIAN_POINT('Ctrl Pts',(-56.7143577610805,-111.21809931942,178.072094410988));
#23381=CARTESIAN_POINT('Ctrl Pts',(-55.8449877273022,-111.216498744632,
177.207792449865));
#23382=CARTESIAN_POINT('Ctrl Pts',(-55.8350497152421,-111.123276974555,
175.985484945604));
#23383=CARTESIAN_POINT('Ctrl Pts',(-55.8251117031819,-111.030055204478,
174.763177441344));
#23384=CARTESIAN_POINT('Ctrl Pts',(-56.6746056830486,-110.845212242287,
173.89887555255));
#23385=CARTESIAN_POINT('Ctrl Pts',(-57.5240996629153,-110.660369280097,
173.034573663757));
#23386=CARTESIAN_POINT('Ctrl Pts',(-58.7295819999841,-110.437575580708,
173.034573714903));
#23387=CARTESIAN_POINT('Ctrl Pts',(-59.9350643370529,-110.214781881319,
173.034573766048));
#23388=CARTESIAN_POINT('Ctrl Pts',(-60.7845582449971,-110.029938926795,
173.898875727171));
#23389=CARTESIAN_POINT('Ctrl Pts',(-61.6340521529414,-109.845095972272,
174.763177688294));
#23390=CARTESIAN_POINT('Ctrl Pts',(-61.6241140391675,-109.751874213038,
175.985485192554));
#23391=CARTESIAN_POINT('Ctrl Pts',(-61.6141759253936,-109.658652453805,
177.207792696815));
#23392=CARTESIAN_POINT('Ctrl Pts',(-60.7448058196929,-109.657051886685,
178.072094585608));
#23393=CARTESIAN_POINT('Ctrl Pts',(-59.8754357139922,-109.655451319565,
178.936396474401));
#23394=CARTESIAN_POINT('Ctrl Pts',(-58.6500772510893,-109.691801489643,
178.936396423256));
#23395=CARTESIAN_POINT('Ctrl Pts',(-57.4247187881865,-109.728151659721,
178.936396372111));
#23396=CARTESIAN_POINT('Ctrl Pts',(-56.5553487544082,-109.726551084934,
178.072094410988));
#23397=CARTESIAN_POINT('Ctrl Pts',(-55.68597872063,-109.724950510147,177.207792449865));
#23398=CARTESIAN_POINT('Ctrl Pts',(-55.6760407085698,-109.63172874007,175.985484945604));
#23399=CARTESIAN_POINT('Ctrl Pts',(-55.6661026965097,-109.538506969993,
174.763177441344));
#23400=CARTESIAN_POINT('Ctrl Pts',(-56.5155966763764,-109.353664007802,
173.89887555255));
#23401=CARTESIAN_POINT('Ctrl Pts',(-57.365090656243,-109.168821045611,173.034573663757));
#23402=CARTESIAN_POINT('Ctrl Pts',(-58.5705729933119,-108.946027346222,
173.034573714903));
#23403=CARTESIAN_POINT('Ctrl Pts',(-59.7760553303807,-108.723233646833,
173.034573766048));
#23404=CARTESIAN_POINT('Ctrl Pts',(-60.6255492383249,-108.53839069231,173.898875727171));
#23405=CARTESIAN_POINT('Ctrl Pts',(-61.4750431462691,-108.353547737786,
174.763177688294));
#23406=CARTESIAN_POINT('Ctrl Pts',(-61.4651050324952,-108.260325978553,
175.985485192554));
#23407=CARTESIAN_POINT('Ctrl Pts',(-61.4551669187214,-108.167104219319,
177.207792696815));
#23408=CARTESIAN_POINT('Ctrl Pts',(-60.5857968130207,-108.165503652199,
178.072094585608));
#23409=CARTESIAN_POINT('Ctrl Pts',(-59.71642670732,-108.163903085079,178.936396474401));
#23410=CARTESIAN_POINT('Ctrl Pts',(-58.4910682444171,-108.200253255158,
178.936396423256));
#23411=CARTESIAN_POINT('Ctrl Pts',(-57.2657097815143,-108.236603425236,
178.936396372111));
#23412=CARTESIAN_POINT('Ctrl Pts',(-56.396339747736,-108.235002850448,178.072094410988));
#23413=CARTESIAN_POINT('Ctrl Pts',(-55.5269697139578,-108.233402275661,
177.207792449865));
#23414=CARTESIAN_POINT('Ctrl Pts',(-55.5170317018976,-108.140180505584,
175.985484945604));
#23415=CARTESIAN_POINT('Ctrl Pts',(-55.5070936898375,-108.046958735507,
174.763177441344));
#23416=CARTESIAN_POINT('Ctrl Pts',(-56.3565876697041,-107.862115773316,
173.89887555255));
#23417=CARTESIAN_POINT('Ctrl Pts',(-57.2060816495708,-107.677272811126,
173.034573663757));
#23418=CARTESIAN_POINT('Ctrl Pts',(-58.4115639866396,-107.454479111736,
173.034573714903));
#23419=CARTESIAN_POINT('Ctrl Pts',(-59.6170463237085,-107.231685412347,
173.034573766048));
#23420=CARTESIAN_POINT('Ctrl Pts',(-60.4665402316527,-107.046842457824,
173.898875727171));
#23421=CARTESIAN_POINT('Ctrl Pts',(-61.3160341395969,-106.861999503301,
174.763177688294));
#23422=CARTESIAN_POINT('Ctrl Pts',(-61.306096025823,-106.768777744067,175.985485192554));
#23423=CARTESIAN_POINT('Ctrl Pts',(-61.2961579120492,-106.675555984834,
177.207792696815));
#23424=CARTESIAN_POINT('Ctrl Pts',(-60.4267878063484,-106.673955417714,
178.072094585608));
#23425=CARTESIAN_POINT('Ctrl Pts',(-59.5574177006478,-106.672354850594,
178.936396474401));
#23426=CARTESIAN_POINT('Ctrl Pts',(-58.3320592377449,-106.708705020672,
178.936396423256));
#23427=CARTESIAN_POINT('Ctrl Pts',(-57.106700774842,-106.74505519075,178.936396372111));
#23428=CARTESIAN_POINT('Ctrl Pts',(-56.2373307410638,-106.743454615963,
178.072094410988));
#23429=CARTESIAN_POINT('Ctrl Pts',(-55.3679607072856,-106.741854041175,
177.207792449865));
#23430=CARTESIAN_POINT('Ctrl Pts',(-55.3580226952254,-106.648632271098,
175.985484945604));
#23431=CARTESIAN_POINT('Ctrl Pts',(-55.3480846831652,-106.555410501021,
174.763177441344));
#23432=CARTESIAN_POINT('Ctrl Pts',(-56.1975786630319,-106.370567538831,
173.89887555255));
#23433=CARTESIAN_POINT('Ctrl Pts',(-57.0470726428986,-106.18572457664,173.034573663757));
#23434=CARTESIAN_POINT('Ctrl Pts',(-58.2525549799674,-105.962930877251,
173.034573714903));
#23435=CARTESIAN_POINT('Ctrl Pts',(-59.4580373170363,-105.740137177862,
173.034573766048));
#23436=CARTESIAN_POINT('Ctrl Pts',(-60.3075312249805,-105.555294223339,
173.898875727171));
#23437=CARTESIAN_POINT('Ctrl Pts',(-61.1570251329247,-105.370451268815,
174.763177688294));
#23438=CARTESIAN_POINT('Ctrl Pts',(-61.1470870191508,-105.277229509582,
175.985485192554));
#23439=CARTESIAN_POINT('Ctrl Pts',(-61.1371489053769,-105.184007750348,
177.207792696815));
#23440=CARTESIAN_POINT('Ctrl Pts',(-60.2677787996762,-105.182407183228,
178.072094585608));
#23441=CARTESIAN_POINT('Ctrl Pts',(-59.3984086939755,-105.180806616108,
178.936396474401));
#23442=CARTESIAN_POINT('Ctrl Pts',(-58.1730502310727,-105.217156786186,
178.936396423256));
#23443=CARTESIAN_POINT('Ctrl Pts',(-56.9476917681698,-105.253506956265,
178.936396372111));
#23444=CARTESIAN_POINT('Ctrl Pts',(-56.0783217343916,-105.251906381477,
178.072094410988));
#23445=CARTESIAN_POINT('Ctrl Pts',(-55.2089517006133,-105.25030580669,177.207792449865));
#23446=CARTESIAN_POINT('Ctrl Pts',(-55.1990136885532,-105.157084036613,
175.985484945604));
#23447=CARTESIAN_POINT('Ctrl Pts',(-55.189075676493,-105.063862266536,174.763177441344));
#23448=CARTESIAN_POINT('Ctrl Pts',(-56.0385696563597,-104.879019304345,
173.89887555255));
#23449=CARTESIAN_POINT('Ctrl Pts',(-56.8880636362264,-104.694176342154,
173.034573663757));
#23450=CARTESIAN_POINT('Ctrl Pts',(-58.0935459732952,-104.471382642765,
173.034573714903));
#23451=CARTESIAN_POINT('Ctrl Pts',(-59.299028310364,-104.248588943376,173.034573766048));
#23452=CARTESIAN_POINT('Ctrl Pts',(-60.1485222183082,-104.063745988853,
173.898875727171));
#23453=CARTESIAN_POINT('Ctrl Pts',(-60.9980161262524,-103.87890303433,174.763177688294));
#23454=CARTESIAN_POINT('Ctrl Pts',(-60.9880780124786,-103.785681275096,
175.985485192554));
#23455=CARTESIAN_POINT('Ctrl Pts',(-60.9781398987047,-103.692459515862,
177.207792696815));
#23456=CARTESIAN_POINT('Ctrl Pts',(-60.108769793004,-103.690858948742,178.072094585608));
#23457=CARTESIAN_POINT('Ctrl Pts',(-59.2393996873033,-103.689258381622,
178.936396474401));
#23458=CARTESIAN_POINT('Ctrl Pts',(-58.0140412244004,-103.725608551701,
178.936396423256));
#23459=CARTESIAN_POINT('Ctrl Pts',(-56.7886827614976,-103.761958721779,
178.936396372111));
#23460=CARTESIAN_POINT('Ctrl Pts',(-55.9193127277193,-103.760358146992,
178.072094410988));
#23461=CARTESIAN_POINT('Ctrl Pts',(-55.0499426939411,-103.758757572204,
177.207792449865));
#23462=CARTESIAN_POINT('Ctrl Pts',(-55.0400046818809,-103.665535802127,
175.985484945604));
#23463=CARTESIAN_POINT('Ctrl Pts',(-55.0300666698208,-103.57231403205,174.763177441344));
#23464=CARTESIAN_POINT('Ctrl Pts',(-55.8795606496874,-103.387471069859,
173.89887555255));
#23465=CARTESIAN_POINT('Ctrl Pts',(-56.7290546295541,-103.202628107669,
173.034573663757));
#23466=CARTESIAN_POINT('Ctrl Pts',(-57.934536966623,-102.97983440828,173.034573714903));
#23467=CARTESIAN_POINT('Ctrl Pts',(-59.1400193036918,-102.757040708891,
173.034573766048));
#23468=CARTESIAN_POINT('Ctrl Pts',(-59.989513211636,-102.572197754367,173.898875727171));
#23469=CARTESIAN_POINT('Ctrl Pts',(-60.8390071195802,-102.387354799844,
174.763177688294));
#23470=CARTESIAN_POINT('Ctrl Pts',(-60.8290690058063,-102.29413304061,175.985485192554));
#23471=CARTESIAN_POINT('Ctrl Pts',(-60.8191308920325,-102.200911281377,
177.207792696815));
#23472=CARTESIAN_POINT('Ctrl Pts',(-59.9497607863318,-102.199310714257,
178.072094585608));
#23473=CARTESIAN_POINT('Ctrl Pts',(-59.0803906806311,-102.197710147137,
178.936396474401));
#23474=CARTESIAN_POINT('Ctrl Pts',(-57.8550322177282,-102.234060317215,
178.936396423256));
#23475=CARTESIAN_POINT('Ctrl Pts',(-56.6296737548253,-102.270410487293,
178.936396372111));
#23476=CARTESIAN_POINT('Ctrl Pts',(-55.7603037210471,-102.268809912506,
178.072094410988));
#23477=CARTESIAN_POINT('Ctrl Pts',(-54.8909336872689,-102.267209337719,
177.207792449865));
#23478=CARTESIAN_POINT('Ctrl Pts',(-54.8809956752087,-102.173987567642,
175.985484945604));
#23479=CARTESIAN_POINT('Ctrl Pts',(-54.8710576631486,-102.080765797565,
174.763177441344));
#23480=CARTESIAN_POINT('Ctrl Pts',(-55.7205516430152,-101.895922835374,
173.89887555255));
#23481=CARTESIAN_POINT('Ctrl Pts',(-56.5700456228819,-101.711079873183,
173.034573663757));
#23482=CARTESIAN_POINT('Ctrl Pts',(-57.7755279599507,-101.488286173794,
173.034573714903));
#23483=CARTESIAN_POINT('Ctrl Pts',(-58.9810102970196,-101.265492474405,
173.034573766048));
#23484=CARTESIAN_POINT('Ctrl Pts',(-59.8305042049638,-101.080649519882,
173.898875727171));
#23485=CARTESIAN_POINT('Ctrl Pts',(-60.679998112908,-100.895806565358,174.763177688294));
#23486=CARTESIAN_POINT('Ctrl Pts',(-60.6700599991341,-100.802584806125,
175.985485192554));
#23487=CARTESIAN_POINT('Ctrl Pts',(-60.6601218853602,-100.709363046891,
177.207792696815));
#23488=CARTESIAN_POINT('Ctrl Pts',(-59.7907517796595,-100.707762479771,
178.072094585608));
#23489=CARTESIAN_POINT('Ctrl Pts',(-58.9213816739588,-100.706161912651,
178.936396474401));
#23490=CARTESIAN_POINT('Ctrl Pts',(-57.696023211056,-100.742512082729,178.936396423256));
#23491=CARTESIAN_POINT('Ctrl Pts',(-56.4706647481531,-100.778862252808,
178.936396372111));
#23492=CARTESIAN_POINT('Ctrl Pts',(-55.6012947143749,-100.77726167802,178.072094410988));
#23493=CARTESIAN_POINT('Ctrl Pts',(-54.7319246805966,-100.775661103233,
177.207792449865));
#23494=CARTESIAN_POINT('Ctrl Pts',(-54.7219866685365,-100.682439333156,
175.985484945604));
#23495=CARTESIAN_POINT('Ctrl Pts',(-54.7120486564763,-100.589217563079,
174.763177441344));
#23496=CARTESIAN_POINT('Ctrl Pts',(-55.561542636343,-100.404374600888,173.89887555255));
#23497=CARTESIAN_POINT('Ctrl Pts',(-56.4110366162097,-100.219531638698,
173.034573663757));
#23498=CARTESIAN_POINT('Ctrl Pts',(-57.6165189532785,-99.9967379393085,
173.034573714903));
#23499=CARTESIAN_POINT('Ctrl Pts',(-58.8220012903473,-99.7739442399195,
173.034573766048));
#23500=CARTESIAN_POINT('Ctrl Pts',(-59.6714951982915,-99.5891012853962,
173.898875727171));
#23501=CARTESIAN_POINT('Ctrl Pts',(-60.5209891062358,-99.4042583308729,
174.763177688294));
#23502=CARTESIAN_POINT('Ctrl Pts',(-60.5110509924619,-99.3110365716392,
175.985485192554));
#23503=CARTESIAN_POINT('Ctrl Pts',(-60.501112878688,-99.2178148124055,177.207792696815));
#23504=CARTESIAN_POINT('Ctrl Pts',(-59.6317427729873,-99.2162142452855,
178.072094585608));
#23505=CARTESIAN_POINT('Ctrl Pts',(-58.7623726672866,-99.2146136781656,
178.936396474401));
#23506=CARTESIAN_POINT('Ctrl Pts',(-57.5370142043838,-99.2509638482439,
178.936396423256));
#23507=CARTESIAN_POINT('Ctrl Pts',(-56.3116557414809,-99.2873140183222,
178.936396372111));
#23508=CARTESIAN_POINT('Ctrl Pts',(-55.4422857077027,-99.2857134435348,
178.072094410988));
#23509=CARTESIAN_POINT('Ctrl Pts',(-54.5729156739244,-99.2841128687474,
177.207792449865));
#23510=CARTESIAN_POINT('Ctrl Pts',(-54.5629776618643,-99.1908910986704,
175.985484945604));
#23511=CARTESIAN_POINT('Ctrl Pts',(-54.5530396498041,-99.0976693285933,
174.763177441344));
#23512=CARTESIAN_POINT('Ctrl Pts',(-55.4025336296708,-98.9128263664026,
173.89887555255));
#23513=CARTESIAN_POINT('Ctrl Pts',(-56.2520276095374,-98.727983404212,173.034573663757));
#23514=CARTESIAN_POINT('Ctrl Pts',(-57.4575099466063,-98.5051897048229,
173.034573714903));
#23515=CARTESIAN_POINT('Ctrl Pts',(-58.6629922836751,-98.2823960054338,
173.034573766048));
#23516=CARTESIAN_POINT('Ctrl Pts',(-59.5124861916193,-98.0975530509106,
173.898875727171));
#23517=CARTESIAN_POINT('Ctrl Pts',(-60.3619800995635,-97.9127100963873,
174.763177688294));
#23518=CARTESIAN_POINT('Ctrl Pts',(-60.3520419857897,-97.8194883371536,
175.985485192554));
#23519=CARTESIAN_POINT('Ctrl Pts',(-60.3421038720158,-97.7262665779199,
177.207792696815));
#23520=CARTESIAN_POINT('Ctrl Pts',(-59.4727337663151,-97.7246660108,178.072094585608));
#23521=CARTESIAN_POINT('Ctrl Pts',(-58.6033636606144,-97.72306544368,178.936396474401));
#23522=CARTESIAN_POINT('Ctrl Pts',(-57.3780051977115,-97.7594156137583,
178.936396423256));
#23523=CARTESIAN_POINT('Ctrl Pts',(-56.1526467348087,-97.7957657838366,
178.936396372111));
#23524=CARTESIAN_POINT('Ctrl Pts',(-55.2832767010304,-97.7941652090492,
178.072094410988));
#23525=CARTESIAN_POINT('Ctrl Pts',(-56.1707931031902,-113.117197303651,
178.813912075476));
#23526=CARTESIAN_POINT('Ctrl Pts',(-54.9958834532485,-113.148169293224,
177.6423391512));
#23527=CARTESIAN_POINT('Ctrl Pts',(-54.9859454592686,-113.05494752122,175.985484901707));
#23528=CARTESIAN_POINT('Ctrl Pts',(-54.9760074652888,-112.961725749215,
174.328630652215));
#23529=CARTESIAN_POINT('Ctrl Pts',(-56.1310410868884,-112.744310219938,
173.157057825983));
#23530=CARTESIAN_POINT('Ctrl Pts',(-57.286074708488,-112.52689469066,171.985484999752));
#23531=CARTESIAN_POINT('Ctrl Pts',(-58.9236553326579,-112.258036427063,
171.985485069079));
#23532=CARTESIAN_POINT('Ctrl Pts',(-60.5612359568277,-111.989178163466,
171.985485138407));
#23533=CARTESIAN_POINT('Ctrl Pts',(-61.7162694809355,-111.771762644582,
173.157058062683));
#23534=CARTESIAN_POINT('Ctrl Pts',(-62.8713030050432,-111.554347125698,
174.328630986959));
#23535=CARTESIAN_POINT('Ctrl Pts',(-62.861364873189,-111.461125368392,175.985485236451));
#23536=CARTESIAN_POINT('Ctrl Pts',(-62.8514267413349,-111.367903611086,
177.642339485944));
#23537=CARTESIAN_POINT('Ctrl Pts',(-61.6765169939012,-111.398875611052,
178.813912312176));
#23538=CARTESIAN_POINT('Ctrl Pts',(-60.5016072464676,-111.429847611019,
179.985485138407));
#23539=CARTESIAN_POINT('Ctrl Pts',(-58.8441504964637,-111.512262345305,
179.985485069079));
#23540=CARTESIAN_POINT('Ctrl Pts',(-57.1866937464598,-111.594677079592,
179.985484999752));
#23541=CARTESIAN_POINT('Ctrl Pts',(-56.011784096518,-111.625649069165,178.813912075476));
#23542=CARTESIAN_POINT('Ctrl Pts',(-54.8368744465762,-111.656621058739,
177.6423391512));
#23543=CARTESIAN_POINT('Ctrl Pts',(-54.8269364525964,-111.563399286734,
175.985484901707));
#23544=CARTESIAN_POINT('Ctrl Pts',(-54.8169984586165,-111.47017751473,174.328630652215));
#23545=CARTESIAN_POINT('Ctrl Pts',(-55.9720320802161,-111.252761985452,
173.157057825983));
#23546=CARTESIAN_POINT('Ctrl Pts',(-57.1270657018158,-111.035346456175,
171.985484999752));
#23547=CARTESIAN_POINT('Ctrl Pts',(-58.7646463259856,-110.766488192578,
171.985485069079));
#23548=CARTESIAN_POINT('Ctrl Pts',(-60.4022269501555,-110.497629928981,
171.985485138407));
#23549=CARTESIAN_POINT('Ctrl Pts',(-61.5572604742632,-110.280214410097,
173.157058062683));
#23550=CARTESIAN_POINT('Ctrl Pts',(-62.712293998371,-110.062798891212,174.328630986959));
#23551=CARTESIAN_POINT('Ctrl Pts',(-62.7023558665168,-109.969577133906,
175.985485236451));
#23552=CARTESIAN_POINT('Ctrl Pts',(-62.6924177346626,-109.8763553766,177.642339485944));
#23553=CARTESIAN_POINT('Ctrl Pts',(-61.517507987229,-109.907327376567,178.813912312176));
#23554=CARTESIAN_POINT('Ctrl Pts',(-60.3425982397954,-109.938299376534,
179.985485138407));
#23555=CARTESIAN_POINT('Ctrl Pts',(-58.6851414897915,-110.02071411082,179.985485069079));
#23556=CARTESIAN_POINT('Ctrl Pts',(-57.0276847397876,-110.103128845106,
179.985484999752));
#23557=CARTESIAN_POINT('Ctrl Pts',(-55.8527750898458,-110.13410083468,178.813912075476));
#23558=CARTESIAN_POINT('Ctrl Pts',(-54.677865439904,-110.165072824253,177.6423391512));
#23559=CARTESIAN_POINT('Ctrl Pts',(-54.6679274459242,-110.071851052249,
175.985484901707));
#23560=CARTESIAN_POINT('Ctrl Pts',(-54.6579894519443,-109.978629280244,
174.328630652215));
#23561=CARTESIAN_POINT('Ctrl Pts',(-55.8130230735439,-109.761213750967,
173.157057825983));
#23562=CARTESIAN_POINT('Ctrl Pts',(-56.9680566951435,-109.543798221689,
171.985484999752));
#23563=CARTESIAN_POINT('Ctrl Pts',(-58.6056373193134,-109.274939958092,
171.985485069079));
#23564=CARTESIAN_POINT('Ctrl Pts',(-60.2432179434833,-109.006081694495,
171.985485138407));
#23565=CARTESIAN_POINT('Ctrl Pts',(-61.398251467591,-108.788666175611,173.157058062683));
#23566=CARTESIAN_POINT('Ctrl Pts',(-62.5532849916988,-108.571250656727,
174.328630986959));
#23567=CARTESIAN_POINT('Ctrl Pts',(-62.5433468598446,-108.478028899421,
175.985485236451));
#23568=CARTESIAN_POINT('Ctrl Pts',(-62.5334087279904,-108.384807142114,
177.642339485944));
#23569=CARTESIAN_POINT('Ctrl Pts',(-61.3584989805568,-108.415779142081,
178.813912312176));
#23570=CARTESIAN_POINT('Ctrl Pts',(-60.1835892331231,-108.446751142048,
179.985485138407));
#23571=CARTESIAN_POINT('Ctrl Pts',(-58.5261324831192,-108.529165876334,
179.985485069079));
#23572=CARTESIAN_POINT('Ctrl Pts',(-56.8686757331153,-108.611580610621,
179.985484999752));
#23573=CARTESIAN_POINT('Ctrl Pts',(-55.6937660831736,-108.642552600194,
178.813912075476));
#23574=CARTESIAN_POINT('Ctrl Pts',(-54.5188564332318,-108.673524589768,
177.6423391512));
#23575=CARTESIAN_POINT('Ctrl Pts',(-54.5089184392519,-108.580302817763,
175.985484901707));
#23576=CARTESIAN_POINT('Ctrl Pts',(-54.4989804452721,-108.487081045759,
174.328630652215));
#23577=CARTESIAN_POINT('Ctrl Pts',(-55.6540140668717,-108.269665516481,
173.157057825983));
#23578=CARTESIAN_POINT('Ctrl Pts',(-56.8090476884713,-108.052249987204,
171.985484999752));
#23579=CARTESIAN_POINT('Ctrl Pts',(-58.4466283126412,-107.783391723607,
171.985485069079));
#23580=CARTESIAN_POINT('Ctrl Pts',(-60.084208936811,-107.51453346001,171.985485138407));
#23581=CARTESIAN_POINT('Ctrl Pts',(-61.2392424609188,-107.297117941125,
173.157058062683));
#23582=CARTESIAN_POINT('Ctrl Pts',(-62.3942759850265,-107.079702422241,
174.328630986959));
#23583=CARTESIAN_POINT('Ctrl Pts',(-62.3843378531723,-106.986480664935,
175.985485236451));
#23584=CARTESIAN_POINT('Ctrl Pts',(-62.3743997213182,-106.893258907629,
177.642339485944));
#23585=CARTESIAN_POINT('Ctrl Pts',(-61.1994899738845,-106.924230907596,
178.813912312176));
#23586=CARTESIAN_POINT('Ctrl Pts',(-60.0245802264509,-106.955202907562,
179.985485138407));
#23587=CARTESIAN_POINT('Ctrl Pts',(-58.367123476447,-107.037617641849,179.985485069079));
#23588=CARTESIAN_POINT('Ctrl Pts',(-56.7096667264431,-107.120032376135,
179.985484999752));
#23589=CARTESIAN_POINT('Ctrl Pts',(-55.5347570765013,-107.151004365708,
178.813912075476));
#23590=CARTESIAN_POINT('Ctrl Pts',(-54.3598474265596,-107.181976355282,
177.6423391512));
#23591=CARTESIAN_POINT('Ctrl Pts',(-54.3499094325797,-107.088754583277,
175.985484901707));
#23592=CARTESIAN_POINT('Ctrl Pts',(-54.3399714385998,-106.995532811273,
174.328630652215));
#23593=CARTESIAN_POINT('Ctrl Pts',(-55.4950050601995,-106.778117281995,
173.157057825983));
#23594=CARTESIAN_POINT('Ctrl Pts',(-56.6500386817991,-106.560701752718,
171.985484999752));
#23595=CARTESIAN_POINT('Ctrl Pts',(-58.2876193059689,-106.291843489121,
171.985485069079));
#23596=CARTESIAN_POINT('Ctrl Pts',(-59.9251999301388,-106.022985225524,
171.985485138407));
#23597=CARTESIAN_POINT('Ctrl Pts',(-61.0802334542465,-105.80556970664,173.157058062683));
#23598=CARTESIAN_POINT('Ctrl Pts',(-62.2352669783543,-105.588154187756,
174.328630986959));
#23599=CARTESIAN_POINT('Ctrl Pts',(-62.2253288465001,-105.494932430449,
175.985485236451));
#23600=CARTESIAN_POINT('Ctrl Pts',(-62.2153907146459,-105.401710673143,
177.642339485944));
#23601=CARTESIAN_POINT('Ctrl Pts',(-61.0404809672123,-105.43268267311,178.813912312176));
#23602=CARTESIAN_POINT('Ctrl Pts',(-59.8655712197787,-105.463654673077,
179.985485138407));
#23603=CARTESIAN_POINT('Ctrl Pts',(-58.2081144697748,-105.546069407363,
179.985485069079));
#23604=CARTESIAN_POINT('Ctrl Pts',(-56.5506577197709,-105.628484141649,
179.985484999752));
#23605=CARTESIAN_POINT('Ctrl Pts',(-55.3757480698291,-105.659456131223,
178.813912075476));
#23606=CARTESIAN_POINT('Ctrl Pts',(-54.2008384198873,-105.690428120796,
177.6423391512));
#23607=CARTESIAN_POINT('Ctrl Pts',(-54.1909004259075,-105.597206348792,
175.985484901707));
#23608=CARTESIAN_POINT('Ctrl Pts',(-54.1809624319276,-105.503984576787,
174.328630652215));
#23609=CARTESIAN_POINT('Ctrl Pts',(-55.3359960535272,-105.28656904751,173.157057825983));
#23610=CARTESIAN_POINT('Ctrl Pts',(-56.4910296751268,-105.069153518232,
171.985484999752));
#23611=CARTESIAN_POINT('Ctrl Pts',(-58.1286102992967,-104.800295254635,
171.985485069079));
#23612=CARTESIAN_POINT('Ctrl Pts',(-59.7661909234666,-104.531436991038,
171.985485138407));
#23613=CARTESIAN_POINT('Ctrl Pts',(-60.9212244475743,-104.314021472154,
173.157058062683));
#23614=CARTESIAN_POINT('Ctrl Pts',(-62.0762579716821,-104.09660595327,174.328630986959));
#23615=CARTESIAN_POINT('Ctrl Pts',(-62.0663198398279,-104.003384195964,
175.985485236451));
#23616=CARTESIAN_POINT('Ctrl Pts',(-62.0563817079737,-103.910162438658,
177.642339485944));
#23617=CARTESIAN_POINT('Ctrl Pts',(-60.8814719605401,-103.941134438624,
178.813912312176));
#23618=CARTESIAN_POINT('Ctrl Pts',(-59.7065622131064,-103.972106438591,
179.985485138407));
#23619=CARTESIAN_POINT('Ctrl Pts',(-58.0491054631025,-104.054521172878,
179.985485069079));
#23620=CARTESIAN_POINT('Ctrl Pts',(-56.3916487130987,-104.136935907164,
179.985484999752));
#23621=CARTESIAN_POINT('Ctrl Pts',(-55.2167390631569,-104.167907896737,
178.813912075476));
#23622=CARTESIAN_POINT('Ctrl Pts',(-54.0418294132151,-104.198879886311,
177.6423391512));
#23623=CARTESIAN_POINT('Ctrl Pts',(-54.0318914192353,-104.105658114306,
175.985484901707));
#23624=CARTESIAN_POINT('Ctrl Pts',(-54.0219534252554,-104.012436342302,
174.328630652215));
#23625=CARTESIAN_POINT('Ctrl Pts',(-55.176987046855,-103.795020813024,173.157057825983));
#23626=CARTESIAN_POINT('Ctrl Pts',(-56.3320206684546,-103.577605283747,
171.985484999752));
#23627=CARTESIAN_POINT('Ctrl Pts',(-57.9696012926245,-103.30874702015,171.985485069079));
#23628=CARTESIAN_POINT('Ctrl Pts',(-59.6071819167943,-103.039888756553,
171.985485138407));
#23629=CARTESIAN_POINT('Ctrl Pts',(-60.7622154409021,-102.822473237669,
173.157058062683));
#23630=CARTESIAN_POINT('Ctrl Pts',(-61.9172489650099,-102.605057718784,
174.328630986959));
#23631=CARTESIAN_POINT('Ctrl Pts',(-61.9073108331557,-102.511835961478,
175.985485236451));
#23632=CARTESIAN_POINT('Ctrl Pts',(-61.8973727013015,-102.418614204172,
177.642339485944));
#23633=CARTESIAN_POINT('Ctrl Pts',(-60.7224629538678,-102.449586204139,
178.813912312176));
#23634=CARTESIAN_POINT('Ctrl Pts',(-59.5475532064342,-102.480558204106,
179.985485138407));
#23635=CARTESIAN_POINT('Ctrl Pts',(-57.8900964564303,-102.562972938392,
179.985485069079));
#23636=CARTESIAN_POINT('Ctrl Pts',(-56.2326397064264,-102.645387672678,
179.985484999752));
#23637=CARTESIAN_POINT('Ctrl Pts',(-55.0577300564847,-102.676359662252,
178.813912075476));
#23638=CARTESIAN_POINT('Ctrl Pts',(-53.8828204065429,-102.707331651825,
177.6423391512));
#23639=CARTESIAN_POINT('Ctrl Pts',(-53.872882412563,-102.614109879821,175.985484901707));
#23640=CARTESIAN_POINT('Ctrl Pts',(-53.8629444185832,-102.520888107816,
174.328630652215));
#23641=CARTESIAN_POINT('Ctrl Pts',(-55.0179780401828,-102.303472578539,
173.157057825983));
#23642=CARTESIAN_POINT('Ctrl Pts',(-56.1730116617824,-102.086057049261,
171.985484999752));
#23643=CARTESIAN_POINT('Ctrl Pts',(-57.8105922859523,-101.817198785664,
171.985485069079));
#23644=CARTESIAN_POINT('Ctrl Pts',(-59.4481729101221,-101.548340522067,
171.985485138407));
#23645=CARTESIAN_POINT('Ctrl Pts',(-60.6032064342299,-101.330925003183,
173.157058062683));
#23646=CARTESIAN_POINT('Ctrl Pts',(-61.7582399583376,-101.113509484299,
174.328630986959));
#23647=CARTESIAN_POINT('Ctrl Pts',(-61.7483018264834,-101.020287726993,
175.985485236451));
#23648=CARTESIAN_POINT('Ctrl Pts',(-61.7383636946293,-100.927065969686,
177.642339485944));
#23649=CARTESIAN_POINT('Ctrl Pts',(-60.5634539471956,-100.958037969653,
178.813912312176));
#23650=CARTESIAN_POINT('Ctrl Pts',(-59.388544199762,-100.98900996962,179.985485138407));
#23651=CARTESIAN_POINT('Ctrl Pts',(-57.7310874497581,-101.071424703906,
179.985485069079));
#23652=CARTESIAN_POINT('Ctrl Pts',(-56.0736306997542,-101.153839438193,
179.985484999752));
#23653=CARTESIAN_POINT('Ctrl Pts',(-54.8987210498124,-101.184811427766,
178.813912075476));
#23654=CARTESIAN_POINT('Ctrl Pts',(-53.7238113998707,-101.21578341734,177.6423391512));
#23655=CARTESIAN_POINT('Ctrl Pts',(-53.7138734058908,-101.122561645335,
175.985484901707));
#23656=CARTESIAN_POINT('Ctrl Pts',(-53.7039354119109,-101.029339873331,
174.328630652215));
#23657=CARTESIAN_POINT('Ctrl Pts',(-54.8589690335105,-100.811924344053,
173.157057825983));
#23658=CARTESIAN_POINT('Ctrl Pts',(-56.0140026551102,-100.594508814776,
171.985484999752));
#23659=CARTESIAN_POINT('Ctrl Pts',(-57.65158327928,-100.325650551179,171.985485069079));
#23660=CARTESIAN_POINT('Ctrl Pts',(-59.2891639034499,-100.056792287582,
171.985485138407));
#23661=CARTESIAN_POINT('Ctrl Pts',(-60.4441974275576,-99.8393767686974,
173.157058062683));
#23662=CARTESIAN_POINT('Ctrl Pts',(-61.5992309516654,-99.6219612498133,
174.328630986959));
#23663=CARTESIAN_POINT('Ctrl Pts',(-61.5892928198112,-99.528739492507,175.985485236451));
#23664=CARTESIAN_POINT('Ctrl Pts',(-61.579354687957,-99.4355177352008,177.642339485944));
#23665=CARTESIAN_POINT('Ctrl Pts',(-60.4044449405234,-99.4664897351676,
178.813912312176));
#23666=CARTESIAN_POINT('Ctrl Pts',(-59.2295351930898,-99.4974617351344,
179.985485138407));
#23667=CARTESIAN_POINT('Ctrl Pts',(-57.5720784430859,-99.5798764694207,
179.985485069079));
#23668=CARTESIAN_POINT('Ctrl Pts',(-55.914621693082,-99.662291203707,179.985484999752));
#23669=CARTESIAN_POINT('Ctrl Pts',(-54.7397120431402,-99.6932631932805,
178.813912075476));
#23670=CARTESIAN_POINT('Ctrl Pts',(-53.5648023931984,-99.724235182854,177.6423391512));
#23671=CARTESIAN_POINT('Ctrl Pts',(-53.5548643992186,-99.6310134108495,
175.985484901707));
#23672=CARTESIAN_POINT('Ctrl Pts',(-53.5449264052387,-99.5377916388449,
174.328630652215));
#23673=CARTESIAN_POINT('Ctrl Pts',(-54.6999600268383,-99.3203761095675,
173.157057825983));
#23674=CARTESIAN_POINT('Ctrl Pts',(-55.8549936484379,-99.10296058029,171.985484999752));
#23675=CARTESIAN_POINT('Ctrl Pts',(-57.4925742726078,-98.834102316693,171.985485069079));
#23676=CARTESIAN_POINT('Ctrl Pts',(-59.1301548967777,-98.565244053096,171.985485138407));
#23677=CARTESIAN_POINT('Ctrl Pts',(-60.2851884208854,-98.3478285342118,
173.157058062683));
#23678=CARTESIAN_POINT('Ctrl Pts',(-61.4402219449932,-98.1304130153276,
174.328630986959));
#23679=CARTESIAN_POINT('Ctrl Pts',(-61.430283813139,-98.0371912580215,175.985485236451));
#23680=CARTESIAN_POINT('Ctrl Pts',(-61.4203456812848,-97.9439695007152,
177.642339485944));
#23681=CARTESIAN_POINT('Ctrl Pts',(-60.2454359338512,-97.974941500682,178.813912312176));
#23682=CARTESIAN_POINT('Ctrl Pts',(-59.0705261864175,-98.0059135006488,
179.985485138407));
#23683=CARTESIAN_POINT('Ctrl Pts',(-57.4130694364136,-98.0883282349351,
179.985485069079));
#23684=CARTESIAN_POINT('Ctrl Pts',(-55.7556126864097,-98.1707429692214,
179.985484999752));
#23685=CARTESIAN_POINT('Ctrl Pts',(-54.580703036468,-98.2017149587949,178.813912075476));
#23686=CARTESIAN_POINT('Ctrl Pts',(-61.9716326179341,-111.393034424893,
178.485485069079));
#23687=CARTESIAN_POINT('Ctrl Pts',(-61.8330604135774,-111.39474894277,178.657813499464));
#23688=CARTESIAN_POINT('Ctrl Pts',(-61.6765169939012,-111.398875611052,
178.813912312176));
#23689=CARTESIAN_POINT('Ctrl Pts',(-60.5016072464676,-111.429847611019,
179.985485138407));
#23690=CARTESIAN_POINT('Ctrl Pts',(-58.8441504964637,-111.512262345305,
179.985485069079));
#23691=CARTESIAN_POINT('Ctrl Pts',(-57.1866937464598,-111.594677079592,
179.985484999752));
#23692=CARTESIAN_POINT('Ctrl Pts',(-56.011784096518,-111.625649069165,178.813912075476));
#23693=CARTESIAN_POINT('Ctrl Pts',(-54.8368744465762,-111.656621058739,
177.6423391512));
#23694=CARTESIAN_POINT('Ctrl Pts',(-54.8269364525964,-111.563399286734,
175.985484901707));
#23695=CARTESIAN_POINT('Ctrl Pts',(-54.8169984586165,-111.47017751473,174.328630652215));
#23696=CARTESIAN_POINT('Ctrl Pts',(-55.9720320802161,-111.252761985452,
173.157057825983));
#23697=CARTESIAN_POINT('Ctrl Pts',(-57.1270657018158,-111.035346456175,
171.985484999752));
#23698=CARTESIAN_POINT('Ctrl Pts',(-58.7646463259856,-110.766488192578,
171.985485069079));
#23699=CARTESIAN_POINT('Ctrl Pts',(-60.4022269501555,-110.497629928981,
171.985485138407));
#23700=CARTESIAN_POINT('Ctrl Pts',(-61.5572604742632,-110.280214410097,
173.157058062683));
#23701=CARTESIAN_POINT('Ctrl Pts',(-61.7111554952164,-110.251246276154,
173.313156769748));
#23702=CARTESIAN_POINT('Ctrl Pts',(-61.8469746991872,-110.223708846972,
173.485485069079));
#23703=CARTESIAN_POINT('Ctrl Pts',(-56.2237961054143,-113.614380048479,
178.813912075476));
#23704=CARTESIAN_POINT('Ctrl Pts',(-55.0488864554725,-113.645352038053,
177.6423391512));
#23705=CARTESIAN_POINT('Ctrl Pts',(-55.0389484614927,-113.552130266048,
175.985484901707));
#23706=CARTESIAN_POINT('Ctrl Pts',(-55.0290104675128,-113.458908494044,
174.328630652215));
#23707=CARTESIAN_POINT('Ctrl Pts',(-56.1840440891124,-113.241492964766,
173.157057825983));
#23708=CARTESIAN_POINT('Ctrl Pts',(-57.3390777107121,-113.024077435489,
171.985484999752));
#23709=CARTESIAN_POINT('Ctrl Pts',(-58.9766583348819,-112.755219171892,
171.985485069079));
#23710=CARTESIAN_POINT('Ctrl Pts',(-60.6142389590518,-112.486360908295,
171.985485138407));
#23711=CARTESIAN_POINT('Ctrl Pts',(-61.7692724831595,-112.268945389411,
173.157058062683));
#23712=CARTESIAN_POINT('Ctrl Pts',(-62.9243060072673,-112.051529870527,
174.328630986959));
#23713=CARTESIAN_POINT('Ctrl Pts',(-62.9143678754131,-111.95830811322,175.985485236451));
#23714=CARTESIAN_POINT('Ctrl Pts',(-62.9044297435589,-111.865086355914,
177.642339485944));
#23715=CARTESIAN_POINT('Ctrl Pts',(-61.7295199961253,-111.896058355881,
178.813912312176));
#23716=CARTESIAN_POINT('Ctrl Pts',(-60.5546102486917,-111.927030355848,
179.985485138407));
#23717=CARTESIAN_POINT('Ctrl Pts',(-58.8971534986878,-112.009445090134,
179.985485069079));
#23718=CARTESIAN_POINT('Ctrl Pts',(-57.2396967486839,-112.09185982442,179.985484999752));
#23719=CARTESIAN_POINT('Ctrl Pts',(-56.0647870987421,-112.122831813994,
178.813912075476));
#23720=CARTESIAN_POINT('Ctrl Pts',(-54.8898774488003,-112.153803803567,
177.6423391512));
#23721=CARTESIAN_POINT('Ctrl Pts',(-54.8799394548205,-112.060582031563,
175.985484901707));
#23722=CARTESIAN_POINT('Ctrl Pts',(-54.8700014608406,-111.967360259558,
174.328630652215));
#23723=CARTESIAN_POINT('Ctrl Pts',(-56.0250350824402,-111.749944730281,
173.157057825983));
#23724=CARTESIAN_POINT('Ctrl Pts',(-57.1800687040398,-111.532529201003,
171.985484999752));
#23725=CARTESIAN_POINT('Ctrl Pts',(-58.8176493282097,-111.263670937406,
171.985485069079));
#23726=CARTESIAN_POINT('Ctrl Pts',(-60.4552299523796,-110.994812673809,
171.985485138407));
#23727=CARTESIAN_POINT('Ctrl Pts',(-61.6102634764873,-110.777397154925,
173.157058062683));
#23728=CARTESIAN_POINT('Ctrl Pts',(-62.7652970005951,-110.559981636041,
174.328630986959));
#23729=CARTESIAN_POINT('Ctrl Pts',(-62.7553588687409,-110.466759878735,
175.985485236451));
#23730=CARTESIAN_POINT('Ctrl Pts',(-62.7454207368867,-110.373538121429,
177.642339485944));
#23731=CARTESIAN_POINT('Ctrl Pts',(-61.5705109894531,-110.404510121395,
178.813912312176));
#23732=CARTESIAN_POINT('Ctrl Pts',(-60.3956012420194,-110.435482121362,
179.985485138407));
#23733=CARTESIAN_POINT('Ctrl Pts',(-58.7381444920155,-110.517896855648,
179.985485069079));
#23734=CARTESIAN_POINT('Ctrl Pts',(-57.0806877420116,-110.600311589935,
179.985484999752));
#23735=CARTESIAN_POINT('Ctrl Pts',(-55.9057780920699,-110.631283579508,
178.813912075476));
#23736=CARTESIAN_POINT('Ctrl Pts',(-54.7308684421281,-110.662255569082,
177.6423391512));
#23737=CARTESIAN_POINT('Ctrl Pts',(-54.7209304481482,-110.569033797077,
175.985484901707));
#23738=CARTESIAN_POINT('Ctrl Pts',(-54.7109924541684,-110.475812025073,
174.328630652215));
#23739=CARTESIAN_POINT('Ctrl Pts',(-55.866026075768,-110.258396495795,173.157057825983));
#23740=CARTESIAN_POINT('Ctrl Pts',(-57.0210596973676,-110.040980966518,
171.985484999752));
#23741=CARTESIAN_POINT('Ctrl Pts',(-58.6586403215375,-109.772122702921,
171.985485069079));
#23742=CARTESIAN_POINT('Ctrl Pts',(-60.2962209457073,-109.503264439324,
171.985485138407));
#23743=CARTESIAN_POINT('Ctrl Pts',(-61.4512544698151,-109.28584892044,173.157058062683));
#23744=CARTESIAN_POINT('Ctrl Pts',(-62.6062879939228,-109.068433401555,
174.328630986959));
#23745=CARTESIAN_POINT('Ctrl Pts',(-62.5963498620687,-108.975211644249,
175.985485236451));
#23746=CARTESIAN_POINT('Ctrl Pts',(-62.5864117302145,-108.881989886943,
177.642339485944));
#23747=CARTESIAN_POINT('Ctrl Pts',(-61.4115019827808,-108.91296188691,178.813912312176));
#23748=CARTESIAN_POINT('Ctrl Pts',(-60.2365922353472,-108.943933886877,
179.985485138407));
#23749=CARTESIAN_POINT('Ctrl Pts',(-58.5791354853433,-109.026348621163,
179.985485069079));
#23750=CARTESIAN_POINT('Ctrl Pts',(-56.9216787353394,-109.108763355449,
179.985484999752));
#23751=CARTESIAN_POINT('Ctrl Pts',(-55.7467690853976,-109.139735345023,
178.813912075476));
#23752=CARTESIAN_POINT('Ctrl Pts',(-54.5718594354559,-109.170707334596,
177.6423391512));
#23753=CARTESIAN_POINT('Ctrl Pts',(-54.561921441476,-109.077485562592,175.985484901707));
#23754=CARTESIAN_POINT('Ctrl Pts',(-54.5519834474962,-108.984263790587,
174.328630652215));
#23755=CARTESIAN_POINT('Ctrl Pts',(-55.7070170690958,-108.76684826131,173.157057825983));
#23756=CARTESIAN_POINT('Ctrl Pts',(-56.8620506906954,-108.549432732032,
171.985484999752));
#23757=CARTESIAN_POINT('Ctrl Pts',(-58.4996313148652,-108.280574468435,
171.985485069079));
#23758=CARTESIAN_POINT('Ctrl Pts',(-60.1372119390351,-108.011716204838,
171.985485138407));
#23759=CARTESIAN_POINT('Ctrl Pts',(-61.2922454631428,-107.794300685954,
173.157058062683));
#23760=CARTESIAN_POINT('Ctrl Pts',(-62.4472789872506,-107.57688516707,174.328630986959));
#23761=CARTESIAN_POINT('Ctrl Pts',(-62.4373408553964,-107.483663409764,
175.985485236451));
#23762=CARTESIAN_POINT('Ctrl Pts',(-62.4274027235423,-107.390441652457,
177.642339485944));
#23763=CARTESIAN_POINT('Ctrl Pts',(-61.2524929761086,-107.421413652424,
178.813912312176));
#23764=CARTESIAN_POINT('Ctrl Pts',(-60.077583228675,-107.452385652391,179.985485138407));
#23765=CARTESIAN_POINT('Ctrl Pts',(-58.4201264786711,-107.534800386677,
179.985485069079));
#23766=CARTESIAN_POINT('Ctrl Pts',(-56.7626697286672,-107.617215120964,
179.985484999752));
#23767=CARTESIAN_POINT('Ctrl Pts',(-55.5877600787254,-107.648187110537,
178.813912075476));
#23768=CARTESIAN_POINT('Ctrl Pts',(-54.4128504287836,-107.67915910011,177.6423391512));
#23769=CARTESIAN_POINT('Ctrl Pts',(-54.4029124348038,-107.585937328106,
175.985484901707));
#23770=CARTESIAN_POINT('Ctrl Pts',(-54.3929744408239,-107.492715556102,
174.328630652215));
#23771=CARTESIAN_POINT('Ctrl Pts',(-55.5480080624235,-107.275300026824,
173.157057825983));
#23772=CARTESIAN_POINT('Ctrl Pts',(-56.7030416840231,-107.057884497547,
171.985484999752));
#23773=CARTESIAN_POINT('Ctrl Pts',(-58.340622308193,-106.78902623395,171.985485069079));
#23774=CARTESIAN_POINT('Ctrl Pts',(-59.9782029323629,-106.520167970353,
171.985485138407));
#23775=CARTESIAN_POINT('Ctrl Pts',(-61.1332364564706,-106.302752451468,
173.157058062683));
#23776=CARTESIAN_POINT('Ctrl Pts',(-62.2882699805784,-106.085336932584,
174.328630986959));
#23777=CARTESIAN_POINT('Ctrl Pts',(-62.2783318487242,-105.992115175278,
175.985485236451));
#23778=CARTESIAN_POINT('Ctrl Pts',(-62.26839371687,-105.898893417972,177.642339485944));
#23779=CARTESIAN_POINT('Ctrl Pts',(-61.0934839694364,-105.929865417939,
178.813912312176));
#23780=CARTESIAN_POINT('Ctrl Pts',(-59.9185742220028,-105.960837417905,
179.985485138407));
#23781=CARTESIAN_POINT('Ctrl Pts',(-58.2611174719989,-106.043252152192,
179.985485069079));
#23782=CARTESIAN_POINT('Ctrl Pts',(-56.603660721995,-106.125666886478,179.985484999752));
#23783=CARTESIAN_POINT('Ctrl Pts',(-55.4287510720532,-106.156638876051,
178.813912075476));
#23784=CARTESIAN_POINT('Ctrl Pts',(-54.2538414221114,-106.187610865625,
177.6423391512));
#23785=CARTESIAN_POINT('Ctrl Pts',(-54.2439034281315,-106.09438909362,175.985484901707));
#23786=CARTESIAN_POINT('Ctrl Pts',(-54.2339654341517,-106.001167321616,
174.328630652215));
#23787=CARTESIAN_POINT('Ctrl Pts',(-55.3889990557513,-105.783751792338,
173.157057825983));
#23788=CARTESIAN_POINT('Ctrl Pts',(-56.5440326773509,-105.566336263061,
171.985484999752));
#23789=CARTESIAN_POINT('Ctrl Pts',(-58.1816133015208,-105.297477999464,
171.985485069079));
#23790=CARTESIAN_POINT('Ctrl Pts',(-59.8191939256906,-105.028619735867,
171.985485138407));
#23791=CARTESIAN_POINT('Ctrl Pts',(-60.9742274497984,-104.811204216983,
173.157058062683));
#23792=CARTESIAN_POINT('Ctrl Pts',(-62.1292609739061,-104.593788698099,
174.328630986959));
#23793=CARTESIAN_POINT('Ctrl Pts',(-62.119322842052,-104.500566940792,175.985485236451));
#23794=CARTESIAN_POINT('Ctrl Pts',(-62.1093847101978,-104.407345183486,
177.642339485944));
#23795=CARTESIAN_POINT('Ctrl Pts',(-60.9344749627642,-104.438317183453,
178.813912312176));
#23796=CARTESIAN_POINT('Ctrl Pts',(-59.7595652153305,-104.46928918342,179.985485138407));
#23797=CARTESIAN_POINT('Ctrl Pts',(-58.1021084653266,-104.551703917706,
179.985485069079));
#23798=CARTESIAN_POINT('Ctrl Pts',(-56.4446517153227,-104.634118651992,
179.985484999752));
#23799=CARTESIAN_POINT('Ctrl Pts',(-55.269742065381,-104.665090641566,178.813912075476));
#23800=CARTESIAN_POINT('Ctrl Pts',(-54.0948324154392,-104.696062631139,
177.6423391512));
#23801=CARTESIAN_POINT('Ctrl Pts',(-54.0848944214593,-104.602840859135,
175.985484901707));
#23802=CARTESIAN_POINT('Ctrl Pts',(-54.0749564274795,-104.50961908713,174.328630652215));
#23803=CARTESIAN_POINT('Ctrl Pts',(-55.2299900490791,-104.292203557853,
173.157057825983));
#23804=CARTESIAN_POINT('Ctrl Pts',(-56.3850236706787,-104.074788028575,
171.985484999752));
#23805=CARTESIAN_POINT('Ctrl Pts',(-58.0226042948486,-103.805929764978,
171.985485069079));
#23806=CARTESIAN_POINT('Ctrl Pts',(-59.6601849190184,-103.537071501381,
171.985485138407));
#23807=CARTESIAN_POINT('Ctrl Pts',(-60.8152184431262,-103.319655982497,
173.157058062683));
#23808=CARTESIAN_POINT('Ctrl Pts',(-61.9702519672339,-103.102240463613,
174.328630986959));
#23809=CARTESIAN_POINT('Ctrl Pts',(-61.9603138353797,-103.009018706307,
175.985485236451));
#23810=CARTESIAN_POINT('Ctrl Pts',(-61.9503757035256,-102.915796949001,
177.642339485944));
#23811=CARTESIAN_POINT('Ctrl Pts',(-60.7754659560919,-102.946768948967,
178.813912312176));
#23812=CARTESIAN_POINT('Ctrl Pts',(-59.6005562086583,-102.977740948934,
179.985485138407));
#23813=CARTESIAN_POINT('Ctrl Pts',(-57.9430994586544,-103.06015568322,179.985485069079));
#23814=CARTESIAN_POINT('Ctrl Pts',(-56.2856427086505,-103.142570417507,
179.985484999752));
#23815=CARTESIAN_POINT('Ctrl Pts',(-55.1107330587087,-103.17354240708,178.813912075476));
#23816=CARTESIAN_POINT('Ctrl Pts',(-53.935823408767,-103.204514396654,177.6423391512));
#23817=CARTESIAN_POINT('Ctrl Pts',(-53.9258854147871,-103.111292624649,
175.985484901707));
#23818=CARTESIAN_POINT('Ctrl Pts',(-53.9159474208072,-103.018070852645,
174.328630652215));
#23819=CARTESIAN_POINT('Ctrl Pts',(-55.0709810424069,-102.800655323367,
173.157057825983));
#23820=CARTESIAN_POINT('Ctrl Pts',(-56.2260146640065,-102.58323979409,171.985484999752));
#23821=CARTESIAN_POINT('Ctrl Pts',(-57.8635952881763,-102.314381530493,
171.985485069079));
#23822=CARTESIAN_POINT('Ctrl Pts',(-59.5011759123462,-102.045523266896,
171.985485138407));
#23823=CARTESIAN_POINT('Ctrl Pts',(-60.6562094364539,-101.828107748012,
173.157058062683));
#23824=CARTESIAN_POINT('Ctrl Pts',(-61.8112429605617,-101.610692229127,
174.328630986959));
#23825=CARTESIAN_POINT('Ctrl Pts',(-61.8013048287075,-101.517470471821,
175.985485236451));
#23826=CARTESIAN_POINT('Ctrl Pts',(-61.7913666968533,-101.424248714515,
177.642339485944));
#23827=CARTESIAN_POINT('Ctrl Pts',(-60.6164569494197,-101.455220714482,
178.813912312176));
#23828=CARTESIAN_POINT('Ctrl Pts',(-59.4415472019861,-101.486192714449,
179.985485138407));
#23829=CARTESIAN_POINT('Ctrl Pts',(-57.7840904519822,-101.568607448735,
179.985485069079));
#23830=CARTESIAN_POINT('Ctrl Pts',(-56.1266337019783,-101.651022183021,
179.985484999752));
#23831=CARTESIAN_POINT('Ctrl Pts',(-54.9517240520365,-101.681994172595,
178.813912075476));
#23832=CARTESIAN_POINT('Ctrl Pts',(-53.7768144020947,-101.712966162168,
177.6423391512));
#23833=CARTESIAN_POINT('Ctrl Pts',(-53.7668764081149,-101.619744390164,
175.985484901707));
#23834=CARTESIAN_POINT('Ctrl Pts',(-53.756938414135,-101.526522618159,174.328630652215));
#23835=CARTESIAN_POINT('Ctrl Pts',(-54.9119720357346,-101.309107088882,
173.157057825983));
#23836=CARTESIAN_POINT('Ctrl Pts',(-56.0670056573342,-101.091691559604,
171.985484999752));
#23837=CARTESIAN_POINT('Ctrl Pts',(-57.7045862815041,-100.822833296007,
171.985485069079));
#23838=CARTESIAN_POINT('Ctrl Pts',(-59.342166905674,-100.55397503241,171.985485138407));
#23839=CARTESIAN_POINT('Ctrl Pts',(-60.4972004297817,-100.336559513526,
173.157058062683));
#23840=CARTESIAN_POINT('Ctrl Pts',(-61.6522339538895,-100.119143994642,
174.328630986959));
#23841=CARTESIAN_POINT('Ctrl Pts',(-61.6422958220353,-100.025922237336,
175.985485236451));
#23842=CARTESIAN_POINT('Ctrl Pts',(-61.6323576901811,-99.9327004800294,
177.642339485944));
#23843=CARTESIAN_POINT('Ctrl Pts',(-60.4574479427475,-99.9636724799962,
178.813912312176));
#23844=CARTESIAN_POINT('Ctrl Pts',(-59.2825381953138,-99.994644479963,179.985485138407));
#23845=CARTESIAN_POINT('Ctrl Pts',(-57.6250814453099,-100.077059214249,
179.985485069079));
#23846=CARTESIAN_POINT('Ctrl Pts',(-55.9676246953061,-100.159473948536,
179.985484999752));
#23847=CARTESIAN_POINT('Ctrl Pts',(-54.7927150453643,-100.190445938109,
178.813912075476));
#23848=CARTESIAN_POINT('Ctrl Pts',(-53.6178053954225,-100.221417927683,
177.6423391512));
#23849=CARTESIAN_POINT('Ctrl Pts',(-53.6078674014426,-100.128196155678,
175.985484901707));
#23850=CARTESIAN_POINT('Ctrl Pts',(-53.5979294074628,-100.034974383673,
174.328630652215));
#23851=CARTESIAN_POINT('Ctrl Pts',(-54.7529630290624,-99.817558854396,173.157057825983));
#23852=CARTESIAN_POINT('Ctrl Pts',(-55.907996650662,-99.6001433251185,171.985484999752));
#23853=CARTESIAN_POINT('Ctrl Pts',(-57.5455772748319,-99.3312850615215,
171.985485069079));
#23854=CARTESIAN_POINT('Ctrl Pts',(-59.1831578990017,-99.0624267979246,
171.985485138407));
#23855=CARTESIAN_POINT('Ctrl Pts',(-60.3381914231095,-98.8450112790404,
173.157058062683));
#23856=CARTESIAN_POINT('Ctrl Pts',(-61.4932249472172,-98.6275957601562,
174.328630986959));
#23857=CARTESIAN_POINT('Ctrl Pts',(-61.4832868153631,-98.53437400285,175.985485236451));
#23858=CARTESIAN_POINT('Ctrl Pts',(-61.4733486835089,-98.4411522455438,
177.642339485944));
#23859=CARTESIAN_POINT('Ctrl Pts',(-60.2984389360752,-98.4721242455106,
178.813912312176));
#23860=CARTESIAN_POINT('Ctrl Pts',(-59.1235291886416,-98.5030962454774,
179.985485138407));
#23861=CARTESIAN_POINT('Ctrl Pts',(-57.4660724386377,-98.5855109797636,
179.985485069079));
#23862=CARTESIAN_POINT('Ctrl Pts',(-55.8086156886338,-98.6679257140499,
179.985484999752));
#23863=CARTESIAN_POINT('Ctrl Pts',(-54.633706038692,-98.6988977036234,178.813912075476));
#23864=CARTESIAN_POINT('Ctrl Pts',(-56.9964983346804,-113.864655531781,
178.072094410988));
#23865=CARTESIAN_POINT('Ctrl Pts',(-56.1271283009022,-113.863054956993,
177.207792449865));
#23866=CARTESIAN_POINT('Ctrl Pts',(-56.117190288842,-113.769833186916,175.985484945604));
#23867=CARTESIAN_POINT('Ctrl Pts',(-56.1072522767819,-113.676611416839,
174.763177441344));
#23868=CARTESIAN_POINT('Ctrl Pts',(-56.9567462566485,-113.491768454648,
173.89887555255));
#23869=CARTESIAN_POINT('Ctrl Pts',(-57.8062402365152,-113.306925492458,
173.034573663757));
#23870=CARTESIAN_POINT('Ctrl Pts',(-59.011722573584,-113.084131793069,173.034573714903));
#23871=CARTESIAN_POINT('Ctrl Pts',(-60.2172049106529,-112.86133809368,173.034573766048));
#23872=CARTESIAN_POINT('Ctrl Pts',(-61.0666988185971,-112.676495139156,
173.898875727171));
#23873=CARTESIAN_POINT('Ctrl Pts',(-61.9161927265413,-112.491652184633,
174.763177688294));
#23874=CARTESIAN_POINT('Ctrl Pts',(-61.9062546127674,-112.398430425399,
175.985485192554));
#23875=CARTESIAN_POINT('Ctrl Pts',(-61.8963164989935,-112.305208666166,
177.207792696815));
#23876=CARTESIAN_POINT('Ctrl Pts',(-61.0269463932928,-112.303608099046,
178.072094585608));
#23877=CARTESIAN_POINT('Ctrl Pts',(-60.1575762875921,-112.302007531926,
178.936396474401));
#23878=CARTESIAN_POINT('Ctrl Pts',(-58.9322178246893,-112.338357702004,
178.936396423256));
#23879=CARTESIAN_POINT('Ctrl Pts',(-57.7068593617864,-112.374707872082,
178.936396372111));
#23880=CARTESIAN_POINT('Ctrl Pts',(-56.8374893280082,-112.373107297295,
178.072094410988));
#23881=CARTESIAN_POINT('Ctrl Pts',(-55.9681192942299,-112.371506722508,
177.207792449865));
#23882=CARTESIAN_POINT('Ctrl Pts',(-55.9581812821698,-112.278284952431,
175.985484945604));
#23883=CARTESIAN_POINT('Ctrl Pts',(-55.9482432701096,-112.185063182354,
174.763177441344));
#23884=CARTESIAN_POINT('Ctrl Pts',(-56.7977372499763,-112.000220220163,
173.89887555255));
#23885=CARTESIAN_POINT('Ctrl Pts',(-57.647231229843,-111.815377257972,173.034573663757));
#23886=CARTESIAN_POINT('Ctrl Pts',(-58.8527135669118,-111.592583558583,
173.034573714903));
#23887=CARTESIAN_POINT('Ctrl Pts',(-60.0581959039807,-111.369789859194,
173.034573766048));
#23888=CARTESIAN_POINT('Ctrl Pts',(-60.9076898119249,-111.184946904671,
173.898875727171));
#23889=CARTESIAN_POINT('Ctrl Pts',(-61.7571837198691,-111.000103950148,
174.763177688294));
#23890=CARTESIAN_POINT('Ctrl Pts',(-61.7472456060952,-110.906882190914,
175.985485192554));
#23891=CARTESIAN_POINT('Ctrl Pts',(-61.7373074923213,-110.81366043168,177.207792696815));
#23892=CARTESIAN_POINT('Ctrl Pts',(-60.8679373866206,-110.81205986456,178.072094585608));
#23893=CARTESIAN_POINT('Ctrl Pts',(-59.9985672809199,-110.81045929744,178.936396474401));
#23894=CARTESIAN_POINT('Ctrl Pts',(-58.7732088180171,-110.846809467519,
178.936396423256));
#23895=CARTESIAN_POINT('Ctrl Pts',(-57.5478503551142,-110.883159637597,
178.936396372111));
#23896=CARTESIAN_POINT('Ctrl Pts',(-56.6784803213359,-110.881559062809,
178.072094410988));
#23897=CARTESIAN_POINT('Ctrl Pts',(-55.8091102875577,-110.879958488022,
177.207792449865));
#23898=CARTESIAN_POINT('Ctrl Pts',(-55.7991722754976,-110.786736717945,
175.985484945604));
#23899=CARTESIAN_POINT('Ctrl Pts',(-55.7892342634374,-110.693514947868,
174.763177441344));
#23900=CARTESIAN_POINT('Ctrl Pts',(-56.6387282433041,-110.508671985677,
173.89887555255));
#23901=CARTESIAN_POINT('Ctrl Pts',(-57.4882222231708,-110.323829023487,
173.034573663757));
#23902=CARTESIAN_POINT('Ctrl Pts',(-58.6937045602396,-110.101035324098,
173.034573714903));
#23903=CARTESIAN_POINT('Ctrl Pts',(-59.8991868973084,-109.878241624709,
173.034573766048));
#23904=CARTESIAN_POINT('Ctrl Pts',(-60.7486808052526,-109.693398670185,
173.898875727171));
#23905=CARTESIAN_POINT('Ctrl Pts',(-61.5981747131968,-109.508555715662,
174.763177688294));
#23906=CARTESIAN_POINT('Ctrl Pts',(-61.588236599423,-109.415333956428,175.985485192554));
#23907=CARTESIAN_POINT('Ctrl Pts',(-61.5782984856491,-109.322112197195,
177.207792696815));
#23908=CARTESIAN_POINT('Ctrl Pts',(-60.7089283799484,-109.320511630075,
178.072094585608));
#23909=CARTESIAN_POINT('Ctrl Pts',(-59.8395582742477,-109.318911062955,
178.936396474401));
#23910=CARTESIAN_POINT('Ctrl Pts',(-58.6141998113448,-109.355261233033,
178.936396423256));
#23911=CARTESIAN_POINT('Ctrl Pts',(-57.388841348442,-109.391611403111,178.936396372111));
#23912=CARTESIAN_POINT('Ctrl Pts',(-56.5194713146637,-109.390010828324,
178.072094410988));
#23913=CARTESIAN_POINT('Ctrl Pts',(-55.6501012808855,-109.388410253536,
177.207792449865));
#23914=CARTESIAN_POINT('Ctrl Pts',(-55.6401632688253,-109.295188483459,
175.985484945604));
#23915=CARTESIAN_POINT('Ctrl Pts',(-55.6302252567652,-109.201966713382,
174.763177441344));
#23916=CARTESIAN_POINT('Ctrl Pts',(-56.4797192366319,-109.017123751192,
173.89887555255));
#23917=CARTESIAN_POINT('Ctrl Pts',(-57.3292132164985,-108.832280789001,
173.034573663757));
#23918=CARTESIAN_POINT('Ctrl Pts',(-58.5346955535674,-108.609487089612,
173.034573714903));
#23919=CARTESIAN_POINT('Ctrl Pts',(-59.7401778906362,-108.386693390223,
173.034573766048));
#23920=CARTESIAN_POINT('Ctrl Pts',(-60.5896717985804,-108.2018504357,173.898875727171));
#23921=CARTESIAN_POINT('Ctrl Pts',(-61.4391657065246,-108.017007481176,
174.763177688294));
#23922=CARTESIAN_POINT('Ctrl Pts',(-61.4292275927507,-107.923785721943,
175.985485192554));
#23923=CARTESIAN_POINT('Ctrl Pts',(-61.4192894789769,-107.830563962709,
177.207792696815));
#23924=CARTESIAN_POINT('Ctrl Pts',(-60.5499193732762,-107.828963395589,
178.072094585608));
#23925=CARTESIAN_POINT('Ctrl Pts',(-59.6805492675755,-107.827362828469,
178.936396474401));
#23926=CARTESIAN_POINT('Ctrl Pts',(-58.4551908046726,-107.863712998547,
178.936396423256));
#23927=CARTESIAN_POINT('Ctrl Pts',(-57.2298323417698,-107.900063168626,
178.936396372111));
#23928=CARTESIAN_POINT('Ctrl Pts',(-56.3604623079915,-107.898462593838,
178.072094410988));
#23929=CARTESIAN_POINT('Ctrl Pts',(-55.4910922742133,-107.896862019051,
177.207792449865));
#23930=CARTESIAN_POINT('Ctrl Pts',(-55.4811542621531,-107.803640248974,
175.985484945604));
#23931=CARTESIAN_POINT('Ctrl Pts',(-55.471216250093,-107.710418478897,174.763177441344));
#23932=CARTESIAN_POINT('Ctrl Pts',(-56.3207102299596,-107.525575516706,
173.89887555255));
#23933=CARTESIAN_POINT('Ctrl Pts',(-57.1702042098263,-107.340732554515,
173.034573663757));
#23934=CARTESIAN_POINT('Ctrl Pts',(-58.3756865468951,-107.117938855126,
173.034573714903));
#23935=CARTESIAN_POINT('Ctrl Pts',(-59.581168883964,-106.895145155737,173.034573766048));
#23936=CARTESIAN_POINT('Ctrl Pts',(-60.4306627919082,-106.710302201214,
173.898875727171));
#23937=CARTESIAN_POINT('Ctrl Pts',(-61.2801566998524,-106.525459246691,
174.763177688294));
#23938=CARTESIAN_POINT('Ctrl Pts',(-61.2702185860785,-106.432237487457,
175.985485192554));
#23939=CARTESIAN_POINT('Ctrl Pts',(-61.2602804723046,-106.339015728223,
177.207792696815));
#23940=CARTESIAN_POINT('Ctrl Pts',(-60.3909103666039,-106.337415161103,
178.072094585608));
#23941=CARTESIAN_POINT('Ctrl Pts',(-59.5215402609032,-106.335814593983,
178.936396474401));
#23942=CARTESIAN_POINT('Ctrl Pts',(-58.2961817980004,-106.372164764062,
178.936396423256));
#23943=CARTESIAN_POINT('Ctrl Pts',(-57.0708233350975,-106.40851493414,178.936396372111));
#23944=CARTESIAN_POINT('Ctrl Pts',(-56.2014533013193,-106.406914359353,
178.072094410988));
#23945=CARTESIAN_POINT('Ctrl Pts',(-55.332083267541,-106.405313784565,177.207792449865));
#23946=CARTESIAN_POINT('Ctrl Pts',(-55.3221452554809,-106.312092014488,
175.985484945604));
#23947=CARTESIAN_POINT('Ctrl Pts',(-55.3122072434207,-106.218870244411,
174.763177441344));
#23948=CARTESIAN_POINT('Ctrl Pts',(-56.1617012232874,-106.034027282221,
173.89887555255));
#23949=CARTESIAN_POINT('Ctrl Pts',(-57.0111952031541,-105.84918432003,173.034573663757));
#23950=CARTESIAN_POINT('Ctrl Pts',(-58.2166775402229,-105.626390620641,
173.034573714903));
#23951=CARTESIAN_POINT('Ctrl Pts',(-59.4221598772917,-105.403596921252,
173.034573766048));
#23952=CARTESIAN_POINT('Ctrl Pts',(-60.2716537852359,-105.218753966728,
173.898875727171));
#23953=CARTESIAN_POINT('Ctrl Pts',(-61.1211476931802,-105.033911012205,
174.763177688294));
#23954=CARTESIAN_POINT('Ctrl Pts',(-61.1112095794063,-104.940689252971,
175.985485192554));
#23955=CARTESIAN_POINT('Ctrl Pts',(-61.1012714656324,-104.847467493738,
177.207792696815));
#23956=CARTESIAN_POINT('Ctrl Pts',(-60.2319013599317,-104.845866926618,
178.072094585608));
#23957=CARTESIAN_POINT('Ctrl Pts',(-59.362531254231,-104.844266359498,178.936396474401));
#23958=CARTESIAN_POINT('Ctrl Pts',(-58.1371727913281,-104.880616529576,
178.936396423256));
#23959=CARTESIAN_POINT('Ctrl Pts',(-56.9118143284253,-104.916966699654,
178.936396372111));
#23960=CARTESIAN_POINT('Ctrl Pts',(-56.042444294647,-104.915366124867,178.072094410988));
#23961=CARTESIAN_POINT('Ctrl Pts',(-55.1730742608688,-104.91376555008,177.207792449865));
#23962=CARTESIAN_POINT('Ctrl Pts',(-55.1631362488087,-104.820543780003,
175.985484945604));
#23963=CARTESIAN_POINT('Ctrl Pts',(-55.1531982367485,-104.727322009926,
174.763177441344));
#23964=CARTESIAN_POINT('Ctrl Pts',(-56.0026922166152,-104.542479047735,
173.89887555255));
#23965=CARTESIAN_POINT('Ctrl Pts',(-56.8521861964818,-104.357636085544,
173.034573663757));
#23966=CARTESIAN_POINT('Ctrl Pts',(-58.0576685335507,-104.134842386155,
173.034573714903));
#23967=CARTESIAN_POINT('Ctrl Pts',(-59.2631508706195,-103.912048686766,
173.034573766048));
#23968=CARTESIAN_POINT('Ctrl Pts',(-60.1126447785637,-103.727205732243,
173.898875727171));
#23969=CARTESIAN_POINT('Ctrl Pts',(-60.9621386865079,-103.54236277772,174.763177688294));
#23970=CARTESIAN_POINT('Ctrl Pts',(-60.952200572734,-103.449141018486,175.985485192554));
#23971=CARTESIAN_POINT('Ctrl Pts',(-60.9422624589602,-103.355919259252,
177.207792696815));
#23972=CARTESIAN_POINT('Ctrl Pts',(-60.0728923532595,-103.354318692132,
178.072094585608));
#23973=CARTESIAN_POINT('Ctrl Pts',(-59.2035222475588,-103.352718125012,
178.936396474401));
#23974=CARTESIAN_POINT('Ctrl Pts',(-57.9781637846559,-103.389068295091,
178.936396423256));
#23975=CARTESIAN_POINT('Ctrl Pts',(-56.7528053217531,-103.425418465169,
178.936396372111));
#23976=CARTESIAN_POINT('Ctrl Pts',(-55.8834352879748,-103.423817890381,
178.072094410988));
#23977=CARTESIAN_POINT('Ctrl Pts',(-55.0140652541966,-103.422217315594,
177.207792449865));
#23978=CARTESIAN_POINT('Ctrl Pts',(-55.0041272421364,-103.328995545517,
175.985484945604));
#23979=CARTESIAN_POINT('Ctrl Pts',(-54.9941892300763,-103.23577377544,174.763177441344));
#23980=CARTESIAN_POINT('Ctrl Pts',(-55.8436832099429,-103.050930813249,
173.89887555255));
#23981=CARTESIAN_POINT('Ctrl Pts',(-56.6931771898096,-102.866087851059,
173.034573663757));
#23982=CARTESIAN_POINT('Ctrl Pts',(-57.8986595268784,-102.64329415167,173.034573714903));
#23983=CARTESIAN_POINT('Ctrl Pts',(-59.1041418639473,-102.420500452281,
173.034573766048));
#23984=CARTESIAN_POINT('Ctrl Pts',(-59.9536357718915,-102.235657497757,
173.898875727171));
#23985=CARTESIAN_POINT('Ctrl Pts',(-60.8031296798357,-102.050814543234,
174.763177688294));
#23986=CARTESIAN_POINT('Ctrl Pts',(-60.7931915660618,-101.957592784,175.985485192554));
#23987=CARTESIAN_POINT('Ctrl Pts',(-60.783253452288,-101.864371024767,177.207792696815));
#23988=CARTESIAN_POINT('Ctrl Pts',(-59.9138833465873,-101.862770457647,
178.072094585608));
#23989=CARTESIAN_POINT('Ctrl Pts',(-59.0445132408866,-101.861169890527,
178.936396474401));
#23990=CARTESIAN_POINT('Ctrl Pts',(-57.8191547779837,-101.897520060605,
178.936396423256));
#23991=CARTESIAN_POINT('Ctrl Pts',(-56.5937963150808,-101.933870230683,
178.936396372111));
#23992=CARTESIAN_POINT('Ctrl Pts',(-55.7244262813026,-101.932269655896,
178.072094410988));
#23993=CARTESIAN_POINT('Ctrl Pts',(-54.8550562475244,-101.930669081108,
177.207792449865));
#23994=CARTESIAN_POINT('Ctrl Pts',(-54.8451182354642,-101.837447311031,
175.985484945604));
#23995=CARTESIAN_POINT('Ctrl Pts',(-54.8351802234041,-101.744225540954,
174.763177441344));
#23996=CARTESIAN_POINT('Ctrl Pts',(-55.6846742032707,-101.559382578764,
173.89887555255));
#23997=CARTESIAN_POINT('Ctrl Pts',(-56.5341681831374,-101.374539616573,
173.034573663757));
#23998=CARTESIAN_POINT('Ctrl Pts',(-57.7396505202062,-101.151745917184,
173.034573714903));
#23999=CARTESIAN_POINT('Ctrl Pts',(-58.9451328572751,-100.928952217795,
173.034573766048));
#24000=CARTESIAN_POINT('Ctrl Pts',(-59.7946267652193,-100.744109263272,
173.898875727171));
#24001=CARTESIAN_POINT('Ctrl Pts',(-60.6441206731635,-100.559266308748,
174.763177688294));
#24002=CARTESIAN_POINT('Ctrl Pts',(-60.6341825593896,-100.466044549515,
175.985485192554));
#24003=CARTESIAN_POINT('Ctrl Pts',(-60.6242444456157,-100.372822790281,
177.207792696815));
#24004=CARTESIAN_POINT('Ctrl Pts',(-59.754874339915,-100.371222223161,178.072094585608));
#24005=CARTESIAN_POINT('Ctrl Pts',(-58.8855042342143,-100.369621656041,
178.936396474401));
#24006=CARTESIAN_POINT('Ctrl Pts',(-57.6601457713115,-100.405971826119,
178.936396423256));
#24007=CARTESIAN_POINT('Ctrl Pts',(-56.4347873084086,-100.442321996198,
178.936396372111));
#24008=CARTESIAN_POINT('Ctrl Pts',(-55.5654172746304,-100.44072142141,178.072094410988));
#24009=CARTESIAN_POINT('Ctrl Pts',(-54.6960472408521,-100.439120846623,
177.207792449865));
#24010=CARTESIAN_POINT('Ctrl Pts',(-54.686109228792,-100.345899076546,175.985484945604));
#24011=CARTESIAN_POINT('Ctrl Pts',(-54.6761712167318,-100.252677306469,
174.763177441344));
#24012=CARTESIAN_POINT('Ctrl Pts',(-55.5256651965985,-100.067834344278,
173.89887555255));
#24013=CARTESIAN_POINT('Ctrl Pts',(-56.3751591764652,-99.8829913820874,
173.034573663757));
#24014=CARTESIAN_POINT('Ctrl Pts',(-57.580641513534,-99.6601976826983,173.034573714903));
#24015=CARTESIAN_POINT('Ctrl Pts',(-58.7861238506028,-99.4374039833093,
173.034573766048));
#24016=CARTESIAN_POINT('Ctrl Pts',(-59.635617758547,-99.252561028786,173.898875727171));
#24017=CARTESIAN_POINT('Ctrl Pts',(-60.4851116664912,-99.0677180742627,
174.763177688294));
#24018=CARTESIAN_POINT('Ctrl Pts',(-60.4751735527174,-98.9744963150291,
175.985485192554));
#24019=CARTESIAN_POINT('Ctrl Pts',(-60.4652354389435,-98.8812745557954,
177.207792696815));
#24020=CARTESIAN_POINT('Ctrl Pts',(-59.5958653332428,-98.8796739886754,
178.072094585608));
#24021=CARTESIAN_POINT('Ctrl Pts',(-58.7264952275421,-98.8780734215554,
178.936396474401));
#24022=CARTESIAN_POINT('Ctrl Pts',(-57.5011367646392,-98.9144235916337,
178.936396423256));
#24023=CARTESIAN_POINT('Ctrl Pts',(-56.2757783017364,-98.9507737617121,
178.936396372111));
#24024=CARTESIAN_POINT('Ctrl Pts',(-55.4064082679581,-98.9491731869247,
178.072094410988));
#24025=CARTESIAN_POINT('Ctrl Pts',(-60.8888270454861,-111.922827698674,
179.455551290205));
#24026=CARTESIAN_POINT('Ctrl Pts',(-59.9629308875334,-111.956450790096,
179.985485113659));
#24027=CARTESIAN_POINT('Ctrl Pts',(-58.8971534986878,-112.009445090134,
179.985485069079));
#24028=CARTESIAN_POINT('Ctrl Pts',(-57.2396967486839,-112.09185982442,179.985484999752));
#24029=CARTESIAN_POINT('Ctrl Pts',(-56.0647870987421,-112.122831813994,
178.813912075476));
#24030=CARTESIAN_POINT('Ctrl Pts',(-54.8898774488003,-112.153803803567,
177.6423391512));
#24031=CARTESIAN_POINT('Ctrl Pts',(-54.8799394548205,-112.060582031563,
175.985484901707));
#24032=CARTESIAN_POINT('Ctrl Pts',(-54.8700014608406,-111.967360259558,
174.328630652215));
#24033=CARTESIAN_POINT('Ctrl Pts',(-56.0250350824402,-111.749944730281,
173.157057825983));
#24034=CARTESIAN_POINT('Ctrl Pts',(-57.1800687040398,-111.532529201003,
171.985484999752));
#24035=CARTESIAN_POINT('Ctrl Pts',(-58.8176493282097,-111.263670937406,
171.985485069079));
#24036=CARTESIAN_POINT('Ctrl Pts',(-60.4552299523796,-110.994812673809,
171.985485138407));
#24037=CARTESIAN_POINT('Ctrl Pts',(-61.6102634764873,-110.777397154925,
173.157058062683));
#24038=CARTESIAN_POINT('Ctrl Pts',(-61.7641584974405,-110.748429020983,
173.313156769748));
#24039=CARTESIAN_POINT('Ctrl Pts',(-61.8999777014113,-110.7208915918,173.485485069079));
#24040=CARTESIAN_POINT('Ctrl Pts',(-56.1707931031902,-113.117197303651,
178.813912075476));
#24041=CARTESIAN_POINT('Ctrl Pts',(-54.9958834532485,-113.148169293224,
177.6423391512));
#24042=CARTESIAN_POINT('Ctrl Pts',(-54.9859454592686,-113.05494752122,175.985484901707));
#24043=CARTESIAN_POINT('Ctrl Pts',(-54.9760074652888,-112.961725749215,
174.328630652215));
#24044=CARTESIAN_POINT('Ctrl Pts',(-56.1310410868884,-112.744310219938,
173.157057825983));
#24045=CARTESIAN_POINT('Ctrl Pts',(-57.286074708488,-112.52689469066,171.985484999752));
#24046=CARTESIAN_POINT('Ctrl Pts',(-58.9236553326578,-112.258036427063,
171.985485069079));
#24047=CARTESIAN_POINT('Ctrl Pts',(-60.5612359568277,-111.989178163466,
171.985485138407));
#24048=CARTESIAN_POINT('Ctrl Pts',(-61.7162694809355,-111.771762644582,
173.157058062683));
#24049=CARTESIAN_POINT('Ctrl Pts',(-62.8713030050432,-111.554347125698,
174.328630986959));
#24050=CARTESIAN_POINT('Ctrl Pts',(-62.861364873189,-111.461125368392,175.985485236451));
#24051=CARTESIAN_POINT('Ctrl Pts',(-62.8514267413349,-111.367903611086,
177.642339485944));
#24052=CARTESIAN_POINT('Ctrl Pts',(-61.6765169939012,-111.398875611052,
178.813912312176));
#24053=CARTESIAN_POINT('Ctrl Pts',(-60.5016072464676,-111.429847611019,
179.985485138407));
#24054=CARTESIAN_POINT('Ctrl Pts',(-58.8441504964637,-111.512262345305,
179.985485069079));
#24055=CARTESIAN_POINT('Ctrl Pts',(-57.1866937464598,-111.594677079592,
179.985484999752));
#24056=CARTESIAN_POINT('Ctrl Pts',(-56.011784096518,-111.625649069165,178.813912075476));
#24057=CARTESIAN_POINT('Ctrl Pts',(-54.8368744465763,-111.656621058739,
177.6423391512));
#24058=CARTESIAN_POINT('Ctrl Pts',(-54.8269364525964,-111.563399286734,
175.985484901707));
#24059=CARTESIAN_POINT('Ctrl Pts',(-54.8169984586165,-111.47017751473,174.328630652215));
#24060=CARTESIAN_POINT('Ctrl Pts',(-55.9720320802161,-111.252761985452,
173.157057825983));
#24061=CARTESIAN_POINT('Ctrl Pts',(-57.1270657018158,-111.035346456175,
171.985484999752));
#24062=CARTESIAN_POINT('Ctrl Pts',(-58.7646463259856,-110.766488192578,
171.985485069079));
#24063=CARTESIAN_POINT('Ctrl Pts',(-60.4022269501555,-110.497629928981,
171.985485138407));
#24064=CARTESIAN_POINT('Ctrl Pts',(-61.5572604742632,-110.280214410097,
173.157058062683));
#24065=CARTESIAN_POINT('Ctrl Pts',(-62.712293998371,-110.062798891212,174.328630986959));
#24066=CARTESIAN_POINT('Ctrl Pts',(-62.7023558665168,-109.969577133906,
175.985485236451));
#24067=CARTESIAN_POINT('Ctrl Pts',(-62.6924177346626,-109.8763553766,177.642339485944));
#24068=CARTESIAN_POINT('Ctrl Pts',(-61.517507987229,-109.907327376567,178.813912312176));
#24069=CARTESIAN_POINT('Ctrl Pts',(-60.3425982397954,-109.938299376534,
179.985485138407));
#24070=CARTESIAN_POINT('Ctrl Pts',(-58.6851414897915,-110.02071411082,179.985485069079));
#24071=CARTESIAN_POINT('Ctrl Pts',(-57.0276847397876,-110.103128845106,
179.985484999752));
#24072=CARTESIAN_POINT('Ctrl Pts',(-55.8527750898458,-110.13410083468,178.813912075476));
#24073=CARTESIAN_POINT('Ctrl Pts',(-54.677865439904,-110.165072824253,177.6423391512));
#24074=CARTESIAN_POINT('Ctrl Pts',(-54.6679274459242,-110.071851052249,
175.985484901707));
#24075=CARTESIAN_POINT('Ctrl Pts',(-54.6579894519443,-109.978629280244,
174.328630652215));
#24076=CARTESIAN_POINT('Ctrl Pts',(-55.8130230735439,-109.761213750967,
173.157057825983));
#24077=CARTESIAN_POINT('Ctrl Pts',(-56.9680566951435,-109.543798221689,
171.985484999752));
#24078=CARTESIAN_POINT('Ctrl Pts',(-58.6056373193134,-109.274939958092,
171.985485069079));
#24079=CARTESIAN_POINT('Ctrl Pts',(-60.2432179434833,-109.006081694495,
171.985485138407));
#24080=CARTESIAN_POINT('Ctrl Pts',(-61.398251467591,-108.788666175611,173.157058062683));
#24081=CARTESIAN_POINT('Ctrl Pts',(-62.5532849916988,-108.571250656727,
174.328630986959));
#24082=CARTESIAN_POINT('Ctrl Pts',(-62.5433468598446,-108.478028899421,
175.985485236451));
#24083=CARTESIAN_POINT('Ctrl Pts',(-62.5334087279904,-108.384807142114,
177.642339485944));
#24084=CARTESIAN_POINT('Ctrl Pts',(-61.3584989805568,-108.415779142081,
178.813912312176));
#24085=CARTESIAN_POINT('Ctrl Pts',(-60.1835892331231,-108.446751142048,
179.985485138407));
#24086=CARTESIAN_POINT('Ctrl Pts',(-58.5261324831192,-108.529165876334,
179.985485069079));
#24087=CARTESIAN_POINT('Ctrl Pts',(-56.8686757331153,-108.611580610621,
179.985484999752));
#24088=CARTESIAN_POINT('Ctrl Pts',(-55.6937660831736,-108.642552600194,
178.813912075476));
#24089=CARTESIAN_POINT('Ctrl Pts',(-54.5188564332318,-108.673524589768,
177.6423391512));
#24090=CARTESIAN_POINT('Ctrl Pts',(-54.5089184392519,-108.580302817763,
175.985484901707));
#24091=CARTESIAN_POINT('Ctrl Pts',(-54.4989804452721,-108.487081045759,
174.328630652215));
#24092=CARTESIAN_POINT('Ctrl Pts',(-55.6540140668717,-108.269665516481,
173.157057825983));
#24093=CARTESIAN_POINT('Ctrl Pts',(-56.8090476884713,-108.052249987204,
171.985484999752));
#24094=CARTESIAN_POINT('Ctrl Pts',(-58.4466283126412,-107.783391723607,
171.985485069079));
#24095=CARTESIAN_POINT('Ctrl Pts',(-60.084208936811,-107.51453346001,171.985485138407));
#24096=CARTESIAN_POINT('Ctrl Pts',(-61.2392424609188,-107.297117941125,
173.157058062683));
#24097=CARTESIAN_POINT('Ctrl Pts',(-62.3942759850265,-107.079702422241,
174.328630986959));
#24098=CARTESIAN_POINT('Ctrl Pts',(-62.3843378531723,-106.986480664935,
175.985485236451));
#24099=CARTESIAN_POINT('Ctrl Pts',(-62.3743997213182,-106.893258907629,
177.642339485944));
#24100=CARTESIAN_POINT('Ctrl Pts',(-61.1994899738845,-106.924230907596,
178.813912312176));
#24101=CARTESIAN_POINT('Ctrl Pts',(-60.0245802264509,-106.955202907562,
179.985485138407));
#24102=CARTESIAN_POINT('Ctrl Pts',(-58.367123476447,-107.037617641849,179.985485069079));
#24103=CARTESIAN_POINT('Ctrl Pts',(-56.7096667264431,-107.120032376135,
179.985484999752));
#24104=CARTESIAN_POINT('Ctrl Pts',(-55.5347570765013,-107.151004365708,
178.813912075476));
#24105=CARTESIAN_POINT('Ctrl Pts',(-54.3598474265596,-107.181976355282,
177.6423391512));
#24106=CARTESIAN_POINT('Ctrl Pts',(-54.3499094325797,-107.088754583277,
175.985484901707));
#24107=CARTESIAN_POINT('Ctrl Pts',(-54.3399714385998,-106.995532811273,
174.328630652215));
#24108=CARTESIAN_POINT('Ctrl Pts',(-55.4950050601995,-106.778117281995,
173.157057825983));
#24109=CARTESIAN_POINT('Ctrl Pts',(-56.6500386817991,-106.560701752718,
171.985484999752));
#24110=CARTESIAN_POINT('Ctrl Pts',(-58.2876193059689,-106.291843489121,
171.985485069079));
#24111=CARTESIAN_POINT('Ctrl Pts',(-59.9251999301388,-106.022985225524,
171.985485138407));
#24112=CARTESIAN_POINT('Ctrl Pts',(-61.0802334542465,-105.80556970664,173.157058062683));
#24113=CARTESIAN_POINT('Ctrl Pts',(-62.2352669783543,-105.588154187756,
174.328630986959));
#24114=CARTESIAN_POINT('Ctrl Pts',(-62.2253288465001,-105.494932430449,
175.985485236451));
#24115=CARTESIAN_POINT('Ctrl Pts',(-62.2153907146459,-105.401710673143,
177.642339485944));
#24116=CARTESIAN_POINT('Ctrl Pts',(-61.0404809672123,-105.43268267311,178.813912312176));
#24117=CARTESIAN_POINT('Ctrl Pts',(-59.8655712197787,-105.463654673077,
179.985485138407));
#24118=CARTESIAN_POINT('Ctrl Pts',(-58.2081144697748,-105.546069407363,
179.985485069079));
#24119=CARTESIAN_POINT('Ctrl Pts',(-56.5506577197709,-105.628484141649,
179.985484999752));
#24120=CARTESIAN_POINT('Ctrl Pts',(-55.3757480698291,-105.659456131223,
178.813912075476));
#24121=CARTESIAN_POINT('Ctrl Pts',(-54.2008384198873,-105.690428120796,
177.6423391512));
#24122=CARTESIAN_POINT('Ctrl Pts',(-54.1909004259075,-105.597206348792,
175.985484901707));
#24123=CARTESIAN_POINT('Ctrl Pts',(-54.1809624319276,-105.503984576787,
174.328630652215));
#24124=CARTESIAN_POINT('Ctrl Pts',(-55.3359960535272,-105.28656904751,173.157057825983));
#24125=CARTESIAN_POINT('Ctrl Pts',(-56.4910296751268,-105.069153518232,
171.985484999752));
#24126=CARTESIAN_POINT('Ctrl Pts',(-58.1286102992967,-104.800295254635,
171.985485069079));
#24127=CARTESIAN_POINT('Ctrl Pts',(-59.7661909234666,-104.531436991038,
171.985485138407));
#24128=CARTESIAN_POINT('Ctrl Pts',(-60.9212244475743,-104.314021472154,
173.157058062683));
#24129=CARTESIAN_POINT('Ctrl Pts',(-62.0762579716821,-104.09660595327,174.328630986959));
#24130=CARTESIAN_POINT('Ctrl Pts',(-62.0663198398279,-104.003384195964,
175.985485236451));
#24131=CARTESIAN_POINT('Ctrl Pts',(-62.0563817079737,-103.910162438658,
177.642339485944));
#24132=CARTESIAN_POINT('Ctrl Pts',(-60.8814719605401,-103.941134438624,
178.813912312176));
#24133=CARTESIAN_POINT('Ctrl Pts',(-59.7065622131064,-103.972106438591,
179.985485138407));
#24134=CARTESIAN_POINT('Ctrl Pts',(-58.0491054631025,-104.054521172878,
179.985485069079));
#24135=CARTESIAN_POINT('Ctrl Pts',(-56.3916487130987,-104.136935907164,
179.985484999752));
#24136=CARTESIAN_POINT('Ctrl Pts',(-55.2167390631569,-104.167907896737,
178.813912075476));
#24137=CARTESIAN_POINT('Ctrl Pts',(-54.0418294132151,-104.198879886311,
177.6423391512));
#24138=CARTESIAN_POINT('Ctrl Pts',(-54.0318914192353,-104.105658114306,
175.985484901707));
#24139=CARTESIAN_POINT('Ctrl Pts',(-54.0219534252554,-104.012436342302,
174.328630652215));
#24140=CARTESIAN_POINT('Ctrl Pts',(-55.176987046855,-103.795020813024,173.157057825983));
#24141=CARTESIAN_POINT('Ctrl Pts',(-56.3320206684546,-103.577605283747,
171.985484999752));
#24142=CARTESIAN_POINT('Ctrl Pts',(-57.9696012926245,-103.30874702015,171.985485069079));
#24143=CARTESIAN_POINT('Ctrl Pts',(-59.6071819167943,-103.039888756553,
171.985485138407));
#24144=CARTESIAN_POINT('Ctrl Pts',(-60.7622154409021,-102.822473237669,
173.157058062683));
#24145=CARTESIAN_POINT('Ctrl Pts',(-61.9172489650099,-102.605057718784,
174.328630986959));
#24146=CARTESIAN_POINT('Ctrl Pts',(-61.9073108331557,-102.511835961478,
175.985485236451));
#24147=CARTESIAN_POINT('Ctrl Pts',(-61.8973727013015,-102.418614204172,
177.642339485944));
#24148=CARTESIAN_POINT('Ctrl Pts',(-60.7224629538678,-102.449586204139,
178.813912312176));
#24149=CARTESIAN_POINT('Ctrl Pts',(-59.5475532064342,-102.480558204106,
179.985485138407));
#24150=CARTESIAN_POINT('Ctrl Pts',(-57.8900964564303,-102.562972938392,
179.985485069079));
#24151=CARTESIAN_POINT('Ctrl Pts',(-56.2326397064264,-102.645387672678,
179.985484999752));
#24152=CARTESIAN_POINT('Ctrl Pts',(-55.0577300564847,-102.676359662252,
178.813912075476));
#24153=CARTESIAN_POINT('Ctrl Pts',(-53.8828204065429,-102.707331651825,
177.6423391512));
#24154=CARTESIAN_POINT('Ctrl Pts',(-53.872882412563,-102.614109879821,175.985484901707));
#24155=CARTESIAN_POINT('Ctrl Pts',(-53.8629444185832,-102.520888107816,
174.328630652215));
#24156=CARTESIAN_POINT('Ctrl Pts',(-55.0179780401828,-102.303472578539,
173.157057825983));
#24157=CARTESIAN_POINT('Ctrl Pts',(-56.1730116617824,-102.086057049261,
171.985484999752));
#24158=CARTESIAN_POINT('Ctrl Pts',(-57.8105922859523,-101.817198785664,
171.985485069079));
#24159=CARTESIAN_POINT('Ctrl Pts',(-59.4481729101221,-101.548340522067,
171.985485138407));
#24160=CARTESIAN_POINT('Ctrl Pts',(-60.6032064342299,-101.330925003183,
173.157058062683));
#24161=CARTESIAN_POINT('Ctrl Pts',(-61.7582399583376,-101.113509484299,
174.328630986959));
#24162=CARTESIAN_POINT('Ctrl Pts',(-61.7483018264834,-101.020287726993,
175.985485236451));
#24163=CARTESIAN_POINT('Ctrl Pts',(-61.7383636946293,-100.927065969686,
177.642339485944));
#24164=CARTESIAN_POINT('Ctrl Pts',(-60.5634539471956,-100.958037969653,
178.813912312176));
#24165=CARTESIAN_POINT('Ctrl Pts',(-59.388544199762,-100.98900996962,179.985485138407));
#24166=CARTESIAN_POINT('Ctrl Pts',(-57.7310874497581,-101.071424703906,
179.985485069079));
#24167=CARTESIAN_POINT('Ctrl Pts',(-56.0736306997542,-101.153839438193,
179.985484999752));
#24168=CARTESIAN_POINT('Ctrl Pts',(-54.8987210498124,-101.184811427766,
178.813912075476));
#24169=CARTESIAN_POINT('Ctrl Pts',(-53.7238113998707,-101.21578341734,177.6423391512));
#24170=CARTESIAN_POINT('Ctrl Pts',(-53.7138734058908,-101.122561645335,
175.985484901707));
#24171=CARTESIAN_POINT('Ctrl Pts',(-53.7039354119109,-101.029339873331,
174.328630652215));
#24172=CARTESIAN_POINT('Ctrl Pts',(-54.8589690335105,-100.811924344053,
173.157057825983));
#24173=CARTESIAN_POINT('Ctrl Pts',(-56.0140026551102,-100.594508814776,
171.985484999752));
#24174=CARTESIAN_POINT('Ctrl Pts',(-57.65158327928,-100.325650551179,171.985485069079));
#24175=CARTESIAN_POINT('Ctrl Pts',(-59.2891639034499,-100.056792287582,
171.985485138407));
#24176=CARTESIAN_POINT('Ctrl Pts',(-60.4441974275576,-99.8393767686974,
173.157058062683));
#24177=CARTESIAN_POINT('Ctrl Pts',(-61.5992309516654,-99.6219612498133,
174.328630986959));
#24178=CARTESIAN_POINT('Ctrl Pts',(-61.5892928198112,-99.528739492507,175.985485236451));
#24179=CARTESIAN_POINT('Ctrl Pts',(-61.579354687957,-99.4355177352008,177.642339485944));
#24180=CARTESIAN_POINT('Ctrl Pts',(-60.4044449405234,-99.4664897351676,
178.813912312176));
#24181=CARTESIAN_POINT('Ctrl Pts',(-59.2295351930898,-99.4974617351344,
179.985485138407));
#24182=CARTESIAN_POINT('Ctrl Pts',(-57.5720784430859,-99.5798764694207,
179.985485069079));
#24183=CARTESIAN_POINT('Ctrl Pts',(-55.914621693082,-99.662291203707,179.985484999752));
#24184=CARTESIAN_POINT('Ctrl Pts',(-54.7397120431402,-99.6932631932805,
178.813912075476));
#24185=CARTESIAN_POINT('Ctrl Pts',(-53.5648023931984,-99.724235182854,177.6423391512));
#24186=CARTESIAN_POINT('Ctrl Pts',(-53.5548643992186,-99.6310134108495,
175.985484901707));
#24187=CARTESIAN_POINT('Ctrl Pts',(-53.5449264052387,-99.5377916388449,
174.328630652215));
#24188=CARTESIAN_POINT('Ctrl Pts',(-54.6999600268383,-99.3203761095675,
173.157057825983));
#24189=CARTESIAN_POINT('Ctrl Pts',(-55.8549936484379,-99.10296058029,171.985484999752));
#24190=CARTESIAN_POINT('Ctrl Pts',(-57.4925742726078,-98.834102316693,171.985485069079));
#24191=CARTESIAN_POINT('Ctrl Pts',(-59.1301548967777,-98.5652440530961,
171.985485138407));
#24192=CARTESIAN_POINT('Ctrl Pts',(-60.2851884208854,-98.3478285342118,
173.157058062683));
#24193=CARTESIAN_POINT('Ctrl Pts',(-61.4402219449932,-98.1304130153276,
174.328630986959));
#24194=CARTESIAN_POINT('Ctrl Pts',(-61.430283813139,-98.0371912580215,175.985485236451));
#24195=CARTESIAN_POINT('Ctrl Pts',(-61.4203456812848,-97.9439695007152,
177.642339485944));
#24196=CARTESIAN_POINT('Ctrl Pts',(-60.2454359338512,-97.974941500682,178.813912312176));
#24197=CARTESIAN_POINT('Ctrl Pts',(-59.0705261864175,-98.0059135006488,
179.985485138407));
#24198=CARTESIAN_POINT('Ctrl Pts',(-57.4130694364136,-98.0883282349351,
179.985485069079));
#24199=CARTESIAN_POINT('Ctrl Pts',(-55.7556126864097,-98.1707429692214,
179.985484999752));
#24200=CARTESIAN_POINT('Ctrl Pts',(-54.580703036468,-98.2017149587949,178.813912075476));
#24201=CARTESIAN_POINT('Ctrl Pts',(-56.181115489574,-113.283598570176,178.821287383467));
#24202=CARTESIAN_POINT('Ctrl Pts',(-55.0031681001975,-113.314894403068,
177.646659506339));
#24203=CARTESIAN_POINT('Ctrl Pts',(-54.9932301063974,-113.221672631044,
175.985484901271));
#24204=CARTESIAN_POINT('Ctrl Pts',(-54.9832921125973,-113.12845085902,174.324310296203));
#24205=CARTESIAN_POINT('Ctrl Pts',(-56.1413634738858,-112.910711486397,
173.149682517375));
#24206=CARTESIAN_POINT('Ctrl Pts',(-57.2994348351743,-112.692972113774,
171.975054738546));
#24207=CARTESIAN_POINT('Ctrl Pts',(-58.9413114718314,-112.423655866545,
171.975054808055));
#24208=CARTESIAN_POINT('Ctrl Pts',(-60.5831881084886,-112.154339619316,
171.975054877564));
#24209=CARTESIAN_POINT('Ctrl Pts',(-61.741259372031,-111.936600257113,173.149682754692));
#24210=CARTESIAN_POINT('Ctrl Pts',(-62.8993306355734,-111.71886089491,174.32431063182));
#24211=CARTESIAN_POINT('Ctrl Pts',(-62.8893925035395,-111.625639137623,
175.985485236888));
#24212=CARTESIAN_POINT('Ctrl Pts',(-62.8794543715055,-111.532417380336,
177.646659841956));
#24213=CARTESIAN_POINT('Ctrl Pts',(-61.701506884383,-111.563713223648,178.821287620784));
#24214=CARTESIAN_POINT('Ctrl Pts',(-60.5235593972605,-111.595009066961,
179.995915399612));
#24215=CARTESIAN_POINT('Ctrl Pts',(-58.8618066347693,-111.677881784879,
179.995915330104));
#24216=CARTESIAN_POINT('Ctrl Pts',(-57.2000538722782,-111.760754502798,
179.995915260595));
#24217=CARTESIAN_POINT('Ctrl Pts',(-56.0221064829017,-111.79205033569,178.821287383467));
#24218=CARTESIAN_POINT('Ctrl Pts',(-54.8441590935253,-111.823346168582,
177.646659506339));
#24219=CARTESIAN_POINT('Ctrl Pts',(-54.8342210997252,-111.730124396559,
175.985484901271));
#24220=CARTESIAN_POINT('Ctrl Pts',(-54.8242831059251,-111.636902624535,
174.324310296203));
#24221=CARTESIAN_POINT('Ctrl Pts',(-55.9823544672136,-111.419163251912,
173.149682517375));
#24222=CARTESIAN_POINT('Ctrl Pts',(-57.1404258285021,-111.201423879289,
171.975054738546));
#24223=CARTESIAN_POINT('Ctrl Pts',(-58.7823024651592,-110.932107632059,
171.975054808055));
#24224=CARTESIAN_POINT('Ctrl Pts',(-60.4241791018163,-110.66279138483,171.975054877564));
#24225=CARTESIAN_POINT('Ctrl Pts',(-61.5822503653587,-110.445052022627,
173.149682754692));
#24226=CARTESIAN_POINT('Ctrl Pts',(-62.7403216289012,-110.227312660424,
174.32431063182));
#24227=CARTESIAN_POINT('Ctrl Pts',(-62.7303834968672,-110.134090903137,
175.985485236888));
#24228=CARTESIAN_POINT('Ctrl Pts',(-62.7204453648333,-110.04086914585,177.646659841956));
#24229=CARTESIAN_POINT('Ctrl Pts',(-61.5424978777108,-110.072164989163,
178.821287620784));
#24230=CARTESIAN_POINT('Ctrl Pts',(-60.3645503905882,-110.103460832475,
179.995915399612));
#24231=CARTESIAN_POINT('Ctrl Pts',(-58.7027976280971,-110.186333550394,
179.995915330104));
#24232=CARTESIAN_POINT('Ctrl Pts',(-57.041044865606,-110.269206268313,179.995915260595));
#24233=CARTESIAN_POINT('Ctrl Pts',(-55.8630974762295,-110.300502101205,
178.821287383467));
#24234=CARTESIAN_POINT('Ctrl Pts',(-54.6851500868531,-110.331797934097,
177.646659506339));
#24235=CARTESIAN_POINT('Ctrl Pts',(-54.675212093053,-110.238576162073,175.985484901271));
#24236=CARTESIAN_POINT('Ctrl Pts',(-54.6652740992529,-110.145354390049,
174.324310296203));
#24237=CARTESIAN_POINT('Ctrl Pts',(-55.8233454605414,-109.927615017426,
173.149682517375));
#24238=CARTESIAN_POINT('Ctrl Pts',(-56.9814168218299,-109.709875644803,
171.975054738546));
#24239=CARTESIAN_POINT('Ctrl Pts',(-58.623293458487,-109.440559397574,171.975054808055));
#24240=CARTESIAN_POINT('Ctrl Pts',(-60.2651700951441,-109.171243150344,
171.975054877564));
#24241=CARTESIAN_POINT('Ctrl Pts',(-61.4232413586865,-108.953503788142,
173.149682754692));
#24242=CARTESIAN_POINT('Ctrl Pts',(-62.581312622229,-108.735764425939,174.32431063182));
#24243=CARTESIAN_POINT('Ctrl Pts',(-62.571374490195,-108.642542668652,175.985485236888));
#24244=CARTESIAN_POINT('Ctrl Pts',(-62.5614363581611,-108.549320911365,
177.646659841956));
#24245=CARTESIAN_POINT('Ctrl Pts',(-61.3834888710385,-108.580616754677,
178.821287620784));
#24246=CARTESIAN_POINT('Ctrl Pts',(-60.205541383916,-108.61191259799,179.995915399612));
#24247=CARTESIAN_POINT('Ctrl Pts',(-58.5437886214249,-108.694785315908,
179.995915330104));
#24248=CARTESIAN_POINT('Ctrl Pts',(-56.8820358589338,-108.777658033827,
179.995915260595));
#24249=CARTESIAN_POINT('Ctrl Pts',(-55.7040884695573,-108.808953866719,
178.821287383467));
#24250=CARTESIAN_POINT('Ctrl Pts',(-54.5261410801808,-108.840249699611,
177.646659506339));
#24251=CARTESIAN_POINT('Ctrl Pts',(-54.5162030863807,-108.747027927587,
175.985484901271));
#24252=CARTESIAN_POINT('Ctrl Pts',(-54.5062650925806,-108.653806155564,
174.324310296203));
#24253=CARTESIAN_POINT('Ctrl Pts',(-55.6643364538691,-108.436066782941,
173.149682517375));
#24254=CARTESIAN_POINT('Ctrl Pts',(-56.8224078151577,-108.218327410317,
171.975054738546));
#24255=CARTESIAN_POINT('Ctrl Pts',(-58.4642844518147,-107.949011163088,
171.975054808055));
#24256=CARTESIAN_POINT('Ctrl Pts',(-60.1061610884719,-107.679694915859,
171.975054877564));
#24257=CARTESIAN_POINT('Ctrl Pts',(-61.2642323520143,-107.461955553656,
173.149682754692));
#24258=CARTESIAN_POINT('Ctrl Pts',(-62.4223036155567,-107.244216191453,
174.32431063182));
#24259=CARTESIAN_POINT('Ctrl Pts',(-62.4123654835228,-107.150994434166,
175.985485236888));
#24260=CARTESIAN_POINT('Ctrl Pts',(-62.4024273514889,-107.057772676879,
177.646659841956));
#24261=CARTESIAN_POINT('Ctrl Pts',(-61.2244798643663,-107.089068520192,
178.821287620784));
#24262=CARTESIAN_POINT('Ctrl Pts',(-60.0465323772438,-107.120364363504,
179.995915399612));
#24263=CARTESIAN_POINT('Ctrl Pts',(-58.3847796147526,-107.203237081423,
179.995915330104));
#24264=CARTESIAN_POINT('Ctrl Pts',(-56.7230268522615,-107.286109799341,
179.995915260595));
#24265=CARTESIAN_POINT('Ctrl Pts',(-55.5450794628851,-107.317405632233,
178.821287383467));
#24266=CARTESIAN_POINT('Ctrl Pts',(-54.3671320735086,-107.348701465125,
177.646659506339));
#24267=CARTESIAN_POINT('Ctrl Pts',(-54.3571940797085,-107.255479693102,
175.985484901271));
#24268=CARTESIAN_POINT('Ctrl Pts',(-54.3472560859084,-107.162257921078,
174.324310296203));
#24269=CARTESIAN_POINT('Ctrl Pts',(-55.5053274471969,-106.944518548455,
173.149682517375));
#24270=CARTESIAN_POINT('Ctrl Pts',(-56.6633988084854,-106.726779175832,
171.975054738546));
#24271=CARTESIAN_POINT('Ctrl Pts',(-58.3052754451425,-106.457462928602,
171.975054808055));
#24272=CARTESIAN_POINT('Ctrl Pts',(-59.9471520817997,-106.188146681373,
171.975054877564));
#24273=CARTESIAN_POINT('Ctrl Pts',(-61.1052233453421,-105.97040731917,173.149682754692));
#24274=CARTESIAN_POINT('Ctrl Pts',(-62.2632946088845,-105.752667956968,
174.32431063182));
#24275=CARTESIAN_POINT('Ctrl Pts',(-62.2533564768505,-105.659446199681,
175.985485236888));
#24276=CARTESIAN_POINT('Ctrl Pts',(-62.2434183448166,-105.566224442394,
177.646659841956));
#24277=CARTESIAN_POINT('Ctrl Pts',(-61.0654708576941,-105.597520285706,
178.821287620784));
#24278=CARTESIAN_POINT('Ctrl Pts',(-59.8875233705716,-105.628816129018,
179.995915399612));
#24279=CARTESIAN_POINT('Ctrl Pts',(-58.2257706080804,-105.711688846937,
179.995915330104));
#24280=CARTESIAN_POINT('Ctrl Pts',(-56.5640178455893,-105.794561564856,
179.995915260595));
#24281=CARTESIAN_POINT('Ctrl Pts',(-55.3860704562128,-105.825857397748,
178.821287383467));
#24282=CARTESIAN_POINT('Ctrl Pts',(-54.2081230668364,-105.85715323064,177.646659506339));
#24283=CARTESIAN_POINT('Ctrl Pts',(-54.1981850730363,-105.763931458616,
175.985484901271));
#24284=CARTESIAN_POINT('Ctrl Pts',(-54.1882470792362,-105.670709686593,
174.324310296203));
#24285=CARTESIAN_POINT('Ctrl Pts',(-55.3463184405247,-105.452970313969,
173.149682517375));
#24286=CARTESIAN_POINT('Ctrl Pts',(-56.5043898018132,-105.235230941346,
171.975054738546));
#24287=CARTESIAN_POINT('Ctrl Pts',(-58.1462664384703,-104.965914694117,
171.975054808055));
#24288=CARTESIAN_POINT('Ctrl Pts',(-59.7881430751274,-104.696598446888,
171.975054877564));
#24289=CARTESIAN_POINT('Ctrl Pts',(-60.9462143386698,-104.478859084685,
173.149682754692));
#24290=CARTESIAN_POINT('Ctrl Pts',(-62.1042856022123,-104.261119722482,
174.32431063182));
#24291=CARTESIAN_POINT('Ctrl Pts',(-62.0943474701783,-104.167897965195,
175.985485236888));
#24292=CARTESIAN_POINT('Ctrl Pts',(-62.0844093381444,-104.074676207908,
177.646659841956));
#24293=CARTESIAN_POINT('Ctrl Pts',(-60.9064618510219,-104.10597205122,178.821287620784));
#24294=CARTESIAN_POINT('Ctrl Pts',(-59.7285143638993,-104.137267894533,
179.995915399612));
#24295=CARTESIAN_POINT('Ctrl Pts',(-58.0667616014082,-104.220140612451,
179.995915330104));
#24296=CARTESIAN_POINT('Ctrl Pts',(-56.4050088389171,-104.30301333037,179.995915260595));
#24297=CARTESIAN_POINT('Ctrl Pts',(-55.2270614495406,-104.334309163262,
178.821287383467));
#24298=CARTESIAN_POINT('Ctrl Pts',(-54.0491140601642,-104.365604996154,
177.646659506339));
#24299=CARTESIAN_POINT('Ctrl Pts',(-54.039176066364,-104.272383224131,175.985484901271));
#24300=CARTESIAN_POINT('Ctrl Pts',(-54.029238072564,-104.179161452107,174.324310296203));
#24301=CARTESIAN_POINT('Ctrl Pts',(-55.1873094338524,-103.961422079484,
173.149682517375));
#24302=CARTESIAN_POINT('Ctrl Pts',(-56.345380795141,-103.743682706861,171.975054738546));
#24303=CARTESIAN_POINT('Ctrl Pts',(-57.9872574317981,-103.474366459631,
171.975054808055));
#24304=CARTESIAN_POINT('Ctrl Pts',(-59.6291340684552,-103.205050212402,
171.975054877564));
#24305=CARTESIAN_POINT('Ctrl Pts',(-60.7872053319976,-102.987310850199,
173.149682754692));
#24306=CARTESIAN_POINT('Ctrl Pts',(-61.94527659554,-102.769571487996,174.32431063182));
#24307=CARTESIAN_POINT('Ctrl Pts',(-61.9353384635061,-102.676349730709,
175.985485236888));
#24308=CARTESIAN_POINT('Ctrl Pts',(-61.9254003314722,-102.583127973422,
177.646659841956));
#24309=CARTESIAN_POINT('Ctrl Pts',(-60.7474528443496,-102.614423816735,
178.821287620784));
#24310=CARTESIAN_POINT('Ctrl Pts',(-59.5695053572271,-102.645719660047,
179.995915399612));
#24311=CARTESIAN_POINT('Ctrl Pts',(-57.907752594736,-102.728592377966,179.995915330104));
#24312=CARTESIAN_POINT('Ctrl Pts',(-56.2459998322448,-102.811465095885,
179.995915260595));
#24313=CARTESIAN_POINT('Ctrl Pts',(-55.0680524428684,-102.842760928777,
178.821287383467));
#24314=CARTESIAN_POINT('Ctrl Pts',(-53.8901050534919,-102.874056761669,
177.646659506339));
#24315=CARTESIAN_POINT('Ctrl Pts',(-53.8801670596918,-102.780834989645,
175.985484901271));
#24316=CARTESIAN_POINT('Ctrl Pts',(-53.8702290658917,-102.687613217621,
174.324310296203));
#24317=CARTESIAN_POINT('Ctrl Pts',(-55.0283004271802,-102.469873844998,
173.149682517375));
#24318=CARTESIAN_POINT('Ctrl Pts',(-56.1863717884687,-102.252134472375,
171.975054738546));
#24319=CARTESIAN_POINT('Ctrl Pts',(-57.8282484251258,-101.982818225146,
171.975054808055));
#24320=CARTESIAN_POINT('Ctrl Pts',(-59.470125061783,-101.713501977916,171.975054877564));
#24321=CARTESIAN_POINT('Ctrl Pts',(-60.6281963253254,-101.495762615714,
173.149682754692));
#24322=CARTESIAN_POINT('Ctrl Pts',(-61.7862675888678,-101.278023253511,
174.32431063182));
#24323=CARTESIAN_POINT('Ctrl Pts',(-61.7763294568339,-101.184801496224,
175.985485236888));
#24324=CARTESIAN_POINT('Ctrl Pts',(-61.7663913247999,-101.091579738937,
177.646659841956));
#24325=CARTESIAN_POINT('Ctrl Pts',(-60.5884438376774,-101.122875582249,
178.821287620784));
#24326=CARTESIAN_POINT('Ctrl Pts',(-59.4104963505549,-101.154171425562,
179.995915399612));
#24327=CARTESIAN_POINT('Ctrl Pts',(-57.7487435880637,-101.23704414348,179.995915330104));
#24328=CARTESIAN_POINT('Ctrl Pts',(-56.0869908255726,-101.319916861399,
179.995915260595));
#24329=CARTESIAN_POINT('Ctrl Pts',(-54.9090434361961,-101.351212694291,
178.821287383467));
#24330=CARTESIAN_POINT('Ctrl Pts',(-53.7310960468197,-101.382508527183,
177.646659506339));
#24331=CARTESIAN_POINT('Ctrl Pts',(-53.7211580530196,-101.289286755159,
175.985484901271));
#24332=CARTESIAN_POINT('Ctrl Pts',(-53.7112200592195,-101.196064983136,
174.324310296203));
#24333=CARTESIAN_POINT('Ctrl Pts',(-54.869291420508,-100.978325610513,173.149682517375));
#24334=CARTESIAN_POINT('Ctrl Pts',(-56.0273627817965,-100.760586237889,
171.975054738546));
#24335=CARTESIAN_POINT('Ctrl Pts',(-57.6692394184536,-100.49126999066,171.975054808055));
#24336=CARTESIAN_POINT('Ctrl Pts',(-59.3111160551107,-100.221953743431,
171.975054877564));
#24337=CARTESIAN_POINT('Ctrl Pts',(-60.4691873186531,-100.004214381228,
173.149682754692));
#24338=CARTESIAN_POINT('Ctrl Pts',(-61.6272585821956,-99.7864750190253,
174.32431063182));
#24339=CARTESIAN_POINT('Ctrl Pts',(-61.6173204501616,-99.6932532617382,
175.985485236888));
#24340=CARTESIAN_POINT('Ctrl Pts',(-61.6073823181277,-99.6000315044512,
177.646659841956));
#24341=CARTESIAN_POINT('Ctrl Pts',(-60.4294348310052,-99.6313273477637,
178.821287620784));
#24342=CARTESIAN_POINT('Ctrl Pts',(-59.2514873438827,-99.6626231910761,
179.995915399612));
#24343=CARTESIAN_POINT('Ctrl Pts',(-57.5897345813915,-99.7454959089947,
179.995915330104));
#24344=CARTESIAN_POINT('Ctrl Pts',(-55.9279818189004,-99.8283686269133,
179.995915260595));
#24345=CARTESIAN_POINT('Ctrl Pts',(-54.7500344295239,-99.8596644598054,
178.821287383467));
#24346=CARTESIAN_POINT('Ctrl Pts',(-53.5720870401475,-99.8909602926975,
177.646659506339));
#24347=CARTESIAN_POINT('Ctrl Pts',(-53.5621490463474,-99.7977385206737,
175.985484901271));
#24348=CARTESIAN_POINT('Ctrl Pts',(-53.5522110525473,-99.7045167486501,
174.324310296203));
#24349=CARTESIAN_POINT('Ctrl Pts',(-54.7102824138358,-99.4867773760269,
173.149682517375));
#24350=CARTESIAN_POINT('Ctrl Pts',(-55.8683537751243,-99.2690380034038,
171.975054738546));
#24351=CARTESIAN_POINT('Ctrl Pts',(-57.5102304117814,-98.9997217561745,
171.975054808055));
#24352=CARTESIAN_POINT('Ctrl Pts',(-59.1521070484385,-98.7304055089452,
171.975054877564));
#24353=CARTESIAN_POINT('Ctrl Pts',(-60.3101783119809,-98.5126661467424,
173.149682754692));
#24354=CARTESIAN_POINT('Ctrl Pts',(-61.4682495755234,-98.2949267845397,
174.32431063182));
#24355=CARTESIAN_POINT('Ctrl Pts',(-61.4583114434894,-98.2017050272526,
175.985485236888));
#24356=CARTESIAN_POINT('Ctrl Pts',(-61.4483733114555,-98.1084832699656,
177.646659841956));
#24357=CARTESIAN_POINT('Ctrl Pts',(-60.2704258243329,-98.139779113278,178.821287620784));
#24358=CARTESIAN_POINT('Ctrl Pts',(-59.0924783372104,-98.1710749565905,
179.995915399612));
#24359=CARTESIAN_POINT('Ctrl Pts',(-57.4307255747193,-98.2539476745091,
179.995915330104));
#24360=CARTESIAN_POINT('Ctrl Pts',(-55.7689728122282,-98.3368203924277,
179.995915260595));
#24361=CARTESIAN_POINT('Ctrl Pts',(-54.5910254228517,-98.3681162253198,
178.821287383467));
#24362=CARTESIAN_POINT('Ctrl Pts',(-56.1988062143188,-113.449542435949,
178.821287383467));
#24363=CARTESIAN_POINT('Ctrl Pts',(-55.0208588249424,-113.480838268841,
177.646659506339));
#24364=CARTESIAN_POINT('Ctrl Pts',(-55.0109208311422,-113.387616496817,
175.985484901271));
#24365=CARTESIAN_POINT('Ctrl Pts',(-55.0009828373422,-113.294394724794,
174.324310296203));
#24366=CARTESIAN_POINT('Ctrl Pts',(-56.1590541986307,-113.07665535217,173.149682517375));
#24367=CARTESIAN_POINT('Ctrl Pts',(-57.3171255599192,-112.858915979547,
171.975054738546));
#24368=CARTESIAN_POINT('Ctrl Pts',(-58.9590021965763,-112.589599732318,
171.975054808055));
#24369=CARTESIAN_POINT('Ctrl Pts',(-60.6008788332334,-112.320283485089,
171.975054877564));
#24370=CARTESIAN_POINT('Ctrl Pts',(-61.7589500967758,-112.102544122886,
173.149682754692));
#24371=CARTESIAN_POINT('Ctrl Pts',(-62.9170213603182,-111.884804760683,
174.32431063182));
#24372=CARTESIAN_POINT('Ctrl Pts',(-62.9070832282843,-111.791583003396,
175.985485236888));
#24373=CARTESIAN_POINT('Ctrl Pts',(-62.8971450962504,-111.698361246109,
177.646659841956));
#24374=CARTESIAN_POINT('Ctrl Pts',(-61.7191976091278,-111.729657089422,
178.821287620784));
#24375=CARTESIAN_POINT('Ctrl Pts',(-60.5412501220053,-111.760952932734,
179.995915399612));
#24376=CARTESIAN_POINT('Ctrl Pts',(-58.8794973595142,-111.843825650653,
179.995915330104));
#24377=CARTESIAN_POINT('Ctrl Pts',(-57.217744597023,-111.926698368571,179.995915260595));
#24378=CARTESIAN_POINT('Ctrl Pts',(-56.0397972076466,-111.957994201463,
178.821287383467));
#24379=CARTESIAN_POINT('Ctrl Pts',(-54.8618498182701,-111.989290034355,
177.646659506339));
#24380=CARTESIAN_POINT('Ctrl Pts',(-54.85191182447,-111.896068262332,175.985484901271));
#24381=CARTESIAN_POINT('Ctrl Pts',(-54.8419738306699,-111.802846490308,
174.324310296203));
#24382=CARTESIAN_POINT('Ctrl Pts',(-56.0000451919584,-111.585107117685,
173.149682517375));
#24383=CARTESIAN_POINT('Ctrl Pts',(-57.158116553247,-111.367367745062,171.975054738546));
#24384=CARTESIAN_POINT('Ctrl Pts',(-58.799993189904,-111.098051497832,171.975054808055));
#24385=CARTESIAN_POINT('Ctrl Pts',(-60.4418698265612,-110.828735250603,
171.975054877564));
#24386=CARTESIAN_POINT('Ctrl Pts',(-61.5999410901036,-110.6109958884,173.149682754692));
#24387=CARTESIAN_POINT('Ctrl Pts',(-62.758012353646,-110.393256526198,174.32431063182));
#24388=CARTESIAN_POINT('Ctrl Pts',(-62.7480742216121,-110.30003476891,175.985485236888));
#24389=CARTESIAN_POINT('Ctrl Pts',(-62.7381360895782,-110.206813011623,
177.646659841956));
#24390=CARTESIAN_POINT('Ctrl Pts',(-61.5601886024556,-110.238108854936,
178.821287620784));
#24391=CARTESIAN_POINT('Ctrl Pts',(-60.3822411153331,-110.269404698248,
179.995915399612));
#24392=CARTESIAN_POINT('Ctrl Pts',(-58.7204883528419,-110.352277416167,
179.995915330104));
#24393=CARTESIAN_POINT('Ctrl Pts',(-57.0587355903508,-110.435150134086,
179.995915260595));
#24394=CARTESIAN_POINT('Ctrl Pts',(-55.8807882009743,-110.466445966978,
178.821287383467));
#24395=CARTESIAN_POINT('Ctrl Pts',(-54.7028408115979,-110.49774179987,177.646659506339));
#24396=CARTESIAN_POINT('Ctrl Pts',(-54.6929028177978,-110.404520027846,
175.985484901271));
#24397=CARTESIAN_POINT('Ctrl Pts',(-54.6829648239977,-110.311298255822,
174.324310296203));
#24398=CARTESIAN_POINT('Ctrl Pts',(-55.8410361852862,-110.093558883199,
173.149682517375));
#24399=CARTESIAN_POINT('Ctrl Pts',(-56.9991075465747,-109.875819510576,
171.975054738546));
#24400=CARTESIAN_POINT('Ctrl Pts',(-58.6409841832318,-109.606503263347,
171.975054808055));
#24401=CARTESIAN_POINT('Ctrl Pts',(-60.2828608198889,-109.337187016117,
171.975054877564));
#24402=CARTESIAN_POINT('Ctrl Pts',(-61.4409320834313,-109.119447653915,
173.149682754692));
#24403=CARTESIAN_POINT('Ctrl Pts',(-62.5990033469738,-108.901708291712,
174.32431063182));
#24404=CARTESIAN_POINT('Ctrl Pts',(-62.5890652149398,-108.808486534425,
175.985485236888));
#24405=CARTESIAN_POINT('Ctrl Pts',(-62.5791270829059,-108.715264777138,
177.646659841956));
#24406=CARTESIAN_POINT('Ctrl Pts',(-61.4011795957834,-108.74656062045,178.821287620784));
#24407=CARTESIAN_POINT('Ctrl Pts',(-60.2232321086609,-108.777856463763,
179.995915399612));
#24408=CARTESIAN_POINT('Ctrl Pts',(-58.5614793461697,-108.860729181681,
179.995915330104));
#24409=CARTESIAN_POINT('Ctrl Pts',(-56.8997265836786,-108.9436018996,179.995915260595));
#24410=CARTESIAN_POINT('Ctrl Pts',(-55.7217791943021,-108.974897732492,
178.821287383467));
#24411=CARTESIAN_POINT('Ctrl Pts',(-54.5438318049257,-109.006193565384,
177.646659506339));
#24412=CARTESIAN_POINT('Ctrl Pts',(-54.5338938111256,-108.91297179336,175.985484901271));
#24413=CARTESIAN_POINT('Ctrl Pts',(-54.5239558173255,-108.819750021337,
174.324310296203));
#24414=CARTESIAN_POINT('Ctrl Pts',(-55.682027178614,-108.602010648714,173.149682517375));
#24415=CARTESIAN_POINT('Ctrl Pts',(-56.8400985399025,-108.384271276091,
171.975054738546));
#24416=CARTESIAN_POINT('Ctrl Pts',(-58.4819751765596,-108.114955028861,
171.975054808055));
#24417=CARTESIAN_POINT('Ctrl Pts',(-60.1238518132167,-107.845638781632,
171.975054877564));
#24418=CARTESIAN_POINT('Ctrl Pts',(-61.2819230767591,-107.627899419429,
173.149682754692));
#24419=CARTESIAN_POINT('Ctrl Pts',(-62.4399943403016,-107.410160057226,
174.32431063182));
#24420=CARTESIAN_POINT('Ctrl Pts',(-62.4300562082676,-107.316938299939,
175.985485236888));
#24421=CARTESIAN_POINT('Ctrl Pts',(-62.4201180762337,-107.223716542652,
177.646659841956));
#24422=CARTESIAN_POINT('Ctrl Pts',(-61.2421705891111,-107.255012385965,
178.821287620784));
#24423=CARTESIAN_POINT('Ctrl Pts',(-60.0642231019886,-107.286308229277,
179.995915399612));
#24424=CARTESIAN_POINT('Ctrl Pts',(-58.4024703394975,-107.369180947196,
179.995915330104));
#24425=CARTESIAN_POINT('Ctrl Pts',(-56.7407175770064,-107.452053665114,
179.995915260595));
#24426=CARTESIAN_POINT('Ctrl Pts',(-55.5627701876299,-107.483349498006,
178.821287383467));
#24427=CARTESIAN_POINT('Ctrl Pts',(-54.3848227982534,-107.514645330899,
177.646659506339));
#24428=CARTESIAN_POINT('Ctrl Pts',(-54.3748848044533,-107.421423558875,
175.985484901271));
#24429=CARTESIAN_POINT('Ctrl Pts',(-54.3649468106533,-107.328201786851,
174.324310296203));
#24430=CARTESIAN_POINT('Ctrl Pts',(-55.5230181719417,-107.110462414228,
173.149682517375));
#24431=CARTESIAN_POINT('Ctrl Pts',(-56.6810895332303,-106.892723041605,
171.975054738546));
#24432=CARTESIAN_POINT('Ctrl Pts',(-58.3229661698874,-106.623406794376,
171.975054808055));
#24433=CARTESIAN_POINT('Ctrl Pts',(-59.9648428065445,-106.354090547146,
171.975054877564));
#24434=CARTESIAN_POINT('Ctrl Pts',(-61.1229140700869,-106.136351184943,
173.149682754692));
#24435=CARTESIAN_POINT('Ctrl Pts',(-62.2809853336293,-105.918611822741,
174.32431063182));
#24436=CARTESIAN_POINT('Ctrl Pts',(-62.2710472015954,-105.825390065454,
175.985485236888));
#24437=CARTESIAN_POINT('Ctrl Pts',(-62.2611090695615,-105.732168308167,
177.646659841956));
#24438=CARTESIAN_POINT('Ctrl Pts',(-61.0831615824389,-105.763464151479,
178.821287620784));
#24439=CARTESIAN_POINT('Ctrl Pts',(-59.9052140953164,-105.794759994792,
179.995915399612));
#24440=CARTESIAN_POINT('Ctrl Pts',(-58.2434613328252,-105.87763271271,179.995915330104));
#24441=CARTESIAN_POINT('Ctrl Pts',(-56.5817085703341,-105.960505430629,
179.995915260595));
#24442=CARTESIAN_POINT('Ctrl Pts',(-55.4037611809577,-105.991801263521,
178.821287383467));
#24443=CARTESIAN_POINT('Ctrl Pts',(-54.2258137915812,-106.023097096413,
177.646659506339));
#24444=CARTESIAN_POINT('Ctrl Pts',(-54.2158757977811,-105.929875324389,
175.985484901271));
#24445=CARTESIAN_POINT('Ctrl Pts',(-54.205937803981,-105.836653552366,174.324310296203));
#24446=CARTESIAN_POINT('Ctrl Pts',(-55.3640091652695,-105.618914179742,
173.149682517375));
#24447=CARTESIAN_POINT('Ctrl Pts',(-56.522080526558,-105.401174807119,171.975054738546));
#24448=CARTESIAN_POINT('Ctrl Pts',(-58.1639571632151,-105.13185855989,171.975054808055));
#24449=CARTESIAN_POINT('Ctrl Pts',(-59.8058337998722,-104.862542312661,
171.975054877564));
#24450=CARTESIAN_POINT('Ctrl Pts',(-60.9639050634147,-104.644802950458,
173.149682754692));
#24451=CARTESIAN_POINT('Ctrl Pts',(-62.1219763269571,-104.427063588255,
174.32431063182));
#24452=CARTESIAN_POINT('Ctrl Pts',(-62.1120381949232,-104.333841830968,
175.985485236888));
#24453=CARTESIAN_POINT('Ctrl Pts',(-62.1021000628892,-104.240620073681,
177.646659841956));
#24454=CARTESIAN_POINT('Ctrl Pts',(-60.9241525757667,-104.271915916993,
178.821287620784));
#24455=CARTESIAN_POINT('Ctrl Pts',(-59.7462050886442,-104.303211760306,
179.995915399612));
#24456=CARTESIAN_POINT('Ctrl Pts',(-58.084452326153,-104.386084478225,179.995915330104));
#24457=CARTESIAN_POINT('Ctrl Pts',(-56.4226995636619,-104.468957196143,
179.995915260595));
#24458=CARTESIAN_POINT('Ctrl Pts',(-55.2447521742854,-104.500253029035,
178.821287383467));
#24459=CARTESIAN_POINT('Ctrl Pts',(-54.066804784909,-104.531548861927,177.646659506339));
#24460=CARTESIAN_POINT('Ctrl Pts',(-54.0568667911089,-104.438327089904,
175.985484901271));
#24461=CARTESIAN_POINT('Ctrl Pts',(-54.0469287973088,-104.34510531788,174.324310296203));
#24462=CARTESIAN_POINT('Ctrl Pts',(-55.2050001585973,-104.127365945257,
173.149682517375));
#24463=CARTESIAN_POINT('Ctrl Pts',(-56.3630715198858,-103.909626572634,
171.975054738546));
#24464=CARTESIAN_POINT('Ctrl Pts',(-58.0049481565429,-103.640310325404,
171.975054808055));
#24465=CARTESIAN_POINT('Ctrl Pts',(-59.6468247932,-103.370994078175,171.975054877564));
#24466=CARTESIAN_POINT('Ctrl Pts',(-60.8048960567424,-103.153254715972,
173.149682754692));
#24467=CARTESIAN_POINT('Ctrl Pts',(-61.9629673202849,-102.93551535377,174.32431063182));
#24468=CARTESIAN_POINT('Ctrl Pts',(-61.9530291882509,-102.842293596483,
175.985485236888));
#24469=CARTESIAN_POINT('Ctrl Pts',(-61.943091056217,-102.749071839196,177.646659841956));
#24470=CARTESIAN_POINT('Ctrl Pts',(-60.7651435690945,-102.780367682508,
178.821287620784));
#24471=CARTESIAN_POINT('Ctrl Pts',(-59.587196081972,-102.81166352582,179.995915399612));
#24472=CARTESIAN_POINT('Ctrl Pts',(-57.9254433194808,-102.894536243739,
179.995915330104));
#24473=CARTESIAN_POINT('Ctrl Pts',(-56.2636905569897,-102.977408961658,
179.995915260595));
#24474=CARTESIAN_POINT('Ctrl Pts',(-55.0857431676132,-103.00870479455,178.821287383467));
#24475=CARTESIAN_POINT('Ctrl Pts',(-53.9077957782368,-103.040000627442,
177.646659506339));
#24476=CARTESIAN_POINT('Ctrl Pts',(-53.8978577844367,-102.946778855418,
175.985484901271));
#24477=CARTESIAN_POINT('Ctrl Pts',(-53.8879197906366,-102.853557083394,
174.324310296203));
#24478=CARTESIAN_POINT('Ctrl Pts',(-55.0459911519251,-102.635817710771,
173.149682517375));
#24479=CARTESIAN_POINT('Ctrl Pts',(-56.2040625132136,-102.418078338148,
171.975054738546));
#24480=CARTESIAN_POINT('Ctrl Pts',(-57.8459391498707,-102.148762090919,
171.975054808055));
#24481=CARTESIAN_POINT('Ctrl Pts',(-59.4878157865278,-101.879445843689,
171.975054877564));
#24482=CARTESIAN_POINT('Ctrl Pts',(-60.6458870500702,-101.661706481487,
173.149682754692));
#24483=CARTESIAN_POINT('Ctrl Pts',(-61.8039583136126,-101.443967119284,
174.32431063182));
#24484=CARTESIAN_POINT('Ctrl Pts',(-61.7940201815787,-101.350745361997,
175.985485236888));
#24485=CARTESIAN_POINT('Ctrl Pts',(-61.7840820495448,-101.25752360471,177.646659841956));
#24486=CARTESIAN_POINT('Ctrl Pts',(-60.6061345624222,-101.288819448022,
178.821287620784));
#24487=CARTESIAN_POINT('Ctrl Pts',(-59.4281870752997,-101.320115291335,
179.995915399612));
#24488=CARTESIAN_POINT('Ctrl Pts',(-57.7664343128086,-101.402988009253,
179.995915330104));
#24489=CARTESIAN_POINT('Ctrl Pts',(-56.1046815503175,-101.485860727172,
179.995915260595));
#24490=CARTESIAN_POINT('Ctrl Pts',(-54.926734160941,-101.517156560064,178.821287383467));
#24491=CARTESIAN_POINT('Ctrl Pts',(-53.7487867715645,-101.548452392956,
177.646659506339));
#24492=CARTESIAN_POINT('Ctrl Pts',(-53.7388487777644,-101.455230620932,
175.985484901271));
#24493=CARTESIAN_POINT('Ctrl Pts',(-53.7289107839643,-101.362008848909,
174.324310296203));
#24494=CARTESIAN_POINT('Ctrl Pts',(-54.8869821452528,-101.144269476286,
173.149682517375));
#24495=CARTESIAN_POINT('Ctrl Pts',(-56.0450535065414,-100.926530103662,
171.975054738546));
#24496=CARTESIAN_POINT('Ctrl Pts',(-57.6869301431984,-100.657213856433,
171.975054808055));
#24497=CARTESIAN_POINT('Ctrl Pts',(-59.3288067798556,-100.387897609204,
171.975054877564));
#24498=CARTESIAN_POINT('Ctrl Pts',(-60.486878043398,-100.170158247001,173.149682754692));
#24499=CARTESIAN_POINT('Ctrl Pts',(-61.6449493069404,-99.9524188847983,
174.32431063182));
#24500=CARTESIAN_POINT('Ctrl Pts',(-61.6350111749065,-99.8591971275113,
175.985485236888));
#24501=CARTESIAN_POINT('Ctrl Pts',(-61.6250730428726,-99.7659753702243,
177.646659841956));
#24502=CARTESIAN_POINT('Ctrl Pts',(-60.44712555575,-99.7972712135367,178.821287620784));
#24503=CARTESIAN_POINT('Ctrl Pts',(-59.2691780686275,-99.8285670568492,
179.995915399612));
#24504=CARTESIAN_POINT('Ctrl Pts',(-57.6074253061363,-99.9114397747677,
179.995915330104));
#24505=CARTESIAN_POINT('Ctrl Pts',(-55.9456725436452,-99.9943124926864,
179.995915260595));
#24506=CARTESIAN_POINT('Ctrl Pts',(-54.7677251542687,-100.025608325578,
178.821287383467));
#24507=CARTESIAN_POINT('Ctrl Pts',(-53.5897777648923,-100.05690415847,177.646659506339));
#24508=CARTESIAN_POINT('Ctrl Pts',(-53.5798397710922,-99.9636823864468,
175.985484901271));
#24509=CARTESIAN_POINT('Ctrl Pts',(-53.5699017772921,-99.8704606144232,
174.324310296203));
#24510=CARTESIAN_POINT('Ctrl Pts',(-54.7279731385806,-99.6527212418,173.149682517375));
#24511=CARTESIAN_POINT('Ctrl Pts',(-55.8860444998691,-99.4349818691769,
171.975054738546));
#24512=CARTESIAN_POINT('Ctrl Pts',(-57.5279211365262,-99.1656656219475,
171.975054808055));
#24513=CARTESIAN_POINT('Ctrl Pts',(-59.1697977731833,-98.8963493747183,
171.975054877564));
#24514=CARTESIAN_POINT('Ctrl Pts',(-60.3278690367257,-98.6786100125155,
173.149682754692));
#24515=CARTESIAN_POINT('Ctrl Pts',(-61.4859403002682,-98.4608706503128,
174.32431063182));
#24516=CARTESIAN_POINT('Ctrl Pts',(-61.4760021682342,-98.3676488930257,
175.985485236888));
#24517=CARTESIAN_POINT('Ctrl Pts',(-61.4660640362003,-98.2744271357387,
177.646659841956));
#24518=CARTESIAN_POINT('Ctrl Pts',(-60.2881165490778,-98.3057229790511,
178.821287620784));
#24519=CARTESIAN_POINT('Ctrl Pts',(-59.1101690619552,-98.3370188223636,
179.995915399612));
#24520=CARTESIAN_POINT('Ctrl Pts',(-57.4484162994641,-98.4198915402821,
179.995915330104));
#24521=CARTESIAN_POINT('Ctrl Pts',(-55.786663536973,-98.5027642582008,179.995915260595));
#24522=CARTESIAN_POINT('Ctrl Pts',(-54.6087161475965,-98.5340600910929,
178.821287383467));
#24523=CARTESIAN_POINT('Ctrl Pts',(-56.2237961054143,-113.614380048479,
178.813912075476));
#24524=CARTESIAN_POINT('Ctrl Pts',(-55.0488864554725,-113.645352038053,
177.6423391512));
#24525=CARTESIAN_POINT('Ctrl Pts',(-55.0389484614927,-113.552130266048,
175.985484901707));
#24526=CARTESIAN_POINT('Ctrl Pts',(-55.0290104675128,-113.458908494044,
174.328630652215));
#24527=CARTESIAN_POINT('Ctrl Pts',(-56.1840440891124,-113.241492964766,
173.157057825983));
#24528=CARTESIAN_POINT('Ctrl Pts',(-57.3390777107121,-113.024077435489,
171.985484999752));
#24529=CARTESIAN_POINT('Ctrl Pts',(-58.9766583348819,-112.755219171892,
171.985485069079));
#24530=CARTESIAN_POINT('Ctrl Pts',(-60.6142389590518,-112.486360908295,
171.985485138407));
#24531=CARTESIAN_POINT('Ctrl Pts',(-61.7692724831595,-112.268945389411,
173.157058062683));
#24532=CARTESIAN_POINT('Ctrl Pts',(-62.9243060072673,-112.051529870527,
174.328630986959));
#24533=CARTESIAN_POINT('Ctrl Pts',(-62.9143678754131,-111.95830811322,175.985485236451));
#24534=CARTESIAN_POINT('Ctrl Pts',(-62.9044297435589,-111.865086355914,
177.642339485944));
#24535=CARTESIAN_POINT('Ctrl Pts',(-61.7295199961253,-111.896058355881,
178.813912312176));
#24536=CARTESIAN_POINT('Ctrl Pts',(-60.5546102486917,-111.927030355848,
179.985485138407));
#24537=CARTESIAN_POINT('Ctrl Pts',(-58.8971534986878,-112.009445090134,
179.985485069079));
#24538=CARTESIAN_POINT('Ctrl Pts',(-57.2396967486839,-112.09185982442,179.985484999752));
#24539=CARTESIAN_POINT('Ctrl Pts',(-56.0647870987421,-112.122831813994,
178.813912075476));
#24540=CARTESIAN_POINT('Ctrl Pts',(-54.8898774488003,-112.153803803567,
177.6423391512));
#24541=CARTESIAN_POINT('Ctrl Pts',(-54.8799394548205,-112.060582031563,
175.985484901707));
#24542=CARTESIAN_POINT('Ctrl Pts',(-54.8700014608406,-111.967360259558,
174.328630652215));
#24543=CARTESIAN_POINT('Ctrl Pts',(-56.0250350824402,-111.749944730281,
173.157057825983));
#24544=CARTESIAN_POINT('Ctrl Pts',(-57.1800687040398,-111.532529201003,
171.985484999752));
#24545=CARTESIAN_POINT('Ctrl Pts',(-58.8176493282097,-111.263670937406,
171.985485069079));
#24546=CARTESIAN_POINT('Ctrl Pts',(-60.4552299523796,-110.994812673809,
171.985485138407));
#24547=CARTESIAN_POINT('Ctrl Pts',(-61.6102634764873,-110.777397154925,
173.157058062683));
#24548=CARTESIAN_POINT('Ctrl Pts',(-62.7652970005951,-110.559981636041,
174.328630986959));
#24549=CARTESIAN_POINT('Ctrl Pts',(-62.7553588687409,-110.466759878735,
175.985485236451));
#24550=CARTESIAN_POINT('Ctrl Pts',(-62.7454207368867,-110.373538121429,
177.642339485944));
#24551=CARTESIAN_POINT('Ctrl Pts',(-61.5705109894531,-110.404510121395,
178.813912312176));
#24552=CARTESIAN_POINT('Ctrl Pts',(-60.3956012420194,-110.435482121362,
179.985485138407));
#24553=CARTESIAN_POINT('Ctrl Pts',(-58.7381444920155,-110.517896855648,
179.985485069079));
#24554=CARTESIAN_POINT('Ctrl Pts',(-57.0806877420116,-110.600311589935,
179.985484999752));
#24555=CARTESIAN_POINT('Ctrl Pts',(-55.9057780920699,-110.631283579508,
178.813912075476));
#24556=CARTESIAN_POINT('Ctrl Pts',(-54.7308684421281,-110.662255569082,
177.6423391512));
#24557=CARTESIAN_POINT('Ctrl Pts',(-54.7209304481482,-110.569033797077,
175.985484901707));
#24558=CARTESIAN_POINT('Ctrl Pts',(-54.7109924541684,-110.475812025073,
174.328630652215));
#24559=CARTESIAN_POINT('Ctrl Pts',(-55.866026075768,-110.258396495795,173.157057825983));
#24560=CARTESIAN_POINT('Ctrl Pts',(-57.0210596973676,-110.040980966518,
171.985484999752));
#24561=CARTESIAN_POINT('Ctrl Pts',(-58.6586403215375,-109.772122702921,
171.985485069079));
#24562=CARTESIAN_POINT('Ctrl Pts',(-60.2962209457073,-109.503264439324,
171.985485138407));
#24563=CARTESIAN_POINT('Ctrl Pts',(-61.4512544698151,-109.28584892044,173.157058062683));
#24564=CARTESIAN_POINT('Ctrl Pts',(-62.6062879939228,-109.068433401555,
174.328630986959));
#24565=CARTESIAN_POINT('Ctrl Pts',(-62.5963498620687,-108.975211644249,
175.985485236451));
#24566=CARTESIAN_POINT('Ctrl Pts',(-62.5864117302145,-108.881989886943,
177.642339485944));
#24567=CARTESIAN_POINT('Ctrl Pts',(-61.4115019827808,-108.91296188691,178.813912312176));
#24568=CARTESIAN_POINT('Ctrl Pts',(-60.2365922353472,-108.943933886877,
179.985485138407));
#24569=CARTESIAN_POINT('Ctrl Pts',(-58.5791354853433,-109.026348621163,
179.985485069079));
#24570=CARTESIAN_POINT('Ctrl Pts',(-56.9216787353394,-109.108763355449,
179.985484999752));
#24571=CARTESIAN_POINT('Ctrl Pts',(-55.7467690853976,-109.139735345023,
178.813912075476));
#24572=CARTESIAN_POINT('Ctrl Pts',(-54.5718594354559,-109.170707334596,
177.6423391512));
#24573=CARTESIAN_POINT('Ctrl Pts',(-54.561921441476,-109.077485562592,175.985484901707));
#24574=CARTESIAN_POINT('Ctrl Pts',(-54.5519834474962,-108.984263790587,
174.328630652215));
#24575=CARTESIAN_POINT('Ctrl Pts',(-55.7070170690958,-108.76684826131,173.157057825983));
#24576=CARTESIAN_POINT('Ctrl Pts',(-56.8620506906954,-108.549432732032,
171.985484999752));
#24577=CARTESIAN_POINT('Ctrl Pts',(-58.4996313148652,-108.280574468435,
171.985485069079));
#24578=CARTESIAN_POINT('Ctrl Pts',(-60.1372119390351,-108.011716204838,
171.985485138407));
#24579=CARTESIAN_POINT('Ctrl Pts',(-61.2922454631428,-107.794300685954,
173.157058062683));
#24580=CARTESIAN_POINT('Ctrl Pts',(-62.4472789872506,-107.57688516707,174.328630986959));
#24581=CARTESIAN_POINT('Ctrl Pts',(-62.4373408553964,-107.483663409764,
175.985485236451));
#24582=CARTESIAN_POINT('Ctrl Pts',(-62.4274027235423,-107.390441652457,
177.642339485944));
#24583=CARTESIAN_POINT('Ctrl Pts',(-61.2524929761086,-107.421413652424,
178.813912312176));
#24584=CARTESIAN_POINT('Ctrl Pts',(-60.077583228675,-107.452385652391,179.985485138407));
#24585=CARTESIAN_POINT('Ctrl Pts',(-58.4201264786711,-107.534800386677,
179.985485069079));
#24586=CARTESIAN_POINT('Ctrl Pts',(-56.7626697286672,-107.617215120964,
179.985484999752));
#24587=CARTESIAN_POINT('Ctrl Pts',(-55.5877600787254,-107.648187110537,
178.813912075476));
#24588=CARTESIAN_POINT('Ctrl Pts',(-54.4128504287836,-107.67915910011,177.6423391512));
#24589=CARTESIAN_POINT('Ctrl Pts',(-54.4029124348038,-107.585937328106,
175.985484901707));
#24590=CARTESIAN_POINT('Ctrl Pts',(-54.3929744408239,-107.492715556102,
174.328630652215));
#24591=CARTESIAN_POINT('Ctrl Pts',(-55.5480080624235,-107.275300026824,
173.157057825983));
#24592=CARTESIAN_POINT('Ctrl Pts',(-56.7030416840231,-107.057884497547,
171.985484999752));
#24593=CARTESIAN_POINT('Ctrl Pts',(-58.340622308193,-106.78902623395,171.985485069079));
#24594=CARTESIAN_POINT('Ctrl Pts',(-59.9782029323629,-106.520167970353,
171.985485138407));
#24595=CARTESIAN_POINT('Ctrl Pts',(-61.1332364564706,-106.302752451468,
173.157058062683));
#24596=CARTESIAN_POINT('Ctrl Pts',(-62.2882699805784,-106.085336932584,
174.328630986959));
#24597=CARTESIAN_POINT('Ctrl Pts',(-62.2783318487242,-105.992115175278,
175.985485236451));
#24598=CARTESIAN_POINT('Ctrl Pts',(-62.26839371687,-105.898893417972,177.642339485944));
#24599=CARTESIAN_POINT('Ctrl Pts',(-61.0934839694364,-105.929865417939,
178.813912312176));
#24600=CARTESIAN_POINT('Ctrl Pts',(-59.9185742220028,-105.960837417905,
179.985485138407));
#24601=CARTESIAN_POINT('Ctrl Pts',(-58.2611174719989,-106.043252152192,
179.985485069079));
#24602=CARTESIAN_POINT('Ctrl Pts',(-56.603660721995,-106.125666886478,179.985484999752));
#24603=CARTESIAN_POINT('Ctrl Pts',(-55.4287510720532,-106.156638876051,
178.813912075476));
#24604=CARTESIAN_POINT('Ctrl Pts',(-54.2538414221114,-106.187610865625,
177.6423391512));
#24605=CARTESIAN_POINT('Ctrl Pts',(-54.2439034281315,-106.09438909362,175.985484901707));
#24606=CARTESIAN_POINT('Ctrl Pts',(-54.2339654341517,-106.001167321616,
174.328630652215));
#24607=CARTESIAN_POINT('Ctrl Pts',(-55.3889990557513,-105.783751792338,
173.157057825983));
#24608=CARTESIAN_POINT('Ctrl Pts',(-56.5440326773509,-105.566336263061,
171.985484999752));
#24609=CARTESIAN_POINT('Ctrl Pts',(-58.1816133015208,-105.297477999464,
171.985485069079));
#24610=CARTESIAN_POINT('Ctrl Pts',(-59.8191939256906,-105.028619735867,
171.985485138407));
#24611=CARTESIAN_POINT('Ctrl Pts',(-60.9742274497984,-104.811204216983,
173.157058062683));
#24612=CARTESIAN_POINT('Ctrl Pts',(-62.1292609739061,-104.593788698099,
174.328630986959));
#24613=CARTESIAN_POINT('Ctrl Pts',(-62.119322842052,-104.500566940792,175.985485236451));
#24614=CARTESIAN_POINT('Ctrl Pts',(-62.1093847101978,-104.407345183486,
177.642339485944));
#24615=CARTESIAN_POINT('Ctrl Pts',(-60.9344749627642,-104.438317183453,
178.813912312176));
#24616=CARTESIAN_POINT('Ctrl Pts',(-59.7595652153305,-104.46928918342,179.985485138407));
#24617=CARTESIAN_POINT('Ctrl Pts',(-58.1021084653266,-104.551703917706,
179.985485069079));
#24618=CARTESIAN_POINT('Ctrl Pts',(-56.4446517153227,-104.634118651992,
179.985484999752));
#24619=CARTESIAN_POINT('Ctrl Pts',(-55.269742065381,-104.665090641566,178.813912075476));
#24620=CARTESIAN_POINT('Ctrl Pts',(-54.0948324154392,-104.696062631139,
177.6423391512));
#24621=CARTESIAN_POINT('Ctrl Pts',(-54.0848944214593,-104.602840859135,
175.985484901707));
#24622=CARTESIAN_POINT('Ctrl Pts',(-54.0749564274795,-104.50961908713,174.328630652215));
#24623=CARTESIAN_POINT('Ctrl Pts',(-55.2299900490791,-104.292203557853,
173.157057825983));
#24624=CARTESIAN_POINT('Ctrl Pts',(-56.3850236706787,-104.074788028575,
171.985484999752));
#24625=CARTESIAN_POINT('Ctrl Pts',(-58.0226042948486,-103.805929764978,
171.985485069079));
#24626=CARTESIAN_POINT('Ctrl Pts',(-59.6601849190184,-103.537071501381,
171.985485138407));
#24627=CARTESIAN_POINT('Ctrl Pts',(-60.8152184431262,-103.319655982497,
173.157058062683));
#24628=CARTESIAN_POINT('Ctrl Pts',(-61.9702519672339,-103.102240463613,
174.328630986959));
#24629=CARTESIAN_POINT('Ctrl Pts',(-61.9603138353797,-103.009018706307,
175.985485236451));
#24630=CARTESIAN_POINT('Ctrl Pts',(-61.9503757035256,-102.915796949001,
177.642339485944));
#24631=CARTESIAN_POINT('Ctrl Pts',(-60.7754659560919,-102.946768948967,
178.813912312176));
#24632=CARTESIAN_POINT('Ctrl Pts',(-59.6005562086583,-102.977740948934,
179.985485138407));
#24633=CARTESIAN_POINT('Ctrl Pts',(-57.9430994586544,-103.06015568322,179.985485069079));
#24634=CARTESIAN_POINT('Ctrl Pts',(-56.2856427086505,-103.142570417507,
179.985484999752));
#24635=CARTESIAN_POINT('Ctrl Pts',(-55.1107330587087,-103.17354240708,178.813912075476));
#24636=CARTESIAN_POINT('Ctrl Pts',(-53.935823408767,-103.204514396654,177.6423391512));
#24637=CARTESIAN_POINT('Ctrl Pts',(-53.9258854147871,-103.111292624649,
175.985484901707));
#24638=CARTESIAN_POINT('Ctrl Pts',(-53.9159474208072,-103.018070852645,
174.328630652215));
#24639=CARTESIAN_POINT('Ctrl Pts',(-55.0709810424069,-102.800655323367,
173.157057825983));
#24640=CARTESIAN_POINT('Ctrl Pts',(-56.2260146640065,-102.58323979409,171.985484999752));
#24641=CARTESIAN_POINT('Ctrl Pts',(-57.8635952881763,-102.314381530493,
171.985485069079));
#24642=CARTESIAN_POINT('Ctrl Pts',(-59.5011759123462,-102.045523266896,
171.985485138407));
#24643=CARTESIAN_POINT('Ctrl Pts',(-60.6562094364539,-101.828107748012,
173.157058062683));
#24644=CARTESIAN_POINT('Ctrl Pts',(-61.8112429605617,-101.610692229127,
174.328630986959));
#24645=CARTESIAN_POINT('Ctrl Pts',(-61.8013048287075,-101.517470471821,
175.985485236451));
#24646=CARTESIAN_POINT('Ctrl Pts',(-61.7913666968533,-101.424248714515,
177.642339485944));
#24647=CARTESIAN_POINT('Ctrl Pts',(-60.6164569494197,-101.455220714482,
178.813912312176));
#24648=CARTESIAN_POINT('Ctrl Pts',(-59.4415472019861,-101.486192714449,
179.985485138407));
#24649=CARTESIAN_POINT('Ctrl Pts',(-57.7840904519822,-101.568607448735,
179.985485069079));
#24650=CARTESIAN_POINT('Ctrl Pts',(-56.1266337019783,-101.651022183021,
179.985484999752));
#24651=CARTESIAN_POINT('Ctrl Pts',(-54.9517240520365,-101.681994172595,
178.813912075476));
#24652=CARTESIAN_POINT('Ctrl Pts',(-53.7768144020947,-101.712966162168,
177.6423391512));
#24653=CARTESIAN_POINT('Ctrl Pts',(-53.7668764081149,-101.619744390164,
175.985484901707));
#24654=CARTESIAN_POINT('Ctrl Pts',(-53.756938414135,-101.526522618159,174.328630652215));
#24655=CARTESIAN_POINT('Ctrl Pts',(-54.9119720357346,-101.309107088882,
173.157057825983));
#24656=CARTESIAN_POINT('Ctrl Pts',(-56.0670056573342,-101.091691559604,
171.985484999752));
#24657=CARTESIAN_POINT('Ctrl Pts',(-57.7045862815041,-100.822833296007,
171.985485069079));
#24658=CARTESIAN_POINT('Ctrl Pts',(-59.342166905674,-100.55397503241,171.985485138407));
#24659=CARTESIAN_POINT('Ctrl Pts',(-60.4972004297817,-100.336559513526,
173.157058062683));
#24660=CARTESIAN_POINT('Ctrl Pts',(-61.6522339538895,-100.119143994642,
174.328630986959));
#24661=CARTESIAN_POINT('Ctrl Pts',(-61.6422958220353,-100.025922237336,
175.985485236451));
#24662=CARTESIAN_POINT('Ctrl Pts',(-61.6323576901811,-99.9327004800294,
177.642339485944));
#24663=CARTESIAN_POINT('Ctrl Pts',(-60.4574479427475,-99.9636724799962,
178.813912312176));
#24664=CARTESIAN_POINT('Ctrl Pts',(-59.2825381953138,-99.994644479963,179.985485138407));
#24665=CARTESIAN_POINT('Ctrl Pts',(-57.6250814453099,-100.077059214249,
179.985485069079));
#24666=CARTESIAN_POINT('Ctrl Pts',(-55.9676246953061,-100.159473948536,
179.985484999752));
#24667=CARTESIAN_POINT('Ctrl Pts',(-54.7927150453643,-100.190445938109,
178.813912075476));
#24668=CARTESIAN_POINT('Ctrl Pts',(-53.6178053954225,-100.221417927683,
177.6423391512));
#24669=CARTESIAN_POINT('Ctrl Pts',(-53.6078674014426,-100.128196155678,
175.985484901707));
#24670=CARTESIAN_POINT('Ctrl Pts',(-53.5979294074628,-100.034974383673,
174.328630652215));
#24671=CARTESIAN_POINT('Ctrl Pts',(-54.7529630290624,-99.817558854396,173.157057825983));
#24672=CARTESIAN_POINT('Ctrl Pts',(-55.907996650662,-99.6001433251185,171.985484999752));
#24673=CARTESIAN_POINT('Ctrl Pts',(-57.5455772748319,-99.3312850615215,
171.985485069079));
#24674=CARTESIAN_POINT('Ctrl Pts',(-59.1831578990017,-99.0624267979246,
171.985485138407));
#24675=CARTESIAN_POINT('Ctrl Pts',(-60.3381914231095,-98.8450112790404,
173.157058062683));
#24676=CARTESIAN_POINT('Ctrl Pts',(-61.4932249472172,-98.6275957601562,
174.328630986959));
#24677=CARTESIAN_POINT('Ctrl Pts',(-61.4832868153631,-98.53437400285,175.985485236451));
#24678=CARTESIAN_POINT('Ctrl Pts',(-61.4733486835089,-98.4411522455438,
177.642339485944));
#24679=CARTESIAN_POINT('Ctrl Pts',(-60.2984389360752,-98.4721242455106,
178.813912312176));
#24680=CARTESIAN_POINT('Ctrl Pts',(-59.1235291886416,-98.5030962454774,
179.985485138407));
#24681=CARTESIAN_POINT('Ctrl Pts',(-57.4660724386377,-98.5855109797636,
179.985485069079));
#24682=CARTESIAN_POINT('Ctrl Pts',(-55.8086156886338,-98.6679257140499,
179.985484999752));
#24683=CARTESIAN_POINT('Ctrl Pts',(-54.633706038692,-98.6988977036234,178.813912075476));
#24684=CARTESIAN_POINT('Ctrl Pts',(-56.2237961054143,-113.614380048479,
178.813912075476));
#24685=CARTESIAN_POINT('Ctrl Pts',(-55.0488864554725,-113.645352038053,
177.6423391512));
#24686=CARTESIAN_POINT('Ctrl Pts',(-55.0389484614927,-113.552130266048,
175.985484901707));
#24687=CARTESIAN_POINT('Ctrl Pts',(-55.0290104675128,-113.458908494044,
174.328630652215));
#24688=CARTESIAN_POINT('Ctrl Pts',(-56.1840440891124,-113.241492964766,
173.157057825983));
#24689=CARTESIAN_POINT('Ctrl Pts',(-57.3390777107121,-113.024077435489,
171.985484999752));
#24690=CARTESIAN_POINT('Ctrl Pts',(-58.9766583348819,-112.755219171892,
171.985485069079));
#24691=CARTESIAN_POINT('Ctrl Pts',(-60.6142389590518,-112.486360908295,
171.985485138407));
#24692=CARTESIAN_POINT('Ctrl Pts',(-61.7692724831595,-112.268945389411,
173.157058062683));
#24693=CARTESIAN_POINT('Ctrl Pts',(-62.9243060072673,-112.051529870527,
174.328630986959));
#24694=CARTESIAN_POINT('Ctrl Pts',(-62.9143678754131,-111.95830811322,175.985485236451));
#24695=CARTESIAN_POINT('Ctrl Pts',(-62.9044297435589,-111.865086355914,
177.642339485944));
#24696=CARTESIAN_POINT('Ctrl Pts',(-61.7295199961253,-111.896058355881,
178.813912312176));
#24697=CARTESIAN_POINT('Ctrl Pts',(-60.5546102486917,-111.927030355848,
179.985485138407));
#24698=CARTESIAN_POINT('Ctrl Pts',(-58.8971534986878,-112.009445090134,
179.985485069079));
#24699=CARTESIAN_POINT('Ctrl Pts',(-57.2396967486839,-112.09185982442,179.985484999752));
#24700=CARTESIAN_POINT('Ctrl Pts',(-56.0647870987421,-112.122831813994,
178.813912075476));
#24701=CARTESIAN_POINT('Ctrl Pts',(-54.8898774488003,-112.153803803567,
177.6423391512));
#24702=CARTESIAN_POINT('Ctrl Pts',(-54.8799394548205,-112.060582031563,
175.985484901707));
#24703=CARTESIAN_POINT('Ctrl Pts',(-54.8700014608406,-111.967360259558,
174.328630652215));
#24704=CARTESIAN_POINT('Ctrl Pts',(-56.0250350824402,-111.749944730281,
173.157057825983));
#24705=CARTESIAN_POINT('Ctrl Pts',(-57.1800687040398,-111.532529201003,
171.985484999752));
#24706=CARTESIAN_POINT('Ctrl Pts',(-58.8176493282097,-111.263670937406,
171.985485069079));
#24707=CARTESIAN_POINT('Ctrl Pts',(-60.4552299523796,-110.994812673809,
171.985485138407));
#24708=CARTESIAN_POINT('Ctrl Pts',(-61.6102634764873,-110.777397154925,
173.157058062683));
#24709=CARTESIAN_POINT('Ctrl Pts',(-62.7652970005951,-110.559981636041,
174.328630986959));
#24710=CARTESIAN_POINT('Ctrl Pts',(-62.7553588687409,-110.466759878735,
175.985485236451));
#24711=CARTESIAN_POINT('Ctrl Pts',(-62.7454207368867,-110.373538121429,
177.642339485944));
#24712=CARTESIAN_POINT('Ctrl Pts',(-61.5705109894531,-110.404510121395,
178.813912312176));
#24713=CARTESIAN_POINT('Ctrl Pts',(-60.3956012420194,-110.435482121362,
179.985485138407));
#24714=CARTESIAN_POINT('Ctrl Pts',(-58.7381444920155,-110.517896855648,
179.985485069079));
#24715=CARTESIAN_POINT('Ctrl Pts',(-57.0806877420116,-110.600311589935,
179.985484999752));
#24716=CARTESIAN_POINT('Ctrl Pts',(-55.9057780920699,-110.631283579508,
178.813912075476));
#24717=CARTESIAN_POINT('Ctrl Pts',(-54.7308684421281,-110.662255569082,
177.6423391512));
#24718=CARTESIAN_POINT('Ctrl Pts',(-54.7209304481482,-110.569033797077,
175.985484901707));
#24719=CARTESIAN_POINT('Ctrl Pts',(-54.7109924541684,-110.475812025073,
174.328630652215));
#24720=CARTESIAN_POINT('Ctrl Pts',(-55.866026075768,-110.258396495795,173.157057825983));
#24721=CARTESIAN_POINT('Ctrl Pts',(-57.0210596973676,-110.040980966518,
171.985484999752));
#24722=CARTESIAN_POINT('Ctrl Pts',(-58.6586403215375,-109.772122702921,
171.985485069079));
#24723=CARTESIAN_POINT('Ctrl Pts',(-60.2962209457073,-109.503264439324,
171.985485138407));
#24724=CARTESIAN_POINT('Ctrl Pts',(-61.4512544698151,-109.28584892044,173.157058062683));
#24725=CARTESIAN_POINT('Ctrl Pts',(-62.6062879939228,-109.068433401555,
174.328630986959));
#24726=CARTESIAN_POINT('Ctrl Pts',(-62.5963498620687,-108.975211644249,
175.985485236451));
#24727=CARTESIAN_POINT('Ctrl Pts',(-62.5864117302145,-108.881989886943,
177.642339485944));
#24728=CARTESIAN_POINT('Ctrl Pts',(-61.4115019827808,-108.91296188691,178.813912312176));
#24729=CARTESIAN_POINT('Ctrl Pts',(-60.2365922353472,-108.943933886877,
179.985485138407));
#24730=CARTESIAN_POINT('Ctrl Pts',(-58.5791354853433,-109.026348621163,
179.985485069079));
#24731=CARTESIAN_POINT('Ctrl Pts',(-56.9216787353394,-109.108763355449,
179.985484999752));
#24732=CARTESIAN_POINT('Ctrl Pts',(-55.7467690853976,-109.139735345023,
178.813912075476));
#24733=CARTESIAN_POINT('Ctrl Pts',(-54.5718594354559,-109.170707334596,
177.6423391512));
#24734=CARTESIAN_POINT('Ctrl Pts',(-54.561921441476,-109.077485562592,175.985484901707));
#24735=CARTESIAN_POINT('Ctrl Pts',(-54.5519834474962,-108.984263790587,
174.328630652215));
#24736=CARTESIAN_POINT('Ctrl Pts',(-55.7070170690958,-108.76684826131,173.157057825983));
#24737=CARTESIAN_POINT('Ctrl Pts',(-56.8620506906954,-108.549432732032,
171.985484999752));
#24738=CARTESIAN_POINT('Ctrl Pts',(-58.4996313148652,-108.280574468435,
171.985485069079));
#24739=CARTESIAN_POINT('Ctrl Pts',(-60.1372119390351,-108.011716204838,
171.985485138407));
#24740=CARTESIAN_POINT('Ctrl Pts',(-61.2922454631428,-107.794300685954,
173.157058062683));
#24741=CARTESIAN_POINT('Ctrl Pts',(-62.4472789872506,-107.57688516707,174.328630986959));
#24742=CARTESIAN_POINT('Ctrl Pts',(-62.4373408553964,-107.483663409764,
175.985485236451));
#24743=CARTESIAN_POINT('Ctrl Pts',(-62.4274027235423,-107.390441652457,
177.642339485944));
#24744=CARTESIAN_POINT('Ctrl Pts',(-61.2524929761086,-107.421413652424,
178.813912312176));
#24745=CARTESIAN_POINT('Ctrl Pts',(-60.077583228675,-107.452385652391,179.985485138407));
#24746=CARTESIAN_POINT('Ctrl Pts',(-58.4201264786711,-107.534800386677,
179.985485069079));
#24747=CARTESIAN_POINT('Ctrl Pts',(-56.7626697286672,-107.617215120964,
179.985484999752));
#24748=CARTESIAN_POINT('Ctrl Pts',(-55.5877600787254,-107.648187110537,
178.813912075476));
#24749=CARTESIAN_POINT('Ctrl Pts',(-54.4128504287836,-107.67915910011,177.6423391512));
#24750=CARTESIAN_POINT('Ctrl Pts',(-54.4029124348038,-107.585937328106,
175.985484901707));
#24751=CARTESIAN_POINT('Ctrl Pts',(-54.3929744408239,-107.492715556102,
174.328630652215));
#24752=CARTESIAN_POINT('Ctrl Pts',(-55.5480080624235,-107.275300026824,
173.157057825983));
#24753=CARTESIAN_POINT('Ctrl Pts',(-56.7030416840231,-107.057884497547,
171.985484999752));
#24754=CARTESIAN_POINT('Ctrl Pts',(-58.340622308193,-106.78902623395,171.985485069079));
#24755=CARTESIAN_POINT('Ctrl Pts',(-59.9782029323629,-106.520167970353,
171.985485138407));
#24756=CARTESIAN_POINT('Ctrl Pts',(-61.1332364564706,-106.302752451468,
173.157058062683));
#24757=CARTESIAN_POINT('Ctrl Pts',(-62.2882699805784,-106.085336932584,
174.328630986959));
#24758=CARTESIAN_POINT('Ctrl Pts',(-62.2783318487242,-105.992115175278,
175.985485236451));
#24759=CARTESIAN_POINT('Ctrl Pts',(-62.26839371687,-105.898893417972,177.642339485944));
#24760=CARTESIAN_POINT('Ctrl Pts',(-61.0934839694364,-105.929865417939,
178.813912312176));
#24761=CARTESIAN_POINT('Ctrl Pts',(-59.9185742220028,-105.960837417905,
179.985485138407));
#24762=CARTESIAN_POINT('Ctrl Pts',(-58.2611174719989,-106.043252152192,
179.985485069079));
#24763=CARTESIAN_POINT('Ctrl Pts',(-56.603660721995,-106.125666886478,179.985484999752));
#24764=CARTESIAN_POINT('Ctrl Pts',(-55.4287510720532,-106.156638876051,
178.813912075476));
#24765=CARTESIAN_POINT('Ctrl Pts',(-54.2538414221114,-106.187610865625,
177.6423391512));
#24766=CARTESIAN_POINT('Ctrl Pts',(-54.2439034281315,-106.09438909362,175.985484901707));
#24767=CARTESIAN_POINT('Ctrl Pts',(-54.2339654341517,-106.001167321616,
174.328630652215));
#24768=CARTESIAN_POINT('Ctrl Pts',(-55.3889990557513,-105.783751792338,
173.157057825983));
#24769=CARTESIAN_POINT('Ctrl Pts',(-56.5440326773509,-105.566336263061,
171.985484999752));
#24770=CARTESIAN_POINT('Ctrl Pts',(-58.1816133015208,-105.297477999464,
171.985485069079));
#24771=CARTESIAN_POINT('Ctrl Pts',(-59.8191939256906,-105.028619735867,
171.985485138407));
#24772=CARTESIAN_POINT('Ctrl Pts',(-60.9742274497984,-104.811204216983,
173.157058062683));
#24773=CARTESIAN_POINT('Ctrl Pts',(-62.1292609739061,-104.593788698099,
174.328630986959));
#24774=CARTESIAN_POINT('Ctrl Pts',(-62.119322842052,-104.500566940792,175.985485236451));
#24775=CARTESIAN_POINT('Ctrl Pts',(-62.1093847101978,-104.407345183486,
177.642339485944));
#24776=CARTESIAN_POINT('Ctrl Pts',(-60.9344749627642,-104.438317183453,
178.813912312176));
#24777=CARTESIAN_POINT('Ctrl Pts',(-59.7595652153305,-104.46928918342,179.985485138407));
#24778=CARTESIAN_POINT('Ctrl Pts',(-58.1021084653266,-104.551703917706,
179.985485069079));
#24779=CARTESIAN_POINT('Ctrl Pts',(-56.4446517153227,-104.634118651992,
179.985484999752));
#24780=CARTESIAN_POINT('Ctrl Pts',(-55.269742065381,-104.665090641566,178.813912075476));
#24781=CARTESIAN_POINT('Ctrl Pts',(-54.0948324154392,-104.696062631139,
177.6423391512));
#24782=CARTESIAN_POINT('Ctrl Pts',(-54.0848944214593,-104.602840859135,
175.985484901707));
#24783=CARTESIAN_POINT('Ctrl Pts',(-54.0749564274795,-104.50961908713,174.328630652215));
#24784=CARTESIAN_POINT('Ctrl Pts',(-55.2299900490791,-104.292203557853,
173.157057825983));
#24785=CARTESIAN_POINT('Ctrl Pts',(-56.3850236706787,-104.074788028575,
171.985484999752));
#24786=CARTESIAN_POINT('Ctrl Pts',(-58.0226042948486,-103.805929764978,
171.985485069079));
#24787=CARTESIAN_POINT('Ctrl Pts',(-59.6601849190184,-103.537071501381,
171.985485138407));
#24788=CARTESIAN_POINT('Ctrl Pts',(-60.8152184431262,-103.319655982497,
173.157058062683));
#24789=CARTESIAN_POINT('Ctrl Pts',(-61.9702519672339,-103.102240463613,
174.328630986959));
#24790=CARTESIAN_POINT('Ctrl Pts',(-61.9603138353797,-103.009018706307,
175.985485236451));
#24791=CARTESIAN_POINT('Ctrl Pts',(-61.9503757035256,-102.915796949001,
177.642339485944));
#24792=CARTESIAN_POINT('Ctrl Pts',(-60.7754659560919,-102.946768948967,
178.813912312176));
#24793=CARTESIAN_POINT('Ctrl Pts',(-59.6005562086583,-102.977740948934,
179.985485138407));
#24794=CARTESIAN_POINT('Ctrl Pts',(-57.9430994586544,-103.06015568322,179.985485069079));
#24795=CARTESIAN_POINT('Ctrl Pts',(-56.2856427086505,-103.142570417507,
179.985484999752));
#24796=CARTESIAN_POINT('Ctrl Pts',(-55.1107330587087,-103.17354240708,178.813912075476));
#24797=CARTESIAN_POINT('Ctrl Pts',(-53.935823408767,-103.204514396654,177.6423391512));
#24798=CARTESIAN_POINT('Ctrl Pts',(-53.9258854147871,-103.111292624649,
175.985484901707));
#24799=CARTESIAN_POINT('Ctrl Pts',(-53.9159474208072,-103.018070852645,
174.328630652215));
#24800=CARTESIAN_POINT('Ctrl Pts',(-55.0709810424069,-102.800655323367,
173.157057825983));
#24801=CARTESIAN_POINT('Ctrl Pts',(-56.2260146640065,-102.58323979409,171.985484999752));
#24802=CARTESIAN_POINT('Ctrl Pts',(-57.8635952881763,-102.314381530493,
171.985485069079));
#24803=CARTESIAN_POINT('Ctrl Pts',(-59.5011759123462,-102.045523266896,
171.985485138407));
#24804=CARTESIAN_POINT('Ctrl Pts',(-60.6562094364539,-101.828107748012,
173.157058062683));
#24805=CARTESIAN_POINT('Ctrl Pts',(-61.8112429605617,-101.610692229127,
174.328630986959));
#24806=CARTESIAN_POINT('Ctrl Pts',(-61.8013048287075,-101.517470471821,
175.985485236451));
#24807=CARTESIAN_POINT('Ctrl Pts',(-61.7913666968533,-101.424248714515,
177.642339485944));
#24808=CARTESIAN_POINT('Ctrl Pts',(-60.6164569494197,-101.455220714482,
178.813912312176));
#24809=CARTESIAN_POINT('Ctrl Pts',(-59.4415472019861,-101.486192714449,
179.985485138407));
#24810=CARTESIAN_POINT('Ctrl Pts',(-57.7840904519822,-101.568607448735,
179.985485069079));
#24811=CARTESIAN_POINT('Ctrl Pts',(-56.1266337019783,-101.651022183021,
179.985484999752));
#24812=CARTESIAN_POINT('Ctrl Pts',(-54.9517240520365,-101.681994172595,
178.813912075476));
#24813=CARTESIAN_POINT('Ctrl Pts',(-53.7768144020947,-101.712966162168,
177.6423391512));
#24814=CARTESIAN_POINT('Ctrl Pts',(-53.7668764081149,-101.619744390164,
175.985484901707));
#24815=CARTESIAN_POINT('Ctrl Pts',(-53.756938414135,-101.526522618159,174.328630652215));
#24816=CARTESIAN_POINT('Ctrl Pts',(-54.9119720357346,-101.309107088882,
173.157057825983));
#24817=CARTESIAN_POINT('Ctrl Pts',(-56.0670056573342,-101.091691559604,
171.985484999752));
#24818=CARTESIAN_POINT('Ctrl Pts',(-57.7045862815041,-100.822833296007,
171.985485069079));
#24819=CARTESIAN_POINT('Ctrl Pts',(-59.342166905674,-100.55397503241,171.985485138407));
#24820=CARTESIAN_POINT('Ctrl Pts',(-60.4972004297817,-100.336559513526,
173.157058062683));
#24821=CARTESIAN_POINT('Ctrl Pts',(-61.6522339538895,-100.119143994642,
174.328630986959));
#24822=CARTESIAN_POINT('Ctrl Pts',(-61.6422958220353,-100.025922237336,
175.985485236451));
#24823=CARTESIAN_POINT('Ctrl Pts',(-61.6323576901811,-99.9327004800294,
177.642339485944));
#24824=CARTESIAN_POINT('Ctrl Pts',(-60.4574479427475,-99.9636724799962,
178.813912312176));
#24825=CARTESIAN_POINT('Ctrl Pts',(-59.2825381953138,-99.994644479963,179.985485138407));
#24826=CARTESIAN_POINT('Ctrl Pts',(-57.6250814453099,-100.077059214249,
179.985485069079));
#24827=CARTESIAN_POINT('Ctrl Pts',(-55.9676246953061,-100.159473948536,
179.985484999752));
#24828=CARTESIAN_POINT('Ctrl Pts',(-54.7927150453643,-100.190445938109,
178.813912075476));
#24829=CARTESIAN_POINT('Ctrl Pts',(-53.6178053954225,-100.221417927683,
177.6423391512));
#24830=CARTESIAN_POINT('Ctrl Pts',(-53.6078674014426,-100.128196155678,
175.985484901707));
#24831=CARTESIAN_POINT('Ctrl Pts',(-53.5979294074628,-100.034974383673,
174.328630652215));
#24832=CARTESIAN_POINT('Ctrl Pts',(-54.7529630290624,-99.817558854396,173.157057825983));
#24833=CARTESIAN_POINT('Ctrl Pts',(-55.907996650662,-99.6001433251185,171.985484999752));
#24834=CARTESIAN_POINT('Ctrl Pts',(-57.5455772748319,-99.3312850615215,
171.985485069079));
#24835=CARTESIAN_POINT('Ctrl Pts',(-59.1831578990017,-99.0624267979246,
171.985485138407));
#24836=CARTESIAN_POINT('Ctrl Pts',(-60.3381914231095,-98.8450112790404,
173.157058062683));
#24837=CARTESIAN_POINT('Ctrl Pts',(-61.4932249472172,-98.6275957601562,
174.328630986959));
#24838=CARTESIAN_POINT('Ctrl Pts',(-61.4832868153631,-98.53437400285,175.985485236451));
#24839=CARTESIAN_POINT('Ctrl Pts',(-61.4733486835089,-98.4411522455438,
177.642339485944));
#24840=CARTESIAN_POINT('Ctrl Pts',(-60.2984389360752,-98.4721242455106,
178.813912312176));
#24841=CARTESIAN_POINT('Ctrl Pts',(-59.1235291886416,-98.5030962454774,
179.985485138407));
#24842=CARTESIAN_POINT('Ctrl Pts',(-57.4660724386377,-98.5855109797636,
179.985485069079));
#24843=CARTESIAN_POINT('Ctrl Pts',(-55.8086156886338,-98.6679257140499,
179.985484999752));
#24844=CARTESIAN_POINT('Ctrl Pts',(-54.633706038692,-98.6988977036234,178.813912075476));
#24845=CARTESIAN_POINT('Ctrl Pts',(-56.9964983346804,-113.864655531781,
178.072094410988));
#24846=CARTESIAN_POINT('Ctrl Pts',(-56.1271283009022,-113.863054956993,
177.207792449865));
#24847=CARTESIAN_POINT('Ctrl Pts',(-56.117190288842,-113.769833186916,175.985484945604));
#24848=CARTESIAN_POINT('Ctrl Pts',(-56.1072522767819,-113.676611416839,
174.763177441344));
#24849=CARTESIAN_POINT('Ctrl Pts',(-56.9567462566485,-113.491768454648,
173.89887555255));
#24850=CARTESIAN_POINT('Ctrl Pts',(-57.8062402365152,-113.306925492458,
173.034573663757));
#24851=CARTESIAN_POINT('Ctrl Pts',(-59.011722573584,-113.084131793069,173.034573714903));
#24852=CARTESIAN_POINT('Ctrl Pts',(-60.2172049106529,-112.86133809368,173.034573766048));
#24853=CARTESIAN_POINT('Ctrl Pts',(-61.0666988185971,-112.676495139156,
173.898875727171));
#24854=CARTESIAN_POINT('Ctrl Pts',(-61.9161927265413,-112.491652184633,
174.763177688294));
#24855=CARTESIAN_POINT('Ctrl Pts',(-61.9062546127674,-112.398430425399,
175.985485192554));
#24856=CARTESIAN_POINT('Ctrl Pts',(-61.8963164989935,-112.305208666166,
177.207792696815));
#24857=CARTESIAN_POINT('Ctrl Pts',(-61.0269463932928,-112.303608099046,
178.072094585608));
#24858=CARTESIAN_POINT('Ctrl Pts',(-60.1575762875921,-112.302007531926,
178.936396474401));
#24859=CARTESIAN_POINT('Ctrl Pts',(-58.9322178246893,-112.338357702004,
178.936396423256));
#24860=CARTESIAN_POINT('Ctrl Pts',(-57.7068593617864,-112.374707872082,
178.936396372111));
#24861=CARTESIAN_POINT('Ctrl Pts',(-56.8374893280082,-112.373107297295,
178.072094410988));
#24862=CARTESIAN_POINT('Ctrl Pts',(-55.9681192942299,-112.371506722508,
177.207792449865));
#24863=CARTESIAN_POINT('Ctrl Pts',(-55.9581812821698,-112.278284952431,
175.985484945604));
#24864=CARTESIAN_POINT('Ctrl Pts',(-55.9482432701096,-112.185063182354,
174.763177441344));
#24865=CARTESIAN_POINT('Ctrl Pts',(-56.7977372499763,-112.000220220163,
173.89887555255));
#24866=CARTESIAN_POINT('Ctrl Pts',(-57.647231229843,-111.815377257972,173.034573663757));
#24867=CARTESIAN_POINT('Ctrl Pts',(-58.8527135669118,-111.592583558583,
173.034573714903));
#24868=CARTESIAN_POINT('Ctrl Pts',(-60.0581959039807,-111.369789859194,
173.034573766048));
#24869=CARTESIAN_POINT('Ctrl Pts',(-60.9076898119249,-111.184946904671,
173.898875727171));
#24870=CARTESIAN_POINT('Ctrl Pts',(-61.7571837198691,-111.000103950148,
174.763177688294));
#24871=CARTESIAN_POINT('Ctrl Pts',(-61.7472456060952,-110.906882190914,
175.985485192554));
#24872=CARTESIAN_POINT('Ctrl Pts',(-61.7373074923213,-110.81366043168,177.207792696815));
#24873=CARTESIAN_POINT('Ctrl Pts',(-60.8679373866206,-110.81205986456,178.072094585608));
#24874=CARTESIAN_POINT('Ctrl Pts',(-59.9985672809199,-110.81045929744,178.936396474401));
#24875=CARTESIAN_POINT('Ctrl Pts',(-58.7732088180171,-110.846809467519,
178.936396423256));
#24876=CARTESIAN_POINT('Ctrl Pts',(-57.5478503551142,-110.883159637597,
178.936396372111));
#24877=CARTESIAN_POINT('Ctrl Pts',(-56.6784803213359,-110.881559062809,
178.072094410988));
#24878=CARTESIAN_POINT('Ctrl Pts',(-55.8091102875577,-110.879958488022,
177.207792449865));
#24879=CARTESIAN_POINT('Ctrl Pts',(-55.7991722754976,-110.786736717945,
175.985484945604));
#24880=CARTESIAN_POINT('Ctrl Pts',(-55.7892342634374,-110.693514947868,
174.763177441344));
#24881=CARTESIAN_POINT('Ctrl Pts',(-56.6387282433041,-110.508671985677,
173.89887555255));
#24882=CARTESIAN_POINT('Ctrl Pts',(-57.4882222231708,-110.323829023487,
173.034573663757));
#24883=CARTESIAN_POINT('Ctrl Pts',(-58.6937045602396,-110.101035324098,
173.034573714903));
#24884=CARTESIAN_POINT('Ctrl Pts',(-59.8991868973084,-109.878241624709,
173.034573766048));
#24885=CARTESIAN_POINT('Ctrl Pts',(-60.7486808052526,-109.693398670185,
173.898875727171));
#24886=CARTESIAN_POINT('Ctrl Pts',(-61.5981747131968,-109.508555715662,
174.763177688294));
#24887=CARTESIAN_POINT('Ctrl Pts',(-61.588236599423,-109.415333956428,175.985485192554));
#24888=CARTESIAN_POINT('Ctrl Pts',(-61.5782984856491,-109.322112197195,
177.207792696815));
#24889=CARTESIAN_POINT('Ctrl Pts',(-60.7089283799484,-109.320511630075,
178.072094585608));
#24890=CARTESIAN_POINT('Ctrl Pts',(-59.8395582742477,-109.318911062955,
178.936396474401));
#24891=CARTESIAN_POINT('Ctrl Pts',(-58.6141998113448,-109.355261233033,
178.936396423256));
#24892=CARTESIAN_POINT('Ctrl Pts',(-57.388841348442,-109.391611403111,178.936396372111));
#24893=CARTESIAN_POINT('Ctrl Pts',(-56.5194713146637,-109.390010828324,
178.072094410988));
#24894=CARTESIAN_POINT('Ctrl Pts',(-55.6501012808855,-109.388410253536,
177.207792449865));
#24895=CARTESIAN_POINT('Ctrl Pts',(-55.6401632688253,-109.295188483459,
175.985484945604));
#24896=CARTESIAN_POINT('Ctrl Pts',(-55.6302252567652,-109.201966713382,
174.763177441344));
#24897=CARTESIAN_POINT('Ctrl Pts',(-56.4797192366319,-109.017123751192,
173.89887555255));
#24898=CARTESIAN_POINT('Ctrl Pts',(-57.3292132164985,-108.832280789001,
173.034573663757));
#24899=CARTESIAN_POINT('Ctrl Pts',(-58.5346955535674,-108.609487089612,
173.034573714903));
#24900=CARTESIAN_POINT('Ctrl Pts',(-59.7401778906362,-108.386693390223,
173.034573766048));
#24901=CARTESIAN_POINT('Ctrl Pts',(-60.5896717985804,-108.2018504357,173.898875727171));
#24902=CARTESIAN_POINT('Ctrl Pts',(-61.4391657065246,-108.017007481176,
174.763177688294));
#24903=CARTESIAN_POINT('Ctrl Pts',(-61.4292275927507,-107.923785721943,
175.985485192554));
#24904=CARTESIAN_POINT('Ctrl Pts',(-61.4192894789769,-107.830563962709,
177.207792696815));
#24905=CARTESIAN_POINT('Ctrl Pts',(-60.5499193732762,-107.828963395589,
178.072094585608));
#24906=CARTESIAN_POINT('Ctrl Pts',(-59.6805492675755,-107.827362828469,
178.936396474401));
#24907=CARTESIAN_POINT('Ctrl Pts',(-58.4551908046726,-107.863712998547,
178.936396423256));
#24908=CARTESIAN_POINT('Ctrl Pts',(-57.2298323417698,-107.900063168626,
178.936396372111));
#24909=CARTESIAN_POINT('Ctrl Pts',(-56.3604623079915,-107.898462593838,
178.072094410988));
#24910=CARTESIAN_POINT('Ctrl Pts',(-55.4910922742133,-107.896862019051,
177.207792449865));
#24911=CARTESIAN_POINT('Ctrl Pts',(-55.4811542621531,-107.803640248974,
175.985484945604));
#24912=CARTESIAN_POINT('Ctrl Pts',(-55.471216250093,-107.710418478897,174.763177441344));
#24913=CARTESIAN_POINT('Ctrl Pts',(-56.3207102299596,-107.525575516706,
173.89887555255));
#24914=CARTESIAN_POINT('Ctrl Pts',(-57.1702042098263,-107.340732554515,
173.034573663757));
#24915=CARTESIAN_POINT('Ctrl Pts',(-58.3756865468951,-107.117938855126,
173.034573714903));
#24916=CARTESIAN_POINT('Ctrl Pts',(-59.581168883964,-106.895145155737,173.034573766048));
#24917=CARTESIAN_POINT('Ctrl Pts',(-60.4306627919082,-106.710302201214,
173.898875727171));
#24918=CARTESIAN_POINT('Ctrl Pts',(-61.2801566998524,-106.525459246691,
174.763177688294));
#24919=CARTESIAN_POINT('Ctrl Pts',(-61.2702185860785,-106.432237487457,
175.985485192554));
#24920=CARTESIAN_POINT('Ctrl Pts',(-61.2602804723046,-106.339015728223,
177.207792696815));
#24921=CARTESIAN_POINT('Ctrl Pts',(-60.3909103666039,-106.337415161103,
178.072094585608));
#24922=CARTESIAN_POINT('Ctrl Pts',(-59.5215402609032,-106.335814593983,
178.936396474401));
#24923=CARTESIAN_POINT('Ctrl Pts',(-58.2961817980004,-106.372164764062,
178.936396423256));
#24924=CARTESIAN_POINT('Ctrl Pts',(-57.0708233350975,-106.40851493414,178.936396372111));
#24925=CARTESIAN_POINT('Ctrl Pts',(-56.2014533013193,-106.406914359353,
178.072094410988));
#24926=CARTESIAN_POINT('Ctrl Pts',(-55.332083267541,-106.405313784565,177.207792449865));
#24927=CARTESIAN_POINT('Ctrl Pts',(-55.3221452554809,-106.312092014488,
175.985484945604));
#24928=CARTESIAN_POINT('Ctrl Pts',(-55.3122072434207,-106.218870244411,
174.763177441344));
#24929=CARTESIAN_POINT('Ctrl Pts',(-56.1617012232874,-106.034027282221,
173.89887555255));
#24930=CARTESIAN_POINT('Ctrl Pts',(-57.0111952031541,-105.84918432003,173.034573663757));
#24931=CARTESIAN_POINT('Ctrl Pts',(-58.2166775402229,-105.626390620641,
173.034573714903));
#24932=CARTESIAN_POINT('Ctrl Pts',(-59.4221598772917,-105.403596921252,
173.034573766048));
#24933=CARTESIAN_POINT('Ctrl Pts',(-60.2716537852359,-105.218753966728,
173.898875727171));
#24934=CARTESIAN_POINT('Ctrl Pts',(-61.1211476931802,-105.033911012205,
174.763177688294));
#24935=CARTESIAN_POINT('Ctrl Pts',(-61.1112095794063,-104.940689252971,
175.985485192554));
#24936=CARTESIAN_POINT('Ctrl Pts',(-61.1012714656324,-104.847467493738,
177.207792696815));
#24937=CARTESIAN_POINT('Ctrl Pts',(-60.2319013599317,-104.845866926618,
178.072094585608));
#24938=CARTESIAN_POINT('Ctrl Pts',(-59.362531254231,-104.844266359498,178.936396474401));
#24939=CARTESIAN_POINT('Ctrl Pts',(-58.1371727913281,-104.880616529576,
178.936396423256));
#24940=CARTESIAN_POINT('Ctrl Pts',(-56.9118143284253,-104.916966699654,
178.936396372111));
#24941=CARTESIAN_POINT('Ctrl Pts',(-56.042444294647,-104.915366124867,178.072094410988));
#24942=CARTESIAN_POINT('Ctrl Pts',(-55.1730742608688,-104.91376555008,177.207792449865));
#24943=CARTESIAN_POINT('Ctrl Pts',(-55.1631362488087,-104.820543780003,
175.985484945604));
#24944=CARTESIAN_POINT('Ctrl Pts',(-55.1531982367485,-104.727322009926,
174.763177441344));
#24945=CARTESIAN_POINT('Ctrl Pts',(-56.0026922166152,-104.542479047735,
173.89887555255));
#24946=CARTESIAN_POINT('Ctrl Pts',(-56.8521861964818,-104.357636085544,
173.034573663757));
#24947=CARTESIAN_POINT('Ctrl Pts',(-58.0576685335507,-104.134842386155,
173.034573714903));
#24948=CARTESIAN_POINT('Ctrl Pts',(-59.2631508706195,-103.912048686766,
173.034573766048));
#24949=CARTESIAN_POINT('Ctrl Pts',(-60.1126447785637,-103.727205732243,
173.898875727171));
#24950=CARTESIAN_POINT('Ctrl Pts',(-60.9621386865079,-103.54236277772,174.763177688294));
#24951=CARTESIAN_POINT('Ctrl Pts',(-60.952200572734,-103.449141018486,175.985485192554));
#24952=CARTESIAN_POINT('Ctrl Pts',(-60.9422624589602,-103.355919259252,
177.207792696815));
#24953=CARTESIAN_POINT('Ctrl Pts',(-60.0728923532595,-103.354318692132,
178.072094585608));
#24954=CARTESIAN_POINT('Ctrl Pts',(-59.2035222475588,-103.352718125012,
178.936396474401));
#24955=CARTESIAN_POINT('Ctrl Pts',(-57.9781637846559,-103.389068295091,
178.936396423256));
#24956=CARTESIAN_POINT('Ctrl Pts',(-56.7528053217531,-103.425418465169,
178.936396372111));
#24957=CARTESIAN_POINT('Ctrl Pts',(-55.8834352879748,-103.423817890381,
178.072094410988));
#24958=CARTESIAN_POINT('Ctrl Pts',(-55.0140652541966,-103.422217315594,
177.207792449865));
#24959=CARTESIAN_POINT('Ctrl Pts',(-55.0041272421364,-103.328995545517,
175.985484945604));
#24960=CARTESIAN_POINT('Ctrl Pts',(-54.9941892300763,-103.23577377544,174.763177441344));
#24961=CARTESIAN_POINT('Ctrl Pts',(-55.8436832099429,-103.050930813249,
173.89887555255));
#24962=CARTESIAN_POINT('Ctrl Pts',(-56.6931771898096,-102.866087851059,
173.034573663757));
#24963=CARTESIAN_POINT('Ctrl Pts',(-57.8986595268784,-102.64329415167,173.034573714903));
#24964=CARTESIAN_POINT('Ctrl Pts',(-59.1041418639473,-102.420500452281,
173.034573766048));
#24965=CARTESIAN_POINT('Ctrl Pts',(-59.9536357718915,-102.235657497757,
173.898875727171));
#24966=CARTESIAN_POINT('Ctrl Pts',(-60.8031296798357,-102.050814543234,
174.763177688294));
#24967=CARTESIAN_POINT('Ctrl Pts',(-60.7931915660618,-101.957592784,175.985485192554));
#24968=CARTESIAN_POINT('Ctrl Pts',(-60.783253452288,-101.864371024767,177.207792696815));
#24969=CARTESIAN_POINT('Ctrl Pts',(-59.9138833465873,-101.862770457647,
178.072094585608));
#24970=CARTESIAN_POINT('Ctrl Pts',(-59.0445132408866,-101.861169890527,
178.936396474401));
#24971=CARTESIAN_POINT('Ctrl Pts',(-57.8191547779837,-101.897520060605,
178.936396423256));
#24972=CARTESIAN_POINT('Ctrl Pts',(-56.5937963150808,-101.933870230683,
178.936396372111));
#24973=CARTESIAN_POINT('Ctrl Pts',(-55.7244262813026,-101.932269655896,
178.072094410988));
#24974=CARTESIAN_POINT('Ctrl Pts',(-54.8550562475244,-101.930669081108,
177.207792449865));
#24975=CARTESIAN_POINT('Ctrl Pts',(-54.8451182354642,-101.837447311031,
175.985484945604));
#24976=CARTESIAN_POINT('Ctrl Pts',(-54.8351802234041,-101.744225540954,
174.763177441344));
#24977=CARTESIAN_POINT('Ctrl Pts',(-55.6846742032707,-101.559382578764,
173.89887555255));
#24978=CARTESIAN_POINT('Ctrl Pts',(-56.5341681831374,-101.374539616573,
173.034573663757));
#24979=CARTESIAN_POINT('Ctrl Pts',(-57.7396505202062,-101.151745917184,
173.034573714903));
#24980=CARTESIAN_POINT('Ctrl Pts',(-58.9451328572751,-100.928952217795,
173.034573766048));
#24981=CARTESIAN_POINT('Ctrl Pts',(-59.7946267652193,-100.744109263272,
173.898875727171));
#24982=CARTESIAN_POINT('Ctrl Pts',(-60.6441206731635,-100.559266308748,
174.763177688294));
#24983=CARTESIAN_POINT('Ctrl Pts',(-60.6341825593896,-100.466044549515,
175.985485192554));
#24984=CARTESIAN_POINT('Ctrl Pts',(-60.6242444456157,-100.372822790281,
177.207792696815));
#24985=CARTESIAN_POINT('Ctrl Pts',(-59.754874339915,-100.371222223161,178.072094585608));
#24986=CARTESIAN_POINT('Ctrl Pts',(-58.8855042342143,-100.369621656041,
178.936396474401));
#24987=CARTESIAN_POINT('Ctrl Pts',(-57.6601457713115,-100.405971826119,
178.936396423256));
#24988=CARTESIAN_POINT('Ctrl Pts',(-56.4347873084086,-100.442321996198,
178.936396372111));
#24989=CARTESIAN_POINT('Ctrl Pts',(-55.5654172746304,-100.44072142141,178.072094410988));
#24990=CARTESIAN_POINT('Ctrl Pts',(-54.6960472408521,-100.439120846623,
177.207792449865));
#24991=CARTESIAN_POINT('Ctrl Pts',(-54.686109228792,-100.345899076546,175.985484945604));
#24992=CARTESIAN_POINT('Ctrl Pts',(-54.6761712167318,-100.252677306469,
174.763177441344));
#24993=CARTESIAN_POINT('Ctrl Pts',(-55.5256651965985,-100.067834344278,
173.89887555255));
#24994=CARTESIAN_POINT('Ctrl Pts',(-56.3751591764652,-99.8829913820874,
173.034573663757));
#24995=CARTESIAN_POINT('Ctrl Pts',(-57.580641513534,-99.6601976826983,173.034573714903));
#24996=CARTESIAN_POINT('Ctrl Pts',(-58.7861238506028,-99.4374039833093,
173.034573766048));
#24997=CARTESIAN_POINT('Ctrl Pts',(-59.635617758547,-99.252561028786,173.898875727171));
#24998=CARTESIAN_POINT('Ctrl Pts',(-60.4851116664912,-99.0677180742627,
174.763177688294));
#24999=CARTESIAN_POINT('Ctrl Pts',(-60.4751735527174,-98.9744963150291,
175.985485192554));
#25000=CARTESIAN_POINT('Ctrl Pts',(-60.4652354389435,-98.8812745557954,
177.207792696815));
#25001=CARTESIAN_POINT('Ctrl Pts',(-59.5958653332428,-98.8796739886754,
178.072094585608));
#25002=CARTESIAN_POINT('Ctrl Pts',(-58.7264952275421,-98.8780734215554,
178.936396474401));
#25003=CARTESIAN_POINT('Ctrl Pts',(-57.5011367646392,-98.9144235916337,
178.936396423256));
#25004=CARTESIAN_POINT('Ctrl Pts',(-56.2757783017364,-98.9507737617121,
178.936396372111));
#25005=CARTESIAN_POINT('Ctrl Pts',(-55.4064082679581,-98.9491731869247,
178.072094410988));
#25006=CARTESIAN_POINT('Ctrl Pts',(-61.8656266134859,-110.398668935236,
178.485485069079));
#25007=CARTESIAN_POINT('Ctrl Pts',(-61.7270544091292,-110.400383453113,
178.657813499464));
#25008=CARTESIAN_POINT('Ctrl Pts',(-61.5705109894531,-110.404510121395,
178.813912312176));
#25009=CARTESIAN_POINT('Ctrl Pts',(-60.3956012420194,-110.435482121362,
179.985485138407));
#25010=CARTESIAN_POINT('Ctrl Pts',(-58.7381444920155,-110.517896855648,
179.985485069079));
#25011=CARTESIAN_POINT('Ctrl Pts',(-57.0806877420117,-110.600311589935,
179.985484999752));
#25012=CARTESIAN_POINT('Ctrl Pts',(-55.9057780920699,-110.631283579508,
178.813912075476));
#25013=CARTESIAN_POINT('Ctrl Pts',(-54.7308684421281,-110.662255569082,
177.6423391512));
#25014=CARTESIAN_POINT('Ctrl Pts',(-54.7209304481482,-110.569033797077,
175.985484901707));
#25015=CARTESIAN_POINT('Ctrl Pts',(-54.7109924541684,-110.475812025073,
174.328630652215));
#25016=CARTESIAN_POINT('Ctrl Pts',(-55.866026075768,-110.258396495795,173.157057825983));
#25017=CARTESIAN_POINT('Ctrl Pts',(-57.0210596973676,-110.040980966518,
171.985484999752));
#25018=CARTESIAN_POINT('Ctrl Pts',(-58.6586403215375,-109.772122702921,
171.985485069079));
#25019=CARTESIAN_POINT('Ctrl Pts',(-60.2962209457073,-109.503264439324,
171.985485138407));
#25020=CARTESIAN_POINT('Ctrl Pts',(-61.4512544698151,-109.28584892044,173.157058062683));
#25021=CARTESIAN_POINT('Ctrl Pts',(-61.6051494907682,-109.256880786497,
173.313156769748));
#25022=CARTESIAN_POINT('Ctrl Pts',(-61.740968694739,-109.229343357315,173.485485069079));
#25023=CARTESIAN_POINT('Ctrl Pts',(-56.8733667677527,-112.709647553905,
178.072094410988));
#25024=CARTESIAN_POINT('Ctrl Pts',(-56.0039967339745,-112.708046979118,
177.207792449865));
#25025=CARTESIAN_POINT('Ctrl Pts',(-55.9940587219143,-112.614825209041,
175.985484945604));
#25026=CARTESIAN_POINT('Ctrl Pts',(-55.9841207098542,-112.521603438964,
174.763177441344));
#25027=CARTESIAN_POINT('Ctrl Pts',(-56.8336146897208,-112.336760476773,
173.89887555255));
#25028=CARTESIAN_POINT('Ctrl Pts',(-57.6831086695875,-112.151917514582,
173.034573663757));
#25029=CARTESIAN_POINT('Ctrl Pts',(-58.8885910066563,-111.929123815193,
173.034573714903));
#25030=CARTESIAN_POINT('Ctrl Pts',(-60.0940733437252,-111.706330115804,
173.034573766048));
#25031=CARTESIAN_POINT('Ctrl Pts',(-60.9435672516694,-111.521487161281,
173.898875727171));
#25032=CARTESIAN_POINT('Ctrl Pts',(-61.7930611596136,-111.336644206758,
174.763177688294));
#25033=CARTESIAN_POINT('Ctrl Pts',(-61.7831230458397,-111.243422447524,
175.985485192554));
#25034=CARTESIAN_POINT('Ctrl Pts',(-61.7731849320658,-111.15020068829,177.207792696815));
#25035=CARTESIAN_POINT('Ctrl Pts',(-60.9038148263651,-111.14860012117,178.072094585608));
#25036=CARTESIAN_POINT('Ctrl Pts',(-60.0344447206644,-111.14699955405,178.936396474401));
#25037=CARTESIAN_POINT('Ctrl Pts',(-58.8090862577616,-111.183349724129,
178.936396423256));
#25038=CARTESIAN_POINT('Ctrl Pts',(-57.5837277948587,-111.219699894207,
178.936396372111));
#25039=CARTESIAN_POINT('Ctrl Pts',(-56.7143577610805,-111.21809931942,178.072094410988));
#25040=CARTESIAN_POINT('Ctrl Pts',(-55.8449877273022,-111.216498744632,
177.207792449865));
#25041=CARTESIAN_POINT('Ctrl Pts',(-55.8350497152421,-111.123276974555,
175.985484945604));
#25042=CARTESIAN_POINT('Ctrl Pts',(-55.8251117031819,-111.030055204478,
174.763177441344));
#25043=CARTESIAN_POINT('Ctrl Pts',(-56.6746056830486,-110.845212242287,
173.89887555255));
#25044=CARTESIAN_POINT('Ctrl Pts',(-57.5240996629153,-110.660369280097,
173.034573663757));
#25045=CARTESIAN_POINT('Ctrl Pts',(-58.7295819999841,-110.437575580708,
173.034573714903));
#25046=CARTESIAN_POINT('Ctrl Pts',(-59.9350643370529,-110.214781881319,
173.034573766048));
#25047=CARTESIAN_POINT('Ctrl Pts',(-60.7845582449971,-110.029938926795,
173.898875727171));
#25048=CARTESIAN_POINT('Ctrl Pts',(-61.6340521529414,-109.845095972272,
174.763177688294));
#25049=CARTESIAN_POINT('Ctrl Pts',(-61.6241140391675,-109.751874213038,
175.985485192554));
#25050=CARTESIAN_POINT('Ctrl Pts',(-61.6141759253936,-109.658652453805,
177.207792696815));
#25051=CARTESIAN_POINT('Ctrl Pts',(-60.7448058196929,-109.657051886685,
178.072094585608));
#25052=CARTESIAN_POINT('Ctrl Pts',(-59.8754357139922,-109.655451319565,
178.936396474401));
#25053=CARTESIAN_POINT('Ctrl Pts',(-58.6500772510893,-109.691801489643,
178.936396423256));
#25054=CARTESIAN_POINT('Ctrl Pts',(-57.4247187881865,-109.728151659721,
178.936396372111));
#25055=CARTESIAN_POINT('Ctrl Pts',(-56.5553487544082,-109.726551084934,
178.072094410988));
#25056=CARTESIAN_POINT('Ctrl Pts',(-55.68597872063,-109.724950510147,177.207792449865));
#25057=CARTESIAN_POINT('Ctrl Pts',(-55.6760407085698,-109.63172874007,175.985484945604));
#25058=CARTESIAN_POINT('Ctrl Pts',(-55.6661026965097,-109.538506969993,
174.763177441344));
#25059=CARTESIAN_POINT('Ctrl Pts',(-56.5155966763764,-109.353664007802,
173.89887555255));
#25060=CARTESIAN_POINT('Ctrl Pts',(-57.365090656243,-109.168821045611,173.034573663757));
#25061=CARTESIAN_POINT('Ctrl Pts',(-58.5705729933119,-108.946027346222,
173.034573714903));
#25062=CARTESIAN_POINT('Ctrl Pts',(-59.7760553303807,-108.723233646833,
173.034573766048));
#25063=CARTESIAN_POINT('Ctrl Pts',(-60.6255492383249,-108.53839069231,173.898875727171));
#25064=CARTESIAN_POINT('Ctrl Pts',(-61.4750431462691,-108.353547737786,
174.763177688294));
#25065=CARTESIAN_POINT('Ctrl Pts',(-61.4651050324952,-108.260325978553,
175.985485192554));
#25066=CARTESIAN_POINT('Ctrl Pts',(-61.4551669187214,-108.167104219319,
177.207792696815));
#25067=CARTESIAN_POINT('Ctrl Pts',(-60.5857968130207,-108.165503652199,
178.072094585608));
#25068=CARTESIAN_POINT('Ctrl Pts',(-59.71642670732,-108.163903085079,178.936396474401));
#25069=CARTESIAN_POINT('Ctrl Pts',(-58.4910682444171,-108.200253255158,
178.936396423256));
#25070=CARTESIAN_POINT('Ctrl Pts',(-57.2657097815143,-108.236603425236,
178.936396372111));
#25071=CARTESIAN_POINT('Ctrl Pts',(-56.396339747736,-108.235002850448,178.072094410988));
#25072=CARTESIAN_POINT('Ctrl Pts',(-55.5269697139578,-108.233402275661,
177.207792449865));
#25073=CARTESIAN_POINT('Ctrl Pts',(-55.5170317018976,-108.140180505584,
175.985484945604));
#25074=CARTESIAN_POINT('Ctrl Pts',(-55.5070936898375,-108.046958735507,
174.763177441344));
#25075=CARTESIAN_POINT('Ctrl Pts',(-56.3565876697041,-107.862115773316,
173.89887555255));
#25076=CARTESIAN_POINT('Ctrl Pts',(-57.2060816495708,-107.677272811126,
173.034573663757));
#25077=CARTESIAN_POINT('Ctrl Pts',(-58.4115639866396,-107.454479111736,
173.034573714903));
#25078=CARTESIAN_POINT('Ctrl Pts',(-59.6170463237085,-107.231685412347,
173.034573766048));
#25079=CARTESIAN_POINT('Ctrl Pts',(-60.4665402316527,-107.046842457824,
173.898875727171));
#25080=CARTESIAN_POINT('Ctrl Pts',(-61.3160341395969,-106.861999503301,
174.763177688294));
#25081=CARTESIAN_POINT('Ctrl Pts',(-61.306096025823,-106.768777744067,175.985485192554));
#25082=CARTESIAN_POINT('Ctrl Pts',(-61.2961579120492,-106.675555984834,
177.207792696815));
#25083=CARTESIAN_POINT('Ctrl Pts',(-60.4267878063484,-106.673955417714,
178.072094585608));
#25084=CARTESIAN_POINT('Ctrl Pts',(-59.5574177006478,-106.672354850594,
178.936396474401));
#25085=CARTESIAN_POINT('Ctrl Pts',(-58.3320592377449,-106.708705020672,
178.936396423256));
#25086=CARTESIAN_POINT('Ctrl Pts',(-57.106700774842,-106.74505519075,178.936396372111));
#25087=CARTESIAN_POINT('Ctrl Pts',(-56.2373307410638,-106.743454615963,
178.072094410988));
#25088=CARTESIAN_POINT('Ctrl Pts',(-55.3679607072856,-106.741854041175,
177.207792449865));
#25089=CARTESIAN_POINT('Ctrl Pts',(-55.3580226952254,-106.648632271098,
175.985484945604));
#25090=CARTESIAN_POINT('Ctrl Pts',(-55.3480846831652,-106.555410501021,
174.763177441344));
#25091=CARTESIAN_POINT('Ctrl Pts',(-56.1975786630319,-106.370567538831,
173.89887555255));
#25092=CARTESIAN_POINT('Ctrl Pts',(-57.0470726428986,-106.18572457664,173.034573663757));
#25093=CARTESIAN_POINT('Ctrl Pts',(-58.2525549799674,-105.962930877251,
173.034573714903));
#25094=CARTESIAN_POINT('Ctrl Pts',(-59.4580373170363,-105.740137177862,
173.034573766048));
#25095=CARTESIAN_POINT('Ctrl Pts',(-60.3075312249805,-105.555294223339,
173.898875727171));
#25096=CARTESIAN_POINT('Ctrl Pts',(-61.1570251329247,-105.370451268815,
174.763177688294));
#25097=CARTESIAN_POINT('Ctrl Pts',(-61.1470870191508,-105.277229509582,
175.985485192554));
#25098=CARTESIAN_POINT('Ctrl Pts',(-61.1371489053769,-105.184007750348,
177.207792696815));
#25099=CARTESIAN_POINT('Ctrl Pts',(-60.2677787996762,-105.182407183228,
178.072094585608));
#25100=CARTESIAN_POINT('Ctrl Pts',(-59.3984086939755,-105.180806616108,
178.936396474401));
#25101=CARTESIAN_POINT('Ctrl Pts',(-58.1730502310727,-105.217156786186,
178.936396423256));
#25102=CARTESIAN_POINT('Ctrl Pts',(-56.9476917681698,-105.253506956265,
178.936396372111));
#25103=CARTESIAN_POINT('Ctrl Pts',(-56.0783217343916,-105.251906381477,
178.072094410988));
#25104=CARTESIAN_POINT('Ctrl Pts',(-55.2089517006133,-105.25030580669,177.207792449865));
#25105=CARTESIAN_POINT('Ctrl Pts',(-55.1990136885532,-105.157084036613,
175.985484945604));
#25106=CARTESIAN_POINT('Ctrl Pts',(-55.189075676493,-105.063862266536,174.763177441344));
#25107=CARTESIAN_POINT('Ctrl Pts',(-56.0385696563597,-104.879019304345,
173.89887555255));
#25108=CARTESIAN_POINT('Ctrl Pts',(-56.8880636362264,-104.694176342154,
173.034573663757));
#25109=CARTESIAN_POINT('Ctrl Pts',(-58.0935459732952,-104.471382642765,
173.034573714903));
#25110=CARTESIAN_POINT('Ctrl Pts',(-59.299028310364,-104.248588943376,173.034573766048));
#25111=CARTESIAN_POINT('Ctrl Pts',(-60.1485222183082,-104.063745988853,
173.898875727171));
#25112=CARTESIAN_POINT('Ctrl Pts',(-60.9980161262524,-103.87890303433,174.763177688294));
#25113=CARTESIAN_POINT('Ctrl Pts',(-60.9880780124786,-103.785681275096,
175.985485192554));
#25114=CARTESIAN_POINT('Ctrl Pts',(-60.9781398987047,-103.692459515862,
177.207792696815));
#25115=CARTESIAN_POINT('Ctrl Pts',(-60.108769793004,-103.690858948742,178.072094585608));
#25116=CARTESIAN_POINT('Ctrl Pts',(-59.2393996873033,-103.689258381622,
178.936396474401));
#25117=CARTESIAN_POINT('Ctrl Pts',(-58.0140412244004,-103.725608551701,
178.936396423256));
#25118=CARTESIAN_POINT('Ctrl Pts',(-56.7886827614976,-103.761958721779,
178.936396372111));
#25119=CARTESIAN_POINT('Ctrl Pts',(-55.9193127277193,-103.760358146992,
178.072094410988));
#25120=CARTESIAN_POINT('Ctrl Pts',(-55.0499426939411,-103.758757572204,
177.207792449865));
#25121=CARTESIAN_POINT('Ctrl Pts',(-55.0400046818809,-103.665535802127,
175.985484945604));
#25122=CARTESIAN_POINT('Ctrl Pts',(-55.0300666698208,-103.57231403205,174.763177441344));
#25123=CARTESIAN_POINT('Ctrl Pts',(-55.8795606496874,-103.387471069859,
173.89887555255));
#25124=CARTESIAN_POINT('Ctrl Pts',(-56.7290546295541,-103.202628107669,
173.034573663757));
#25125=CARTESIAN_POINT('Ctrl Pts',(-57.934536966623,-102.97983440828,173.034573714903));
#25126=CARTESIAN_POINT('Ctrl Pts',(-59.1400193036918,-102.757040708891,
173.034573766048));
#25127=CARTESIAN_POINT('Ctrl Pts',(-59.989513211636,-102.572197754367,173.898875727171));
#25128=CARTESIAN_POINT('Ctrl Pts',(-60.8390071195802,-102.387354799844,
174.763177688294));
#25129=CARTESIAN_POINT('Ctrl Pts',(-60.8290690058063,-102.29413304061,175.985485192554));
#25130=CARTESIAN_POINT('Ctrl Pts',(-60.8191308920325,-102.200911281377,
177.207792696815));
#25131=CARTESIAN_POINT('Ctrl Pts',(-59.9497607863318,-102.199310714257,
178.072094585608));
#25132=CARTESIAN_POINT('Ctrl Pts',(-59.0803906806311,-102.197710147137,
178.936396474401));
#25133=CARTESIAN_POINT('Ctrl Pts',(-57.8550322177282,-102.234060317215,
178.936396423256));
#25134=CARTESIAN_POINT('Ctrl Pts',(-56.6296737548253,-102.270410487293,
178.936396372111));
#25135=CARTESIAN_POINT('Ctrl Pts',(-55.7603037210471,-102.268809912506,
178.072094410988));
#25136=CARTESIAN_POINT('Ctrl Pts',(-54.8909336872689,-102.267209337719,
177.207792449865));
#25137=CARTESIAN_POINT('Ctrl Pts',(-54.8809956752087,-102.173987567642,
175.985484945604));
#25138=CARTESIAN_POINT('Ctrl Pts',(-54.8710576631486,-102.080765797565,
174.763177441344));
#25139=CARTESIAN_POINT('Ctrl Pts',(-55.7205516430152,-101.895922835374,
173.89887555255));
#25140=CARTESIAN_POINT('Ctrl Pts',(-56.5700456228819,-101.711079873183,
173.034573663757));
#25141=CARTESIAN_POINT('Ctrl Pts',(-57.7755279599507,-101.488286173794,
173.034573714903));
#25142=CARTESIAN_POINT('Ctrl Pts',(-58.9810102970196,-101.265492474405,
173.034573766048));
#25143=CARTESIAN_POINT('Ctrl Pts',(-59.8305042049638,-101.080649519882,
173.898875727171));
#25144=CARTESIAN_POINT('Ctrl Pts',(-60.679998112908,-100.895806565358,174.763177688294));
#25145=CARTESIAN_POINT('Ctrl Pts',(-60.6700599991341,-100.802584806125,
175.985485192554));
#25146=CARTESIAN_POINT('Ctrl Pts',(-60.6601218853602,-100.709363046891,
177.207792696815));
#25147=CARTESIAN_POINT('Ctrl Pts',(-59.7907517796595,-100.707762479771,
178.072094585608));
#25148=CARTESIAN_POINT('Ctrl Pts',(-58.9213816739588,-100.706161912651,
178.936396474401));
#25149=CARTESIAN_POINT('Ctrl Pts',(-57.696023211056,-100.742512082729,178.936396423256));
#25150=CARTESIAN_POINT('Ctrl Pts',(-56.4706647481531,-100.778862252808,
178.936396372111));
#25151=CARTESIAN_POINT('Ctrl Pts',(-55.6012947143749,-100.77726167802,178.072094410988));
#25152=CARTESIAN_POINT('Ctrl Pts',(-54.7319246805966,-100.775661103233,
177.207792449865));
#25153=CARTESIAN_POINT('Ctrl Pts',(-54.7219866685365,-100.682439333156,
175.985484945604));
#25154=CARTESIAN_POINT('Ctrl Pts',(-54.7120486564763,-100.589217563079,
174.763177441344));
#25155=CARTESIAN_POINT('Ctrl Pts',(-55.561542636343,-100.404374600888,173.89887555255));
#25156=CARTESIAN_POINT('Ctrl Pts',(-56.4110366162097,-100.219531638698,
173.034573663757));
#25157=CARTESIAN_POINT('Ctrl Pts',(-57.6165189532785,-99.9967379393085,
173.034573714903));
#25158=CARTESIAN_POINT('Ctrl Pts',(-58.8220012903473,-99.7739442399195,
173.034573766048));
#25159=CARTESIAN_POINT('Ctrl Pts',(-59.6714951982915,-99.5891012853962,
173.898875727171));
#25160=CARTESIAN_POINT('Ctrl Pts',(-60.5209891062358,-99.4042583308729,
174.763177688294));
#25161=CARTESIAN_POINT('Ctrl Pts',(-60.5110509924619,-99.3110365716392,
175.985485192554));
#25162=CARTESIAN_POINT('Ctrl Pts',(-60.501112878688,-99.2178148124055,177.207792696815));
#25163=CARTESIAN_POINT('Ctrl Pts',(-59.6317427729873,-99.2162142452855,
178.072094585608));
#25164=CARTESIAN_POINT('Ctrl Pts',(-58.7623726672866,-99.2146136781656,
178.936396474401));
#25165=CARTESIAN_POINT('Ctrl Pts',(-57.5370142043838,-99.2509638482439,
178.936396423256));
#25166=CARTESIAN_POINT('Ctrl Pts',(-56.3116557414809,-99.2873140183222,
178.936396372111));
#25167=CARTESIAN_POINT('Ctrl Pts',(-55.4422857077027,-99.2857134435348,
178.072094410988));
#25168=CARTESIAN_POINT('Ctrl Pts',(-54.5729156739244,-99.2841128687474,
177.207792449865));
#25169=CARTESIAN_POINT('Ctrl Pts',(-54.5629776618643,-99.1908910986704,
175.985484945604));
#25170=CARTESIAN_POINT('Ctrl Pts',(-54.5530396498041,-99.0976693285933,
174.763177441344));
#25171=CARTESIAN_POINT('Ctrl Pts',(-55.4025336296708,-98.9128263664026,
173.89887555255));
#25172=CARTESIAN_POINT('Ctrl Pts',(-56.2520276095374,-98.727983404212,173.034573663757));
#25173=CARTESIAN_POINT('Ctrl Pts',(-57.4575099466063,-98.5051897048229,
173.034573714903));
#25174=CARTESIAN_POINT('Ctrl Pts',(-58.6629922836751,-98.2823960054338,
173.034573766048));
#25175=CARTESIAN_POINT('Ctrl Pts',(-59.5124861916193,-98.0975530509106,
173.898875727171));
#25176=CARTESIAN_POINT('Ctrl Pts',(-60.3619800995635,-97.9127100963873,
174.763177688294));
#25177=CARTESIAN_POINT('Ctrl Pts',(-60.3520419857897,-97.8194883371536,
175.985485192554));
#25178=CARTESIAN_POINT('Ctrl Pts',(-60.3421038720158,-97.7262665779199,
177.207792696815));
#25179=CARTESIAN_POINT('Ctrl Pts',(-59.4727337663151,-97.7246660108,178.072094585608));
#25180=CARTESIAN_POINT('Ctrl Pts',(-58.6033636606144,-97.72306544368,178.936396474401));
#25181=CARTESIAN_POINT('Ctrl Pts',(-57.3780051977115,-97.7594156137583,
178.936396423256));
#25182=CARTESIAN_POINT('Ctrl Pts',(-56.1526467348087,-97.7957657838366,
178.936396372111));
#25183=CARTESIAN_POINT('Ctrl Pts',(-55.2832767010304,-97.7941652090492,
178.072094410988));
#25184=CARTESIAN_POINT('Ctrl Pts',(-56.1707931031902,-113.117197303651,
178.813912075476));
#25185=CARTESIAN_POINT('Ctrl Pts',(-54.9958834532485,-113.148169293224,
177.6423391512));
#25186=CARTESIAN_POINT('Ctrl Pts',(-54.9859454592686,-113.05494752122,175.985484901707));
#25187=CARTESIAN_POINT('Ctrl Pts',(-54.9760074652888,-112.961725749215,
174.328630652215));
#25188=CARTESIAN_POINT('Ctrl Pts',(-56.1310410868884,-112.744310219938,
173.157057825983));
#25189=CARTESIAN_POINT('Ctrl Pts',(-57.286074708488,-112.52689469066,171.985484999752));
#25190=CARTESIAN_POINT('Ctrl Pts',(-58.9236553326579,-112.258036427063,
171.985485069079));
#25191=CARTESIAN_POINT('Ctrl Pts',(-60.5612359568277,-111.989178163466,
171.985485138407));
#25192=CARTESIAN_POINT('Ctrl Pts',(-61.7162694809355,-111.771762644582,
173.157058062683));
#25193=CARTESIAN_POINT('Ctrl Pts',(-62.8713030050432,-111.554347125698,
174.328630986959));
#25194=CARTESIAN_POINT('Ctrl Pts',(-62.861364873189,-111.461125368392,175.985485236451));
#25195=CARTESIAN_POINT('Ctrl Pts',(-62.8514267413349,-111.367903611086,
177.642339485944));
#25196=CARTESIAN_POINT('Ctrl Pts',(-61.6765169939012,-111.398875611052,
178.813912312176));
#25197=CARTESIAN_POINT('Ctrl Pts',(-60.5016072464676,-111.429847611019,
179.985485138407));
#25198=CARTESIAN_POINT('Ctrl Pts',(-58.8441504964637,-111.512262345305,
179.985485069079));
#25199=CARTESIAN_POINT('Ctrl Pts',(-57.1866937464598,-111.594677079592,
179.985484999752));
#25200=CARTESIAN_POINT('Ctrl Pts',(-56.011784096518,-111.625649069165,178.813912075476));
#25201=CARTESIAN_POINT('Ctrl Pts',(-54.8368744465762,-111.656621058739,
177.6423391512));
#25202=CARTESIAN_POINT('Ctrl Pts',(-54.8269364525964,-111.563399286734,
175.985484901707));
#25203=CARTESIAN_POINT('Ctrl Pts',(-54.8169984586165,-111.47017751473,174.328630652215));
#25204=CARTESIAN_POINT('Ctrl Pts',(-55.9720320802161,-111.252761985452,
173.157057825983));
#25205=CARTESIAN_POINT('Ctrl Pts',(-57.1270657018158,-111.035346456175,
171.985484999752));
#25206=CARTESIAN_POINT('Ctrl Pts',(-58.7646463259856,-110.766488192578,
171.985485069079));
#25207=CARTESIAN_POINT('Ctrl Pts',(-60.4022269501555,-110.497629928981,
171.985485138407));
#25208=CARTESIAN_POINT('Ctrl Pts',(-61.5572604742632,-110.280214410097,
173.157058062683));
#25209=CARTESIAN_POINT('Ctrl Pts',(-62.712293998371,-110.062798891212,174.328630986959));
#25210=CARTESIAN_POINT('Ctrl Pts',(-62.7023558665168,-109.969577133906,
175.985485236451));
#25211=CARTESIAN_POINT('Ctrl Pts',(-62.6924177346626,-109.8763553766,177.642339485944));
#25212=CARTESIAN_POINT('Ctrl Pts',(-61.517507987229,-109.907327376567,178.813912312176));
#25213=CARTESIAN_POINT('Ctrl Pts',(-60.3425982397954,-109.938299376534,
179.985485138407));
#25214=CARTESIAN_POINT('Ctrl Pts',(-58.6851414897915,-110.02071411082,179.985485069079));
#25215=CARTESIAN_POINT('Ctrl Pts',(-57.0276847397876,-110.103128845106,
179.985484999752));
#25216=CARTESIAN_POINT('Ctrl Pts',(-55.8527750898458,-110.13410083468,178.813912075476));
#25217=CARTESIAN_POINT('Ctrl Pts',(-54.677865439904,-110.165072824253,177.6423391512));
#25218=CARTESIAN_POINT('Ctrl Pts',(-54.6679274459242,-110.071851052249,
175.985484901707));
#25219=CARTESIAN_POINT('Ctrl Pts',(-54.6579894519443,-109.978629280244,
174.328630652215));
#25220=CARTESIAN_POINT('Ctrl Pts',(-55.8130230735439,-109.761213750967,
173.157057825983));
#25221=CARTESIAN_POINT('Ctrl Pts',(-56.9680566951435,-109.543798221689,
171.985484999752));
#25222=CARTESIAN_POINT('Ctrl Pts',(-58.6056373193134,-109.274939958092,
171.985485069079));
#25223=CARTESIAN_POINT('Ctrl Pts',(-60.2432179434833,-109.006081694495,
171.985485138407));
#25224=CARTESIAN_POINT('Ctrl Pts',(-61.398251467591,-108.788666175611,173.157058062683));
#25225=CARTESIAN_POINT('Ctrl Pts',(-62.5532849916988,-108.571250656727,
174.328630986959));
#25226=CARTESIAN_POINT('Ctrl Pts',(-62.5433468598446,-108.478028899421,
175.985485236451));
#25227=CARTESIAN_POINT('Ctrl Pts',(-62.5334087279904,-108.384807142114,
177.642339485944));
#25228=CARTESIAN_POINT('Ctrl Pts',(-61.3584989805568,-108.415779142081,
178.813912312176));
#25229=CARTESIAN_POINT('Ctrl Pts',(-60.1835892331231,-108.446751142048,
179.985485138407));
#25230=CARTESIAN_POINT('Ctrl Pts',(-58.5261324831192,-108.529165876334,
179.985485069079));
#25231=CARTESIAN_POINT('Ctrl Pts',(-56.8686757331153,-108.611580610621,
179.985484999752));
#25232=CARTESIAN_POINT('Ctrl Pts',(-55.6937660831736,-108.642552600194,
178.813912075476));
#25233=CARTESIAN_POINT('Ctrl Pts',(-54.5188564332318,-108.673524589768,
177.6423391512));
#25234=CARTESIAN_POINT('Ctrl Pts',(-54.5089184392519,-108.580302817763,
175.985484901707));
#25235=CARTESIAN_POINT('Ctrl Pts',(-54.4989804452721,-108.487081045759,
174.328630652215));
#25236=CARTESIAN_POINT('Ctrl Pts',(-55.6540140668717,-108.269665516481,
173.157057825983));
#25237=CARTESIAN_POINT('Ctrl Pts',(-56.8090476884713,-108.052249987204,
171.985484999752));
#25238=CARTESIAN_POINT('Ctrl Pts',(-58.4466283126412,-107.783391723607,
171.985485069079));
#25239=CARTESIAN_POINT('Ctrl Pts',(-60.084208936811,-107.51453346001,171.985485138407));
#25240=CARTESIAN_POINT('Ctrl Pts',(-61.2392424609188,-107.297117941125,
173.157058062683));
#25241=CARTESIAN_POINT('Ctrl Pts',(-62.3942759850265,-107.079702422241,
174.328630986959));
#25242=CARTESIAN_POINT('Ctrl Pts',(-62.3843378531723,-106.986480664935,
175.985485236451));
#25243=CARTESIAN_POINT('Ctrl Pts',(-62.3743997213182,-106.893258907629,
177.642339485944));
#25244=CARTESIAN_POINT('Ctrl Pts',(-61.1994899738845,-106.924230907596,
178.813912312176));
#25245=CARTESIAN_POINT('Ctrl Pts',(-60.0245802264509,-106.955202907562,
179.985485138407));
#25246=CARTESIAN_POINT('Ctrl Pts',(-58.367123476447,-107.037617641849,179.985485069079));
#25247=CARTESIAN_POINT('Ctrl Pts',(-56.7096667264431,-107.120032376135,
179.985484999752));
#25248=CARTESIAN_POINT('Ctrl Pts',(-55.5347570765013,-107.151004365708,
178.813912075476));
#25249=CARTESIAN_POINT('Ctrl Pts',(-54.3598474265596,-107.181976355282,
177.6423391512));
#25250=CARTESIAN_POINT('Ctrl Pts',(-54.3499094325797,-107.088754583277,
175.985484901707));
#25251=CARTESIAN_POINT('Ctrl Pts',(-54.3399714385998,-106.995532811273,
174.328630652215));
#25252=CARTESIAN_POINT('Ctrl Pts',(-55.4950050601995,-106.778117281995,
173.157057825983));
#25253=CARTESIAN_POINT('Ctrl Pts',(-56.6500386817991,-106.560701752718,
171.985484999752));
#25254=CARTESIAN_POINT('Ctrl Pts',(-58.2876193059689,-106.291843489121,
171.985485069079));
#25255=CARTESIAN_POINT('Ctrl Pts',(-59.9251999301388,-106.022985225524,
171.985485138407));
#25256=CARTESIAN_POINT('Ctrl Pts',(-61.0802334542465,-105.80556970664,173.157058062683));
#25257=CARTESIAN_POINT('Ctrl Pts',(-62.2352669783543,-105.588154187756,
174.328630986959));
#25258=CARTESIAN_POINT('Ctrl Pts',(-62.2253288465001,-105.494932430449,
175.985485236451));
#25259=CARTESIAN_POINT('Ctrl Pts',(-62.2153907146459,-105.401710673143,
177.642339485944));
#25260=CARTESIAN_POINT('Ctrl Pts',(-61.0404809672123,-105.43268267311,178.813912312176));
#25261=CARTESIAN_POINT('Ctrl Pts',(-59.8655712197787,-105.463654673077,
179.985485138407));
#25262=CARTESIAN_POINT('Ctrl Pts',(-58.2081144697748,-105.546069407363,
179.985485069079));
#25263=CARTESIAN_POINT('Ctrl Pts',(-56.5506577197709,-105.628484141649,
179.985484999752));
#25264=CARTESIAN_POINT('Ctrl Pts',(-55.3757480698291,-105.659456131223,
178.813912075476));
#25265=CARTESIAN_POINT('Ctrl Pts',(-54.2008384198873,-105.690428120796,
177.6423391512));
#25266=CARTESIAN_POINT('Ctrl Pts',(-54.1909004259075,-105.597206348792,
175.985484901707));
#25267=CARTESIAN_POINT('Ctrl Pts',(-54.1809624319276,-105.503984576787,
174.328630652215));
#25268=CARTESIAN_POINT('Ctrl Pts',(-55.3359960535272,-105.28656904751,173.157057825983));
#25269=CARTESIAN_POINT('Ctrl Pts',(-56.4910296751268,-105.069153518232,
171.985484999752));
#25270=CARTESIAN_POINT('Ctrl Pts',(-58.1286102992967,-104.800295254635,
171.985485069079));
#25271=CARTESIAN_POINT('Ctrl Pts',(-59.7661909234666,-104.531436991038,
171.985485138407));
#25272=CARTESIAN_POINT('Ctrl Pts',(-60.9212244475743,-104.314021472154,
173.157058062683));
#25273=CARTESIAN_POINT('Ctrl Pts',(-62.0762579716821,-104.09660595327,174.328630986959));
#25274=CARTESIAN_POINT('Ctrl Pts',(-62.0663198398279,-104.003384195964,
175.985485236451));
#25275=CARTESIAN_POINT('Ctrl Pts',(-62.0563817079737,-103.910162438658,
177.642339485944));
#25276=CARTESIAN_POINT('Ctrl Pts',(-60.8814719605401,-103.941134438624,
178.813912312176));
#25277=CARTESIAN_POINT('Ctrl Pts',(-59.7065622131064,-103.972106438591,
179.985485138407));
#25278=CARTESIAN_POINT('Ctrl Pts',(-58.0491054631025,-104.054521172878,
179.985485069079));
#25279=CARTESIAN_POINT('Ctrl Pts',(-56.3916487130987,-104.136935907164,
179.985484999752));
#25280=CARTESIAN_POINT('Ctrl Pts',(-55.2167390631569,-104.167907896737,
178.813912075476));
#25281=CARTESIAN_POINT('Ctrl Pts',(-54.0418294132151,-104.198879886311,
177.6423391512));
#25282=CARTESIAN_POINT('Ctrl Pts',(-54.0318914192353,-104.105658114306,
175.985484901707));
#25283=CARTESIAN_POINT('Ctrl Pts',(-54.0219534252554,-104.012436342302,
174.328630652215));
#25284=CARTESIAN_POINT('Ctrl Pts',(-55.176987046855,-103.795020813024,173.157057825983));
#25285=CARTESIAN_POINT('Ctrl Pts',(-56.3320206684546,-103.577605283747,
171.985484999752));
#25286=CARTESIAN_POINT('Ctrl Pts',(-57.9696012926245,-103.30874702015,171.985485069079));
#25287=CARTESIAN_POINT('Ctrl Pts',(-59.6071819167943,-103.039888756553,
171.985485138407));
#25288=CARTESIAN_POINT('Ctrl Pts',(-60.7622154409021,-102.822473237669,
173.157058062683));
#25289=CARTESIAN_POINT('Ctrl Pts',(-61.9172489650099,-102.605057718784,
174.328630986959));
#25290=CARTESIAN_POINT('Ctrl Pts',(-61.9073108331557,-102.511835961478,
175.985485236451));
#25291=CARTESIAN_POINT('Ctrl Pts',(-61.8973727013015,-102.418614204172,
177.642339485944));
#25292=CARTESIAN_POINT('Ctrl Pts',(-60.7224629538678,-102.449586204139,
178.813912312176));
#25293=CARTESIAN_POINT('Ctrl Pts',(-59.5475532064342,-102.480558204106,
179.985485138407));
#25294=CARTESIAN_POINT('Ctrl Pts',(-57.8900964564303,-102.562972938392,
179.985485069079));
#25295=CARTESIAN_POINT('Ctrl Pts',(-56.2326397064264,-102.645387672678,
179.985484999752));
#25296=CARTESIAN_POINT('Ctrl Pts',(-55.0577300564847,-102.676359662252,
178.813912075476));
#25297=CARTESIAN_POINT('Ctrl Pts',(-53.8828204065429,-102.707331651825,
177.6423391512));
#25298=CARTESIAN_POINT('Ctrl Pts',(-53.872882412563,-102.614109879821,175.985484901707));
#25299=CARTESIAN_POINT('Ctrl Pts',(-53.8629444185832,-102.520888107816,
174.328630652215));
#25300=CARTESIAN_POINT('Ctrl Pts',(-55.0179780401828,-102.303472578539,
173.157057825983));
#25301=CARTESIAN_POINT('Ctrl Pts',(-56.1730116617824,-102.086057049261,
171.985484999752));
#25302=CARTESIAN_POINT('Ctrl Pts',(-57.8105922859523,-101.817198785664,
171.985485069079));
#25303=CARTESIAN_POINT('Ctrl Pts',(-59.4481729101221,-101.548340522067,
171.985485138407));
#25304=CARTESIAN_POINT('Ctrl Pts',(-60.6032064342299,-101.330925003183,
173.157058062683));
#25305=CARTESIAN_POINT('Ctrl Pts',(-61.7582399583376,-101.113509484299,
174.328630986959));
#25306=CARTESIAN_POINT('Ctrl Pts',(-61.7483018264834,-101.020287726993,
175.985485236451));
#25307=CARTESIAN_POINT('Ctrl Pts',(-61.7383636946293,-100.927065969686,
177.642339485944));
#25308=CARTESIAN_POINT('Ctrl Pts',(-60.5634539471956,-100.958037969653,
178.813912312176));
#25309=CARTESIAN_POINT('Ctrl Pts',(-59.388544199762,-100.98900996962,179.985485138407));
#25310=CARTESIAN_POINT('Ctrl Pts',(-57.7310874497581,-101.071424703906,
179.985485069079));
#25311=CARTESIAN_POINT('Ctrl Pts',(-56.0736306997542,-101.153839438193,
179.985484999752));
#25312=CARTESIAN_POINT('Ctrl Pts',(-54.8987210498124,-101.184811427766,
178.813912075476));
#25313=CARTESIAN_POINT('Ctrl Pts',(-53.7238113998707,-101.21578341734,177.6423391512));
#25314=CARTESIAN_POINT('Ctrl Pts',(-53.7138734058908,-101.122561645335,
175.985484901707));
#25315=CARTESIAN_POINT('Ctrl Pts',(-53.7039354119109,-101.029339873331,
174.328630652215));
#25316=CARTESIAN_POINT('Ctrl Pts',(-54.8589690335105,-100.811924344053,
173.157057825983));
#25317=CARTESIAN_POINT('Ctrl Pts',(-56.0140026551102,-100.594508814776,
171.985484999752));
#25318=CARTESIAN_POINT('Ctrl Pts',(-57.65158327928,-100.325650551179,171.985485069079));
#25319=CARTESIAN_POINT('Ctrl Pts',(-59.2891639034499,-100.056792287582,
171.985485138407));
#25320=CARTESIAN_POINT('Ctrl Pts',(-60.4441974275576,-99.8393767686974,
173.157058062683));
#25321=CARTESIAN_POINT('Ctrl Pts',(-61.5992309516654,-99.6219612498133,
174.328630986959));
#25322=CARTESIAN_POINT('Ctrl Pts',(-61.5892928198112,-99.528739492507,175.985485236451));
#25323=CARTESIAN_POINT('Ctrl Pts',(-61.579354687957,-99.4355177352008,177.642339485944));
#25324=CARTESIAN_POINT('Ctrl Pts',(-60.4044449405234,-99.4664897351676,
178.813912312176));
#25325=CARTESIAN_POINT('Ctrl Pts',(-59.2295351930898,-99.4974617351344,
179.985485138407));
#25326=CARTESIAN_POINT('Ctrl Pts',(-57.5720784430859,-99.5798764694207,
179.985485069079));
#25327=CARTESIAN_POINT('Ctrl Pts',(-55.914621693082,-99.662291203707,179.985484999752));
#25328=CARTESIAN_POINT('Ctrl Pts',(-54.7397120431402,-99.6932631932805,
178.813912075476));
#25329=CARTESIAN_POINT('Ctrl Pts',(-53.5648023931984,-99.724235182854,177.6423391512));
#25330=CARTESIAN_POINT('Ctrl Pts',(-53.5548643992186,-99.6310134108495,
175.985484901707));
#25331=CARTESIAN_POINT('Ctrl Pts',(-53.5449264052387,-99.5377916388449,
174.328630652215));
#25332=CARTESIAN_POINT('Ctrl Pts',(-54.6999600268383,-99.3203761095675,
173.157057825983));
#25333=CARTESIAN_POINT('Ctrl Pts',(-55.8549936484379,-99.10296058029,171.985484999752));
#25334=CARTESIAN_POINT('Ctrl Pts',(-57.4925742726078,-98.834102316693,171.985485069079));
#25335=CARTESIAN_POINT('Ctrl Pts',(-59.1301548967777,-98.565244053096,171.985485138407));
#25336=CARTESIAN_POINT('Ctrl Pts',(-60.2851884208854,-98.3478285342118,
173.157058062683));
#25337=CARTESIAN_POINT('Ctrl Pts',(-61.4402219449932,-98.1304130153276,
174.328630986959));
#25338=CARTESIAN_POINT('Ctrl Pts',(-61.430283813139,-98.0371912580215,175.985485236451));
#25339=CARTESIAN_POINT('Ctrl Pts',(-61.4203456812848,-97.9439695007152,
177.642339485944));
#25340=CARTESIAN_POINT('Ctrl Pts',(-60.2454359338512,-97.974941500682,178.813912312176));
#25341=CARTESIAN_POINT('Ctrl Pts',(-59.0705261864175,-98.0059135006488,
179.985485138407));
#25342=CARTESIAN_POINT('Ctrl Pts',(-57.4130694364136,-98.0883282349351,
179.985485069079));
#25343=CARTESIAN_POINT('Ctrl Pts',(-55.7556126864097,-98.1707429692214,
179.985484999752));
#25344=CARTESIAN_POINT('Ctrl Pts',(-54.580703036468,-98.2017149587949,178.813912075476));
#25345=CARTESIAN_POINT('Ctrl Pts',(-61.8126236112619,-109.901486190407,
178.485485069079));
#25346=CARTESIAN_POINT('Ctrl Pts',(-61.6740514069051,-109.903200708285,
178.657813499464));
#25347=CARTESIAN_POINT('Ctrl Pts',(-61.517507987229,-109.907327376567,178.813912312176));
#25348=CARTESIAN_POINT('Ctrl Pts',(-60.3425982397954,-109.938299376534,
179.985485138407));
#25349=CARTESIAN_POINT('Ctrl Pts',(-58.6851414897915,-110.02071411082,179.985485069079));
#25350=CARTESIAN_POINT('Ctrl Pts',(-57.0276847397876,-110.103128845106,
179.985484999752));
#25351=CARTESIAN_POINT('Ctrl Pts',(-55.8527750898458,-110.13410083468,178.813912075476));
#25352=CARTESIAN_POINT('Ctrl Pts',(-54.677865439904,-110.165072824253,177.6423391512));
#25353=CARTESIAN_POINT('Ctrl Pts',(-54.6679274459242,-110.071851052249,
175.985484901707));
#25354=CARTESIAN_POINT('Ctrl Pts',(-54.6579894519443,-109.978629280244,
174.328630652215));
#25355=CARTESIAN_POINT('Ctrl Pts',(-55.8130230735439,-109.761213750967,
173.157057825983));
#25356=CARTESIAN_POINT('Ctrl Pts',(-56.9680566951435,-109.543798221689,
171.985484999752));
#25357=CARTESIAN_POINT('Ctrl Pts',(-58.6056373193134,-109.274939958092,
171.985485069079));
#25358=CARTESIAN_POINT('Ctrl Pts',(-60.2432179434833,-109.006081694495,
171.985485138407));
#25359=CARTESIAN_POINT('Ctrl Pts',(-61.398251467591,-108.788666175611,173.157058062683));
#25360=CARTESIAN_POINT('Ctrl Pts',(-61.5521464885441,-108.759698041669,
173.313156769748));
#25361=CARTESIAN_POINT('Ctrl Pts',(-61.687965692515,-108.732160612486,173.485485069079));
#25362=CARTESIAN_POINT('Ctrl Pts',(-56.1707931031902,-113.117197303651,
178.813912075476));
#25363=CARTESIAN_POINT('Ctrl Pts',(-54.9958834532485,-113.148169293224,
177.6423391512));
#25364=CARTESIAN_POINT('Ctrl Pts',(-54.9859454592686,-113.05494752122,175.985484901707));
#25365=CARTESIAN_POINT('Ctrl Pts',(-54.9760074652888,-112.961725749215,
174.328630652215));
#25366=CARTESIAN_POINT('Ctrl Pts',(-56.1310410868884,-112.744310219938,
173.157057825983));
#25367=CARTESIAN_POINT('Ctrl Pts',(-57.286074708488,-112.52689469066,171.985484999752));
#25368=CARTESIAN_POINT('Ctrl Pts',(-58.9236553326578,-112.258036427063,
171.985485069079));
#25369=CARTESIAN_POINT('Ctrl Pts',(-60.5612359568277,-111.989178163466,
171.985485138407));
#25370=CARTESIAN_POINT('Ctrl Pts',(-61.7162694809355,-111.771762644582,
173.157058062683));
#25371=CARTESIAN_POINT('Ctrl Pts',(-62.8713030050432,-111.554347125698,
174.328630986959));
#25372=CARTESIAN_POINT('Ctrl Pts',(-62.861364873189,-111.461125368392,175.985485236451));
#25373=CARTESIAN_POINT('Ctrl Pts',(-62.8514267413349,-111.367903611086,
177.642339485944));
#25374=CARTESIAN_POINT('Ctrl Pts',(-61.6765169939012,-111.398875611052,
178.813912312176));
#25375=CARTESIAN_POINT('Ctrl Pts',(-60.5016072464676,-111.429847611019,
179.985485138407));
#25376=CARTESIAN_POINT('Ctrl Pts',(-58.8441504964637,-111.512262345305,
179.985485069079));
#25377=CARTESIAN_POINT('Ctrl Pts',(-57.1866937464598,-111.594677079592,
179.985484999752));
#25378=CARTESIAN_POINT('Ctrl Pts',(-56.011784096518,-111.625649069165,178.813912075476));
#25379=CARTESIAN_POINT('Ctrl Pts',(-54.8368744465763,-111.656621058739,
177.6423391512));
#25380=CARTESIAN_POINT('Ctrl Pts',(-54.8269364525964,-111.563399286734,
175.985484901707));
#25381=CARTESIAN_POINT('Ctrl Pts',(-54.8169984586165,-111.47017751473,174.328630652215));
#25382=CARTESIAN_POINT('Ctrl Pts',(-55.9720320802161,-111.252761985452,
173.157057825983));
#25383=CARTESIAN_POINT('Ctrl Pts',(-57.1270657018158,-111.035346456175,
171.985484999752));
#25384=CARTESIAN_POINT('Ctrl Pts',(-58.7646463259856,-110.766488192578,
171.985485069079));
#25385=CARTESIAN_POINT('Ctrl Pts',(-60.4022269501555,-110.497629928981,
171.985485138407));
#25386=CARTESIAN_POINT('Ctrl Pts',(-61.5572604742632,-110.280214410097,
173.157058062683));
#25387=CARTESIAN_POINT('Ctrl Pts',(-62.712293998371,-110.062798891212,174.328630986959));
#25388=CARTESIAN_POINT('Ctrl Pts',(-62.7023558665168,-109.969577133906,
175.985485236451));
#25389=CARTESIAN_POINT('Ctrl Pts',(-62.6924177346626,-109.8763553766,177.642339485944));
#25390=CARTESIAN_POINT('Ctrl Pts',(-61.517507987229,-109.907327376567,178.813912312176));
#25391=CARTESIAN_POINT('Ctrl Pts',(-60.3425982397954,-109.938299376534,
179.985485138407));
#25392=CARTESIAN_POINT('Ctrl Pts',(-58.6851414897915,-110.02071411082,179.985485069079));
#25393=CARTESIAN_POINT('Ctrl Pts',(-57.0276847397876,-110.103128845106,
179.985484999752));
#25394=CARTESIAN_POINT('Ctrl Pts',(-55.8527750898458,-110.13410083468,178.813912075476));
#25395=CARTESIAN_POINT('Ctrl Pts',(-54.677865439904,-110.165072824253,177.6423391512));
#25396=CARTESIAN_POINT('Ctrl Pts',(-54.6679274459242,-110.071851052249,
175.985484901707));
#25397=CARTESIAN_POINT('Ctrl Pts',(-54.6579894519443,-109.978629280244,
174.328630652215));
#25398=CARTESIAN_POINT('Ctrl Pts',(-55.8130230735439,-109.761213750967,
173.157057825983));
#25399=CARTESIAN_POINT('Ctrl Pts',(-56.9680566951435,-109.543798221689,
171.985484999752));
#25400=CARTESIAN_POINT('Ctrl Pts',(-58.6056373193134,-109.274939958092,
171.985485069079));
#25401=CARTESIAN_POINT('Ctrl Pts',(-60.2432179434833,-109.006081694495,
171.985485138407));
#25402=CARTESIAN_POINT('Ctrl Pts',(-61.398251467591,-108.788666175611,173.157058062683));
#25403=CARTESIAN_POINT('Ctrl Pts',(-62.5532849916988,-108.571250656727,
174.328630986959));
#25404=CARTESIAN_POINT('Ctrl Pts',(-62.5433468598446,-108.478028899421,
175.985485236451));
#25405=CARTESIAN_POINT('Ctrl Pts',(-62.5334087279904,-108.384807142114,
177.642339485944));
#25406=CARTESIAN_POINT('Ctrl Pts',(-61.3584989805568,-108.415779142081,
178.813912312176));
#25407=CARTESIAN_POINT('Ctrl Pts',(-60.1835892331231,-108.446751142048,
179.985485138407));
#25408=CARTESIAN_POINT('Ctrl Pts',(-58.5261324831192,-108.529165876334,
179.985485069079));
#25409=CARTESIAN_POINT('Ctrl Pts',(-56.8686757331153,-108.611580610621,
179.985484999752));
#25410=CARTESIAN_POINT('Ctrl Pts',(-55.6937660831736,-108.642552600194,
178.813912075476));
#25411=CARTESIAN_POINT('Ctrl Pts',(-54.5188564332318,-108.673524589768,
177.6423391512));
#25412=CARTESIAN_POINT('Ctrl Pts',(-54.5089184392519,-108.580302817763,
175.985484901707));
#25413=CARTESIAN_POINT('Ctrl Pts',(-54.4989804452721,-108.487081045759,
174.328630652215));
#25414=CARTESIAN_POINT('Ctrl Pts',(-55.6540140668717,-108.269665516481,
173.157057825983));
#25415=CARTESIAN_POINT('Ctrl Pts',(-56.8090476884713,-108.052249987204,
171.985484999752));
#25416=CARTESIAN_POINT('Ctrl Pts',(-58.4466283126412,-107.783391723607,
171.985485069079));
#25417=CARTESIAN_POINT('Ctrl Pts',(-60.084208936811,-107.51453346001,171.985485138407));
#25418=CARTESIAN_POINT('Ctrl Pts',(-61.2392424609188,-107.297117941125,
173.157058062683));
#25419=CARTESIAN_POINT('Ctrl Pts',(-62.3942759850265,-107.079702422241,
174.328630986959));
#25420=CARTESIAN_POINT('Ctrl Pts',(-62.3843378531723,-106.986480664935,
175.985485236451));
#25421=CARTESIAN_POINT('Ctrl Pts',(-62.3743997213182,-106.893258907629,
177.642339485944));
#25422=CARTESIAN_POINT('Ctrl Pts',(-61.1994899738845,-106.924230907596,
178.813912312176));
#25423=CARTESIAN_POINT('Ctrl Pts',(-60.0245802264509,-106.955202907562,
179.985485138407));
#25424=CARTESIAN_POINT('Ctrl Pts',(-58.367123476447,-107.037617641849,179.985485069079));
#25425=CARTESIAN_POINT('Ctrl Pts',(-56.7096667264431,-107.120032376135,
179.985484999752));
#25426=CARTESIAN_POINT('Ctrl Pts',(-55.5347570765013,-107.151004365708,
178.813912075476));
#25427=CARTESIAN_POINT('Ctrl Pts',(-54.3598474265596,-107.181976355282,
177.6423391512));
#25428=CARTESIAN_POINT('Ctrl Pts',(-54.3499094325797,-107.088754583277,
175.985484901707));
#25429=CARTESIAN_POINT('Ctrl Pts',(-54.3399714385998,-106.995532811273,
174.328630652215));
#25430=CARTESIAN_POINT('Ctrl Pts',(-55.4950050601995,-106.778117281995,
173.157057825983));
#25431=CARTESIAN_POINT('Ctrl Pts',(-56.6500386817991,-106.560701752718,
171.985484999752));
#25432=CARTESIAN_POINT('Ctrl Pts',(-58.2876193059689,-106.291843489121,
171.985485069079));
#25433=CARTESIAN_POINT('Ctrl Pts',(-59.9251999301388,-106.022985225524,
171.985485138407));
#25434=CARTESIAN_POINT('Ctrl Pts',(-61.0802334542465,-105.80556970664,173.157058062683));
#25435=CARTESIAN_POINT('Ctrl Pts',(-62.2352669783543,-105.588154187756,
174.328630986959));
#25436=CARTESIAN_POINT('Ctrl Pts',(-62.2253288465001,-105.494932430449,
175.985485236451));
#25437=CARTESIAN_POINT('Ctrl Pts',(-62.2153907146459,-105.401710673143,
177.642339485944));
#25438=CARTESIAN_POINT('Ctrl Pts',(-61.0404809672123,-105.43268267311,178.813912312176));
#25439=CARTESIAN_POINT('Ctrl Pts',(-59.8655712197787,-105.463654673077,
179.985485138407));
#25440=CARTESIAN_POINT('Ctrl Pts',(-58.2081144697748,-105.546069407363,
179.985485069079));
#25441=CARTESIAN_POINT('Ctrl Pts',(-56.5506577197709,-105.628484141649,
179.985484999752));
#25442=CARTESIAN_POINT('Ctrl Pts',(-55.3757480698291,-105.659456131223,
178.813912075476));
#25443=CARTESIAN_POINT('Ctrl Pts',(-54.2008384198873,-105.690428120796,
177.6423391512));
#25444=CARTESIAN_POINT('Ctrl Pts',(-54.1909004259075,-105.597206348792,
175.985484901707));
#25445=CARTESIAN_POINT('Ctrl Pts',(-54.1809624319276,-105.503984576787,
174.328630652215));
#25446=CARTESIAN_POINT('Ctrl Pts',(-55.3359960535272,-105.28656904751,173.157057825983));
#25447=CARTESIAN_POINT('Ctrl Pts',(-56.4910296751268,-105.069153518232,
171.985484999752));
#25448=CARTESIAN_POINT('Ctrl Pts',(-58.1286102992967,-104.800295254635,
171.985485069079));
#25449=CARTESIAN_POINT('Ctrl Pts',(-59.7661909234666,-104.531436991038,
171.985485138407));
#25450=CARTESIAN_POINT('Ctrl Pts',(-60.9212244475743,-104.314021472154,
173.157058062683));
#25451=CARTESIAN_POINT('Ctrl Pts',(-62.0762579716821,-104.09660595327,174.328630986959));
#25452=CARTESIAN_POINT('Ctrl Pts',(-62.0663198398279,-104.003384195964,
175.985485236451));
#25453=CARTESIAN_POINT('Ctrl Pts',(-62.0563817079737,-103.910162438658,
177.642339485944));
#25454=CARTESIAN_POINT('Ctrl Pts',(-60.8814719605401,-103.941134438624,
178.813912312176));
#25455=CARTESIAN_POINT('Ctrl Pts',(-59.7065622131064,-103.972106438591,
179.985485138407));
#25456=CARTESIAN_POINT('Ctrl Pts',(-58.0491054631025,-104.054521172878,
179.985485069079));
#25457=CARTESIAN_POINT('Ctrl Pts',(-56.3916487130987,-104.136935907164,
179.985484999752));
#25458=CARTESIAN_POINT('Ctrl Pts',(-55.2167390631569,-104.167907896737,
178.813912075476));
#25459=CARTESIAN_POINT('Ctrl Pts',(-54.0418294132151,-104.198879886311,
177.6423391512));
#25460=CARTESIAN_POINT('Ctrl Pts',(-54.0318914192353,-104.105658114306,
175.985484901707));
#25461=CARTESIAN_POINT('Ctrl Pts',(-54.0219534252554,-104.012436342302,
174.328630652215));
#25462=CARTESIAN_POINT('Ctrl Pts',(-55.176987046855,-103.795020813024,173.157057825983));
#25463=CARTESIAN_POINT('Ctrl Pts',(-56.3320206684546,-103.577605283747,
171.985484999752));
#25464=CARTESIAN_POINT('Ctrl Pts',(-57.9696012926245,-103.30874702015,171.985485069079));
#25465=CARTESIAN_POINT('Ctrl Pts',(-59.6071819167943,-103.039888756553,
171.985485138407));
#25466=CARTESIAN_POINT('Ctrl Pts',(-60.7622154409021,-102.822473237669,
173.157058062683));
#25467=CARTESIAN_POINT('Ctrl Pts',(-61.9172489650099,-102.605057718784,
174.328630986959));
#25468=CARTESIAN_POINT('Ctrl Pts',(-61.9073108331557,-102.511835961478,
175.985485236451));
#25469=CARTESIAN_POINT('Ctrl Pts',(-61.8973727013015,-102.418614204172,
177.642339485944));
#25470=CARTESIAN_POINT('Ctrl Pts',(-60.7224629538678,-102.449586204139,
178.813912312176));
#25471=CARTESIAN_POINT('Ctrl Pts',(-59.5475532064342,-102.480558204106,
179.985485138407));
#25472=CARTESIAN_POINT('Ctrl Pts',(-57.8900964564303,-102.562972938392,
179.985485069079));
#25473=CARTESIAN_POINT('Ctrl Pts',(-56.2326397064264,-102.645387672678,
179.985484999752));
#25474=CARTESIAN_POINT('Ctrl Pts',(-55.0577300564847,-102.676359662252,
178.813912075476));
#25475=CARTESIAN_POINT('Ctrl Pts',(-53.8828204065429,-102.707331651825,
177.6423391512));
#25476=CARTESIAN_POINT('Ctrl Pts',(-53.872882412563,-102.614109879821,175.985484901707));
#25477=CARTESIAN_POINT('Ctrl Pts',(-53.8629444185832,-102.520888107816,
174.328630652215));
#25478=CARTESIAN_POINT('Ctrl Pts',(-55.0179780401828,-102.303472578539,
173.157057825983));
#25479=CARTESIAN_POINT('Ctrl Pts',(-56.1730116617824,-102.086057049261,
171.985484999752));
#25480=CARTESIAN_POINT('Ctrl Pts',(-57.8105922859523,-101.817198785664,
171.985485069079));
#25481=CARTESIAN_POINT('Ctrl Pts',(-59.4481729101221,-101.548340522067,
171.985485138407));
#25482=CARTESIAN_POINT('Ctrl Pts',(-60.6032064342299,-101.330925003183,
173.157058062683));
#25483=CARTESIAN_POINT('Ctrl Pts',(-61.7582399583376,-101.113509484299,
174.328630986959));
#25484=CARTESIAN_POINT('Ctrl Pts',(-61.7483018264834,-101.020287726993,
175.985485236451));
#25485=CARTESIAN_POINT('Ctrl Pts',(-61.7383636946293,-100.927065969686,
177.642339485944));
#25486=CARTESIAN_POINT('Ctrl Pts',(-60.5634539471956,-100.958037969653,
178.813912312176));
#25487=CARTESIAN_POINT('Ctrl Pts',(-59.388544199762,-100.98900996962,179.985485138407));
#25488=CARTESIAN_POINT('Ctrl Pts',(-57.7310874497581,-101.071424703906,
179.985485069079));
#25489=CARTESIAN_POINT('Ctrl Pts',(-56.0736306997542,-101.153839438193,
179.985484999752));
#25490=CARTESIAN_POINT('Ctrl Pts',(-54.8987210498124,-101.184811427766,
178.813912075476));
#25491=CARTESIAN_POINT('Ctrl Pts',(-53.7238113998707,-101.21578341734,177.6423391512));
#25492=CARTESIAN_POINT('Ctrl Pts',(-53.7138734058908,-101.122561645335,
175.985484901707));
#25493=CARTESIAN_POINT('Ctrl Pts',(-53.7039354119109,-101.029339873331,
174.328630652215));
#25494=CARTESIAN_POINT('Ctrl Pts',(-54.8589690335105,-100.811924344053,
173.157057825983));
#25495=CARTESIAN_POINT('Ctrl Pts',(-56.0140026551102,-100.594508814776,
171.985484999752));
#25496=CARTESIAN_POINT('Ctrl Pts',(-57.65158327928,-100.325650551179,171.985485069079));
#25497=CARTESIAN_POINT('Ctrl Pts',(-59.2891639034499,-100.056792287582,
171.985485138407));
#25498=CARTESIAN_POINT('Ctrl Pts',(-60.4441974275576,-99.8393767686974,
173.157058062683));
#25499=CARTESIAN_POINT('Ctrl Pts',(-61.5992309516654,-99.6219612498133,
174.328630986959));
#25500=CARTESIAN_POINT('Ctrl Pts',(-61.5892928198112,-99.528739492507,175.985485236451));
#25501=CARTESIAN_POINT('Ctrl Pts',(-61.579354687957,-99.4355177352008,177.642339485944));
#25502=CARTESIAN_POINT('Ctrl Pts',(-60.4044449405234,-99.4664897351676,
178.813912312176));
#25503=CARTESIAN_POINT('Ctrl Pts',(-59.2295351930898,-99.4974617351344,
179.985485138407));
#25504=CARTESIAN_POINT('Ctrl Pts',(-57.5720784430859,-99.5798764694207,
179.985485069079));
#25505=CARTESIAN_POINT('Ctrl Pts',(-55.914621693082,-99.662291203707,179.985484999752));
#25506=CARTESIAN_POINT('Ctrl Pts',(-54.7397120431402,-99.6932631932805,
178.813912075476));
#25507=CARTESIAN_POINT('Ctrl Pts',(-53.5648023931984,-99.724235182854,177.6423391512));
#25508=CARTESIAN_POINT('Ctrl Pts',(-53.5548643992186,-99.6310134108495,
175.985484901707));
#25509=CARTESIAN_POINT('Ctrl Pts',(-53.5449264052387,-99.5377916388449,
174.328630652215));
#25510=CARTESIAN_POINT('Ctrl Pts',(-54.6999600268383,-99.3203761095675,
173.157057825983));
#25511=CARTESIAN_POINT('Ctrl Pts',(-55.8549936484379,-99.10296058029,171.985484999752));
#25512=CARTESIAN_POINT('Ctrl Pts',(-57.4925742726078,-98.834102316693,171.985485069079));
#25513=CARTESIAN_POINT('Ctrl Pts',(-59.1301548967777,-98.5652440530961,
171.985485138407));
#25514=CARTESIAN_POINT('Ctrl Pts',(-60.2851884208854,-98.3478285342118,
173.157058062683));
#25515=CARTESIAN_POINT('Ctrl Pts',(-61.4402219449932,-98.1304130153276,
174.328630986959));
#25516=CARTESIAN_POINT('Ctrl Pts',(-61.430283813139,-98.0371912580215,175.985485236451));
#25517=CARTESIAN_POINT('Ctrl Pts',(-61.4203456812848,-97.9439695007152,
177.642339485944));
#25518=CARTESIAN_POINT('Ctrl Pts',(-60.2454359338512,-97.974941500682,178.813912312176));
#25519=CARTESIAN_POINT('Ctrl Pts',(-59.0705261864175,-98.0059135006488,
179.985485138407));
#25520=CARTESIAN_POINT('Ctrl Pts',(-57.4130694364136,-98.0883282349351,
179.985485069079));
#25521=CARTESIAN_POINT('Ctrl Pts',(-55.7556126864097,-98.1707429692214,
179.985484999752));
#25522=CARTESIAN_POINT('Ctrl Pts',(-54.580703036468,-98.2017149587949,178.813912075476));
#25523=CARTESIAN_POINT('Ctrl Pts',(-56.181115489574,-113.283598570176,178.821287383467));
#25524=CARTESIAN_POINT('Ctrl Pts',(-55.0031681001975,-113.314894403068,
177.646659506339));
#25525=CARTESIAN_POINT('Ctrl Pts',(-54.9932301063974,-113.221672631044,
175.985484901271));
#25526=CARTESIAN_POINT('Ctrl Pts',(-54.9832921125973,-113.12845085902,174.324310296203));
#25527=CARTESIAN_POINT('Ctrl Pts',(-56.1413634738858,-112.910711486397,
173.149682517375));
#25528=CARTESIAN_POINT('Ctrl Pts',(-57.2994348351743,-112.692972113774,
171.975054738546));
#25529=CARTESIAN_POINT('Ctrl Pts',(-58.9413114718314,-112.423655866545,
171.975054808055));
#25530=CARTESIAN_POINT('Ctrl Pts',(-60.5831881084886,-112.154339619316,
171.975054877564));
#25531=CARTESIAN_POINT('Ctrl Pts',(-61.741259372031,-111.936600257113,173.149682754692));
#25532=CARTESIAN_POINT('Ctrl Pts',(-62.8993306355734,-111.71886089491,174.32431063182));
#25533=CARTESIAN_POINT('Ctrl Pts',(-62.8893925035395,-111.625639137623,
175.985485236888));
#25534=CARTESIAN_POINT('Ctrl Pts',(-62.8794543715055,-111.532417380336,
177.646659841956));
#25535=CARTESIAN_POINT('Ctrl Pts',(-61.701506884383,-111.563713223648,178.821287620784));
#25536=CARTESIAN_POINT('Ctrl Pts',(-60.5235593972605,-111.595009066961,
179.995915399612));
#25537=CARTESIAN_POINT('Ctrl Pts',(-58.8618066347693,-111.677881784879,
179.995915330104));
#25538=CARTESIAN_POINT('Ctrl Pts',(-57.2000538722782,-111.760754502798,
179.995915260595));
#25539=CARTESIAN_POINT('Ctrl Pts',(-56.0221064829017,-111.79205033569,178.821287383467));
#25540=CARTESIAN_POINT('Ctrl Pts',(-54.8441590935253,-111.823346168582,
177.646659506339));
#25541=CARTESIAN_POINT('Ctrl Pts',(-54.8342210997252,-111.730124396559,
175.985484901271));
#25542=CARTESIAN_POINT('Ctrl Pts',(-54.8242831059251,-111.636902624535,
174.324310296203));
#25543=CARTESIAN_POINT('Ctrl Pts',(-55.9823544672136,-111.419163251912,
173.149682517375));
#25544=CARTESIAN_POINT('Ctrl Pts',(-57.1404258285021,-111.201423879289,
171.975054738546));
#25545=CARTESIAN_POINT('Ctrl Pts',(-58.7823024651592,-110.932107632059,
171.975054808055));
#25546=CARTESIAN_POINT('Ctrl Pts',(-60.4241791018163,-110.66279138483,171.975054877564));
#25547=CARTESIAN_POINT('Ctrl Pts',(-61.5822503653587,-110.445052022627,
173.149682754692));
#25548=CARTESIAN_POINT('Ctrl Pts',(-62.7403216289012,-110.227312660424,
174.32431063182));
#25549=CARTESIAN_POINT('Ctrl Pts',(-62.7303834968672,-110.134090903137,
175.985485236888));
#25550=CARTESIAN_POINT('Ctrl Pts',(-62.7204453648333,-110.04086914585,177.646659841956));
#25551=CARTESIAN_POINT('Ctrl Pts',(-61.5424978777108,-110.072164989163,
178.821287620784));
#25552=CARTESIAN_POINT('Ctrl Pts',(-60.3645503905882,-110.103460832475,
179.995915399612));
#25553=CARTESIAN_POINT('Ctrl Pts',(-58.7027976280971,-110.186333550394,
179.995915330104));
#25554=CARTESIAN_POINT('Ctrl Pts',(-57.041044865606,-110.269206268313,179.995915260595));
#25555=CARTESIAN_POINT('Ctrl Pts',(-55.8630974762295,-110.300502101205,
178.821287383467));
#25556=CARTESIAN_POINT('Ctrl Pts',(-54.6851500868531,-110.331797934097,
177.646659506339));
#25557=CARTESIAN_POINT('Ctrl Pts',(-54.675212093053,-110.238576162073,175.985484901271));
#25558=CARTESIAN_POINT('Ctrl Pts',(-54.6652740992529,-110.145354390049,
174.324310296203));
#25559=CARTESIAN_POINT('Ctrl Pts',(-55.8233454605414,-109.927615017426,
173.149682517375));
#25560=CARTESIAN_POINT('Ctrl Pts',(-56.9814168218299,-109.709875644803,
171.975054738546));
#25561=CARTESIAN_POINT('Ctrl Pts',(-58.623293458487,-109.440559397574,171.975054808055));
#25562=CARTESIAN_POINT('Ctrl Pts',(-60.2651700951441,-109.171243150344,
171.975054877564));
#25563=CARTESIAN_POINT('Ctrl Pts',(-61.4232413586865,-108.953503788142,
173.149682754692));
#25564=CARTESIAN_POINT('Ctrl Pts',(-62.581312622229,-108.735764425939,174.32431063182));
#25565=CARTESIAN_POINT('Ctrl Pts',(-62.571374490195,-108.642542668652,175.985485236888));
#25566=CARTESIAN_POINT('Ctrl Pts',(-62.5614363581611,-108.549320911365,
177.646659841956));
#25567=CARTESIAN_POINT('Ctrl Pts',(-61.3834888710385,-108.580616754677,
178.821287620784));
#25568=CARTESIAN_POINT('Ctrl Pts',(-60.205541383916,-108.61191259799,179.995915399612));
#25569=CARTESIAN_POINT('Ctrl Pts',(-58.5437886214249,-108.694785315908,
179.995915330104));
#25570=CARTESIAN_POINT('Ctrl Pts',(-56.8820358589338,-108.777658033827,
179.995915260595));
#25571=CARTESIAN_POINT('Ctrl Pts',(-55.7040884695573,-108.808953866719,
178.821287383467));
#25572=CARTESIAN_POINT('Ctrl Pts',(-54.5261410801808,-108.840249699611,
177.646659506339));
#25573=CARTESIAN_POINT('Ctrl Pts',(-54.5162030863807,-108.747027927587,
175.985484901271));
#25574=CARTESIAN_POINT('Ctrl Pts',(-54.5062650925806,-108.653806155564,
174.324310296203));
#25575=CARTESIAN_POINT('Ctrl Pts',(-55.6643364538691,-108.436066782941,
173.149682517375));
#25576=CARTESIAN_POINT('Ctrl Pts',(-56.8224078151577,-108.218327410317,
171.975054738546));
#25577=CARTESIAN_POINT('Ctrl Pts',(-58.4642844518147,-107.949011163088,
171.975054808055));
#25578=CARTESIAN_POINT('Ctrl Pts',(-60.1061610884719,-107.679694915859,
171.975054877564));
#25579=CARTESIAN_POINT('Ctrl Pts',(-61.2642323520143,-107.461955553656,
173.149682754692));
#25580=CARTESIAN_POINT('Ctrl Pts',(-62.4223036155567,-107.244216191453,
174.32431063182));
#25581=CARTESIAN_POINT('Ctrl Pts',(-62.4123654835228,-107.150994434166,
175.985485236888));
#25582=CARTESIAN_POINT('Ctrl Pts',(-62.4024273514889,-107.057772676879,
177.646659841956));
#25583=CARTESIAN_POINT('Ctrl Pts',(-61.2244798643663,-107.089068520192,
178.821287620784));
#25584=CARTESIAN_POINT('Ctrl Pts',(-60.0465323772438,-107.120364363504,
179.995915399612));
#25585=CARTESIAN_POINT('Ctrl Pts',(-58.3847796147526,-107.203237081423,
179.995915330104));
#25586=CARTESIAN_POINT('Ctrl Pts',(-56.7230268522615,-107.286109799341,
179.995915260595));
#25587=CARTESIAN_POINT('Ctrl Pts',(-55.5450794628851,-107.317405632233,
178.821287383467));
#25588=CARTESIAN_POINT('Ctrl Pts',(-54.3671320735086,-107.348701465125,
177.646659506339));
#25589=CARTESIAN_POINT('Ctrl Pts',(-54.3571940797085,-107.255479693102,
175.985484901271));
#25590=CARTESIAN_POINT('Ctrl Pts',(-54.3472560859084,-107.162257921078,
174.324310296203));
#25591=CARTESIAN_POINT('Ctrl Pts',(-55.5053274471969,-106.944518548455,
173.149682517375));
#25592=CARTESIAN_POINT('Ctrl Pts',(-56.6633988084854,-106.726779175832,
171.975054738546));
#25593=CARTESIAN_POINT('Ctrl Pts',(-58.3052754451425,-106.457462928602,
171.975054808055));
#25594=CARTESIAN_POINT('Ctrl Pts',(-59.9471520817997,-106.188146681373,
171.975054877564));
#25595=CARTESIAN_POINT('Ctrl Pts',(-61.1052233453421,-105.97040731917,173.149682754692));
#25596=CARTESIAN_POINT('Ctrl Pts',(-62.2632946088845,-105.752667956968,
174.32431063182));
#25597=CARTESIAN_POINT('Ctrl Pts',(-62.2533564768505,-105.659446199681,
175.985485236888));
#25598=CARTESIAN_POINT('Ctrl Pts',(-62.2434183448166,-105.566224442394,
177.646659841956));
#25599=CARTESIAN_POINT('Ctrl Pts',(-61.0654708576941,-105.597520285706,
178.821287620784));
#25600=CARTESIAN_POINT('Ctrl Pts',(-59.8875233705716,-105.628816129018,
179.995915399612));
#25601=CARTESIAN_POINT('Ctrl Pts',(-58.2257706080804,-105.711688846937,
179.995915330104));
#25602=CARTESIAN_POINT('Ctrl Pts',(-56.5640178455893,-105.794561564856,
179.995915260595));
#25603=CARTESIAN_POINT('Ctrl Pts',(-55.3860704562128,-105.825857397748,
178.821287383467));
#25604=CARTESIAN_POINT('Ctrl Pts',(-54.2081230668364,-105.85715323064,177.646659506339));
#25605=CARTESIAN_POINT('Ctrl Pts',(-54.1981850730363,-105.763931458616,
175.985484901271));
#25606=CARTESIAN_POINT('Ctrl Pts',(-54.1882470792362,-105.670709686593,
174.324310296203));
#25607=CARTESIAN_POINT('Ctrl Pts',(-55.3463184405247,-105.452970313969,
173.149682517375));
#25608=CARTESIAN_POINT('Ctrl Pts',(-56.5043898018132,-105.235230941346,
171.975054738546));
#25609=CARTESIAN_POINT('Ctrl Pts',(-58.1462664384703,-104.965914694117,
171.975054808055));
#25610=CARTESIAN_POINT('Ctrl Pts',(-59.7881430751274,-104.696598446888,
171.975054877564));
#25611=CARTESIAN_POINT('Ctrl Pts',(-60.9462143386698,-104.478859084685,
173.149682754692));
#25612=CARTESIAN_POINT('Ctrl Pts',(-62.1042856022123,-104.261119722482,
174.32431063182));
#25613=CARTESIAN_POINT('Ctrl Pts',(-62.0943474701783,-104.167897965195,
175.985485236888));
#25614=CARTESIAN_POINT('Ctrl Pts',(-62.0844093381444,-104.074676207908,
177.646659841956));
#25615=CARTESIAN_POINT('Ctrl Pts',(-60.9064618510219,-104.10597205122,178.821287620784));
#25616=CARTESIAN_POINT('Ctrl Pts',(-59.7285143638993,-104.137267894533,
179.995915399612));
#25617=CARTESIAN_POINT('Ctrl Pts',(-58.0667616014082,-104.220140612451,
179.995915330104));
#25618=CARTESIAN_POINT('Ctrl Pts',(-56.4050088389171,-104.30301333037,179.995915260595));
#25619=CARTESIAN_POINT('Ctrl Pts',(-55.2270614495406,-104.334309163262,
178.821287383467));
#25620=CARTESIAN_POINT('Ctrl Pts',(-54.0491140601642,-104.365604996154,
177.646659506339));
#25621=CARTESIAN_POINT('Ctrl Pts',(-54.039176066364,-104.272383224131,175.985484901271));
#25622=CARTESIAN_POINT('Ctrl Pts',(-54.029238072564,-104.179161452107,174.324310296203));
#25623=CARTESIAN_POINT('Ctrl Pts',(-55.1873094338524,-103.961422079484,
173.149682517375));
#25624=CARTESIAN_POINT('Ctrl Pts',(-56.345380795141,-103.743682706861,171.975054738546));
#25625=CARTESIAN_POINT('Ctrl Pts',(-57.9872574317981,-103.474366459631,
171.975054808055));
#25626=CARTESIAN_POINT('Ctrl Pts',(-59.6291340684552,-103.205050212402,
171.975054877564));
#25627=CARTESIAN_POINT('Ctrl Pts',(-60.7872053319976,-102.987310850199,
173.149682754692));
#25628=CARTESIAN_POINT('Ctrl Pts',(-61.94527659554,-102.769571487996,174.32431063182));
#25629=CARTESIAN_POINT('Ctrl Pts',(-61.9353384635061,-102.676349730709,
175.985485236888));
#25630=CARTESIAN_POINT('Ctrl Pts',(-61.9254003314722,-102.583127973422,
177.646659841956));
#25631=CARTESIAN_POINT('Ctrl Pts',(-60.7474528443496,-102.614423816735,
178.821287620784));
#25632=CARTESIAN_POINT('Ctrl Pts',(-59.5695053572271,-102.645719660047,
179.995915399612));
#25633=CARTESIAN_POINT('Ctrl Pts',(-57.907752594736,-102.728592377966,179.995915330104));
#25634=CARTESIAN_POINT('Ctrl Pts',(-56.2459998322448,-102.811465095885,
179.995915260595));
#25635=CARTESIAN_POINT('Ctrl Pts',(-55.0680524428684,-102.842760928777,
178.821287383467));
#25636=CARTESIAN_POINT('Ctrl Pts',(-53.8901050534919,-102.874056761669,
177.646659506339));
#25637=CARTESIAN_POINT('Ctrl Pts',(-53.8801670596918,-102.780834989645,
175.985484901271));
#25638=CARTESIAN_POINT('Ctrl Pts',(-53.8702290658917,-102.687613217621,
174.324310296203));
#25639=CARTESIAN_POINT('Ctrl Pts',(-55.0283004271802,-102.469873844998,
173.149682517375));
#25640=CARTESIAN_POINT('Ctrl Pts',(-56.1863717884687,-102.252134472375,
171.975054738546));
#25641=CARTESIAN_POINT('Ctrl Pts',(-57.8282484251258,-101.982818225146,
171.975054808055));
#25642=CARTESIAN_POINT('Ctrl Pts',(-59.470125061783,-101.713501977916,171.975054877564));
#25643=CARTESIAN_POINT('Ctrl Pts',(-60.6281963253254,-101.495762615714,
173.149682754692));
#25644=CARTESIAN_POINT('Ctrl Pts',(-61.7862675888678,-101.278023253511,
174.32431063182));
#25645=CARTESIAN_POINT('Ctrl Pts',(-61.7763294568339,-101.184801496224,
175.985485236888));
#25646=CARTESIAN_POINT('Ctrl Pts',(-61.7663913247999,-101.091579738937,
177.646659841956));
#25647=CARTESIAN_POINT('Ctrl Pts',(-60.5884438376774,-101.122875582249,
178.821287620784));
#25648=CARTESIAN_POINT('Ctrl Pts',(-59.4104963505549,-101.154171425562,
179.995915399612));
#25649=CARTESIAN_POINT('Ctrl Pts',(-57.7487435880637,-101.23704414348,179.995915330104));
#25650=CARTESIAN_POINT('Ctrl Pts',(-56.0869908255726,-101.319916861399,
179.995915260595));
#25651=CARTESIAN_POINT('Ctrl Pts',(-54.9090434361961,-101.351212694291,
178.821287383467));
#25652=CARTESIAN_POINT('Ctrl Pts',(-53.7310960468197,-101.382508527183,
177.646659506339));
#25653=CARTESIAN_POINT('Ctrl Pts',(-53.7211580530196,-101.289286755159,
175.985484901271));
#25654=CARTESIAN_POINT('Ctrl Pts',(-53.7112200592195,-101.196064983136,
174.324310296203));
#25655=CARTESIAN_POINT('Ctrl Pts',(-54.869291420508,-100.978325610513,173.149682517375));
#25656=CARTESIAN_POINT('Ctrl Pts',(-56.0273627817965,-100.760586237889,
171.975054738546));
#25657=CARTESIAN_POINT('Ctrl Pts',(-57.6692394184536,-100.49126999066,171.975054808055));
#25658=CARTESIAN_POINT('Ctrl Pts',(-59.3111160551107,-100.221953743431,
171.975054877564));
#25659=CARTESIAN_POINT('Ctrl Pts',(-60.4691873186531,-100.004214381228,
173.149682754692));
#25660=CARTESIAN_POINT('Ctrl Pts',(-61.6272585821956,-99.7864750190253,
174.32431063182));
#25661=CARTESIAN_POINT('Ctrl Pts',(-61.6173204501616,-99.6932532617382,
175.985485236888));
#25662=CARTESIAN_POINT('Ctrl Pts',(-61.6073823181277,-99.6000315044512,
177.646659841956));
#25663=CARTESIAN_POINT('Ctrl Pts',(-60.4294348310052,-99.6313273477637,
178.821287620784));
#25664=CARTESIAN_POINT('Ctrl Pts',(-59.2514873438827,-99.6626231910761,
179.995915399612));
#25665=CARTESIAN_POINT('Ctrl Pts',(-57.5897345813915,-99.7454959089947,
179.995915330104));
#25666=CARTESIAN_POINT('Ctrl Pts',(-55.9279818189004,-99.8283686269133,
179.995915260595));
#25667=CARTESIAN_POINT('Ctrl Pts',(-54.7500344295239,-99.8596644598054,
178.821287383467));
#25668=CARTESIAN_POINT('Ctrl Pts',(-53.5720870401475,-99.8909602926975,
177.646659506339));
#25669=CARTESIAN_POINT('Ctrl Pts',(-53.5621490463474,-99.7977385206737,
175.985484901271));
#25670=CARTESIAN_POINT('Ctrl Pts',(-53.5522110525473,-99.7045167486501,
174.324310296203));
#25671=CARTESIAN_POINT('Ctrl Pts',(-54.7102824138358,-99.4867773760269,
173.149682517375));
#25672=CARTESIAN_POINT('Ctrl Pts',(-55.8683537751243,-99.2690380034038,
171.975054738546));
#25673=CARTESIAN_POINT('Ctrl Pts',(-57.5102304117814,-98.9997217561745,
171.975054808055));
#25674=CARTESIAN_POINT('Ctrl Pts',(-59.1521070484385,-98.7304055089452,
171.975054877564));
#25675=CARTESIAN_POINT('Ctrl Pts',(-60.3101783119809,-98.5126661467424,
173.149682754692));
#25676=CARTESIAN_POINT('Ctrl Pts',(-61.4682495755234,-98.2949267845397,
174.32431063182));
#25677=CARTESIAN_POINT('Ctrl Pts',(-61.4583114434894,-98.2017050272526,
175.985485236888));
#25678=CARTESIAN_POINT('Ctrl Pts',(-61.4483733114555,-98.1084832699656,
177.646659841956));
#25679=CARTESIAN_POINT('Ctrl Pts',(-60.2704258243329,-98.139779113278,178.821287620784));
#25680=CARTESIAN_POINT('Ctrl Pts',(-59.0924783372104,-98.1710749565905,
179.995915399612));
#25681=CARTESIAN_POINT('Ctrl Pts',(-57.4307255747193,-98.2539476745091,
179.995915330104));
#25682=CARTESIAN_POINT('Ctrl Pts',(-55.7689728122282,-98.3368203924277,
179.995915260595));
#25683=CARTESIAN_POINT('Ctrl Pts',(-54.5910254228517,-98.3681162253198,
178.821287383467));
#25684=CARTESIAN_POINT('Ctrl Pts',(-56.1988062143188,-113.449542435949,
178.821287383467));
#25685=CARTESIAN_POINT('Ctrl Pts',(-55.0208588249424,-113.480838268841,
177.646659506339));
#25686=CARTESIAN_POINT('Ctrl Pts',(-55.0109208311422,-113.387616496817,
175.985484901271));
#25687=CARTESIAN_POINT('Ctrl Pts',(-55.0009828373422,-113.294394724794,
174.324310296203));
#25688=CARTESIAN_POINT('Ctrl Pts',(-56.1590541986307,-113.07665535217,173.149682517375));
#25689=CARTESIAN_POINT('Ctrl Pts',(-57.3171255599192,-112.858915979547,
171.975054738546));
#25690=CARTESIAN_POINT('Ctrl Pts',(-58.9590021965763,-112.589599732318,
171.975054808055));
#25691=CARTESIAN_POINT('Ctrl Pts',(-60.6008788332334,-112.320283485089,
171.975054877564));
#25692=CARTESIAN_POINT('Ctrl Pts',(-61.7589500967758,-112.102544122886,
173.149682754692));
#25693=CARTESIAN_POINT('Ctrl Pts',(-62.9170213603182,-111.884804760683,
174.32431063182));
#25694=CARTESIAN_POINT('Ctrl Pts',(-62.9070832282843,-111.791583003396,
175.985485236888));
#25695=CARTESIAN_POINT('Ctrl Pts',(-62.8971450962504,-111.698361246109,
177.646659841956));
#25696=CARTESIAN_POINT('Ctrl Pts',(-61.7191976091278,-111.729657089422,
178.821287620784));
#25697=CARTESIAN_POINT('Ctrl Pts',(-60.5412501220053,-111.760952932734,
179.995915399612));
#25698=CARTESIAN_POINT('Ctrl Pts',(-58.8794973595142,-111.843825650653,
179.995915330104));
#25699=CARTESIAN_POINT('Ctrl Pts',(-57.217744597023,-111.926698368571,179.995915260595));
#25700=CARTESIAN_POINT('Ctrl Pts',(-56.0397972076466,-111.957994201463,
178.821287383467));
#25701=CARTESIAN_POINT('Ctrl Pts',(-54.8618498182701,-111.989290034355,
177.646659506339));
#25702=CARTESIAN_POINT('Ctrl Pts',(-54.85191182447,-111.896068262332,175.985484901271));
#25703=CARTESIAN_POINT('Ctrl Pts',(-54.8419738306699,-111.802846490308,
174.324310296203));
#25704=CARTESIAN_POINT('Ctrl Pts',(-56.0000451919584,-111.585107117685,
173.149682517375));
#25705=CARTESIAN_POINT('Ctrl Pts',(-57.158116553247,-111.367367745062,171.975054738546));
#25706=CARTESIAN_POINT('Ctrl Pts',(-58.799993189904,-111.098051497832,171.975054808055));
#25707=CARTESIAN_POINT('Ctrl Pts',(-60.4418698265612,-110.828735250603,
171.975054877564));
#25708=CARTESIAN_POINT('Ctrl Pts',(-61.5999410901036,-110.6109958884,173.149682754692));
#25709=CARTESIAN_POINT('Ctrl Pts',(-62.758012353646,-110.393256526198,174.32431063182));
#25710=CARTESIAN_POINT('Ctrl Pts',(-62.7480742216121,-110.30003476891,175.985485236888));
#25711=CARTESIAN_POINT('Ctrl Pts',(-62.7381360895782,-110.206813011623,
177.646659841956));
#25712=CARTESIAN_POINT('Ctrl Pts',(-61.5601886024556,-110.238108854936,
178.821287620784));
#25713=CARTESIAN_POINT('Ctrl Pts',(-60.3822411153331,-110.269404698248,
179.995915399612));
#25714=CARTESIAN_POINT('Ctrl Pts',(-58.7204883528419,-110.352277416167,
179.995915330104));
#25715=CARTESIAN_POINT('Ctrl Pts',(-57.0587355903508,-110.435150134086,
179.995915260595));
#25716=CARTESIAN_POINT('Ctrl Pts',(-55.8807882009743,-110.466445966978,
178.821287383467));
#25717=CARTESIAN_POINT('Ctrl Pts',(-54.7028408115979,-110.49774179987,177.646659506339));
#25718=CARTESIAN_POINT('Ctrl Pts',(-54.6929028177978,-110.404520027846,
175.985484901271));
#25719=CARTESIAN_POINT('Ctrl Pts',(-54.6829648239977,-110.311298255822,
174.324310296203));
#25720=CARTESIAN_POINT('Ctrl Pts',(-55.8410361852862,-110.093558883199,
173.149682517375));
#25721=CARTESIAN_POINT('Ctrl Pts',(-56.9991075465747,-109.875819510576,
171.975054738546));
#25722=CARTESIAN_POINT('Ctrl Pts',(-58.6409841832318,-109.606503263347,
171.975054808055));
#25723=CARTESIAN_POINT('Ctrl Pts',(-60.2828608198889,-109.337187016117,
171.975054877564));
#25724=CARTESIAN_POINT('Ctrl Pts',(-61.4409320834313,-109.119447653915,
173.149682754692));
#25725=CARTESIAN_POINT('Ctrl Pts',(-62.5990033469738,-108.901708291712,
174.32431063182));
#25726=CARTESIAN_POINT('Ctrl Pts',(-62.5890652149398,-108.808486534425,
175.985485236888));
#25727=CARTESIAN_POINT('Ctrl Pts',(-62.5791270829059,-108.715264777138,
177.646659841956));
#25728=CARTESIAN_POINT('Ctrl Pts',(-61.4011795957834,-108.74656062045,178.821287620784));
#25729=CARTESIAN_POINT('Ctrl Pts',(-60.2232321086609,-108.777856463763,
179.995915399612));
#25730=CARTESIAN_POINT('Ctrl Pts',(-58.5614793461697,-108.860729181681,
179.995915330104));
#25731=CARTESIAN_POINT('Ctrl Pts',(-56.8997265836786,-108.9436018996,179.995915260595));
#25732=CARTESIAN_POINT('Ctrl Pts',(-55.7217791943021,-108.974897732492,
178.821287383467));
#25733=CARTESIAN_POINT('Ctrl Pts',(-54.5438318049257,-109.006193565384,
177.646659506339));
#25734=CARTESIAN_POINT('Ctrl Pts',(-54.5338938111256,-108.91297179336,175.985484901271));
#25735=CARTESIAN_POINT('Ctrl Pts',(-54.5239558173255,-108.819750021337,
174.324310296203));
#25736=CARTESIAN_POINT('Ctrl Pts',(-55.682027178614,-108.602010648714,173.149682517375));
#25737=CARTESIAN_POINT('Ctrl Pts',(-56.8400985399025,-108.384271276091,
171.975054738546));
#25738=CARTESIAN_POINT('Ctrl Pts',(-58.4819751765596,-108.114955028861,
171.975054808055));
#25739=CARTESIAN_POINT('Ctrl Pts',(-60.1238518132167,-107.845638781632,
171.975054877564));
#25740=CARTESIAN_POINT('Ctrl Pts',(-61.2819230767591,-107.627899419429,
173.149682754692));
#25741=CARTESIAN_POINT('Ctrl Pts',(-62.4399943403016,-107.410160057226,
174.32431063182));
#25742=CARTESIAN_POINT('Ctrl Pts',(-62.4300562082676,-107.316938299939,
175.985485236888));
#25743=CARTESIAN_POINT('Ctrl Pts',(-62.4201180762337,-107.223716542652,
177.646659841956));
#25744=CARTESIAN_POINT('Ctrl Pts',(-61.2421705891111,-107.255012385965,
178.821287620784));
#25745=CARTESIAN_POINT('Ctrl Pts',(-60.0642231019886,-107.286308229277,
179.995915399612));
#25746=CARTESIAN_POINT('Ctrl Pts',(-58.4024703394975,-107.369180947196,
179.995915330104));
#25747=CARTESIAN_POINT('Ctrl Pts',(-56.7407175770064,-107.452053665114,
179.995915260595));
#25748=CARTESIAN_POINT('Ctrl Pts',(-55.5627701876299,-107.483349498006,
178.821287383467));
#25749=CARTESIAN_POINT('Ctrl Pts',(-54.3848227982534,-107.514645330899,
177.646659506339));
#25750=CARTESIAN_POINT('Ctrl Pts',(-54.3748848044533,-107.421423558875,
175.985484901271));
#25751=CARTESIAN_POINT('Ctrl Pts',(-54.3649468106533,-107.328201786851,
174.324310296203));
#25752=CARTESIAN_POINT('Ctrl Pts',(-55.5230181719417,-107.110462414228,
173.149682517375));
#25753=CARTESIAN_POINT('Ctrl Pts',(-56.6810895332303,-106.892723041605,
171.975054738546));
#25754=CARTESIAN_POINT('Ctrl Pts',(-58.3229661698874,-106.623406794376,
171.975054808055));
#25755=CARTESIAN_POINT('Ctrl Pts',(-59.9648428065445,-106.354090547146,
171.975054877564));
#25756=CARTESIAN_POINT('Ctrl Pts',(-61.1229140700869,-106.136351184943,
173.149682754692));
#25757=CARTESIAN_POINT('Ctrl Pts',(-62.2809853336293,-105.918611822741,
174.32431063182));
#25758=CARTESIAN_POINT('Ctrl Pts',(-62.2710472015954,-105.825390065454,
175.985485236888));
#25759=CARTESIAN_POINT('Ctrl Pts',(-62.2611090695615,-105.732168308167,
177.646659841956));
#25760=CARTESIAN_POINT('Ctrl Pts',(-61.0831615824389,-105.763464151479,
178.821287620784));
#25761=CARTESIAN_POINT('Ctrl Pts',(-59.9052140953164,-105.794759994792,
179.995915399612));
#25762=CARTESIAN_POINT('Ctrl Pts',(-58.2434613328252,-105.87763271271,179.995915330104));
#25763=CARTESIAN_POINT('Ctrl Pts',(-56.5817085703341,-105.960505430629,
179.995915260595));
#25764=CARTESIAN_POINT('Ctrl Pts',(-55.4037611809577,-105.991801263521,
178.821287383467));
#25765=CARTESIAN_POINT('Ctrl Pts',(-54.2258137915812,-106.023097096413,
177.646659506339));
#25766=CARTESIAN_POINT('Ctrl Pts',(-54.2158757977811,-105.929875324389,
175.985484901271));
#25767=CARTESIAN_POINT('Ctrl Pts',(-54.205937803981,-105.836653552366,174.324310296203));
#25768=CARTESIAN_POINT('Ctrl Pts',(-55.3640091652695,-105.618914179742,
173.149682517375));
#25769=CARTESIAN_POINT('Ctrl Pts',(-56.522080526558,-105.401174807119,171.975054738546));
#25770=CARTESIAN_POINT('Ctrl Pts',(-58.1639571632151,-105.13185855989,171.975054808055));
#25771=CARTESIAN_POINT('Ctrl Pts',(-59.8058337998722,-104.862542312661,
171.975054877564));
#25772=CARTESIAN_POINT('Ctrl Pts',(-60.9639050634147,-104.644802950458,
173.149682754692));
#25773=CARTESIAN_POINT('Ctrl Pts',(-62.1219763269571,-104.427063588255,
174.32431063182));
#25774=CARTESIAN_POINT('Ctrl Pts',(-62.1120381949232,-104.333841830968,
175.985485236888));
#25775=CARTESIAN_POINT('Ctrl Pts',(-62.1021000628892,-104.240620073681,
177.646659841956));
#25776=CARTESIAN_POINT('Ctrl Pts',(-60.9241525757667,-104.271915916993,
178.821287620784));
#25777=CARTESIAN_POINT('Ctrl Pts',(-59.7462050886442,-104.303211760306,
179.995915399612));
#25778=CARTESIAN_POINT('Ctrl Pts',(-58.084452326153,-104.386084478225,179.995915330104));
#25779=CARTESIAN_POINT('Ctrl Pts',(-56.4226995636619,-104.468957196143,
179.995915260595));
#25780=CARTESIAN_POINT('Ctrl Pts',(-55.2447521742854,-104.500253029035,
178.821287383467));
#25781=CARTESIAN_POINT('Ctrl Pts',(-54.066804784909,-104.531548861927,177.646659506339));
#25782=CARTESIAN_POINT('Ctrl Pts',(-54.0568667911089,-104.438327089904,
175.985484901271));
#25783=CARTESIAN_POINT('Ctrl Pts',(-54.0469287973088,-104.34510531788,174.324310296203));
#25784=CARTESIAN_POINT('Ctrl Pts',(-55.2050001585973,-104.127365945257,
173.149682517375));
#25785=CARTESIAN_POINT('Ctrl Pts',(-56.3630715198858,-103.909626572634,
171.975054738546));
#25786=CARTESIAN_POINT('Ctrl Pts',(-58.0049481565429,-103.640310325404,
171.975054808055));
#25787=CARTESIAN_POINT('Ctrl Pts',(-59.6468247932,-103.370994078175,171.975054877564));
#25788=CARTESIAN_POINT('Ctrl Pts',(-60.8048960567424,-103.153254715972,
173.149682754692));
#25789=CARTESIAN_POINT('Ctrl Pts',(-61.9629673202849,-102.93551535377,174.32431063182));
#25790=CARTESIAN_POINT('Ctrl Pts',(-61.9530291882509,-102.842293596483,
175.985485236888));
#25791=CARTESIAN_POINT('Ctrl Pts',(-61.943091056217,-102.749071839196,177.646659841956));
#25792=CARTESIAN_POINT('Ctrl Pts',(-60.7651435690945,-102.780367682508,
178.821287620784));
#25793=CARTESIAN_POINT('Ctrl Pts',(-59.587196081972,-102.81166352582,179.995915399612));
#25794=CARTESIAN_POINT('Ctrl Pts',(-57.9254433194808,-102.894536243739,
179.995915330104));
#25795=CARTESIAN_POINT('Ctrl Pts',(-56.2636905569897,-102.977408961658,
179.995915260595));
#25796=CARTESIAN_POINT('Ctrl Pts',(-55.0857431676132,-103.00870479455,178.821287383467));
#25797=CARTESIAN_POINT('Ctrl Pts',(-53.9077957782368,-103.040000627442,
177.646659506339));
#25798=CARTESIAN_POINT('Ctrl Pts',(-53.8978577844367,-102.946778855418,
175.985484901271));
#25799=CARTESIAN_POINT('Ctrl Pts',(-53.8879197906366,-102.853557083394,
174.324310296203));
#25800=CARTESIAN_POINT('Ctrl Pts',(-55.0459911519251,-102.635817710771,
173.149682517375));
#25801=CARTESIAN_POINT('Ctrl Pts',(-56.2040625132136,-102.418078338148,
171.975054738546));
#25802=CARTESIAN_POINT('Ctrl Pts',(-57.8459391498707,-102.148762090919,
171.975054808055));
#25803=CARTESIAN_POINT('Ctrl Pts',(-59.4878157865278,-101.879445843689,
171.975054877564));
#25804=CARTESIAN_POINT('Ctrl Pts',(-60.6458870500702,-101.661706481487,
173.149682754692));
#25805=CARTESIAN_POINT('Ctrl Pts',(-61.8039583136126,-101.443967119284,
174.32431063182));
#25806=CARTESIAN_POINT('Ctrl Pts',(-61.7940201815787,-101.350745361997,
175.985485236888));
#25807=CARTESIAN_POINT('Ctrl Pts',(-61.7840820495448,-101.25752360471,177.646659841956));
#25808=CARTESIAN_POINT('Ctrl Pts',(-60.6061345624222,-101.288819448022,
178.821287620784));
#25809=CARTESIAN_POINT('Ctrl Pts',(-59.4281870752997,-101.320115291335,
179.995915399612));
#25810=CARTESIAN_POINT('Ctrl Pts',(-57.7664343128086,-101.402988009253,
179.995915330104));
#25811=CARTESIAN_POINT('Ctrl Pts',(-56.1046815503175,-101.485860727172,
179.995915260595));
#25812=CARTESIAN_POINT('Ctrl Pts',(-54.926734160941,-101.517156560064,178.821287383467));
#25813=CARTESIAN_POINT('Ctrl Pts',(-53.7487867715645,-101.548452392956,
177.646659506339));
#25814=CARTESIAN_POINT('Ctrl Pts',(-53.7388487777644,-101.455230620932,
175.985484901271));
#25815=CARTESIAN_POINT('Ctrl Pts',(-53.7289107839643,-101.362008848909,
174.324310296203));
#25816=CARTESIAN_POINT('Ctrl Pts',(-54.8869821452528,-101.144269476286,
173.149682517375));
#25817=CARTESIAN_POINT('Ctrl Pts',(-56.0450535065414,-100.926530103662,
171.975054738546));
#25818=CARTESIAN_POINT('Ctrl Pts',(-57.6869301431984,-100.657213856433,
171.975054808055));
#25819=CARTESIAN_POINT('Ctrl Pts',(-59.3288067798556,-100.387897609204,
171.975054877564));
#25820=CARTESIAN_POINT('Ctrl Pts',(-60.486878043398,-100.170158247001,173.149682754692));
#25821=CARTESIAN_POINT('Ctrl Pts',(-61.6449493069404,-99.9524188847983,
174.32431063182));
#25822=CARTESIAN_POINT('Ctrl Pts',(-61.6350111749065,-99.8591971275113,
175.985485236888));
#25823=CARTESIAN_POINT('Ctrl Pts',(-61.6250730428726,-99.7659753702243,
177.646659841956));
#25824=CARTESIAN_POINT('Ctrl Pts',(-60.44712555575,-99.7972712135367,178.821287620784));
#25825=CARTESIAN_POINT('Ctrl Pts',(-59.2691780686275,-99.8285670568492,
179.995915399612));
#25826=CARTESIAN_POINT('Ctrl Pts',(-57.6074253061363,-99.9114397747677,
179.995915330104));
#25827=CARTESIAN_POINT('Ctrl Pts',(-55.9456725436452,-99.9943124926864,
179.995915260595));
#25828=CARTESIAN_POINT('Ctrl Pts',(-54.7677251542687,-100.025608325578,
178.821287383467));
#25829=CARTESIAN_POINT('Ctrl Pts',(-53.5897777648923,-100.05690415847,177.646659506339));
#25830=CARTESIAN_POINT('Ctrl Pts',(-53.5798397710922,-99.9636823864468,
175.985484901271));
#25831=CARTESIAN_POINT('Ctrl Pts',(-53.5699017772921,-99.8704606144232,
174.324310296203));
#25832=CARTESIAN_POINT('Ctrl Pts',(-54.7279731385806,-99.6527212418,173.149682517375));
#25833=CARTESIAN_POINT('Ctrl Pts',(-55.8860444998691,-99.4349818691769,
171.975054738546));
#25834=CARTESIAN_POINT('Ctrl Pts',(-57.5279211365262,-99.1656656219475,
171.975054808055));
#25835=CARTESIAN_POINT('Ctrl Pts',(-59.1697977731833,-98.8963493747183,
171.975054877564));
#25836=CARTESIAN_POINT('Ctrl Pts',(-60.3278690367257,-98.6786100125155,
173.149682754692));
#25837=CARTESIAN_POINT('Ctrl Pts',(-61.4859403002682,-98.4608706503128,
174.32431063182));
#25838=CARTESIAN_POINT('Ctrl Pts',(-61.4760021682342,-98.3676488930257,
175.985485236888));
#25839=CARTESIAN_POINT('Ctrl Pts',(-61.4660640362003,-98.2744271357387,
177.646659841956));
#25840=CARTESIAN_POINT('Ctrl Pts',(-60.2881165490778,-98.3057229790511,
178.821287620784));
#25841=CARTESIAN_POINT('Ctrl Pts',(-59.1101690619552,-98.3370188223636,
179.995915399612));
#25842=CARTESIAN_POINT('Ctrl Pts',(-57.4484162994641,-98.4198915402821,
179.995915330104));
#25843=CARTESIAN_POINT('Ctrl Pts',(-55.786663536973,-98.5027642582008,179.995915260595));
#25844=CARTESIAN_POINT('Ctrl Pts',(-54.6087161475965,-98.5340600910929,
178.821287383467));
#25845=CARTESIAN_POINT('Ctrl Pts',(-56.2237961054143,-113.614380048479,
178.813912075476));
#25846=CARTESIAN_POINT('Ctrl Pts',(-55.0488864554725,-113.645352038053,
177.6423391512));
#25847=CARTESIAN_POINT('Ctrl Pts',(-55.0389484614927,-113.552130266048,
175.985484901707));
#25848=CARTESIAN_POINT('Ctrl Pts',(-55.0290104675128,-113.458908494044,
174.328630652215));
#25849=CARTESIAN_POINT('Ctrl Pts',(-56.1840440891124,-113.241492964766,
173.157057825983));
#25850=CARTESIAN_POINT('Ctrl Pts',(-57.3390777107121,-113.024077435489,
171.985484999752));
#25851=CARTESIAN_POINT('Ctrl Pts',(-58.9766583348819,-112.755219171892,
171.985485069079));
#25852=CARTESIAN_POINT('Ctrl Pts',(-60.6142389590518,-112.486360908295,
171.985485138407));
#25853=CARTESIAN_POINT('Ctrl Pts',(-61.7692724831595,-112.268945389411,
173.157058062683));
#25854=CARTESIAN_POINT('Ctrl Pts',(-62.9243060072673,-112.051529870527,
174.328630986959));
#25855=CARTESIAN_POINT('Ctrl Pts',(-62.9143678754131,-111.95830811322,175.985485236451));
#25856=CARTESIAN_POINT('Ctrl Pts',(-62.9044297435589,-111.865086355914,
177.642339485944));
#25857=CARTESIAN_POINT('Ctrl Pts',(-61.7295199961253,-111.896058355881,
178.813912312176));
#25858=CARTESIAN_POINT('Ctrl Pts',(-60.5546102486917,-111.927030355848,
179.985485138407));
#25859=CARTESIAN_POINT('Ctrl Pts',(-58.8971534986878,-112.009445090134,
179.985485069079));
#25860=CARTESIAN_POINT('Ctrl Pts',(-57.2396967486839,-112.09185982442,179.985484999752));
#25861=CARTESIAN_POINT('Ctrl Pts',(-56.0647870987421,-112.122831813994,
178.813912075476));
#25862=CARTESIAN_POINT('Ctrl Pts',(-54.8898774488003,-112.153803803567,
177.6423391512));
#25863=CARTESIAN_POINT('Ctrl Pts',(-54.8799394548205,-112.060582031563,
175.985484901707));
#25864=CARTESIAN_POINT('Ctrl Pts',(-54.8700014608406,-111.967360259558,
174.328630652215));
#25865=CARTESIAN_POINT('Ctrl Pts',(-56.0250350824402,-111.749944730281,
173.157057825983));
#25866=CARTESIAN_POINT('Ctrl Pts',(-57.1800687040398,-111.532529201003,
171.985484999752));
#25867=CARTESIAN_POINT('Ctrl Pts',(-58.8176493282097,-111.263670937406,
171.985485069079));
#25868=CARTESIAN_POINT('Ctrl Pts',(-60.4552299523796,-110.994812673809,
171.985485138407));
#25869=CARTESIAN_POINT('Ctrl Pts',(-61.6102634764873,-110.777397154925,
173.157058062683));
#25870=CARTESIAN_POINT('Ctrl Pts',(-62.7652970005951,-110.559981636041,
174.328630986959));
#25871=CARTESIAN_POINT('Ctrl Pts',(-62.7553588687409,-110.466759878735,
175.985485236451));
#25872=CARTESIAN_POINT('Ctrl Pts',(-62.7454207368867,-110.373538121429,
177.642339485944));
#25873=CARTESIAN_POINT('Ctrl Pts',(-61.5705109894531,-110.404510121395,
178.813912312176));
#25874=CARTESIAN_POINT('Ctrl Pts',(-60.3956012420194,-110.435482121362,
179.985485138407));
#25875=CARTESIAN_POINT('Ctrl Pts',(-58.7381444920155,-110.517896855648,
179.985485069079));
#25876=CARTESIAN_POINT('Ctrl Pts',(-57.0806877420116,-110.600311589935,
179.985484999752));
#25877=CARTESIAN_POINT('Ctrl Pts',(-55.9057780920699,-110.631283579508,
178.813912075476));
#25878=CARTESIAN_POINT('Ctrl Pts',(-54.7308684421281,-110.662255569082,
177.6423391512));
#25879=CARTESIAN_POINT('Ctrl Pts',(-54.7209304481482,-110.569033797077,
175.985484901707));
#25880=CARTESIAN_POINT('Ctrl Pts',(-54.7109924541684,-110.475812025073,
174.328630652215));
#25881=CARTESIAN_POINT('Ctrl Pts',(-55.866026075768,-110.258396495795,173.157057825983));
#25882=CARTESIAN_POINT('Ctrl Pts',(-57.0210596973676,-110.040980966518,
171.985484999752));
#25883=CARTESIAN_POINT('Ctrl Pts',(-58.6586403215375,-109.772122702921,
171.985485069079));
#25884=CARTESIAN_POINT('Ctrl Pts',(-60.2962209457073,-109.503264439324,
171.985485138407));
#25885=CARTESIAN_POINT('Ctrl Pts',(-61.4512544698151,-109.28584892044,173.157058062683));
#25886=CARTESIAN_POINT('Ctrl Pts',(-62.6062879939228,-109.068433401555,
174.328630986959));
#25887=CARTESIAN_POINT('Ctrl Pts',(-62.5963498620687,-108.975211644249,
175.985485236451));
#25888=CARTESIAN_POINT('Ctrl Pts',(-62.5864117302145,-108.881989886943,
177.642339485944));
#25889=CARTESIAN_POINT('Ctrl Pts',(-61.4115019827808,-108.91296188691,178.813912312176));
#25890=CARTESIAN_POINT('Ctrl Pts',(-60.2365922353472,-108.943933886877,
179.985485138407));
#25891=CARTESIAN_POINT('Ctrl Pts',(-58.5791354853433,-109.026348621163,
179.985485069079));
#25892=CARTESIAN_POINT('Ctrl Pts',(-56.9216787353394,-109.108763355449,
179.985484999752));
#25893=CARTESIAN_POINT('Ctrl Pts',(-55.7467690853976,-109.139735345023,
178.813912075476));
#25894=CARTESIAN_POINT('Ctrl Pts',(-54.5718594354559,-109.170707334596,
177.6423391512));
#25895=CARTESIAN_POINT('Ctrl Pts',(-54.561921441476,-109.077485562592,175.985484901707));
#25896=CARTESIAN_POINT('Ctrl Pts',(-54.5519834474962,-108.984263790587,
174.328630652215));
#25897=CARTESIAN_POINT('Ctrl Pts',(-55.7070170690958,-108.76684826131,173.157057825983));
#25898=CARTESIAN_POINT('Ctrl Pts',(-56.8620506906954,-108.549432732032,
171.985484999752));
#25899=CARTESIAN_POINT('Ctrl Pts',(-58.4996313148652,-108.280574468435,
171.985485069079));
#25900=CARTESIAN_POINT('Ctrl Pts',(-60.1372119390351,-108.011716204838,
171.985485138407));
#25901=CARTESIAN_POINT('Ctrl Pts',(-61.2922454631428,-107.794300685954,
173.157058062683));
#25902=CARTESIAN_POINT('Ctrl Pts',(-62.4472789872506,-107.57688516707,174.328630986959));
#25903=CARTESIAN_POINT('Ctrl Pts',(-62.4373408553964,-107.483663409764,
175.985485236451));
#25904=CARTESIAN_POINT('Ctrl Pts',(-62.4274027235423,-107.390441652457,
177.642339485944));
#25905=CARTESIAN_POINT('Ctrl Pts',(-61.2524929761086,-107.421413652424,
178.813912312176));
#25906=CARTESIAN_POINT('Ctrl Pts',(-60.077583228675,-107.452385652391,179.985485138407));
#25907=CARTESIAN_POINT('Ctrl Pts',(-58.4201264786711,-107.534800386677,
179.985485069079));
#25908=CARTESIAN_POINT('Ctrl Pts',(-56.7626697286672,-107.617215120964,
179.985484999752));
#25909=CARTESIAN_POINT('Ctrl Pts',(-55.5877600787254,-107.648187110537,
178.813912075476));
#25910=CARTESIAN_POINT('Ctrl Pts',(-54.4128504287836,-107.67915910011,177.6423391512));
#25911=CARTESIAN_POINT('Ctrl Pts',(-54.4029124348038,-107.585937328106,
175.985484901707));
#25912=CARTESIAN_POINT('Ctrl Pts',(-54.3929744408239,-107.492715556102,
174.328630652215));
#25913=CARTESIAN_POINT('Ctrl Pts',(-55.5480080624235,-107.275300026824,
173.157057825983));
#25914=CARTESIAN_POINT('Ctrl Pts',(-56.7030416840231,-107.057884497547,
171.985484999752));
#25915=CARTESIAN_POINT('Ctrl Pts',(-58.340622308193,-106.78902623395,171.985485069079));
#25916=CARTESIAN_POINT('Ctrl Pts',(-59.9782029323629,-106.520167970353,
171.985485138407));
#25917=CARTESIAN_POINT('Ctrl Pts',(-61.1332364564706,-106.302752451468,
173.157058062683));
#25918=CARTESIAN_POINT('Ctrl Pts',(-62.2882699805784,-106.085336932584,
174.328630986959));
#25919=CARTESIAN_POINT('Ctrl Pts',(-62.2783318487242,-105.992115175278,
175.985485236451));
#25920=CARTESIAN_POINT('Ctrl Pts',(-62.26839371687,-105.898893417972,177.642339485944));
#25921=CARTESIAN_POINT('Ctrl Pts',(-61.0934839694364,-105.929865417939,
178.813912312176));
#25922=CARTESIAN_POINT('Ctrl Pts',(-59.9185742220028,-105.960837417905,
179.985485138407));
#25923=CARTESIAN_POINT('Ctrl Pts',(-58.2611174719989,-106.043252152192,
179.985485069079));
#25924=CARTESIAN_POINT('Ctrl Pts',(-56.603660721995,-106.125666886478,179.985484999752));
#25925=CARTESIAN_POINT('Ctrl Pts',(-55.4287510720532,-106.156638876051,
178.813912075476));
#25926=CARTESIAN_POINT('Ctrl Pts',(-54.2538414221114,-106.187610865625,
177.6423391512));
#25927=CARTESIAN_POINT('Ctrl Pts',(-54.2439034281315,-106.09438909362,175.985484901707));
#25928=CARTESIAN_POINT('Ctrl Pts',(-54.2339654341517,-106.001167321616,
174.328630652215));
#25929=CARTESIAN_POINT('Ctrl Pts',(-55.3889990557513,-105.783751792338,
173.157057825983));
#25930=CARTESIAN_POINT('Ctrl Pts',(-56.5440326773509,-105.566336263061,
171.985484999752));
#25931=CARTESIAN_POINT('Ctrl Pts',(-58.1816133015208,-105.297477999464,
171.985485069079));
#25932=CARTESIAN_POINT('Ctrl Pts',(-59.8191939256906,-105.028619735867,
171.985485138407));
#25933=CARTESIAN_POINT('Ctrl Pts',(-60.9742274497984,-104.811204216983,
173.157058062683));
#25934=CARTESIAN_POINT('Ctrl Pts',(-62.1292609739061,-104.593788698099,
174.328630986959));
#25935=CARTESIAN_POINT('Ctrl Pts',(-62.119322842052,-104.500566940792,175.985485236451));
#25936=CARTESIAN_POINT('Ctrl Pts',(-62.1093847101978,-104.407345183486,
177.642339485944));
#25937=CARTESIAN_POINT('Ctrl Pts',(-60.9344749627642,-104.438317183453,
178.813912312176));
#25938=CARTESIAN_POINT('Ctrl Pts',(-59.7595652153305,-104.46928918342,179.985485138407));
#25939=CARTESIAN_POINT('Ctrl Pts',(-58.1021084653266,-104.551703917706,
179.985485069079));
#25940=CARTESIAN_POINT('Ctrl Pts',(-56.4446517153227,-104.634118651992,
179.985484999752));
#25941=CARTESIAN_POINT('Ctrl Pts',(-55.269742065381,-104.665090641566,178.813912075476));
#25942=CARTESIAN_POINT('Ctrl Pts',(-54.0948324154392,-104.696062631139,
177.6423391512));
#25943=CARTESIAN_POINT('Ctrl Pts',(-54.0848944214593,-104.602840859135,
175.985484901707));
#25944=CARTESIAN_POINT('Ctrl Pts',(-54.0749564274795,-104.50961908713,174.328630652215));
#25945=CARTESIAN_POINT('Ctrl Pts',(-55.2299900490791,-104.292203557853,
173.157057825983));
#25946=CARTESIAN_POINT('Ctrl Pts',(-56.3850236706787,-104.074788028575,
171.985484999752));
#25947=CARTESIAN_POINT('Ctrl Pts',(-58.0226042948486,-103.805929764978,
171.985485069079));
#25948=CARTESIAN_POINT('Ctrl Pts',(-59.6601849190184,-103.537071501381,
171.985485138407));
#25949=CARTESIAN_POINT('Ctrl Pts',(-60.8152184431262,-103.319655982497,
173.157058062683));
#25950=CARTESIAN_POINT('Ctrl Pts',(-61.9702519672339,-103.102240463613,
174.328630986959));
#25951=CARTESIAN_POINT('Ctrl Pts',(-61.9603138353797,-103.009018706307,
175.985485236451));
#25952=CARTESIAN_POINT('Ctrl Pts',(-61.9503757035256,-102.915796949001,
177.642339485944));
#25953=CARTESIAN_POINT('Ctrl Pts',(-60.7754659560919,-102.946768948967,
178.813912312176));
#25954=CARTESIAN_POINT('Ctrl Pts',(-59.6005562086583,-102.977740948934,
179.985485138407));
#25955=CARTESIAN_POINT('Ctrl Pts',(-57.9430994586544,-103.06015568322,179.985485069079));
#25956=CARTESIAN_POINT('Ctrl Pts',(-56.2856427086505,-103.142570417507,
179.985484999752));
#25957=CARTESIAN_POINT('Ctrl Pts',(-55.1107330587087,-103.17354240708,178.813912075476));
#25958=CARTESIAN_POINT('Ctrl Pts',(-53.935823408767,-103.204514396654,177.6423391512));
#25959=CARTESIAN_POINT('Ctrl Pts',(-53.9258854147871,-103.111292624649,
175.985484901707));
#25960=CARTESIAN_POINT('Ctrl Pts',(-53.9159474208072,-103.018070852645,
174.328630652215));
#25961=CARTESIAN_POINT('Ctrl Pts',(-55.0709810424069,-102.800655323367,
173.157057825983));
#25962=CARTESIAN_POINT('Ctrl Pts',(-56.2260146640065,-102.58323979409,171.985484999752));
#25963=CARTESIAN_POINT('Ctrl Pts',(-57.8635952881763,-102.314381530493,
171.985485069079));
#25964=CARTESIAN_POINT('Ctrl Pts',(-59.5011759123462,-102.045523266896,
171.985485138407));
#25965=CARTESIAN_POINT('Ctrl Pts',(-60.6562094364539,-101.828107748012,
173.157058062683));
#25966=CARTESIAN_POINT('Ctrl Pts',(-61.8112429605617,-101.610692229127,
174.328630986959));
#25967=CARTESIAN_POINT('Ctrl Pts',(-61.8013048287075,-101.517470471821,
175.985485236451));
#25968=CARTESIAN_POINT('Ctrl Pts',(-61.7913666968533,-101.424248714515,
177.642339485944));
#25969=CARTESIAN_POINT('Ctrl Pts',(-60.6164569494197,-101.455220714482,
178.813912312176));
#25970=CARTESIAN_POINT('Ctrl Pts',(-59.4415472019861,-101.486192714449,
179.985485138407));
#25971=CARTESIAN_POINT('Ctrl Pts',(-57.7840904519822,-101.568607448735,
179.985485069079));
#25972=CARTESIAN_POINT('Ctrl Pts',(-56.1266337019783,-101.651022183021,
179.985484999752));
#25973=CARTESIAN_POINT('Ctrl Pts',(-54.9517240520365,-101.681994172595,
178.813912075476));
#25974=CARTESIAN_POINT('Ctrl Pts',(-53.7768144020947,-101.712966162168,
177.6423391512));
#25975=CARTESIAN_POINT('Ctrl Pts',(-53.7668764081149,-101.619744390164,
175.985484901707));
#25976=CARTESIAN_POINT('Ctrl Pts',(-53.756938414135,-101.526522618159,174.328630652215));
#25977=CARTESIAN_POINT('Ctrl Pts',(-54.9119720357346,-101.309107088882,
173.157057825983));
#25978=CARTESIAN_POINT('Ctrl Pts',(-56.0670056573342,-101.091691559604,
171.985484999752));
#25979=CARTESIAN_POINT('Ctrl Pts',(-57.7045862815041,-100.822833296007,
171.985485069079));
#25980=CARTESIAN_POINT('Ctrl Pts',(-59.342166905674,-100.55397503241,171.985485138407));
#25981=CARTESIAN_POINT('Ctrl Pts',(-60.4972004297817,-100.336559513526,
173.157058062683));
#25982=CARTESIAN_POINT('Ctrl Pts',(-61.6522339538895,-100.119143994642,
174.328630986959));
#25983=CARTESIAN_POINT('Ctrl Pts',(-61.6422958220353,-100.025922237336,
175.985485236451));
#25984=CARTESIAN_POINT('Ctrl Pts',(-61.6323576901811,-99.9327004800294,
177.642339485944));
#25985=CARTESIAN_POINT('Ctrl Pts',(-60.4574479427475,-99.9636724799962,
178.813912312176));
#25986=CARTESIAN_POINT('Ctrl Pts',(-59.2825381953138,-99.994644479963,179.985485138407));
#25987=CARTESIAN_POINT('Ctrl Pts',(-57.6250814453099,-100.077059214249,
179.985485069079));
#25988=CARTESIAN_POINT('Ctrl Pts',(-55.9676246953061,-100.159473948536,
179.985484999752));
#25989=CARTESIAN_POINT('Ctrl Pts',(-54.7927150453643,-100.190445938109,
178.813912075476));
#25990=CARTESIAN_POINT('Ctrl Pts',(-53.6178053954225,-100.221417927683,
177.6423391512));
#25991=CARTESIAN_POINT('Ctrl Pts',(-53.6078674014426,-100.128196155678,
175.985484901707));
#25992=CARTESIAN_POINT('Ctrl Pts',(-53.5979294074628,-100.034974383673,
174.328630652215));
#25993=CARTESIAN_POINT('Ctrl Pts',(-54.7529630290624,-99.817558854396,173.157057825983));
#25994=CARTESIAN_POINT('Ctrl Pts',(-55.907996650662,-99.6001433251185,171.985484999752));
#25995=CARTESIAN_POINT('Ctrl Pts',(-57.5455772748319,-99.3312850615215,
171.985485069079));
#25996=CARTESIAN_POINT('Ctrl Pts',(-59.1831578990017,-99.0624267979246,
171.985485138407));
#25997=CARTESIAN_POINT('Ctrl Pts',(-60.3381914231095,-98.8450112790404,
173.157058062683));
#25998=CARTESIAN_POINT('Ctrl Pts',(-61.4932249472172,-98.6275957601562,
174.328630986959));
#25999=CARTESIAN_POINT('Ctrl Pts',(-61.4832868153631,-98.53437400285,175.985485236451));
#26000=CARTESIAN_POINT('Ctrl Pts',(-61.4733486835089,-98.4411522455438,
177.642339485944));
#26001=CARTESIAN_POINT('Ctrl Pts',(-60.2984389360752,-98.4721242455106,
178.813912312176));
#26002=CARTESIAN_POINT('Ctrl Pts',(-59.1235291886416,-98.5030962454774,
179.985485138407));
#26003=CARTESIAN_POINT('Ctrl Pts',(-57.4660724386377,-98.5855109797636,
179.985485069079));
#26004=CARTESIAN_POINT('Ctrl Pts',(-55.8086156886338,-98.6679257140499,
179.985484999752));
#26005=CARTESIAN_POINT('Ctrl Pts',(-54.633706038692,-98.6988977036234,178.813912075476));
#26006=CARTESIAN_POINT('Ctrl Pts',(-56.2237961054143,-113.614380048479,
178.813912075476));
#26007=CARTESIAN_POINT('Ctrl Pts',(-55.0488864554725,-113.645352038053,
177.6423391512));
#26008=CARTESIAN_POINT('Ctrl Pts',(-55.0389484614927,-113.552130266048,
175.985484901707));
#26009=CARTESIAN_POINT('Ctrl Pts',(-55.0290104675128,-113.458908494044,
174.328630652215));
#26010=CARTESIAN_POINT('Ctrl Pts',(-56.1840440891124,-113.241492964766,
173.157057825983));
#26011=CARTESIAN_POINT('Ctrl Pts',(-57.3390777107121,-113.024077435489,
171.985484999752));
#26012=CARTESIAN_POINT('Ctrl Pts',(-58.9766583348819,-112.755219171892,
171.985485069079));
#26013=CARTESIAN_POINT('Ctrl Pts',(-60.6142389590518,-112.486360908295,
171.985485138407));
#26014=CARTESIAN_POINT('Ctrl Pts',(-61.7692724831595,-112.268945389411,
173.157058062683));
#26015=CARTESIAN_POINT('Ctrl Pts',(-62.9243060072673,-112.051529870527,
174.328630986959));
#26016=CARTESIAN_POINT('Ctrl Pts',(-62.9143678754131,-111.95830811322,175.985485236451));
#26017=CARTESIAN_POINT('Ctrl Pts',(-62.9044297435589,-111.865086355914,
177.642339485944));
#26018=CARTESIAN_POINT('Ctrl Pts',(-61.7295199961253,-111.896058355881,
178.813912312176));
#26019=CARTESIAN_POINT('Ctrl Pts',(-60.5546102486917,-111.927030355848,
179.985485138407));
#26020=CARTESIAN_POINT('Ctrl Pts',(-58.8971534986878,-112.009445090134,
179.985485069079));
#26021=CARTESIAN_POINT('Ctrl Pts',(-57.2396967486839,-112.09185982442,179.985484999752));
#26022=CARTESIAN_POINT('Ctrl Pts',(-56.0647870987421,-112.122831813994,
178.813912075476));
#26023=CARTESIAN_POINT('Ctrl Pts',(-54.8898774488003,-112.153803803567,
177.6423391512));
#26024=CARTESIAN_POINT('Ctrl Pts',(-54.8799394548205,-112.060582031563,
175.985484901707));
#26025=CARTESIAN_POINT('Ctrl Pts',(-54.8700014608406,-111.967360259558,
174.328630652215));
#26026=CARTESIAN_POINT('Ctrl Pts',(-56.0250350824402,-111.749944730281,
173.157057825983));
#26027=CARTESIAN_POINT('Ctrl Pts',(-57.1800687040398,-111.532529201003,
171.985484999752));
#26028=CARTESIAN_POINT('Ctrl Pts',(-58.8176493282097,-111.263670937406,
171.985485069079));
#26029=CARTESIAN_POINT('Ctrl Pts',(-60.4552299523796,-110.994812673809,
171.985485138407));
#26030=CARTESIAN_POINT('Ctrl Pts',(-61.6102634764873,-110.777397154925,
173.157058062683));
#26031=CARTESIAN_POINT('Ctrl Pts',(-62.7652970005951,-110.559981636041,
174.328630986959));
#26032=CARTESIAN_POINT('Ctrl Pts',(-62.7553588687409,-110.466759878735,
175.985485236451));
#26033=CARTESIAN_POINT('Ctrl Pts',(-62.7454207368867,-110.373538121429,
177.642339485944));
#26034=CARTESIAN_POINT('Ctrl Pts',(-61.5705109894531,-110.404510121395,
178.813912312176));
#26035=CARTESIAN_POINT('Ctrl Pts',(-60.3956012420194,-110.435482121362,
179.985485138407));
#26036=CARTESIAN_POINT('Ctrl Pts',(-58.7381444920155,-110.517896855648,
179.985485069079));
#26037=CARTESIAN_POINT('Ctrl Pts',(-57.0806877420116,-110.600311589935,
179.985484999752));
#26038=CARTESIAN_POINT('Ctrl Pts',(-55.9057780920699,-110.631283579508,
178.813912075476));
#26039=CARTESIAN_POINT('Ctrl Pts',(-54.7308684421281,-110.662255569082,
177.6423391512));
#26040=CARTESIAN_POINT('Ctrl Pts',(-54.7209304481482,-110.569033797077,
175.985484901707));
#26041=CARTESIAN_POINT('Ctrl Pts',(-54.7109924541684,-110.475812025073,
174.328630652215));
#26042=CARTESIAN_POINT('Ctrl Pts',(-55.866026075768,-110.258396495795,173.157057825983));
#26043=CARTESIAN_POINT('Ctrl Pts',(-57.0210596973676,-110.040980966518,
171.985484999752));
#26044=CARTESIAN_POINT('Ctrl Pts',(-58.6586403215375,-109.772122702921,
171.985485069079));
#26045=CARTESIAN_POINT('Ctrl Pts',(-60.2962209457073,-109.503264439324,
171.985485138407));
#26046=CARTESIAN_POINT('Ctrl Pts',(-61.4512544698151,-109.28584892044,173.157058062683));
#26047=CARTESIAN_POINT('Ctrl Pts',(-62.6062879939228,-109.068433401555,
174.328630986959));
#26048=CARTESIAN_POINT('Ctrl Pts',(-62.5963498620687,-108.975211644249,
175.985485236451));
#26049=CARTESIAN_POINT('Ctrl Pts',(-62.5864117302145,-108.881989886943,
177.642339485944));
#26050=CARTESIAN_POINT('Ctrl Pts',(-61.4115019827808,-108.91296188691,178.813912312176));
#26051=CARTESIAN_POINT('Ctrl Pts',(-60.2365922353472,-108.943933886877,
179.985485138407));
#26052=CARTESIAN_POINT('Ctrl Pts',(-58.5791354853433,-109.026348621163,
179.985485069079));
#26053=CARTESIAN_POINT('Ctrl Pts',(-56.9216787353394,-109.108763355449,
179.985484999752));
#26054=CARTESIAN_POINT('Ctrl Pts',(-55.7467690853976,-109.139735345023,
178.813912075476));
#26055=CARTESIAN_POINT('Ctrl Pts',(-54.5718594354559,-109.170707334596,
177.6423391512));
#26056=CARTESIAN_POINT('Ctrl Pts',(-54.561921441476,-109.077485562592,175.985484901707));
#26057=CARTESIAN_POINT('Ctrl Pts',(-54.5519834474962,-108.984263790587,
174.328630652215));
#26058=CARTESIAN_POINT('Ctrl Pts',(-55.7070170690958,-108.76684826131,173.157057825983));
#26059=CARTESIAN_POINT('Ctrl Pts',(-56.8620506906954,-108.549432732032,
171.985484999752));
#26060=CARTESIAN_POINT('Ctrl Pts',(-58.4996313148652,-108.280574468435,
171.985485069079));
#26061=CARTESIAN_POINT('Ctrl Pts',(-60.1372119390351,-108.011716204838,
171.985485138407));
#26062=CARTESIAN_POINT('Ctrl Pts',(-61.2922454631428,-107.794300685954,
173.157058062683));
#26063=CARTESIAN_POINT('Ctrl Pts',(-62.4472789872506,-107.57688516707,174.328630986959));
#26064=CARTESIAN_POINT('Ctrl Pts',(-62.4373408553964,-107.483663409764,
175.985485236451));
#26065=CARTESIAN_POINT('Ctrl Pts',(-62.4274027235423,-107.390441652457,
177.642339485944));
#26066=CARTESIAN_POINT('Ctrl Pts',(-61.2524929761086,-107.421413652424,
178.813912312176));
#26067=CARTESIAN_POINT('Ctrl Pts',(-60.077583228675,-107.452385652391,179.985485138407));
#26068=CARTESIAN_POINT('Ctrl Pts',(-58.4201264786711,-107.534800386677,
179.985485069079));
#26069=CARTESIAN_POINT('Ctrl Pts',(-56.7626697286672,-107.617215120964,
179.985484999752));
#26070=CARTESIAN_POINT('Ctrl Pts',(-55.5877600787254,-107.648187110537,
178.813912075476));
#26071=CARTESIAN_POINT('Ctrl Pts',(-54.4128504287836,-107.67915910011,177.6423391512));
#26072=CARTESIAN_POINT('Ctrl Pts',(-54.4029124348038,-107.585937328106,
175.985484901707));
#26073=CARTESIAN_POINT('Ctrl Pts',(-54.3929744408239,-107.492715556102,
174.328630652215));
#26074=CARTESIAN_POINT('Ctrl Pts',(-55.5480080624235,-107.275300026824,
173.157057825983));
#26075=CARTESIAN_POINT('Ctrl Pts',(-56.7030416840231,-107.057884497547,
171.985484999752));
#26076=CARTESIAN_POINT('Ctrl Pts',(-58.340622308193,-106.78902623395,171.985485069079));
#26077=CARTESIAN_POINT('Ctrl Pts',(-59.9782029323629,-106.520167970353,
171.985485138407));
#26078=CARTESIAN_POINT('Ctrl Pts',(-61.1332364564706,-106.302752451468,
173.157058062683));
#26079=CARTESIAN_POINT('Ctrl Pts',(-62.2882699805784,-106.085336932584,
174.328630986959));
#26080=CARTESIAN_POINT('Ctrl Pts',(-62.2783318487242,-105.992115175278,
175.985485236451));
#26081=CARTESIAN_POINT('Ctrl Pts',(-62.26839371687,-105.898893417972,177.642339485944));
#26082=CARTESIAN_POINT('Ctrl Pts',(-61.0934839694364,-105.929865417939,
178.813912312176));
#26083=CARTESIAN_POINT('Ctrl Pts',(-59.9185742220028,-105.960837417905,
179.985485138407));
#26084=CARTESIAN_POINT('Ctrl Pts',(-58.2611174719989,-106.043252152192,
179.985485069079));
#26085=CARTESIAN_POINT('Ctrl Pts',(-56.603660721995,-106.125666886478,179.985484999752));
#26086=CARTESIAN_POINT('Ctrl Pts',(-55.4287510720532,-106.156638876051,
178.813912075476));
#26087=CARTESIAN_POINT('Ctrl Pts',(-54.2538414221114,-106.187610865625,
177.6423391512));
#26088=CARTESIAN_POINT('Ctrl Pts',(-54.2439034281315,-106.09438909362,175.985484901707));
#26089=CARTESIAN_POINT('Ctrl Pts',(-54.2339654341517,-106.001167321616,
174.328630652215));
#26090=CARTESIAN_POINT('Ctrl Pts',(-55.3889990557513,-105.783751792338,
173.157057825983));
#26091=CARTESIAN_POINT('Ctrl Pts',(-56.5440326773509,-105.566336263061,
171.985484999752));
#26092=CARTESIAN_POINT('Ctrl Pts',(-58.1816133015208,-105.297477999464,
171.985485069079));
#26093=CARTESIAN_POINT('Ctrl Pts',(-59.8191939256906,-105.028619735867,
171.985485138407));
#26094=CARTESIAN_POINT('Ctrl Pts',(-60.9742274497984,-104.811204216983,
173.157058062683));
#26095=CARTESIAN_POINT('Ctrl Pts',(-62.1292609739061,-104.593788698099,
174.328630986959));
#26096=CARTESIAN_POINT('Ctrl Pts',(-62.119322842052,-104.500566940792,175.985485236451));
#26097=CARTESIAN_POINT('Ctrl Pts',(-62.1093847101978,-104.407345183486,
177.642339485944));
#26098=CARTESIAN_POINT('Ctrl Pts',(-60.9344749627642,-104.438317183453,
178.813912312176));
#26099=CARTESIAN_POINT('Ctrl Pts',(-59.7595652153305,-104.46928918342,179.985485138407));
#26100=CARTESIAN_POINT('Ctrl Pts',(-58.1021084653266,-104.551703917706,
179.985485069079));
#26101=CARTESIAN_POINT('Ctrl Pts',(-56.4446517153227,-104.634118651992,
179.985484999752));
#26102=CARTESIAN_POINT('Ctrl Pts',(-55.269742065381,-104.665090641566,178.813912075476));
#26103=CARTESIAN_POINT('Ctrl Pts',(-54.0948324154392,-104.696062631139,
177.6423391512));
#26104=CARTESIAN_POINT('Ctrl Pts',(-54.0848944214593,-104.602840859135,
175.985484901707));
#26105=CARTESIAN_POINT('Ctrl Pts',(-54.0749564274795,-104.50961908713,174.328630652215));
#26106=CARTESIAN_POINT('Ctrl Pts',(-55.2299900490791,-104.292203557853,
173.157057825983));
#26107=CARTESIAN_POINT('Ctrl Pts',(-56.3850236706787,-104.074788028575,
171.985484999752));
#26108=CARTESIAN_POINT('Ctrl Pts',(-58.0226042948486,-103.805929764978,
171.985485069079));
#26109=CARTESIAN_POINT('Ctrl Pts',(-59.6601849190184,-103.537071501381,
171.985485138407));
#26110=CARTESIAN_POINT('Ctrl Pts',(-60.8152184431262,-103.319655982497,
173.157058062683));
#26111=CARTESIAN_POINT('Ctrl Pts',(-61.9702519672339,-103.102240463613,
174.328630986959));
#26112=CARTESIAN_POINT('Ctrl Pts',(-61.9603138353797,-103.009018706307,
175.985485236451));
#26113=CARTESIAN_POINT('Ctrl Pts',(-61.9503757035256,-102.915796949001,
177.642339485944));
#26114=CARTESIAN_POINT('Ctrl Pts',(-60.7754659560919,-102.946768948967,
178.813912312176));
#26115=CARTESIAN_POINT('Ctrl Pts',(-59.6005562086583,-102.977740948934,
179.985485138407));
#26116=CARTESIAN_POINT('Ctrl Pts',(-57.9430994586544,-103.06015568322,179.985485069079));
#26117=CARTESIAN_POINT('Ctrl Pts',(-56.2856427086505,-103.142570417507,
179.985484999752));
#26118=CARTESIAN_POINT('Ctrl Pts',(-55.1107330587087,-103.17354240708,178.813912075476));
#26119=CARTESIAN_POINT('Ctrl Pts',(-53.935823408767,-103.204514396654,177.6423391512));
#26120=CARTESIAN_POINT('Ctrl Pts',(-53.9258854147871,-103.111292624649,
175.985484901707));
#26121=CARTESIAN_POINT('Ctrl Pts',(-53.9159474208072,-103.018070852645,
174.328630652215));
#26122=CARTESIAN_POINT('Ctrl Pts',(-55.0709810424069,-102.800655323367,
173.157057825983));
#26123=CARTESIAN_POINT('Ctrl Pts',(-56.2260146640065,-102.58323979409,171.985484999752));
#26124=CARTESIAN_POINT('Ctrl Pts',(-57.8635952881763,-102.314381530493,
171.985485069079));
#26125=CARTESIAN_POINT('Ctrl Pts',(-59.5011759123462,-102.045523266896,
171.985485138407));
#26126=CARTESIAN_POINT('Ctrl Pts',(-60.6562094364539,-101.828107748012,
173.157058062683));
#26127=CARTESIAN_POINT('Ctrl Pts',(-61.8112429605617,-101.610692229127,
174.328630986959));
#26128=CARTESIAN_POINT('Ctrl Pts',(-61.8013048287075,-101.517470471821,
175.985485236451));
#26129=CARTESIAN_POINT('Ctrl Pts',(-61.7913666968533,-101.424248714515,
177.642339485944));
#26130=CARTESIAN_POINT('Ctrl Pts',(-60.6164569494197,-101.455220714482,
178.813912312176));
#26131=CARTESIAN_POINT('Ctrl Pts',(-59.4415472019861,-101.486192714449,
179.985485138407));
#26132=CARTESIAN_POINT('Ctrl Pts',(-57.7840904519822,-101.568607448735,
179.985485069079));
#26133=CARTESIAN_POINT('Ctrl Pts',(-56.1266337019783,-101.651022183021,
179.985484999752));
#26134=CARTESIAN_POINT('Ctrl Pts',(-54.9517240520365,-101.681994172595,
178.813912075476));
#26135=CARTESIAN_POINT('Ctrl Pts',(-53.7768144020947,-101.712966162168,
177.6423391512));
#26136=CARTESIAN_POINT('Ctrl Pts',(-53.7668764081149,-101.619744390164,
175.985484901707));
#26137=CARTESIAN_POINT('Ctrl Pts',(-53.756938414135,-101.526522618159,174.328630652215));
#26138=CARTESIAN_POINT('Ctrl Pts',(-54.9119720357346,-101.309107088882,
173.157057825983));
#26139=CARTESIAN_POINT('Ctrl Pts',(-56.0670056573342,-101.091691559604,
171.985484999752));
#26140=CARTESIAN_POINT('Ctrl Pts',(-57.7045862815041,-100.822833296007,
171.985485069079));
#26141=CARTESIAN_POINT('Ctrl Pts',(-59.342166905674,-100.55397503241,171.985485138407));
#26142=CARTESIAN_POINT('Ctrl Pts',(-60.4972004297817,-100.336559513526,
173.157058062683));
#26143=CARTESIAN_POINT('Ctrl Pts',(-61.6522339538895,-100.119143994642,
174.328630986959));
#26144=CARTESIAN_POINT('Ctrl Pts',(-61.6422958220353,-100.025922237336,
175.985485236451));
#26145=CARTESIAN_POINT('Ctrl Pts',(-61.6323576901811,-99.9327004800294,
177.642339485944));
#26146=CARTESIAN_POINT('Ctrl Pts',(-60.4574479427475,-99.9636724799962,
178.813912312176));
#26147=CARTESIAN_POINT('Ctrl Pts',(-59.2825381953138,-99.994644479963,179.985485138407));
#26148=CARTESIAN_POINT('Ctrl Pts',(-57.6250814453099,-100.077059214249,
179.985485069079));
#26149=CARTESIAN_POINT('Ctrl Pts',(-55.9676246953061,-100.159473948536,
179.985484999752));
#26150=CARTESIAN_POINT('Ctrl Pts',(-54.7927150453643,-100.190445938109,
178.813912075476));
#26151=CARTESIAN_POINT('Ctrl Pts',(-53.6178053954225,-100.221417927683,
177.6423391512));
#26152=CARTESIAN_POINT('Ctrl Pts',(-53.6078674014426,-100.128196155678,
175.985484901707));
#26153=CARTESIAN_POINT('Ctrl Pts',(-53.5979294074628,-100.034974383673,
174.328630652215));
#26154=CARTESIAN_POINT('Ctrl Pts',(-54.7529630290624,-99.817558854396,173.157057825983));
#26155=CARTESIAN_POINT('Ctrl Pts',(-55.907996650662,-99.6001433251185,171.985484999752));
#26156=CARTESIAN_POINT('Ctrl Pts',(-57.5455772748319,-99.3312850615215,
171.985485069079));
#26157=CARTESIAN_POINT('Ctrl Pts',(-59.1831578990017,-99.0624267979246,
171.985485138407));
#26158=CARTESIAN_POINT('Ctrl Pts',(-60.3381914231095,-98.8450112790404,
173.157058062683));
#26159=CARTESIAN_POINT('Ctrl Pts',(-61.4932249472172,-98.6275957601562,
174.328630986959));
#26160=CARTESIAN_POINT('Ctrl Pts',(-61.4832868153631,-98.53437400285,175.985485236451));
#26161=CARTESIAN_POINT('Ctrl Pts',(-61.4733486835089,-98.4411522455438,
177.642339485944));
#26162=CARTESIAN_POINT('Ctrl Pts',(-60.2984389360752,-98.4721242455106,
178.813912312176));
#26163=CARTESIAN_POINT('Ctrl Pts',(-59.1235291886416,-98.5030962454774,
179.985485138407));
#26164=CARTESIAN_POINT('Ctrl Pts',(-57.4660724386377,-98.5855109797636,
179.985485069079));
#26165=CARTESIAN_POINT('Ctrl Pts',(-55.8086156886338,-98.6679257140499,
179.985484999752));
#26166=CARTESIAN_POINT('Ctrl Pts',(-54.633706038692,-98.6988977036234,178.813912075476));
#26167=CARTESIAN_POINT('Ctrl Pts',(-56.9964983346804,-113.864655531781,
178.072094410988));
#26168=CARTESIAN_POINT('Ctrl Pts',(-56.1271283009022,-113.863054956993,
177.207792449865));
#26169=CARTESIAN_POINT('Ctrl Pts',(-56.117190288842,-113.769833186916,175.985484945604));
#26170=CARTESIAN_POINT('Ctrl Pts',(-56.1072522767819,-113.676611416839,
174.763177441344));
#26171=CARTESIAN_POINT('Ctrl Pts',(-56.9567462566485,-113.491768454648,
173.89887555255));
#26172=CARTESIAN_POINT('Ctrl Pts',(-57.8062402365152,-113.306925492458,
173.034573663757));
#26173=CARTESIAN_POINT('Ctrl Pts',(-59.011722573584,-113.084131793069,173.034573714903));
#26174=CARTESIAN_POINT('Ctrl Pts',(-60.2172049106529,-112.86133809368,173.034573766048));
#26175=CARTESIAN_POINT('Ctrl Pts',(-61.0666988185971,-112.676495139156,
173.898875727171));
#26176=CARTESIAN_POINT('Ctrl Pts',(-61.9161927265413,-112.491652184633,
174.763177688294));
#26177=CARTESIAN_POINT('Ctrl Pts',(-61.9062546127674,-112.398430425399,
175.985485192554));
#26178=CARTESIAN_POINT('Ctrl Pts',(-61.8963164989935,-112.305208666166,
177.207792696815));
#26179=CARTESIAN_POINT('Ctrl Pts',(-61.0269463932928,-112.303608099046,
178.072094585608));
#26180=CARTESIAN_POINT('Ctrl Pts',(-60.1575762875921,-112.302007531926,
178.936396474401));
#26181=CARTESIAN_POINT('Ctrl Pts',(-58.9322178246893,-112.338357702004,
178.936396423256));
#26182=CARTESIAN_POINT('Ctrl Pts',(-57.7068593617864,-112.374707872082,
178.936396372111));
#26183=CARTESIAN_POINT('Ctrl Pts',(-56.8374893280082,-112.373107297295,
178.072094410988));
#26184=CARTESIAN_POINT('Ctrl Pts',(-55.9681192942299,-112.371506722508,
177.207792449865));
#26185=CARTESIAN_POINT('Ctrl Pts',(-55.9581812821698,-112.278284952431,
175.985484945604));
#26186=CARTESIAN_POINT('Ctrl Pts',(-55.9482432701096,-112.185063182354,
174.763177441344));
#26187=CARTESIAN_POINT('Ctrl Pts',(-56.7977372499763,-112.000220220163,
173.89887555255));
#26188=CARTESIAN_POINT('Ctrl Pts',(-57.647231229843,-111.815377257972,173.034573663757));
#26189=CARTESIAN_POINT('Ctrl Pts',(-58.8527135669118,-111.592583558583,
173.034573714903));
#26190=CARTESIAN_POINT('Ctrl Pts',(-60.0581959039807,-111.369789859194,
173.034573766048));
#26191=CARTESIAN_POINT('Ctrl Pts',(-60.9076898119249,-111.184946904671,
173.898875727171));
#26192=CARTESIAN_POINT('Ctrl Pts',(-61.7571837198691,-111.000103950148,
174.763177688294));
#26193=CARTESIAN_POINT('Ctrl Pts',(-61.7472456060952,-110.906882190914,
175.985485192554));
#26194=CARTESIAN_POINT('Ctrl Pts',(-61.7373074923213,-110.81366043168,177.207792696815));
#26195=CARTESIAN_POINT('Ctrl Pts',(-60.8679373866206,-110.81205986456,178.072094585608));
#26196=CARTESIAN_POINT('Ctrl Pts',(-59.9985672809199,-110.81045929744,178.936396474401));
#26197=CARTESIAN_POINT('Ctrl Pts',(-58.7732088180171,-110.846809467519,
178.936396423256));
#26198=CARTESIAN_POINT('Ctrl Pts',(-57.5478503551142,-110.883159637597,
178.936396372111));
#26199=CARTESIAN_POINT('Ctrl Pts',(-56.6784803213359,-110.881559062809,
178.072094410988));
#26200=CARTESIAN_POINT('Ctrl Pts',(-55.8091102875577,-110.879958488022,
177.207792449865));
#26201=CARTESIAN_POINT('Ctrl Pts',(-55.7991722754976,-110.786736717945,
175.985484945604));
#26202=CARTESIAN_POINT('Ctrl Pts',(-55.7892342634374,-110.693514947868,
174.763177441344));
#26203=CARTESIAN_POINT('Ctrl Pts',(-56.6387282433041,-110.508671985677,
173.89887555255));
#26204=CARTESIAN_POINT('Ctrl Pts',(-57.4882222231708,-110.323829023487,
173.034573663757));
#26205=CARTESIAN_POINT('Ctrl Pts',(-58.6937045602396,-110.101035324098,
173.034573714903));
#26206=CARTESIAN_POINT('Ctrl Pts',(-59.8991868973084,-109.878241624709,
173.034573766048));
#26207=CARTESIAN_POINT('Ctrl Pts',(-60.7486808052526,-109.693398670185,
173.898875727171));
#26208=CARTESIAN_POINT('Ctrl Pts',(-61.5981747131968,-109.508555715662,
174.763177688294));
#26209=CARTESIAN_POINT('Ctrl Pts',(-61.588236599423,-109.415333956428,175.985485192554));
#26210=CARTESIAN_POINT('Ctrl Pts',(-61.5782984856491,-109.322112197195,
177.207792696815));
#26211=CARTESIAN_POINT('Ctrl Pts',(-60.7089283799484,-109.320511630075,
178.072094585608));
#26212=CARTESIAN_POINT('Ctrl Pts',(-59.8395582742477,-109.318911062955,
178.936396474401));
#26213=CARTESIAN_POINT('Ctrl Pts',(-58.6141998113448,-109.355261233033,
178.936396423256));
#26214=CARTESIAN_POINT('Ctrl Pts',(-57.388841348442,-109.391611403111,178.936396372111));
#26215=CARTESIAN_POINT('Ctrl Pts',(-56.5194713146637,-109.390010828324,
178.072094410988));
#26216=CARTESIAN_POINT('Ctrl Pts',(-55.6501012808855,-109.388410253536,
177.207792449865));
#26217=CARTESIAN_POINT('Ctrl Pts',(-55.6401632688253,-109.295188483459,
175.985484945604));
#26218=CARTESIAN_POINT('Ctrl Pts',(-55.6302252567652,-109.201966713382,
174.763177441344));
#26219=CARTESIAN_POINT('Ctrl Pts',(-56.4797192366319,-109.017123751192,
173.89887555255));
#26220=CARTESIAN_POINT('Ctrl Pts',(-57.3292132164985,-108.832280789001,
173.034573663757));
#26221=CARTESIAN_POINT('Ctrl Pts',(-58.5346955535674,-108.609487089612,
173.034573714903));
#26222=CARTESIAN_POINT('Ctrl Pts',(-59.7401778906362,-108.386693390223,
173.034573766048));
#26223=CARTESIAN_POINT('Ctrl Pts',(-60.5896717985804,-108.2018504357,173.898875727171));
#26224=CARTESIAN_POINT('Ctrl Pts',(-61.4391657065246,-108.017007481176,
174.763177688294));
#26225=CARTESIAN_POINT('Ctrl Pts',(-61.4292275927507,-107.923785721943,
175.985485192554));
#26226=CARTESIAN_POINT('Ctrl Pts',(-61.4192894789769,-107.830563962709,
177.207792696815));
#26227=CARTESIAN_POINT('Ctrl Pts',(-60.5499193732762,-107.828963395589,
178.072094585608));
#26228=CARTESIAN_POINT('Ctrl Pts',(-59.6805492675755,-107.827362828469,
178.936396474401));
#26229=CARTESIAN_POINT('Ctrl Pts',(-58.4551908046726,-107.863712998547,
178.936396423256));
#26230=CARTESIAN_POINT('Ctrl Pts',(-57.2298323417698,-107.900063168626,
178.936396372111));
#26231=CARTESIAN_POINT('Ctrl Pts',(-56.3604623079915,-107.898462593838,
178.072094410988));
#26232=CARTESIAN_POINT('Ctrl Pts',(-55.4910922742133,-107.896862019051,
177.207792449865));
#26233=CARTESIAN_POINT('Ctrl Pts',(-55.4811542621531,-107.803640248974,
175.985484945604));
#26234=CARTESIAN_POINT('Ctrl Pts',(-55.471216250093,-107.710418478897,174.763177441344));
#26235=CARTESIAN_POINT('Ctrl Pts',(-56.3207102299596,-107.525575516706,
173.89887555255));
#26236=CARTESIAN_POINT('Ctrl Pts',(-57.1702042098263,-107.340732554515,
173.034573663757));
#26237=CARTESIAN_POINT('Ctrl Pts',(-58.3756865468951,-107.117938855126,
173.034573714903));
#26238=CARTESIAN_POINT('Ctrl Pts',(-59.581168883964,-106.895145155737,173.034573766048));
#26239=CARTESIAN_POINT('Ctrl Pts',(-60.4306627919082,-106.710302201214,
173.898875727171));
#26240=CARTESIAN_POINT('Ctrl Pts',(-61.2801566998524,-106.525459246691,
174.763177688294));
#26241=CARTESIAN_POINT('Ctrl Pts',(-61.2702185860785,-106.432237487457,
175.985485192554));
#26242=CARTESIAN_POINT('Ctrl Pts',(-61.2602804723046,-106.339015728223,
177.207792696815));
#26243=CARTESIAN_POINT('Ctrl Pts',(-60.3909103666039,-106.337415161103,
178.072094585608));
#26244=CARTESIAN_POINT('Ctrl Pts',(-59.5215402609032,-106.335814593983,
178.936396474401));
#26245=CARTESIAN_POINT('Ctrl Pts',(-58.2961817980004,-106.372164764062,
178.936396423256));
#26246=CARTESIAN_POINT('Ctrl Pts',(-57.0708233350975,-106.40851493414,178.936396372111));
#26247=CARTESIAN_POINT('Ctrl Pts',(-56.2014533013193,-106.406914359353,
178.072094410988));
#26248=CARTESIAN_POINT('Ctrl Pts',(-55.332083267541,-106.405313784565,177.207792449865));
#26249=CARTESIAN_POINT('Ctrl Pts',(-55.3221452554809,-106.312092014488,
175.985484945604));
#26250=CARTESIAN_POINT('Ctrl Pts',(-55.3122072434207,-106.218870244411,
174.763177441344));
#26251=CARTESIAN_POINT('Ctrl Pts',(-56.1617012232874,-106.034027282221,
173.89887555255));
#26252=CARTESIAN_POINT('Ctrl Pts',(-57.0111952031541,-105.84918432003,173.034573663757));
#26253=CARTESIAN_POINT('Ctrl Pts',(-58.2166775402229,-105.626390620641,
173.034573714903));
#26254=CARTESIAN_POINT('Ctrl Pts',(-59.4221598772917,-105.403596921252,
173.034573766048));
#26255=CARTESIAN_POINT('Ctrl Pts',(-60.2716537852359,-105.218753966728,
173.898875727171));
#26256=CARTESIAN_POINT('Ctrl Pts',(-61.1211476931802,-105.033911012205,
174.763177688294));
#26257=CARTESIAN_POINT('Ctrl Pts',(-61.1112095794063,-104.940689252971,
175.985485192554));
#26258=CARTESIAN_POINT('Ctrl Pts',(-61.1012714656324,-104.847467493738,
177.207792696815));
#26259=CARTESIAN_POINT('Ctrl Pts',(-60.2319013599317,-104.845866926618,
178.072094585608));
#26260=CARTESIAN_POINT('Ctrl Pts',(-59.362531254231,-104.844266359498,178.936396474401));
#26261=CARTESIAN_POINT('Ctrl Pts',(-58.1371727913281,-104.880616529576,
178.936396423256));
#26262=CARTESIAN_POINT('Ctrl Pts',(-56.9118143284253,-104.916966699654,
178.936396372111));
#26263=CARTESIAN_POINT('Ctrl Pts',(-56.042444294647,-104.915366124867,178.072094410988));
#26264=CARTESIAN_POINT('Ctrl Pts',(-55.1730742608688,-104.91376555008,177.207792449865));
#26265=CARTESIAN_POINT('Ctrl Pts',(-55.1631362488087,-104.820543780003,
175.985484945604));
#26266=CARTESIAN_POINT('Ctrl Pts',(-55.1531982367485,-104.727322009926,
174.763177441344));
#26267=CARTESIAN_POINT('Ctrl Pts',(-56.0026922166152,-104.542479047735,
173.89887555255));
#26268=CARTESIAN_POINT('Ctrl Pts',(-56.8521861964818,-104.357636085544,
173.034573663757));
#26269=CARTESIAN_POINT('Ctrl Pts',(-58.0576685335507,-104.134842386155,
173.034573714903));
#26270=CARTESIAN_POINT('Ctrl Pts',(-59.2631508706195,-103.912048686766,
173.034573766048));
#26271=CARTESIAN_POINT('Ctrl Pts',(-60.1126447785637,-103.727205732243,
173.898875727171));
#26272=CARTESIAN_POINT('Ctrl Pts',(-60.9621386865079,-103.54236277772,174.763177688294));
#26273=CARTESIAN_POINT('Ctrl Pts',(-60.952200572734,-103.449141018486,175.985485192554));
#26274=CARTESIAN_POINT('Ctrl Pts',(-60.9422624589602,-103.355919259252,
177.207792696815));
#26275=CARTESIAN_POINT('Ctrl Pts',(-60.0728923532595,-103.354318692132,
178.072094585608));
#26276=CARTESIAN_POINT('Ctrl Pts',(-59.2035222475588,-103.352718125012,
178.936396474401));
#26277=CARTESIAN_POINT('Ctrl Pts',(-57.9781637846559,-103.389068295091,
178.936396423256));
#26278=CARTESIAN_POINT('Ctrl Pts',(-56.7528053217531,-103.425418465169,
178.936396372111));
#26279=CARTESIAN_POINT('Ctrl Pts',(-55.8834352879748,-103.423817890381,
178.072094410988));
#26280=CARTESIAN_POINT('Ctrl Pts',(-55.0140652541966,-103.422217315594,
177.207792449865));
#26281=CARTESIAN_POINT('Ctrl Pts',(-55.0041272421364,-103.328995545517,
175.985484945604));
#26282=CARTESIAN_POINT('Ctrl Pts',(-54.9941892300763,-103.23577377544,174.763177441344));
#26283=CARTESIAN_POINT('Ctrl Pts',(-55.8436832099429,-103.050930813249,
173.89887555255));
#26284=CARTESIAN_POINT('Ctrl Pts',(-56.6931771898096,-102.866087851059,
173.034573663757));
#26285=CARTESIAN_POINT('Ctrl Pts',(-57.8986595268784,-102.64329415167,173.034573714903));
#26286=CARTESIAN_POINT('Ctrl Pts',(-59.1041418639473,-102.420500452281,
173.034573766048));
#26287=CARTESIAN_POINT('Ctrl Pts',(-59.9536357718915,-102.235657497757,
173.898875727171));
#26288=CARTESIAN_POINT('Ctrl Pts',(-60.8031296798357,-102.050814543234,
174.763177688294));
#26289=CARTESIAN_POINT('Ctrl Pts',(-60.7931915660618,-101.957592784,175.985485192554));
#26290=CARTESIAN_POINT('Ctrl Pts',(-60.783253452288,-101.864371024767,177.207792696815));
#26291=CARTESIAN_POINT('Ctrl Pts',(-59.9138833465873,-101.862770457647,
178.072094585608));
#26292=CARTESIAN_POINT('Ctrl Pts',(-59.0445132408866,-101.861169890527,
178.936396474401));
#26293=CARTESIAN_POINT('Ctrl Pts',(-57.8191547779837,-101.897520060605,
178.936396423256));
#26294=CARTESIAN_POINT('Ctrl Pts',(-56.5937963150808,-101.933870230683,
178.936396372111));
#26295=CARTESIAN_POINT('Ctrl Pts',(-55.7244262813026,-101.932269655896,
178.072094410988));
#26296=CARTESIAN_POINT('Ctrl Pts',(-54.8550562475244,-101.930669081108,
177.207792449865));
#26297=CARTESIAN_POINT('Ctrl Pts',(-54.8451182354642,-101.837447311031,
175.985484945604));
#26298=CARTESIAN_POINT('Ctrl Pts',(-54.8351802234041,-101.744225540954,
174.763177441344));
#26299=CARTESIAN_POINT('Ctrl Pts',(-55.6846742032707,-101.559382578764,
173.89887555255));
#26300=CARTESIAN_POINT('Ctrl Pts',(-56.5341681831374,-101.374539616573,
173.034573663757));
#26301=CARTESIAN_POINT('Ctrl Pts',(-57.7396505202062,-101.151745917184,
173.034573714903));
#26302=CARTESIAN_POINT('Ctrl Pts',(-58.9451328572751,-100.928952217795,
173.034573766048));
#26303=CARTESIAN_POINT('Ctrl Pts',(-59.7946267652193,-100.744109263272,
173.898875727171));
#26304=CARTESIAN_POINT('Ctrl Pts',(-60.6441206731635,-100.559266308748,
174.763177688294));
#26305=CARTESIAN_POINT('Ctrl Pts',(-60.6341825593896,-100.466044549515,
175.985485192554));
#26306=CARTESIAN_POINT('Ctrl Pts',(-60.6242444456157,-100.372822790281,
177.207792696815));
#26307=CARTESIAN_POINT('Ctrl Pts',(-59.754874339915,-100.371222223161,178.072094585608));
#26308=CARTESIAN_POINT('Ctrl Pts',(-58.8855042342143,-100.369621656041,
178.936396474401));
#26309=CARTESIAN_POINT('Ctrl Pts',(-57.6601457713115,-100.405971826119,
178.936396423256));
#26310=CARTESIAN_POINT('Ctrl Pts',(-56.4347873084086,-100.442321996198,
178.936396372111));
#26311=CARTESIAN_POINT('Ctrl Pts',(-55.5654172746304,-100.44072142141,178.072094410988));
#26312=CARTESIAN_POINT('Ctrl Pts',(-54.6960472408521,-100.439120846623,
177.207792449865));
#26313=CARTESIAN_POINT('Ctrl Pts',(-54.686109228792,-100.345899076546,175.985484945604));
#26314=CARTESIAN_POINT('Ctrl Pts',(-54.6761712167318,-100.252677306469,
174.763177441344));
#26315=CARTESIAN_POINT('Ctrl Pts',(-55.5256651965985,-100.067834344278,
173.89887555255));
#26316=CARTESIAN_POINT('Ctrl Pts',(-56.3751591764652,-99.8829913820874,
173.034573663757));
#26317=CARTESIAN_POINT('Ctrl Pts',(-57.580641513534,-99.6601976826983,173.034573714903));
#26318=CARTESIAN_POINT('Ctrl Pts',(-58.7861238506028,-99.4374039833093,
173.034573766048));
#26319=CARTESIAN_POINT('Ctrl Pts',(-59.635617758547,-99.252561028786,173.898875727171));
#26320=CARTESIAN_POINT('Ctrl Pts',(-60.4851116664912,-99.0677180742627,
174.763177688294));
#26321=CARTESIAN_POINT('Ctrl Pts',(-60.4751735527174,-98.9744963150291,
175.985485192554));
#26322=CARTESIAN_POINT('Ctrl Pts',(-60.4652354389435,-98.8812745557954,
177.207792696815));
#26323=CARTESIAN_POINT('Ctrl Pts',(-59.5958653332428,-98.8796739886754,
178.072094585608));
#26324=CARTESIAN_POINT('Ctrl Pts',(-58.7264952275421,-98.8780734215554,
178.936396474401));
#26325=CARTESIAN_POINT('Ctrl Pts',(-57.5011367646392,-98.9144235916337,
178.936396423256));
#26326=CARTESIAN_POINT('Ctrl Pts',(-56.2757783017364,-98.9507737617121,
178.936396372111));
#26327=CARTESIAN_POINT('Ctrl Pts',(-55.4064082679581,-98.9491731869247,
178.072094410988));
#26328=CARTESIAN_POINT('Ctrl Pts',(-61.7066176068137,-108.90712070075,178.485485069079));
#26329=CARTESIAN_POINT('Ctrl Pts',(-61.568045402457,-108.908835218628,178.657813499464));
#26330=CARTESIAN_POINT('Ctrl Pts',(-61.4115019827808,-108.91296188691,178.813912312176));
#26331=CARTESIAN_POINT('Ctrl Pts',(-60.2365922353472,-108.943933886877,
179.985485138407));
#26332=CARTESIAN_POINT('Ctrl Pts',(-58.5791354853433,-109.026348621163,
179.985485069079));
#26333=CARTESIAN_POINT('Ctrl Pts',(-56.9216787353394,-109.108763355449,
179.985484999752));
#26334=CARTESIAN_POINT('Ctrl Pts',(-55.7467690853976,-109.139735345023,
178.813912075476));
#26335=CARTESIAN_POINT('Ctrl Pts',(-54.5718594354559,-109.170707334596,
177.6423391512));
#26336=CARTESIAN_POINT('Ctrl Pts',(-54.561921441476,-109.077485562592,175.985484901707));
#26337=CARTESIAN_POINT('Ctrl Pts',(-54.5519834474962,-108.984263790587,
174.328630652215));
#26338=CARTESIAN_POINT('Ctrl Pts',(-55.7070170690958,-108.76684826131,173.157057825983));
#26339=CARTESIAN_POINT('Ctrl Pts',(-56.8620506906954,-108.549432732032,
171.985484999752));
#26340=CARTESIAN_POINT('Ctrl Pts',(-58.4996313148652,-108.280574468435,
171.985485069079));
#26341=CARTESIAN_POINT('Ctrl Pts',(-60.1372119390351,-108.011716204838,
171.985485138407));
#26342=CARTESIAN_POINT('Ctrl Pts',(-61.2922454631428,-107.794300685954,
173.157058062683));
#26343=CARTESIAN_POINT('Ctrl Pts',(-61.446140484096,-107.765332552012,173.313156769748));
#26344=CARTESIAN_POINT('Ctrl Pts',(-61.5819596880668,-107.737795122829,
173.485485069079));
#26345=CARTESIAN_POINT('Ctrl Pts',(-56.8733667677527,-112.709647553905,
178.072094410988));
#26346=CARTESIAN_POINT('Ctrl Pts',(-56.0039967339745,-112.708046979118,
177.207792449865));
#26347=CARTESIAN_POINT('Ctrl Pts',(-55.9940587219143,-112.614825209041,
175.985484945604));
#26348=CARTESIAN_POINT('Ctrl Pts',(-55.9841207098542,-112.521603438964,
174.763177441344));
#26349=CARTESIAN_POINT('Ctrl Pts',(-56.8336146897208,-112.336760476773,
173.89887555255));
#26350=CARTESIAN_POINT('Ctrl Pts',(-57.6831086695875,-112.151917514582,
173.034573663757));
#26351=CARTESIAN_POINT('Ctrl Pts',(-58.8885910066563,-111.929123815193,
173.034573714903));
#26352=CARTESIAN_POINT('Ctrl Pts',(-60.0940733437252,-111.706330115804,
173.034573766048));
#26353=CARTESIAN_POINT('Ctrl Pts',(-60.9435672516694,-111.521487161281,
173.898875727171));
#26354=CARTESIAN_POINT('Ctrl Pts',(-61.7930611596136,-111.336644206758,
174.763177688294));
#26355=CARTESIAN_POINT('Ctrl Pts',(-61.7831230458397,-111.243422447524,
175.985485192554));
#26356=CARTESIAN_POINT('Ctrl Pts',(-61.7731849320658,-111.15020068829,177.207792696815));
#26357=CARTESIAN_POINT('Ctrl Pts',(-60.9038148263651,-111.14860012117,178.072094585608));
#26358=CARTESIAN_POINT('Ctrl Pts',(-60.0344447206644,-111.14699955405,178.936396474401));
#26359=CARTESIAN_POINT('Ctrl Pts',(-58.8090862577616,-111.183349724129,
178.936396423256));
#26360=CARTESIAN_POINT('Ctrl Pts',(-57.5837277948587,-111.219699894207,
178.936396372111));
#26361=CARTESIAN_POINT('Ctrl Pts',(-56.7143577610805,-111.21809931942,178.072094410988));
#26362=CARTESIAN_POINT('Ctrl Pts',(-55.8449877273022,-111.216498744632,
177.207792449865));
#26363=CARTESIAN_POINT('Ctrl Pts',(-55.8350497152421,-111.123276974555,
175.985484945604));
#26364=CARTESIAN_POINT('Ctrl Pts',(-55.8251117031819,-111.030055204478,
174.763177441344));
#26365=CARTESIAN_POINT('Ctrl Pts',(-56.6746056830486,-110.845212242287,
173.89887555255));
#26366=CARTESIAN_POINT('Ctrl Pts',(-57.5240996629153,-110.660369280097,
173.034573663757));
#26367=CARTESIAN_POINT('Ctrl Pts',(-58.7295819999841,-110.437575580708,
173.034573714903));
#26368=CARTESIAN_POINT('Ctrl Pts',(-59.9350643370529,-110.214781881319,
173.034573766048));
#26369=CARTESIAN_POINT('Ctrl Pts',(-60.7845582449971,-110.029938926795,
173.898875727171));
#26370=CARTESIAN_POINT('Ctrl Pts',(-61.6340521529414,-109.845095972272,
174.763177688294));
#26371=CARTESIAN_POINT('Ctrl Pts',(-61.6241140391675,-109.751874213038,
175.985485192554));
#26372=CARTESIAN_POINT('Ctrl Pts',(-61.6141759253936,-109.658652453805,
177.207792696815));
#26373=CARTESIAN_POINT('Ctrl Pts',(-60.7448058196929,-109.657051886685,
178.072094585608));
#26374=CARTESIAN_POINT('Ctrl Pts',(-59.8754357139922,-109.655451319565,
178.936396474401));
#26375=CARTESIAN_POINT('Ctrl Pts',(-58.6500772510893,-109.691801489643,
178.936396423256));
#26376=CARTESIAN_POINT('Ctrl Pts',(-57.4247187881865,-109.728151659721,
178.936396372111));
#26377=CARTESIAN_POINT('Ctrl Pts',(-56.5553487544082,-109.726551084934,
178.072094410988));
#26378=CARTESIAN_POINT('Ctrl Pts',(-55.68597872063,-109.724950510147,177.207792449865));
#26379=CARTESIAN_POINT('Ctrl Pts',(-55.6760407085698,-109.63172874007,175.985484945604));
#26380=CARTESIAN_POINT('Ctrl Pts',(-55.6661026965097,-109.538506969993,
174.763177441344));
#26381=CARTESIAN_POINT('Ctrl Pts',(-56.5155966763764,-109.353664007802,
173.89887555255));
#26382=CARTESIAN_POINT('Ctrl Pts',(-57.365090656243,-109.168821045611,173.034573663757));
#26383=CARTESIAN_POINT('Ctrl Pts',(-58.5705729933119,-108.946027346222,
173.034573714903));
#26384=CARTESIAN_POINT('Ctrl Pts',(-59.7760553303807,-108.723233646833,
173.034573766048));
#26385=CARTESIAN_POINT('Ctrl Pts',(-60.6255492383249,-108.53839069231,173.898875727171));
#26386=CARTESIAN_POINT('Ctrl Pts',(-61.4750431462691,-108.353547737786,
174.763177688294));
#26387=CARTESIAN_POINT('Ctrl Pts',(-61.4651050324952,-108.260325978553,
175.985485192554));
#26388=CARTESIAN_POINT('Ctrl Pts',(-61.4551669187214,-108.167104219319,
177.207792696815));
#26389=CARTESIAN_POINT('Ctrl Pts',(-60.5857968130207,-108.165503652199,
178.072094585608));
#26390=CARTESIAN_POINT('Ctrl Pts',(-59.71642670732,-108.163903085079,178.936396474401));
#26391=CARTESIAN_POINT('Ctrl Pts',(-58.4910682444171,-108.200253255158,
178.936396423256));
#26392=CARTESIAN_POINT('Ctrl Pts',(-57.2657097815143,-108.236603425236,
178.936396372111));
#26393=CARTESIAN_POINT('Ctrl Pts',(-56.396339747736,-108.235002850448,178.072094410988));
#26394=CARTESIAN_POINT('Ctrl Pts',(-55.5269697139578,-108.233402275661,
177.207792449865));
#26395=CARTESIAN_POINT('Ctrl Pts',(-55.5170317018976,-108.140180505584,
175.985484945604));
#26396=CARTESIAN_POINT('Ctrl Pts',(-55.5070936898375,-108.046958735507,
174.763177441344));
#26397=CARTESIAN_POINT('Ctrl Pts',(-56.3565876697041,-107.862115773316,
173.89887555255));
#26398=CARTESIAN_POINT('Ctrl Pts',(-57.2060816495708,-107.677272811126,
173.034573663757));
#26399=CARTESIAN_POINT('Ctrl Pts',(-58.4115639866396,-107.454479111736,
173.034573714903));
#26400=CARTESIAN_POINT('Ctrl Pts',(-59.6170463237085,-107.231685412347,
173.034573766048));
#26401=CARTESIAN_POINT('Ctrl Pts',(-60.4665402316527,-107.046842457824,
173.898875727171));
#26402=CARTESIAN_POINT('Ctrl Pts',(-61.3160341395969,-106.861999503301,
174.763177688294));
#26403=CARTESIAN_POINT('Ctrl Pts',(-61.306096025823,-106.768777744067,175.985485192554));
#26404=CARTESIAN_POINT('Ctrl Pts',(-61.2961579120492,-106.675555984834,
177.207792696815));
#26405=CARTESIAN_POINT('Ctrl Pts',(-60.4267878063484,-106.673955417714,
178.072094585608));
#26406=CARTESIAN_POINT('Ctrl Pts',(-59.5574177006478,-106.672354850594,
178.936396474401));
#26407=CARTESIAN_POINT('Ctrl Pts',(-58.3320592377449,-106.708705020672,
178.936396423256));
#26408=CARTESIAN_POINT('Ctrl Pts',(-57.106700774842,-106.74505519075,178.936396372111));
#26409=CARTESIAN_POINT('Ctrl Pts',(-56.2373307410638,-106.743454615963,
178.072094410988));
#26410=CARTESIAN_POINT('Ctrl Pts',(-55.3679607072856,-106.741854041175,
177.207792449865));
#26411=CARTESIAN_POINT('Ctrl Pts',(-55.3580226952254,-106.648632271098,
175.985484945604));
#26412=CARTESIAN_POINT('Ctrl Pts',(-55.3480846831652,-106.555410501021,
174.763177441344));
#26413=CARTESIAN_POINT('Ctrl Pts',(-56.1975786630319,-106.370567538831,
173.89887555255));
#26414=CARTESIAN_POINT('Ctrl Pts',(-57.0470726428986,-106.18572457664,173.034573663757));
#26415=CARTESIAN_POINT('Ctrl Pts',(-58.2525549799674,-105.962930877251,
173.034573714903));
#26416=CARTESIAN_POINT('Ctrl Pts',(-59.4580373170363,-105.740137177862,
173.034573766048));
#26417=CARTESIAN_POINT('Ctrl Pts',(-60.3075312249805,-105.555294223339,
173.898875727171));
#26418=CARTESIAN_POINT('Ctrl Pts',(-61.1570251329247,-105.370451268815,
174.763177688294));
#26419=CARTESIAN_POINT('Ctrl Pts',(-61.1470870191508,-105.277229509582,
175.985485192554));
#26420=CARTESIAN_POINT('Ctrl Pts',(-61.1371489053769,-105.184007750348,
177.207792696815));
#26421=CARTESIAN_POINT('Ctrl Pts',(-60.2677787996762,-105.182407183228,
178.072094585608));
#26422=CARTESIAN_POINT('Ctrl Pts',(-59.3984086939755,-105.180806616108,
178.936396474401));
#26423=CARTESIAN_POINT('Ctrl Pts',(-58.1730502310727,-105.217156786186,
178.936396423256));
#26424=CARTESIAN_POINT('Ctrl Pts',(-56.9476917681698,-105.253506956265,
178.936396372111));
#26425=CARTESIAN_POINT('Ctrl Pts',(-56.0783217343916,-105.251906381477,
178.072094410988));
#26426=CARTESIAN_POINT('Ctrl Pts',(-55.2089517006133,-105.25030580669,177.207792449865));
#26427=CARTESIAN_POINT('Ctrl Pts',(-55.1990136885532,-105.157084036613,
175.985484945604));
#26428=CARTESIAN_POINT('Ctrl Pts',(-55.189075676493,-105.063862266536,174.763177441344));
#26429=CARTESIAN_POINT('Ctrl Pts',(-56.0385696563597,-104.879019304345,
173.89887555255));
#26430=CARTESIAN_POINT('Ctrl Pts',(-56.8880636362264,-104.694176342154,
173.034573663757));
#26431=CARTESIAN_POINT('Ctrl Pts',(-58.0935459732952,-104.471382642765,
173.034573714903));
#26432=CARTESIAN_POINT('Ctrl Pts',(-59.299028310364,-104.248588943376,173.034573766048));
#26433=CARTESIAN_POINT('Ctrl Pts',(-60.1485222183082,-104.063745988853,
173.898875727171));
#26434=CARTESIAN_POINT('Ctrl Pts',(-60.9980161262524,-103.87890303433,174.763177688294));
#26435=CARTESIAN_POINT('Ctrl Pts',(-60.9880780124786,-103.785681275096,
175.985485192554));
#26436=CARTESIAN_POINT('Ctrl Pts',(-60.9781398987047,-103.692459515862,
177.207792696815));
#26437=CARTESIAN_POINT('Ctrl Pts',(-60.108769793004,-103.690858948742,178.072094585608));
#26438=CARTESIAN_POINT('Ctrl Pts',(-59.2393996873033,-103.689258381622,
178.936396474401));
#26439=CARTESIAN_POINT('Ctrl Pts',(-58.0140412244004,-103.725608551701,
178.936396423256));
#26440=CARTESIAN_POINT('Ctrl Pts',(-56.7886827614976,-103.761958721779,
178.936396372111));
#26441=CARTESIAN_POINT('Ctrl Pts',(-55.9193127277193,-103.760358146992,
178.072094410988));
#26442=CARTESIAN_POINT('Ctrl Pts',(-55.0499426939411,-103.758757572204,
177.207792449865));
#26443=CARTESIAN_POINT('Ctrl Pts',(-55.0400046818809,-103.665535802127,
175.985484945604));
#26444=CARTESIAN_POINT('Ctrl Pts',(-55.0300666698208,-103.57231403205,174.763177441344));
#26445=CARTESIAN_POINT('Ctrl Pts',(-55.8795606496874,-103.387471069859,
173.89887555255));
#26446=CARTESIAN_POINT('Ctrl Pts',(-56.7290546295541,-103.202628107669,
173.034573663757));
#26447=CARTESIAN_POINT('Ctrl Pts',(-57.934536966623,-102.97983440828,173.034573714903));
#26448=CARTESIAN_POINT('Ctrl Pts',(-59.1400193036918,-102.757040708891,
173.034573766048));
#26449=CARTESIAN_POINT('Ctrl Pts',(-59.989513211636,-102.572197754367,173.898875727171));
#26450=CARTESIAN_POINT('Ctrl Pts',(-60.8390071195802,-102.387354799844,
174.763177688294));
#26451=CARTESIAN_POINT('Ctrl Pts',(-60.8290690058063,-102.29413304061,175.985485192554));
#26452=CARTESIAN_POINT('Ctrl Pts',(-60.8191308920325,-102.200911281377,
177.207792696815));
#26453=CARTESIAN_POINT('Ctrl Pts',(-59.9497607863318,-102.199310714257,
178.072094585608));
#26454=CARTESIAN_POINT('Ctrl Pts',(-59.0803906806311,-102.197710147137,
178.936396474401));
#26455=CARTESIAN_POINT('Ctrl Pts',(-57.8550322177282,-102.234060317215,
178.936396423256));
#26456=CARTESIAN_POINT('Ctrl Pts',(-56.6296737548253,-102.270410487293,
178.936396372111));
#26457=CARTESIAN_POINT('Ctrl Pts',(-55.7603037210471,-102.268809912506,
178.072094410988));
#26458=CARTESIAN_POINT('Ctrl Pts',(-54.8909336872689,-102.267209337719,
177.207792449865));
#26459=CARTESIAN_POINT('Ctrl Pts',(-54.8809956752087,-102.173987567642,
175.985484945604));
#26460=CARTESIAN_POINT('Ctrl Pts',(-54.8710576631486,-102.080765797565,
174.763177441344));
#26461=CARTESIAN_POINT('Ctrl Pts',(-55.7205516430152,-101.895922835374,
173.89887555255));
#26462=CARTESIAN_POINT('Ctrl Pts',(-56.5700456228819,-101.711079873183,
173.034573663757));
#26463=CARTESIAN_POINT('Ctrl Pts',(-57.7755279599507,-101.488286173794,
173.034573714903));
#26464=CARTESIAN_POINT('Ctrl Pts',(-58.9810102970196,-101.265492474405,
173.034573766048));
#26465=CARTESIAN_POINT('Ctrl Pts',(-59.8305042049638,-101.080649519882,
173.898875727171));
#26466=CARTESIAN_POINT('Ctrl Pts',(-60.679998112908,-100.895806565358,174.763177688294));
#26467=CARTESIAN_POINT('Ctrl Pts',(-60.6700599991341,-100.802584806125,
175.985485192554));
#26468=CARTESIAN_POINT('Ctrl Pts',(-60.6601218853602,-100.709363046891,
177.207792696815));
#26469=CARTESIAN_POINT('Ctrl Pts',(-59.7907517796595,-100.707762479771,
178.072094585608));
#26470=CARTESIAN_POINT('Ctrl Pts',(-58.9213816739588,-100.706161912651,
178.936396474401));
#26471=CARTESIAN_POINT('Ctrl Pts',(-57.696023211056,-100.742512082729,178.936396423256));
#26472=CARTESIAN_POINT('Ctrl Pts',(-56.4706647481531,-100.778862252808,
178.936396372111));
#26473=CARTESIAN_POINT('Ctrl Pts',(-55.6012947143749,-100.77726167802,178.072094410988));
#26474=CARTESIAN_POINT('Ctrl Pts',(-54.7319246805966,-100.775661103233,
177.207792449865));
#26475=CARTESIAN_POINT('Ctrl Pts',(-54.7219866685365,-100.682439333156,
175.985484945604));
#26476=CARTESIAN_POINT('Ctrl Pts',(-54.7120486564763,-100.589217563079,
174.763177441344));
#26477=CARTESIAN_POINT('Ctrl Pts',(-55.561542636343,-100.404374600888,173.89887555255));
#26478=CARTESIAN_POINT('Ctrl Pts',(-56.4110366162097,-100.219531638698,
173.034573663757));
#26479=CARTESIAN_POINT('Ctrl Pts',(-57.6165189532785,-99.9967379393085,
173.034573714903));
#26480=CARTESIAN_POINT('Ctrl Pts',(-58.8220012903473,-99.7739442399195,
173.034573766048));
#26481=CARTESIAN_POINT('Ctrl Pts',(-59.6714951982915,-99.5891012853962,
173.898875727171));
#26482=CARTESIAN_POINT('Ctrl Pts',(-60.5209891062358,-99.4042583308729,
174.763177688294));
#26483=CARTESIAN_POINT('Ctrl Pts',(-60.5110509924619,-99.3110365716392,
175.985485192554));
#26484=CARTESIAN_POINT('Ctrl Pts',(-60.501112878688,-99.2178148124055,177.207792696815));
#26485=CARTESIAN_POINT('Ctrl Pts',(-59.6317427729873,-99.2162142452855,
178.072094585608));
#26486=CARTESIAN_POINT('Ctrl Pts',(-58.7623726672866,-99.2146136781656,
178.936396474401));
#26487=CARTESIAN_POINT('Ctrl Pts',(-57.5370142043838,-99.2509638482439,
178.936396423256));
#26488=CARTESIAN_POINT('Ctrl Pts',(-56.3116557414809,-99.2873140183222,
178.936396372111));
#26489=CARTESIAN_POINT('Ctrl Pts',(-55.4422857077027,-99.2857134435348,
178.072094410988));
#26490=CARTESIAN_POINT('Ctrl Pts',(-54.5729156739244,-99.2841128687474,
177.207792449865));
#26491=CARTESIAN_POINT('Ctrl Pts',(-54.5629776618643,-99.1908910986704,
175.985484945604));
#26492=CARTESIAN_POINT('Ctrl Pts',(-54.5530396498041,-99.0976693285933,
174.763177441344));
#26493=CARTESIAN_POINT('Ctrl Pts',(-55.4025336296708,-98.9128263664026,
173.89887555255));
#26494=CARTESIAN_POINT('Ctrl Pts',(-56.2520276095374,-98.727983404212,173.034573663757));
#26495=CARTESIAN_POINT('Ctrl Pts',(-57.4575099466063,-98.5051897048229,
173.034573714903));
#26496=CARTESIAN_POINT('Ctrl Pts',(-58.6629922836751,-98.2823960054338,
173.034573766048));
#26497=CARTESIAN_POINT('Ctrl Pts',(-59.5124861916193,-98.0975530509106,
173.898875727171));
#26498=CARTESIAN_POINT('Ctrl Pts',(-60.3619800995635,-97.9127100963873,
174.763177688294));
#26499=CARTESIAN_POINT('Ctrl Pts',(-60.3520419857897,-97.8194883371536,
175.985485192554));
#26500=CARTESIAN_POINT('Ctrl Pts',(-60.3421038720158,-97.7262665779199,
177.207792696815));
#26501=CARTESIAN_POINT('Ctrl Pts',(-59.4727337663151,-97.7246660108,178.072094585608));
#26502=CARTESIAN_POINT('Ctrl Pts',(-58.6033636606144,-97.72306544368,178.936396474401));
#26503=CARTESIAN_POINT('Ctrl Pts',(-57.3780051977115,-97.7594156137583,
178.936396423256));
#26504=CARTESIAN_POINT('Ctrl Pts',(-56.1526467348087,-97.7957657838366,
178.936396372111));
#26505=CARTESIAN_POINT('Ctrl Pts',(-55.2832767010304,-97.7941652090492,
178.072094410988));
#26506=CARTESIAN_POINT('Ctrl Pts',(-56.1707931031902,-113.117197303651,
178.813912075476));
#26507=CARTESIAN_POINT('Ctrl Pts',(-54.9958834532485,-113.148169293224,
177.6423391512));
#26508=CARTESIAN_POINT('Ctrl Pts',(-54.9859454592686,-113.05494752122,175.985484901707));
#26509=CARTESIAN_POINT('Ctrl Pts',(-54.9760074652888,-112.961725749215,
174.328630652215));
#26510=CARTESIAN_POINT('Ctrl Pts',(-56.1310410868884,-112.744310219938,
173.157057825983));
#26511=CARTESIAN_POINT('Ctrl Pts',(-57.286074708488,-112.52689469066,171.985484999752));
#26512=CARTESIAN_POINT('Ctrl Pts',(-58.9236553326579,-112.258036427063,
171.985485069079));
#26513=CARTESIAN_POINT('Ctrl Pts',(-60.5612359568277,-111.989178163466,
171.985485138407));
#26514=CARTESIAN_POINT('Ctrl Pts',(-61.7162694809355,-111.771762644582,
173.157058062683));
#26515=CARTESIAN_POINT('Ctrl Pts',(-62.8713030050432,-111.554347125698,
174.328630986959));
#26516=CARTESIAN_POINT('Ctrl Pts',(-62.861364873189,-111.461125368392,175.985485236451));
#26517=CARTESIAN_POINT('Ctrl Pts',(-62.8514267413349,-111.367903611086,
177.642339485944));
#26518=CARTESIAN_POINT('Ctrl Pts',(-61.6765169939012,-111.398875611052,
178.813912312176));
#26519=CARTESIAN_POINT('Ctrl Pts',(-60.5016072464676,-111.429847611019,
179.985485138407));
#26520=CARTESIAN_POINT('Ctrl Pts',(-58.8441504964637,-111.512262345305,
179.985485069079));
#26521=CARTESIAN_POINT('Ctrl Pts',(-57.1866937464598,-111.594677079592,
179.985484999752));
#26522=CARTESIAN_POINT('Ctrl Pts',(-56.011784096518,-111.625649069165,178.813912075476));
#26523=CARTESIAN_POINT('Ctrl Pts',(-54.8368744465762,-111.656621058739,
177.6423391512));
#26524=CARTESIAN_POINT('Ctrl Pts',(-54.8269364525964,-111.563399286734,
175.985484901707));
#26525=CARTESIAN_POINT('Ctrl Pts',(-54.8169984586165,-111.47017751473,174.328630652215));
#26526=CARTESIAN_POINT('Ctrl Pts',(-55.9720320802161,-111.252761985452,
173.157057825983));
#26527=CARTESIAN_POINT('Ctrl Pts',(-57.1270657018158,-111.035346456175,
171.985484999752));
#26528=CARTESIAN_POINT('Ctrl Pts',(-58.7646463259856,-110.766488192578,
171.985485069079));
#26529=CARTESIAN_POINT('Ctrl Pts',(-60.4022269501555,-110.497629928981,
171.985485138407));
#26530=CARTESIAN_POINT('Ctrl Pts',(-61.5572604742632,-110.280214410097,
173.157058062683));
#26531=CARTESIAN_POINT('Ctrl Pts',(-62.712293998371,-110.062798891212,174.328630986959));
#26532=CARTESIAN_POINT('Ctrl Pts',(-62.7023558665168,-109.969577133906,
175.985485236451));
#26533=CARTESIAN_POINT('Ctrl Pts',(-62.6924177346626,-109.8763553766,177.642339485944));
#26534=CARTESIAN_POINT('Ctrl Pts',(-61.517507987229,-109.907327376567,178.813912312176));
#26535=CARTESIAN_POINT('Ctrl Pts',(-60.3425982397954,-109.938299376534,
179.985485138407));
#26536=CARTESIAN_POINT('Ctrl Pts',(-58.6851414897915,-110.02071411082,179.985485069079));
#26537=CARTESIAN_POINT('Ctrl Pts',(-57.0276847397876,-110.103128845106,
179.985484999752));
#26538=CARTESIAN_POINT('Ctrl Pts',(-55.8527750898458,-110.13410083468,178.813912075476));
#26539=CARTESIAN_POINT('Ctrl Pts',(-54.677865439904,-110.165072824253,177.6423391512));
#26540=CARTESIAN_POINT('Ctrl Pts',(-54.6679274459242,-110.071851052249,
175.985484901707));
#26541=CARTESIAN_POINT('Ctrl Pts',(-54.6579894519443,-109.978629280244,
174.328630652215));
#26542=CARTESIAN_POINT('Ctrl Pts',(-55.8130230735439,-109.761213750967,
173.157057825983));
#26543=CARTESIAN_POINT('Ctrl Pts',(-56.9680566951435,-109.543798221689,
171.985484999752));
#26544=CARTESIAN_POINT('Ctrl Pts',(-58.6056373193134,-109.274939958092,
171.985485069079));
#26545=CARTESIAN_POINT('Ctrl Pts',(-60.2432179434833,-109.006081694495,
171.985485138407));
#26546=CARTESIAN_POINT('Ctrl Pts',(-61.398251467591,-108.788666175611,173.157058062683));
#26547=CARTESIAN_POINT('Ctrl Pts',(-62.5532849916988,-108.571250656727,
174.328630986959));
#26548=CARTESIAN_POINT('Ctrl Pts',(-62.5433468598446,-108.478028899421,
175.985485236451));
#26549=CARTESIAN_POINT('Ctrl Pts',(-62.5334087279904,-108.384807142114,
177.642339485944));
#26550=CARTESIAN_POINT('Ctrl Pts',(-61.3584989805568,-108.415779142081,
178.813912312176));
#26551=CARTESIAN_POINT('Ctrl Pts',(-60.1835892331231,-108.446751142048,
179.985485138407));
#26552=CARTESIAN_POINT('Ctrl Pts',(-58.5261324831192,-108.529165876334,
179.985485069079));
#26553=CARTESIAN_POINT('Ctrl Pts',(-56.8686757331153,-108.611580610621,
179.985484999752));
#26554=CARTESIAN_POINT('Ctrl Pts',(-55.6937660831736,-108.642552600194,
178.813912075476));
#26555=CARTESIAN_POINT('Ctrl Pts',(-54.5188564332318,-108.673524589768,
177.6423391512));
#26556=CARTESIAN_POINT('Ctrl Pts',(-54.5089184392519,-108.580302817763,
175.985484901707));
#26557=CARTESIAN_POINT('Ctrl Pts',(-54.4989804452721,-108.487081045759,
174.328630652215));
#26558=CARTESIAN_POINT('Ctrl Pts',(-55.6540140668717,-108.269665516481,
173.157057825983));
#26559=CARTESIAN_POINT('Ctrl Pts',(-56.8090476884713,-108.052249987204,
171.985484999752));
#26560=CARTESIAN_POINT('Ctrl Pts',(-58.4466283126412,-107.783391723607,
171.985485069079));
#26561=CARTESIAN_POINT('Ctrl Pts',(-60.084208936811,-107.51453346001,171.985485138407));
#26562=CARTESIAN_POINT('Ctrl Pts',(-61.2392424609188,-107.297117941125,
173.157058062683));
#26563=CARTESIAN_POINT('Ctrl Pts',(-62.3942759850265,-107.079702422241,
174.328630986959));
#26564=CARTESIAN_POINT('Ctrl Pts',(-62.3843378531723,-106.986480664935,
175.985485236451));
#26565=CARTESIAN_POINT('Ctrl Pts',(-62.3743997213182,-106.893258907629,
177.642339485944));
#26566=CARTESIAN_POINT('Ctrl Pts',(-61.1994899738845,-106.924230907596,
178.813912312176));
#26567=CARTESIAN_POINT('Ctrl Pts',(-60.0245802264509,-106.955202907562,
179.985485138407));
#26568=CARTESIAN_POINT('Ctrl Pts',(-58.367123476447,-107.037617641849,179.985485069079));
#26569=CARTESIAN_POINT('Ctrl Pts',(-56.7096667264431,-107.120032376135,
179.985484999752));
#26570=CARTESIAN_POINT('Ctrl Pts',(-55.5347570765013,-107.151004365708,
178.813912075476));
#26571=CARTESIAN_POINT('Ctrl Pts',(-54.3598474265596,-107.181976355282,
177.6423391512));
#26572=CARTESIAN_POINT('Ctrl Pts',(-54.3499094325797,-107.088754583277,
175.985484901707));
#26573=CARTESIAN_POINT('Ctrl Pts',(-54.3399714385998,-106.995532811273,
174.328630652215));
#26574=CARTESIAN_POINT('Ctrl Pts',(-55.4950050601995,-106.778117281995,
173.157057825983));
#26575=CARTESIAN_POINT('Ctrl Pts',(-56.6500386817991,-106.560701752718,
171.985484999752));
#26576=CARTESIAN_POINT('Ctrl Pts',(-58.2876193059689,-106.291843489121,
171.985485069079));
#26577=CARTESIAN_POINT('Ctrl Pts',(-59.9251999301388,-106.022985225524,
171.985485138407));
#26578=CARTESIAN_POINT('Ctrl Pts',(-61.0802334542465,-105.80556970664,173.157058062683));
#26579=CARTESIAN_POINT('Ctrl Pts',(-62.2352669783543,-105.588154187756,
174.328630986959));
#26580=CARTESIAN_POINT('Ctrl Pts',(-62.2253288465001,-105.494932430449,
175.985485236451));
#26581=CARTESIAN_POINT('Ctrl Pts',(-62.2153907146459,-105.401710673143,
177.642339485944));
#26582=CARTESIAN_POINT('Ctrl Pts',(-61.0404809672123,-105.43268267311,178.813912312176));
#26583=CARTESIAN_POINT('Ctrl Pts',(-59.8655712197787,-105.463654673077,
179.985485138407));
#26584=CARTESIAN_POINT('Ctrl Pts',(-58.2081144697748,-105.546069407363,
179.985485069079));
#26585=CARTESIAN_POINT('Ctrl Pts',(-56.5506577197709,-105.628484141649,
179.985484999752));
#26586=CARTESIAN_POINT('Ctrl Pts',(-55.3757480698291,-105.659456131223,
178.813912075476));
#26587=CARTESIAN_POINT('Ctrl Pts',(-54.2008384198873,-105.690428120796,
177.6423391512));
#26588=CARTESIAN_POINT('Ctrl Pts',(-54.1909004259075,-105.597206348792,
175.985484901707));
#26589=CARTESIAN_POINT('Ctrl Pts',(-54.1809624319276,-105.503984576787,
174.328630652215));
#26590=CARTESIAN_POINT('Ctrl Pts',(-55.3359960535272,-105.28656904751,173.157057825983));
#26591=CARTESIAN_POINT('Ctrl Pts',(-56.4910296751268,-105.069153518232,
171.985484999752));
#26592=CARTESIAN_POINT('Ctrl Pts',(-58.1286102992967,-104.800295254635,
171.985485069079));
#26593=CARTESIAN_POINT('Ctrl Pts',(-59.7661909234666,-104.531436991038,
171.985485138407));
#26594=CARTESIAN_POINT('Ctrl Pts',(-60.9212244475743,-104.314021472154,
173.157058062683));
#26595=CARTESIAN_POINT('Ctrl Pts',(-62.0762579716821,-104.09660595327,174.328630986959));
#26596=CARTESIAN_POINT('Ctrl Pts',(-62.0663198398279,-104.003384195964,
175.985485236451));
#26597=CARTESIAN_POINT('Ctrl Pts',(-62.0563817079737,-103.910162438658,
177.642339485944));
#26598=CARTESIAN_POINT('Ctrl Pts',(-60.8814719605401,-103.941134438624,
178.813912312176));
#26599=CARTESIAN_POINT('Ctrl Pts',(-59.7065622131064,-103.972106438591,
179.985485138407));
#26600=CARTESIAN_POINT('Ctrl Pts',(-58.0491054631025,-104.054521172878,
179.985485069079));
#26601=CARTESIAN_POINT('Ctrl Pts',(-56.3916487130987,-104.136935907164,
179.985484999752));
#26602=CARTESIAN_POINT('Ctrl Pts',(-55.2167390631569,-104.167907896737,
178.813912075476));
#26603=CARTESIAN_POINT('Ctrl Pts',(-54.0418294132151,-104.198879886311,
177.6423391512));
#26604=CARTESIAN_POINT('Ctrl Pts',(-54.0318914192353,-104.105658114306,
175.985484901707));
#26605=CARTESIAN_POINT('Ctrl Pts',(-54.0219534252554,-104.012436342302,
174.328630652215));
#26606=CARTESIAN_POINT('Ctrl Pts',(-55.176987046855,-103.795020813024,173.157057825983));
#26607=CARTESIAN_POINT('Ctrl Pts',(-56.3320206684546,-103.577605283747,
171.985484999752));
#26608=CARTESIAN_POINT('Ctrl Pts',(-57.9696012926245,-103.30874702015,171.985485069079));
#26609=CARTESIAN_POINT('Ctrl Pts',(-59.6071819167943,-103.039888756553,
171.985485138407));
#26610=CARTESIAN_POINT('Ctrl Pts',(-60.7622154409021,-102.822473237669,
173.157058062683));
#26611=CARTESIAN_POINT('Ctrl Pts',(-61.9172489650099,-102.605057718784,
174.328630986959));
#26612=CARTESIAN_POINT('Ctrl Pts',(-61.9073108331557,-102.511835961478,
175.985485236451));
#26613=CARTESIAN_POINT('Ctrl Pts',(-61.8973727013015,-102.418614204172,
177.642339485944));
#26614=CARTESIAN_POINT('Ctrl Pts',(-60.7224629538678,-102.449586204139,
178.813912312176));
#26615=CARTESIAN_POINT('Ctrl Pts',(-59.5475532064342,-102.480558204106,
179.985485138407));
#26616=CARTESIAN_POINT('Ctrl Pts',(-57.8900964564303,-102.562972938392,
179.985485069079));
#26617=CARTESIAN_POINT('Ctrl Pts',(-56.2326397064264,-102.645387672678,
179.985484999752));
#26618=CARTESIAN_POINT('Ctrl Pts',(-55.0577300564847,-102.676359662252,
178.813912075476));
#26619=CARTESIAN_POINT('Ctrl Pts',(-53.8828204065429,-102.707331651825,
177.6423391512));
#26620=CARTESIAN_POINT('Ctrl Pts',(-53.872882412563,-102.614109879821,175.985484901707));
#26621=CARTESIAN_POINT('Ctrl Pts',(-53.8629444185832,-102.520888107816,
174.328630652215));
#26622=CARTESIAN_POINT('Ctrl Pts',(-55.0179780401828,-102.303472578539,
173.157057825983));
#26623=CARTESIAN_POINT('Ctrl Pts',(-56.1730116617824,-102.086057049261,
171.985484999752));
#26624=CARTESIAN_POINT('Ctrl Pts',(-57.8105922859523,-101.817198785664,
171.985485069079));
#26625=CARTESIAN_POINT('Ctrl Pts',(-59.4481729101221,-101.548340522067,
171.985485138407));
#26626=CARTESIAN_POINT('Ctrl Pts',(-60.6032064342299,-101.330925003183,
173.157058062683));
#26627=CARTESIAN_POINT('Ctrl Pts',(-61.7582399583376,-101.113509484299,
174.328630986959));
#26628=CARTESIAN_POINT('Ctrl Pts',(-61.7483018264834,-101.020287726993,
175.985485236451));
#26629=CARTESIAN_POINT('Ctrl Pts',(-61.7383636946293,-100.927065969686,
177.642339485944));
#26630=CARTESIAN_POINT('Ctrl Pts',(-60.5634539471956,-100.958037969653,
178.813912312176));
#26631=CARTESIAN_POINT('Ctrl Pts',(-59.388544199762,-100.98900996962,179.985485138407));
#26632=CARTESIAN_POINT('Ctrl Pts',(-57.7310874497581,-101.071424703906,
179.985485069079));
#26633=CARTESIAN_POINT('Ctrl Pts',(-56.0736306997542,-101.153839438193,
179.985484999752));
#26634=CARTESIAN_POINT('Ctrl Pts',(-54.8987210498124,-101.184811427766,
178.813912075476));
#26635=CARTESIAN_POINT('Ctrl Pts',(-53.7238113998707,-101.21578341734,177.6423391512));
#26636=CARTESIAN_POINT('Ctrl Pts',(-53.7138734058908,-101.122561645335,
175.985484901707));
#26637=CARTESIAN_POINT('Ctrl Pts',(-53.7039354119109,-101.029339873331,
174.328630652215));
#26638=CARTESIAN_POINT('Ctrl Pts',(-54.8589690335105,-100.811924344053,
173.157057825983));
#26639=CARTESIAN_POINT('Ctrl Pts',(-56.0140026551102,-100.594508814776,
171.985484999752));
#26640=CARTESIAN_POINT('Ctrl Pts',(-57.65158327928,-100.325650551179,171.985485069079));
#26641=CARTESIAN_POINT('Ctrl Pts',(-59.2891639034499,-100.056792287582,
171.985485138407));
#26642=CARTESIAN_POINT('Ctrl Pts',(-60.4441974275576,-99.8393767686974,
173.157058062683));
#26643=CARTESIAN_POINT('Ctrl Pts',(-61.5992309516654,-99.6219612498133,
174.328630986959));
#26644=CARTESIAN_POINT('Ctrl Pts',(-61.5892928198112,-99.528739492507,175.985485236451));
#26645=CARTESIAN_POINT('Ctrl Pts',(-61.579354687957,-99.4355177352008,177.642339485944));
#26646=CARTESIAN_POINT('Ctrl Pts',(-60.4044449405234,-99.4664897351676,
178.813912312176));
#26647=CARTESIAN_POINT('Ctrl Pts',(-59.2295351930898,-99.4974617351344,
179.985485138407));
#26648=CARTESIAN_POINT('Ctrl Pts',(-57.5720784430859,-99.5798764694207,
179.985485069079));
#26649=CARTESIAN_POINT('Ctrl Pts',(-55.914621693082,-99.662291203707,179.985484999752));
#26650=CARTESIAN_POINT('Ctrl Pts',(-54.7397120431402,-99.6932631932805,
178.813912075476));
#26651=CARTESIAN_POINT('Ctrl Pts',(-53.5648023931984,-99.724235182854,177.6423391512));
#26652=CARTESIAN_POINT('Ctrl Pts',(-53.5548643992186,-99.6310134108495,
175.985484901707));
#26653=CARTESIAN_POINT('Ctrl Pts',(-53.5449264052387,-99.5377916388449,
174.328630652215));
#26654=CARTESIAN_POINT('Ctrl Pts',(-54.6999600268383,-99.3203761095675,
173.157057825983));
#26655=CARTESIAN_POINT('Ctrl Pts',(-55.8549936484379,-99.10296058029,171.985484999752));
#26656=CARTESIAN_POINT('Ctrl Pts',(-57.4925742726078,-98.834102316693,171.985485069079));
#26657=CARTESIAN_POINT('Ctrl Pts',(-59.1301548967777,-98.565244053096,171.985485138407));
#26658=CARTESIAN_POINT('Ctrl Pts',(-60.2851884208854,-98.3478285342118,
173.157058062683));
#26659=CARTESIAN_POINT('Ctrl Pts',(-61.4402219449932,-98.1304130153276,
174.328630986959));
#26660=CARTESIAN_POINT('Ctrl Pts',(-61.430283813139,-98.0371912580215,175.985485236451));
#26661=CARTESIAN_POINT('Ctrl Pts',(-61.4203456812848,-97.9439695007152,
177.642339485944));
#26662=CARTESIAN_POINT('Ctrl Pts',(-60.2454359338512,-97.974941500682,178.813912312176));
#26663=CARTESIAN_POINT('Ctrl Pts',(-59.0705261864175,-98.0059135006488,
179.985485138407));
#26664=CARTESIAN_POINT('Ctrl Pts',(-57.4130694364136,-98.0883282349351,
179.985485069079));
#26665=CARTESIAN_POINT('Ctrl Pts',(-55.7556126864097,-98.1707429692214,
179.985484999752));
#26666=CARTESIAN_POINT('Ctrl Pts',(-54.580703036468,-98.2017149587949,178.813912075476));
#26667=CARTESIAN_POINT('Ctrl Pts',(-61.6536146045897,-108.409937955922,
178.485485069079));
#26668=CARTESIAN_POINT('Ctrl Pts',(-61.5150424002329,-108.411652473799,
178.657813499464));
#26669=CARTESIAN_POINT('Ctrl Pts',(-61.3584989805568,-108.415779142081,
178.813912312176));
#26670=CARTESIAN_POINT('Ctrl Pts',(-60.1835892331231,-108.446751142048,
179.985485138407));
#26671=CARTESIAN_POINT('Ctrl Pts',(-58.5261324831192,-108.529165876334,
179.985485069079));
#26672=CARTESIAN_POINT('Ctrl Pts',(-56.8686757331153,-108.611580610621,
179.985484999752));
#26673=CARTESIAN_POINT('Ctrl Pts',(-55.6937660831736,-108.642552600194,
178.813912075476));
#26674=CARTESIAN_POINT('Ctrl Pts',(-54.5188564332318,-108.673524589768,
177.6423391512));
#26675=CARTESIAN_POINT('Ctrl Pts',(-54.5089184392519,-108.580302817763,
175.985484901707));
#26676=CARTESIAN_POINT('Ctrl Pts',(-54.4989804452721,-108.487081045759,
174.328630652215));
#26677=CARTESIAN_POINT('Ctrl Pts',(-55.6540140668717,-108.269665516481,
173.157057825983));
#26678=CARTESIAN_POINT('Ctrl Pts',(-56.8090476884713,-108.052249987204,
171.985484999752));
#26679=CARTESIAN_POINT('Ctrl Pts',(-58.4466283126412,-107.783391723607,
171.985485069079));
#26680=CARTESIAN_POINT('Ctrl Pts',(-60.084208936811,-107.51453346001,171.985485138407));
#26681=CARTESIAN_POINT('Ctrl Pts',(-61.2392424609188,-107.297117941125,
173.157058062683));
#26682=CARTESIAN_POINT('Ctrl Pts',(-61.3931374818719,-107.268149807183,
173.313156769748));
#26683=CARTESIAN_POINT('Ctrl Pts',(-61.5289566858427,-107.240612378001,
173.485485069079));
#26684=CARTESIAN_POINT('Ctrl Pts',(-56.1707931031902,-113.117197303651,
178.813912075476));
#26685=CARTESIAN_POINT('Ctrl Pts',(-54.9958834532485,-113.148169293224,
177.6423391512));
#26686=CARTESIAN_POINT('Ctrl Pts',(-54.9859454592686,-113.05494752122,175.985484901707));
#26687=CARTESIAN_POINT('Ctrl Pts',(-54.9760074652888,-112.961725749215,
174.328630652215));
#26688=CARTESIAN_POINT('Ctrl Pts',(-56.1310410868884,-112.744310219938,
173.157057825983));
#26689=CARTESIAN_POINT('Ctrl Pts',(-57.286074708488,-112.52689469066,171.985484999752));
#26690=CARTESIAN_POINT('Ctrl Pts',(-58.9236553326578,-112.258036427063,
171.985485069079));
#26691=CARTESIAN_POINT('Ctrl Pts',(-60.5612359568277,-111.989178163466,
171.985485138407));
#26692=CARTESIAN_POINT('Ctrl Pts',(-61.7162694809355,-111.771762644582,
173.157058062683));
#26693=CARTESIAN_POINT('Ctrl Pts',(-62.8713030050432,-111.554347125698,
174.328630986959));
#26694=CARTESIAN_POINT('Ctrl Pts',(-62.861364873189,-111.461125368392,175.985485236451));
#26695=CARTESIAN_POINT('Ctrl Pts',(-62.8514267413349,-111.367903611086,
177.642339485944));
#26696=CARTESIAN_POINT('Ctrl Pts',(-61.6765169939012,-111.398875611052,
178.813912312176));
#26697=CARTESIAN_POINT('Ctrl Pts',(-60.5016072464676,-111.429847611019,
179.985485138407));
#26698=CARTESIAN_POINT('Ctrl Pts',(-58.8441504964637,-111.512262345305,
179.985485069079));
#26699=CARTESIAN_POINT('Ctrl Pts',(-57.1866937464598,-111.594677079592,
179.985484999752));
#26700=CARTESIAN_POINT('Ctrl Pts',(-56.011784096518,-111.625649069165,178.813912075476));
#26701=CARTESIAN_POINT('Ctrl Pts',(-54.8368744465763,-111.656621058739,
177.6423391512));
#26702=CARTESIAN_POINT('Ctrl Pts',(-54.8269364525964,-111.563399286734,
175.985484901707));
#26703=CARTESIAN_POINT('Ctrl Pts',(-54.8169984586165,-111.47017751473,174.328630652215));
#26704=CARTESIAN_POINT('Ctrl Pts',(-55.9720320802161,-111.252761985452,
173.157057825983));
#26705=CARTESIAN_POINT('Ctrl Pts',(-57.1270657018158,-111.035346456175,
171.985484999752));
#26706=CARTESIAN_POINT('Ctrl Pts',(-58.7646463259856,-110.766488192578,
171.985485069079));
#26707=CARTESIAN_POINT('Ctrl Pts',(-60.4022269501555,-110.497629928981,
171.985485138407));
#26708=CARTESIAN_POINT('Ctrl Pts',(-61.5572604742632,-110.280214410097,
173.157058062683));
#26709=CARTESIAN_POINT('Ctrl Pts',(-62.712293998371,-110.062798891212,174.328630986959));
#26710=CARTESIAN_POINT('Ctrl Pts',(-62.7023558665168,-109.969577133906,
175.985485236451));
#26711=CARTESIAN_POINT('Ctrl Pts',(-62.6924177346626,-109.8763553766,177.642339485944));
#26712=CARTESIAN_POINT('Ctrl Pts',(-61.517507987229,-109.907327376567,178.813912312176));
#26713=CARTESIAN_POINT('Ctrl Pts',(-60.3425982397954,-109.938299376534,
179.985485138407));
#26714=CARTESIAN_POINT('Ctrl Pts',(-58.6851414897915,-110.02071411082,179.985485069079));
#26715=CARTESIAN_POINT('Ctrl Pts',(-57.0276847397876,-110.103128845106,
179.985484999752));
#26716=CARTESIAN_POINT('Ctrl Pts',(-55.8527750898458,-110.13410083468,178.813912075476));
#26717=CARTESIAN_POINT('Ctrl Pts',(-54.677865439904,-110.165072824253,177.6423391512));
#26718=CARTESIAN_POINT('Ctrl Pts',(-54.6679274459242,-110.071851052249,
175.985484901707));
#26719=CARTESIAN_POINT('Ctrl Pts',(-54.6579894519443,-109.978629280244,
174.328630652215));
#26720=CARTESIAN_POINT('Ctrl Pts',(-55.8130230735439,-109.761213750967,
173.157057825983));
#26721=CARTESIAN_POINT('Ctrl Pts',(-56.9680566951435,-109.543798221689,
171.985484999752));
#26722=CARTESIAN_POINT('Ctrl Pts',(-58.6056373193134,-109.274939958092,
171.985485069079));
#26723=CARTESIAN_POINT('Ctrl Pts',(-60.2432179434833,-109.006081694495,
171.985485138407));
#26724=CARTESIAN_POINT('Ctrl Pts',(-61.398251467591,-108.788666175611,173.157058062683));
#26725=CARTESIAN_POINT('Ctrl Pts',(-62.5532849916988,-108.571250656727,
174.328630986959));
#26726=CARTESIAN_POINT('Ctrl Pts',(-62.5433468598446,-108.478028899421,
175.985485236451));
#26727=CARTESIAN_POINT('Ctrl Pts',(-62.5334087279904,-108.384807142114,
177.642339485944));
#26728=CARTESIAN_POINT('Ctrl Pts',(-61.3584989805568,-108.415779142081,
178.813912312176));
#26729=CARTESIAN_POINT('Ctrl Pts',(-60.1835892331231,-108.446751142048,
179.985485138407));
#26730=CARTESIAN_POINT('Ctrl Pts',(-58.5261324831192,-108.529165876334,
179.985485069079));
#26731=CARTESIAN_POINT('Ctrl Pts',(-56.8686757331153,-108.611580610621,
179.985484999752));
#26732=CARTESIAN_POINT('Ctrl Pts',(-55.6937660831736,-108.642552600194,
178.813912075476));
#26733=CARTESIAN_POINT('Ctrl Pts',(-54.5188564332318,-108.673524589768,
177.6423391512));
#26734=CARTESIAN_POINT('Ctrl Pts',(-54.5089184392519,-108.580302817763,
175.985484901707));
#26735=CARTESIAN_POINT('Ctrl Pts',(-54.4989804452721,-108.487081045759,
174.328630652215));
#26736=CARTESIAN_POINT('Ctrl Pts',(-55.6540140668717,-108.269665516481,
173.157057825983));
#26737=CARTESIAN_POINT('Ctrl Pts',(-56.8090476884713,-108.052249987204,
171.985484999752));
#26738=CARTESIAN_POINT('Ctrl Pts',(-58.4466283126412,-107.783391723607,
171.985485069079));
#26739=CARTESIAN_POINT('Ctrl Pts',(-60.084208936811,-107.51453346001,171.985485138407));
#26740=CARTESIAN_POINT('Ctrl Pts',(-61.2392424609188,-107.297117941125,
173.157058062683));
#26741=CARTESIAN_POINT('Ctrl Pts',(-62.3942759850265,-107.079702422241,
174.328630986959));
#26742=CARTESIAN_POINT('Ctrl Pts',(-62.3843378531723,-106.986480664935,
175.985485236451));
#26743=CARTESIAN_POINT('Ctrl Pts',(-62.3743997213182,-106.893258907629,
177.642339485944));
#26744=CARTESIAN_POINT('Ctrl Pts',(-61.1994899738845,-106.924230907596,
178.813912312176));
#26745=CARTESIAN_POINT('Ctrl Pts',(-60.0245802264509,-106.955202907562,
179.985485138407));
#26746=CARTESIAN_POINT('Ctrl Pts',(-58.367123476447,-107.037617641849,179.985485069079));
#26747=CARTESIAN_POINT('Ctrl Pts',(-56.7096667264431,-107.120032376135,
179.985484999752));
#26748=CARTESIAN_POINT('Ctrl Pts',(-55.5347570765013,-107.151004365708,
178.813912075476));
#26749=CARTESIAN_POINT('Ctrl Pts',(-54.3598474265596,-107.181976355282,
177.6423391512));
#26750=CARTESIAN_POINT('Ctrl Pts',(-54.3499094325797,-107.088754583277,
175.985484901707));
#26751=CARTESIAN_POINT('Ctrl Pts',(-54.3399714385998,-106.995532811273,
174.328630652215));
#26752=CARTESIAN_POINT('Ctrl Pts',(-55.4950050601995,-106.778117281995,
173.157057825983));
#26753=CARTESIAN_POINT('Ctrl Pts',(-56.6500386817991,-106.560701752718,
171.985484999752));
#26754=CARTESIAN_POINT('Ctrl Pts',(-58.2876193059689,-106.291843489121,
171.985485069079));
#26755=CARTESIAN_POINT('Ctrl Pts',(-59.9251999301388,-106.022985225524,
171.985485138407));
#26756=CARTESIAN_POINT('Ctrl Pts',(-61.0802334542465,-105.80556970664,173.157058062683));
#26757=CARTESIAN_POINT('Ctrl Pts',(-62.2352669783543,-105.588154187756,
174.328630986959));
#26758=CARTESIAN_POINT('Ctrl Pts',(-62.2253288465001,-105.494932430449,
175.985485236451));
#26759=CARTESIAN_POINT('Ctrl Pts',(-62.2153907146459,-105.401710673143,
177.642339485944));
#26760=CARTESIAN_POINT('Ctrl Pts',(-61.0404809672123,-105.43268267311,178.813912312176));
#26761=CARTESIAN_POINT('Ctrl Pts',(-59.8655712197787,-105.463654673077,
179.985485138407));
#26762=CARTESIAN_POINT('Ctrl Pts',(-58.2081144697748,-105.546069407363,
179.985485069079));
#26763=CARTESIAN_POINT('Ctrl Pts',(-56.5506577197709,-105.628484141649,
179.985484999752));
#26764=CARTESIAN_POINT('Ctrl Pts',(-55.3757480698291,-105.659456131223,
178.813912075476));
#26765=CARTESIAN_POINT('Ctrl Pts',(-54.2008384198873,-105.690428120796,
177.6423391512));
#26766=CARTESIAN_POINT('Ctrl Pts',(-54.1909004259075,-105.597206348792,
175.985484901707));
#26767=CARTESIAN_POINT('Ctrl Pts',(-54.1809624319276,-105.503984576787,
174.328630652215));
#26768=CARTESIAN_POINT('Ctrl Pts',(-55.3359960535272,-105.28656904751,173.157057825983));
#26769=CARTESIAN_POINT('Ctrl Pts',(-56.4910296751268,-105.069153518232,
171.985484999752));
#26770=CARTESIAN_POINT('Ctrl Pts',(-58.1286102992967,-104.800295254635,
171.985485069079));
#26771=CARTESIAN_POINT('Ctrl Pts',(-59.7661909234666,-104.531436991038,
171.985485138407));
#26772=CARTESIAN_POINT('Ctrl Pts',(-60.9212244475743,-104.314021472154,
173.157058062683));
#26773=CARTESIAN_POINT('Ctrl Pts',(-62.0762579716821,-104.09660595327,174.328630986959));
#26774=CARTESIAN_POINT('Ctrl Pts',(-62.0663198398279,-104.003384195964,
175.985485236451));
#26775=CARTESIAN_POINT('Ctrl Pts',(-62.0563817079737,-103.910162438658,
177.642339485944));
#26776=CARTESIAN_POINT('Ctrl Pts',(-60.8814719605401,-103.941134438624,
178.813912312176));
#26777=CARTESIAN_POINT('Ctrl Pts',(-59.7065622131064,-103.972106438591,
179.985485138407));
#26778=CARTESIAN_POINT('Ctrl Pts',(-58.0491054631025,-104.054521172878,
179.985485069079));
#26779=CARTESIAN_POINT('Ctrl Pts',(-56.3916487130987,-104.136935907164,
179.985484999752));
#26780=CARTESIAN_POINT('Ctrl Pts',(-55.2167390631569,-104.167907896737,
178.813912075476));
#26781=CARTESIAN_POINT('Ctrl Pts',(-54.0418294132151,-104.198879886311,
177.6423391512));
#26782=CARTESIAN_POINT('Ctrl Pts',(-54.0318914192353,-104.105658114306,
175.985484901707));
#26783=CARTESIAN_POINT('Ctrl Pts',(-54.0219534252554,-104.012436342302,
174.328630652215));
#26784=CARTESIAN_POINT('Ctrl Pts',(-55.176987046855,-103.795020813024,173.157057825983));
#26785=CARTESIAN_POINT('Ctrl Pts',(-56.3320206684546,-103.577605283747,
171.985484999752));
#26786=CARTESIAN_POINT('Ctrl Pts',(-57.9696012926245,-103.30874702015,171.985485069079));
#26787=CARTESIAN_POINT('Ctrl Pts',(-59.6071819167943,-103.039888756553,
171.985485138407));
#26788=CARTESIAN_POINT('Ctrl Pts',(-60.7622154409021,-102.822473237669,
173.157058062683));
#26789=CARTESIAN_POINT('Ctrl Pts',(-61.9172489650099,-102.605057718784,
174.328630986959));
#26790=CARTESIAN_POINT('Ctrl Pts',(-61.9073108331557,-102.511835961478,
175.985485236451));
#26791=CARTESIAN_POINT('Ctrl Pts',(-61.8973727013015,-102.418614204172,
177.642339485944));
#26792=CARTESIAN_POINT('Ctrl Pts',(-60.7224629538678,-102.449586204139,
178.813912312176));
#26793=CARTESIAN_POINT('Ctrl Pts',(-59.5475532064342,-102.480558204106,
179.985485138407));
#26794=CARTESIAN_POINT('Ctrl Pts',(-57.8900964564303,-102.562972938392,
179.985485069079));
#26795=CARTESIAN_POINT('Ctrl Pts',(-56.2326397064264,-102.645387672678,
179.985484999752));
#26796=CARTESIAN_POINT('Ctrl Pts',(-55.0577300564847,-102.676359662252,
178.813912075476));
#26797=CARTESIAN_POINT('Ctrl Pts',(-53.8828204065429,-102.707331651825,
177.6423391512));
#26798=CARTESIAN_POINT('Ctrl Pts',(-53.872882412563,-102.614109879821,175.985484901707));
#26799=CARTESIAN_POINT('Ctrl Pts',(-53.8629444185832,-102.520888107816,
174.328630652215));
#26800=CARTESIAN_POINT('Ctrl Pts',(-55.0179780401828,-102.303472578539,
173.157057825983));
#26801=CARTESIAN_POINT('Ctrl Pts',(-56.1730116617824,-102.086057049261,
171.985484999752));
#26802=CARTESIAN_POINT('Ctrl Pts',(-57.8105922859523,-101.817198785664,
171.985485069079));
#26803=CARTESIAN_POINT('Ctrl Pts',(-59.4481729101221,-101.548340522067,
171.985485138407));
#26804=CARTESIAN_POINT('Ctrl Pts',(-60.6032064342299,-101.330925003183,
173.157058062683));
#26805=CARTESIAN_POINT('Ctrl Pts',(-61.7582399583376,-101.113509484299,
174.328630986959));
#26806=CARTESIAN_POINT('Ctrl Pts',(-61.7483018264834,-101.020287726993,
175.985485236451));
#26807=CARTESIAN_POINT('Ctrl Pts',(-61.7383636946293,-100.927065969686,
177.642339485944));
#26808=CARTESIAN_POINT('Ctrl Pts',(-60.5634539471956,-100.958037969653,
178.813912312176));
#26809=CARTESIAN_POINT('Ctrl Pts',(-59.388544199762,-100.98900996962,179.985485138407));
#26810=CARTESIAN_POINT('Ctrl Pts',(-57.7310874497581,-101.071424703906,
179.985485069079));
#26811=CARTESIAN_POINT('Ctrl Pts',(-56.0736306997542,-101.153839438193,
179.985484999752));
#26812=CARTESIAN_POINT('Ctrl Pts',(-54.8987210498124,-101.184811427766,
178.813912075476));
#26813=CARTESIAN_POINT('Ctrl Pts',(-53.7238113998707,-101.21578341734,177.6423391512));
#26814=CARTESIAN_POINT('Ctrl Pts',(-53.7138734058908,-101.122561645335,
175.985484901707));
#26815=CARTESIAN_POINT('Ctrl Pts',(-53.7039354119109,-101.029339873331,
174.328630652215));
#26816=CARTESIAN_POINT('Ctrl Pts',(-54.8589690335105,-100.811924344053,
173.157057825983));
#26817=CARTESIAN_POINT('Ctrl Pts',(-56.0140026551102,-100.594508814776,
171.985484999752));
#26818=CARTESIAN_POINT('Ctrl Pts',(-57.65158327928,-100.325650551179,171.985485069079));
#26819=CARTESIAN_POINT('Ctrl Pts',(-59.2891639034499,-100.056792287582,
171.985485138407));
#26820=CARTESIAN_POINT('Ctrl Pts',(-60.4441974275576,-99.8393767686974,
173.157058062683));
#26821=CARTESIAN_POINT('Ctrl Pts',(-61.5992309516654,-99.6219612498133,
174.328630986959));
#26822=CARTESIAN_POINT('Ctrl Pts',(-61.5892928198112,-99.528739492507,175.985485236451));
#26823=CARTESIAN_POINT('Ctrl Pts',(-61.579354687957,-99.4355177352008,177.642339485944));
#26824=CARTESIAN_POINT('Ctrl Pts',(-60.4044449405234,-99.4664897351676,
178.813912312176));
#26825=CARTESIAN_POINT('Ctrl Pts',(-59.2295351930898,-99.4974617351344,
179.985485138407));
#26826=CARTESIAN_POINT('Ctrl Pts',(-57.5720784430859,-99.5798764694207,
179.985485069079));
#26827=CARTESIAN_POINT('Ctrl Pts',(-55.914621693082,-99.662291203707,179.985484999752));
#26828=CARTESIAN_POINT('Ctrl Pts',(-54.7397120431402,-99.6932631932805,
178.813912075476));
#26829=CARTESIAN_POINT('Ctrl Pts',(-53.5648023931984,-99.724235182854,177.6423391512));
#26830=CARTESIAN_POINT('Ctrl Pts',(-53.5548643992186,-99.6310134108495,
175.985484901707));
#26831=CARTESIAN_POINT('Ctrl Pts',(-53.5449264052387,-99.5377916388449,
174.328630652215));
#26832=CARTESIAN_POINT('Ctrl Pts',(-54.6999600268383,-99.3203761095675,
173.157057825983));
#26833=CARTESIAN_POINT('Ctrl Pts',(-55.8549936484379,-99.10296058029,171.985484999752));
#26834=CARTESIAN_POINT('Ctrl Pts',(-57.4925742726078,-98.834102316693,171.985485069079));
#26835=CARTESIAN_POINT('Ctrl Pts',(-59.1301548967777,-98.5652440530961,
171.985485138407));
#26836=CARTESIAN_POINT('Ctrl Pts',(-60.2851884208854,-98.3478285342118,
173.157058062683));
#26837=CARTESIAN_POINT('Ctrl Pts',(-61.4402219449932,-98.1304130153276,
174.328630986959));
#26838=CARTESIAN_POINT('Ctrl Pts',(-61.430283813139,-98.0371912580215,175.985485236451));
#26839=CARTESIAN_POINT('Ctrl Pts',(-61.4203456812848,-97.9439695007152,
177.642339485944));
#26840=CARTESIAN_POINT('Ctrl Pts',(-60.2454359338512,-97.974941500682,178.813912312176));
#26841=CARTESIAN_POINT('Ctrl Pts',(-59.0705261864175,-98.0059135006488,
179.985485138407));
#26842=CARTESIAN_POINT('Ctrl Pts',(-57.4130694364136,-98.0883282349351,
179.985485069079));
#26843=CARTESIAN_POINT('Ctrl Pts',(-55.7556126864097,-98.1707429692214,
179.985484999752));
#26844=CARTESIAN_POINT('Ctrl Pts',(-54.580703036468,-98.2017149587949,178.813912075476));
#26845=CARTESIAN_POINT('Ctrl Pts',(-56.181115489574,-113.283598570176,178.821287383467));
#26846=CARTESIAN_POINT('Ctrl Pts',(-55.0031681001975,-113.314894403068,
177.646659506339));
#26847=CARTESIAN_POINT('Ctrl Pts',(-54.9932301063974,-113.221672631044,
175.985484901271));
#26848=CARTESIAN_POINT('Ctrl Pts',(-54.9832921125973,-113.12845085902,174.324310296203));
#26849=CARTESIAN_POINT('Ctrl Pts',(-56.1413634738858,-112.910711486397,
173.149682517375));
#26850=CARTESIAN_POINT('Ctrl Pts',(-57.2994348351743,-112.692972113774,
171.975054738546));
#26851=CARTESIAN_POINT('Ctrl Pts',(-58.9413114718314,-112.423655866545,
171.975054808055));
#26852=CARTESIAN_POINT('Ctrl Pts',(-60.5831881084886,-112.154339619316,
171.975054877564));
#26853=CARTESIAN_POINT('Ctrl Pts',(-61.741259372031,-111.936600257113,173.149682754692));
#26854=CARTESIAN_POINT('Ctrl Pts',(-62.8993306355734,-111.71886089491,174.32431063182));
#26855=CARTESIAN_POINT('Ctrl Pts',(-62.8893925035395,-111.625639137623,
175.985485236888));
#26856=CARTESIAN_POINT('Ctrl Pts',(-62.8794543715055,-111.532417380336,
177.646659841956));
#26857=CARTESIAN_POINT('Ctrl Pts',(-61.701506884383,-111.563713223648,178.821287620784));
#26858=CARTESIAN_POINT('Ctrl Pts',(-60.5235593972605,-111.595009066961,
179.995915399612));
#26859=CARTESIAN_POINT('Ctrl Pts',(-58.8618066347693,-111.677881784879,
179.995915330104));
#26860=CARTESIAN_POINT('Ctrl Pts',(-57.2000538722782,-111.760754502798,
179.995915260595));
#26861=CARTESIAN_POINT('Ctrl Pts',(-56.0221064829017,-111.79205033569,178.821287383467));
#26862=CARTESIAN_POINT('Ctrl Pts',(-54.8441590935253,-111.823346168582,
177.646659506339));
#26863=CARTESIAN_POINT('Ctrl Pts',(-54.8342210997252,-111.730124396559,
175.985484901271));
#26864=CARTESIAN_POINT('Ctrl Pts',(-54.8242831059251,-111.636902624535,
174.324310296203));
#26865=CARTESIAN_POINT('Ctrl Pts',(-55.9823544672136,-111.419163251912,
173.149682517375));
#26866=CARTESIAN_POINT('Ctrl Pts',(-57.1404258285021,-111.201423879289,
171.975054738546));
#26867=CARTESIAN_POINT('Ctrl Pts',(-58.7823024651592,-110.932107632059,
171.975054808055));
#26868=CARTESIAN_POINT('Ctrl Pts',(-60.4241791018163,-110.66279138483,171.975054877564));
#26869=CARTESIAN_POINT('Ctrl Pts',(-61.5822503653587,-110.445052022627,
173.149682754692));
#26870=CARTESIAN_POINT('Ctrl Pts',(-62.7403216289012,-110.227312660424,
174.32431063182));
#26871=CARTESIAN_POINT('Ctrl Pts',(-62.7303834968672,-110.134090903137,
175.985485236888));
#26872=CARTESIAN_POINT('Ctrl Pts',(-62.7204453648333,-110.04086914585,177.646659841956));
#26873=CARTESIAN_POINT('Ctrl Pts',(-61.5424978777108,-110.072164989163,
178.821287620784));
#26874=CARTESIAN_POINT('Ctrl Pts',(-60.3645503905882,-110.103460832475,
179.995915399612));
#26875=CARTESIAN_POINT('Ctrl Pts',(-58.7027976280971,-110.186333550394,
179.995915330104));
#26876=CARTESIAN_POINT('Ctrl Pts',(-57.041044865606,-110.269206268313,179.995915260595));
#26877=CARTESIAN_POINT('Ctrl Pts',(-55.8630974762295,-110.300502101205,
178.821287383467));
#26878=CARTESIAN_POINT('Ctrl Pts',(-54.6851500868531,-110.331797934097,
177.646659506339));
#26879=CARTESIAN_POINT('Ctrl Pts',(-54.675212093053,-110.238576162073,175.985484901271));
#26880=CARTESIAN_POINT('Ctrl Pts',(-54.6652740992529,-110.145354390049,
174.324310296203));
#26881=CARTESIAN_POINT('Ctrl Pts',(-55.8233454605414,-109.927615017426,
173.149682517375));
#26882=CARTESIAN_POINT('Ctrl Pts',(-56.9814168218299,-109.709875644803,
171.975054738546));
#26883=CARTESIAN_POINT('Ctrl Pts',(-58.623293458487,-109.440559397574,171.975054808055));
#26884=CARTESIAN_POINT('Ctrl Pts',(-60.2651700951441,-109.171243150344,
171.975054877564));
#26885=CARTESIAN_POINT('Ctrl Pts',(-61.4232413586865,-108.953503788142,
173.149682754692));
#26886=CARTESIAN_POINT('Ctrl Pts',(-62.581312622229,-108.735764425939,174.32431063182));
#26887=CARTESIAN_POINT('Ctrl Pts',(-62.571374490195,-108.642542668652,175.985485236888));
#26888=CARTESIAN_POINT('Ctrl Pts',(-62.5614363581611,-108.549320911365,
177.646659841956));
#26889=CARTESIAN_POINT('Ctrl Pts',(-61.3834888710385,-108.580616754677,
178.821287620784));
#26890=CARTESIAN_POINT('Ctrl Pts',(-60.205541383916,-108.61191259799,179.995915399612));
#26891=CARTESIAN_POINT('Ctrl Pts',(-58.5437886214249,-108.694785315908,
179.995915330104));
#26892=CARTESIAN_POINT('Ctrl Pts',(-56.8820358589338,-108.777658033827,
179.995915260595));
#26893=CARTESIAN_POINT('Ctrl Pts',(-55.7040884695573,-108.808953866719,
178.821287383467));
#26894=CARTESIAN_POINT('Ctrl Pts',(-54.5261410801808,-108.840249699611,
177.646659506339));
#26895=CARTESIAN_POINT('Ctrl Pts',(-54.5162030863807,-108.747027927587,
175.985484901271));
#26896=CARTESIAN_POINT('Ctrl Pts',(-54.5062650925806,-108.653806155564,
174.324310296203));
#26897=CARTESIAN_POINT('Ctrl Pts',(-55.6643364538691,-108.436066782941,
173.149682517375));
#26898=CARTESIAN_POINT('Ctrl Pts',(-56.8224078151577,-108.218327410317,
171.975054738546));
#26899=CARTESIAN_POINT('Ctrl Pts',(-58.4642844518147,-107.949011163088,
171.975054808055));
#26900=CARTESIAN_POINT('Ctrl Pts',(-60.1061610884719,-107.679694915859,
171.975054877564));
#26901=CARTESIAN_POINT('Ctrl Pts',(-61.2642323520143,-107.461955553656,
173.149682754692));
#26902=CARTESIAN_POINT('Ctrl Pts',(-62.4223036155567,-107.244216191453,
174.32431063182));
#26903=CARTESIAN_POINT('Ctrl Pts',(-62.4123654835228,-107.150994434166,
175.985485236888));
#26904=CARTESIAN_POINT('Ctrl Pts',(-62.4024273514889,-107.057772676879,
177.646659841956));
#26905=CARTESIAN_POINT('Ctrl Pts',(-61.2244798643663,-107.089068520192,
178.821287620784));
#26906=CARTESIAN_POINT('Ctrl Pts',(-60.0465323772438,-107.120364363504,
179.995915399612));
#26907=CARTESIAN_POINT('Ctrl Pts',(-58.3847796147526,-107.203237081423,
179.995915330104));
#26908=CARTESIAN_POINT('Ctrl Pts',(-56.7230268522615,-107.286109799341,
179.995915260595));
#26909=CARTESIAN_POINT('Ctrl Pts',(-55.5450794628851,-107.317405632233,
178.821287383467));
#26910=CARTESIAN_POINT('Ctrl Pts',(-54.3671320735086,-107.348701465125,
177.646659506339));
#26911=CARTESIAN_POINT('Ctrl Pts',(-54.3571940797085,-107.255479693102,
175.985484901271));
#26912=CARTESIAN_POINT('Ctrl Pts',(-54.3472560859084,-107.162257921078,
174.324310296203));
#26913=CARTESIAN_POINT('Ctrl Pts',(-55.5053274471969,-106.944518548455,
173.149682517375));
#26914=CARTESIAN_POINT('Ctrl Pts',(-56.6633988084854,-106.726779175832,
171.975054738546));
#26915=CARTESIAN_POINT('Ctrl Pts',(-58.3052754451425,-106.457462928602,
171.975054808055));
#26916=CARTESIAN_POINT('Ctrl Pts',(-59.9471520817997,-106.188146681373,
171.975054877564));
#26917=CARTESIAN_POINT('Ctrl Pts',(-61.1052233453421,-105.97040731917,173.149682754692));
#26918=CARTESIAN_POINT('Ctrl Pts',(-62.2632946088845,-105.752667956968,
174.32431063182));
#26919=CARTESIAN_POINT('Ctrl Pts',(-62.2533564768505,-105.659446199681,
175.985485236888));
#26920=CARTESIAN_POINT('Ctrl Pts',(-62.2434183448166,-105.566224442394,
177.646659841956));
#26921=CARTESIAN_POINT('Ctrl Pts',(-61.0654708576941,-105.597520285706,
178.821287620784));
#26922=CARTESIAN_POINT('Ctrl Pts',(-59.8875233705716,-105.628816129018,
179.995915399612));
#26923=CARTESIAN_POINT('Ctrl Pts',(-58.2257706080804,-105.711688846937,
179.995915330104));
#26924=CARTESIAN_POINT('Ctrl Pts',(-56.5640178455893,-105.794561564856,
179.995915260595));
#26925=CARTESIAN_POINT('Ctrl Pts',(-55.3860704562128,-105.825857397748,
178.821287383467));
#26926=CARTESIAN_POINT('Ctrl Pts',(-54.2081230668364,-105.85715323064,177.646659506339));
#26927=CARTESIAN_POINT('Ctrl Pts',(-54.1981850730363,-105.763931458616,
175.985484901271));
#26928=CARTESIAN_POINT('Ctrl Pts',(-54.1882470792362,-105.670709686593,
174.324310296203));
#26929=CARTESIAN_POINT('Ctrl Pts',(-55.3463184405247,-105.452970313969,
173.149682517375));
#26930=CARTESIAN_POINT('Ctrl Pts',(-56.5043898018132,-105.235230941346,
171.975054738546));
#26931=CARTESIAN_POINT('Ctrl Pts',(-58.1462664384703,-104.965914694117,
171.975054808055));
#26932=CARTESIAN_POINT('Ctrl Pts',(-59.7881430751274,-104.696598446888,
171.975054877564));
#26933=CARTESIAN_POINT('Ctrl Pts',(-60.9462143386698,-104.478859084685,
173.149682754692));
#26934=CARTESIAN_POINT('Ctrl Pts',(-62.1042856022123,-104.261119722482,
174.32431063182));
#26935=CARTESIAN_POINT('Ctrl Pts',(-62.0943474701783,-104.167897965195,
175.985485236888));
#26936=CARTESIAN_POINT('Ctrl Pts',(-62.0844093381444,-104.074676207908,
177.646659841956));
#26937=CARTESIAN_POINT('Ctrl Pts',(-60.9064618510219,-104.10597205122,178.821287620784));
#26938=CARTESIAN_POINT('Ctrl Pts',(-59.7285143638993,-104.137267894533,
179.995915399612));
#26939=CARTESIAN_POINT('Ctrl Pts',(-58.0667616014082,-104.220140612451,
179.995915330104));
#26940=CARTESIAN_POINT('Ctrl Pts',(-56.4050088389171,-104.30301333037,179.995915260595));
#26941=CARTESIAN_POINT('Ctrl Pts',(-55.2270614495406,-104.334309163262,
178.821287383467));
#26942=CARTESIAN_POINT('Ctrl Pts',(-54.0491140601642,-104.365604996154,
177.646659506339));
#26943=CARTESIAN_POINT('Ctrl Pts',(-54.039176066364,-104.272383224131,175.985484901271));
#26944=CARTESIAN_POINT('Ctrl Pts',(-54.029238072564,-104.179161452107,174.324310296203));
#26945=CARTESIAN_POINT('Ctrl Pts',(-55.1873094338524,-103.961422079484,
173.149682517375));
#26946=CARTESIAN_POINT('Ctrl Pts',(-56.345380795141,-103.743682706861,171.975054738546));
#26947=CARTESIAN_POINT('Ctrl Pts',(-57.9872574317981,-103.474366459631,
171.975054808055));
#26948=CARTESIAN_POINT('Ctrl Pts',(-59.6291340684552,-103.205050212402,
171.975054877564));
#26949=CARTESIAN_POINT('Ctrl Pts',(-60.7872053319976,-102.987310850199,
173.149682754692));
#26950=CARTESIAN_POINT('Ctrl Pts',(-61.94527659554,-102.769571487996,174.32431063182));
#26951=CARTESIAN_POINT('Ctrl Pts',(-61.9353384635061,-102.676349730709,
175.985485236888));
#26952=CARTESIAN_POINT('Ctrl Pts',(-61.9254003314722,-102.583127973422,
177.646659841956));
#26953=CARTESIAN_POINT('Ctrl Pts',(-60.7474528443496,-102.614423816735,
178.821287620784));
#26954=CARTESIAN_POINT('Ctrl Pts',(-59.5695053572271,-102.645719660047,
179.995915399612));
#26955=CARTESIAN_POINT('Ctrl Pts',(-57.907752594736,-102.728592377966,179.995915330104));
#26956=CARTESIAN_POINT('Ctrl Pts',(-56.2459998322448,-102.811465095885,
179.995915260595));
#26957=CARTESIAN_POINT('Ctrl Pts',(-55.0680524428684,-102.842760928777,
178.821287383467));
#26958=CARTESIAN_POINT('Ctrl Pts',(-53.8901050534919,-102.874056761669,
177.646659506339));
#26959=CARTESIAN_POINT('Ctrl Pts',(-53.8801670596918,-102.780834989645,
175.985484901271));
#26960=CARTESIAN_POINT('Ctrl Pts',(-53.8702290658917,-102.687613217621,
174.324310296203));
#26961=CARTESIAN_POINT('Ctrl Pts',(-55.0283004271802,-102.469873844998,
173.149682517375));
#26962=CARTESIAN_POINT('Ctrl Pts',(-56.1863717884687,-102.252134472375,
171.975054738546));
#26963=CARTESIAN_POINT('Ctrl Pts',(-57.8282484251258,-101.982818225146,
171.975054808055));
#26964=CARTESIAN_POINT('Ctrl Pts',(-59.470125061783,-101.713501977916,171.975054877564));
#26965=CARTESIAN_POINT('Ctrl Pts',(-60.6281963253254,-101.495762615714,
173.149682754692));
#26966=CARTESIAN_POINT('Ctrl Pts',(-61.7862675888678,-101.278023253511,
174.32431063182));
#26967=CARTESIAN_POINT('Ctrl Pts',(-61.7763294568339,-101.184801496224,
175.985485236888));
#26968=CARTESIAN_POINT('Ctrl Pts',(-61.7663913247999,-101.091579738937,
177.646659841956));
#26969=CARTESIAN_POINT('Ctrl Pts',(-60.5884438376774,-101.122875582249,
178.821287620784));
#26970=CARTESIAN_POINT('Ctrl Pts',(-59.4104963505549,-101.154171425562,
179.995915399612));
#26971=CARTESIAN_POINT('Ctrl Pts',(-57.7487435880637,-101.23704414348,179.995915330104));
#26972=CARTESIAN_POINT('Ctrl Pts',(-56.0869908255726,-101.319916861399,
179.995915260595));
#26973=CARTESIAN_POINT('Ctrl Pts',(-54.9090434361961,-101.351212694291,
178.821287383467));
#26974=CARTESIAN_POINT('Ctrl Pts',(-53.7310960468197,-101.382508527183,
177.646659506339));
#26975=CARTESIAN_POINT('Ctrl Pts',(-53.7211580530196,-101.289286755159,
175.985484901271));
#26976=CARTESIAN_POINT('Ctrl Pts',(-53.7112200592195,-101.196064983136,
174.324310296203));
#26977=CARTESIAN_POINT('Ctrl Pts',(-54.869291420508,-100.978325610513,173.149682517375));
#26978=CARTESIAN_POINT('Ctrl Pts',(-56.0273627817965,-100.760586237889,
171.975054738546));
#26979=CARTESIAN_POINT('Ctrl Pts',(-57.6692394184536,-100.49126999066,171.975054808055));
#26980=CARTESIAN_POINT('Ctrl Pts',(-59.3111160551107,-100.221953743431,
171.975054877564));
#26981=CARTESIAN_POINT('Ctrl Pts',(-60.4691873186531,-100.004214381228,
173.149682754692));
#26982=CARTESIAN_POINT('Ctrl Pts',(-61.6272585821956,-99.7864750190253,
174.32431063182));
#26983=CARTESIAN_POINT('Ctrl Pts',(-61.6173204501616,-99.6932532617382,
175.985485236888));
#26984=CARTESIAN_POINT('Ctrl Pts',(-61.6073823181277,-99.6000315044512,
177.646659841956));
#26985=CARTESIAN_POINT('Ctrl Pts',(-60.4294348310052,-99.6313273477637,
178.821287620784));
#26986=CARTESIAN_POINT('Ctrl Pts',(-59.2514873438827,-99.6626231910761,
179.995915399612));
#26987=CARTESIAN_POINT('Ctrl Pts',(-57.5897345813915,-99.7454959089947,
179.995915330104));
#26988=CARTESIAN_POINT('Ctrl Pts',(-55.9279818189004,-99.8283686269133,
179.995915260595));
#26989=CARTESIAN_POINT('Ctrl Pts',(-54.7500344295239,-99.8596644598054,
178.821287383467));
#26990=CARTESIAN_POINT('Ctrl Pts',(-53.5720870401475,-99.8909602926975,
177.646659506339));
#26991=CARTESIAN_POINT('Ctrl Pts',(-53.5621490463474,-99.7977385206737,
175.985484901271));
#26992=CARTESIAN_POINT('Ctrl Pts',(-53.5522110525473,-99.7045167486501,
174.324310296203));
#26993=CARTESIAN_POINT('Ctrl Pts',(-54.7102824138358,-99.4867773760269,
173.149682517375));
#26994=CARTESIAN_POINT('Ctrl Pts',(-55.8683537751243,-99.2690380034038,
171.975054738546));
#26995=CARTESIAN_POINT('Ctrl Pts',(-57.5102304117814,-98.9997217561745,
171.975054808055));
#26996=CARTESIAN_POINT('Ctrl Pts',(-59.1521070484385,-98.7304055089452,
171.975054877564));
#26997=CARTESIAN_POINT('Ctrl Pts',(-60.3101783119809,-98.5126661467424,
173.149682754692));
#26998=CARTESIAN_POINT('Ctrl Pts',(-61.4682495755234,-98.2949267845397,
174.32431063182));
#26999=CARTESIAN_POINT('Ctrl Pts',(-61.4583114434894,-98.2017050272526,
175.985485236888));
#27000=CARTESIAN_POINT('Ctrl Pts',(-61.4483733114555,-98.1084832699656,
177.646659841956));
#27001=CARTESIAN_POINT('Ctrl Pts',(-60.2704258243329,-98.139779113278,178.821287620784));
#27002=CARTESIAN_POINT('Ctrl Pts',(-59.0924783372104,-98.1710749565905,
179.995915399612));
#27003=CARTESIAN_POINT('Ctrl Pts',(-57.4307255747193,-98.2539476745091,
179.995915330104));
#27004=CARTESIAN_POINT('Ctrl Pts',(-55.7689728122282,-98.3368203924277,
179.995915260595));
#27005=CARTESIAN_POINT('Ctrl Pts',(-54.5910254228517,-98.3681162253198,
178.821287383467));
#27006=CARTESIAN_POINT('Ctrl Pts',(-56.1988062143188,-113.449542435949,
178.821287383467));
#27007=CARTESIAN_POINT('Ctrl Pts',(-55.0208588249424,-113.480838268841,
177.646659506339));
#27008=CARTESIAN_POINT('Ctrl Pts',(-55.0109208311422,-113.387616496817,
175.985484901271));
#27009=CARTESIAN_POINT('Ctrl Pts',(-55.0009828373422,-113.294394724794,
174.324310296203));
#27010=CARTESIAN_POINT('Ctrl Pts',(-56.1590541986307,-113.07665535217,173.149682517375));
#27011=CARTESIAN_POINT('Ctrl Pts',(-57.3171255599192,-112.858915979547,
171.975054738546));
#27012=CARTESIAN_POINT('Ctrl Pts',(-58.9590021965763,-112.589599732318,
171.975054808055));
#27013=CARTESIAN_POINT('Ctrl Pts',(-60.6008788332334,-112.320283485089,
171.975054877564));
#27014=CARTESIAN_POINT('Ctrl Pts',(-61.7589500967758,-112.102544122886,
173.149682754692));
#27015=CARTESIAN_POINT('Ctrl Pts',(-62.9170213603182,-111.884804760683,
174.32431063182));
#27016=CARTESIAN_POINT('Ctrl Pts',(-62.9070832282843,-111.791583003396,
175.985485236888));
#27017=CARTESIAN_POINT('Ctrl Pts',(-62.8971450962504,-111.698361246109,
177.646659841956));
#27018=CARTESIAN_POINT('Ctrl Pts',(-61.7191976091278,-111.729657089422,
178.821287620784));
#27019=CARTESIAN_POINT('Ctrl Pts',(-60.5412501220053,-111.760952932734,
179.995915399612));
#27020=CARTESIAN_POINT('Ctrl Pts',(-58.8794973595142,-111.843825650653,
179.995915330104));
#27021=CARTESIAN_POINT('Ctrl Pts',(-57.217744597023,-111.926698368571,179.995915260595));
#27022=CARTESIAN_POINT('Ctrl Pts',(-56.0397972076466,-111.957994201463,
178.821287383467));
#27023=CARTESIAN_POINT('Ctrl Pts',(-54.8618498182701,-111.989290034355,
177.646659506339));
#27024=CARTESIAN_POINT('Ctrl Pts',(-54.85191182447,-111.896068262332,175.985484901271));
#27025=CARTESIAN_POINT('Ctrl Pts',(-54.8419738306699,-111.802846490308,
174.324310296203));
#27026=CARTESIAN_POINT('Ctrl Pts',(-56.0000451919584,-111.585107117685,
173.149682517375));
#27027=CARTESIAN_POINT('Ctrl Pts',(-57.158116553247,-111.367367745062,171.975054738546));
#27028=CARTESIAN_POINT('Ctrl Pts',(-58.799993189904,-111.098051497832,171.975054808055));
#27029=CARTESIAN_POINT('Ctrl Pts',(-60.4418698265612,-110.828735250603,
171.975054877564));
#27030=CARTESIAN_POINT('Ctrl Pts',(-61.5999410901036,-110.6109958884,173.149682754692));
#27031=CARTESIAN_POINT('Ctrl Pts',(-62.758012353646,-110.393256526198,174.32431063182));
#27032=CARTESIAN_POINT('Ctrl Pts',(-62.7480742216121,-110.30003476891,175.985485236888));
#27033=CARTESIAN_POINT('Ctrl Pts',(-62.7381360895782,-110.206813011623,
177.646659841956));
#27034=CARTESIAN_POINT('Ctrl Pts',(-61.5601886024556,-110.238108854936,
178.821287620784));
#27035=CARTESIAN_POINT('Ctrl Pts',(-60.3822411153331,-110.269404698248,
179.995915399612));
#27036=CARTESIAN_POINT('Ctrl Pts',(-58.7204883528419,-110.352277416167,
179.995915330104));
#27037=CARTESIAN_POINT('Ctrl Pts',(-57.0587355903508,-110.435150134086,
179.995915260595));
#27038=CARTESIAN_POINT('Ctrl Pts',(-55.8807882009743,-110.466445966978,
178.821287383467));
#27039=CARTESIAN_POINT('Ctrl Pts',(-54.7028408115979,-110.49774179987,177.646659506339));
#27040=CARTESIAN_POINT('Ctrl Pts',(-54.6929028177978,-110.404520027846,
175.985484901271));
#27041=CARTESIAN_POINT('Ctrl Pts',(-54.6829648239977,-110.311298255822,
174.324310296203));
#27042=CARTESIAN_POINT('Ctrl Pts',(-55.8410361852862,-110.093558883199,
173.149682517375));
#27043=CARTESIAN_POINT('Ctrl Pts',(-56.9991075465747,-109.875819510576,
171.975054738546));
#27044=CARTESIAN_POINT('Ctrl Pts',(-58.6409841832318,-109.606503263347,
171.975054808055));
#27045=CARTESIAN_POINT('Ctrl Pts',(-60.2828608198889,-109.337187016117,
171.975054877564));
#27046=CARTESIAN_POINT('Ctrl Pts',(-61.4409320834313,-109.119447653915,
173.149682754692));
#27047=CARTESIAN_POINT('Ctrl Pts',(-62.5990033469738,-108.901708291712,
174.32431063182));
#27048=CARTESIAN_POINT('Ctrl Pts',(-62.5890652149398,-108.808486534425,
175.985485236888));
#27049=CARTESIAN_POINT('Ctrl Pts',(-62.5791270829059,-108.715264777138,
177.646659841956));
#27050=CARTESIAN_POINT('Ctrl Pts',(-61.4011795957834,-108.74656062045,178.821287620784));
#27051=CARTESIAN_POINT('Ctrl Pts',(-60.2232321086609,-108.777856463763,
179.995915399612));
#27052=CARTESIAN_POINT('Ctrl Pts',(-58.5614793461697,-108.860729181681,
179.995915330104));
#27053=CARTESIAN_POINT('Ctrl Pts',(-56.8997265836786,-108.9436018996,179.995915260595));
#27054=CARTESIAN_POINT('Ctrl Pts',(-55.7217791943021,-108.974897732492,
178.821287383467));
#27055=CARTESIAN_POINT('Ctrl Pts',(-54.5438318049257,-109.006193565384,
177.646659506339));
#27056=CARTESIAN_POINT('Ctrl Pts',(-54.5338938111256,-108.91297179336,175.985484901271));
#27057=CARTESIAN_POINT('Ctrl Pts',(-54.5239558173255,-108.819750021337,
174.324310296203));
#27058=CARTESIAN_POINT('Ctrl Pts',(-55.682027178614,-108.602010648714,173.149682517375));
#27059=CARTESIAN_POINT('Ctrl Pts',(-56.8400985399025,-108.384271276091,
171.975054738546));
#27060=CARTESIAN_POINT('Ctrl Pts',(-58.4819751765596,-108.114955028861,
171.975054808055));
#27061=CARTESIAN_POINT('Ctrl Pts',(-60.1238518132167,-107.845638781632,
171.975054877564));
#27062=CARTESIAN_POINT('Ctrl Pts',(-61.2819230767591,-107.627899419429,
173.149682754692));
#27063=CARTESIAN_POINT('Ctrl Pts',(-62.4399943403016,-107.410160057226,
174.32431063182));
#27064=CARTESIAN_POINT('Ctrl Pts',(-62.4300562082676,-107.316938299939,
175.985485236888));
#27065=CARTESIAN_POINT('Ctrl Pts',(-62.4201180762337,-107.223716542652,
177.646659841956));
#27066=CARTESIAN_POINT('Ctrl Pts',(-61.2421705891111,-107.255012385965,
178.821287620784));
#27067=CARTESIAN_POINT('Ctrl Pts',(-60.0642231019886,-107.286308229277,
179.995915399612));
#27068=CARTESIAN_POINT('Ctrl Pts',(-58.4024703394975,-107.369180947196,
179.995915330104));
#27069=CARTESIAN_POINT('Ctrl Pts',(-56.7407175770064,-107.452053665114,
179.995915260595));
#27070=CARTESIAN_POINT('Ctrl Pts',(-55.5627701876299,-107.483349498006,
178.821287383467));
#27071=CARTESIAN_POINT('Ctrl Pts',(-54.3848227982534,-107.514645330899,
177.646659506339));
#27072=CARTESIAN_POINT('Ctrl Pts',(-54.3748848044533,-107.421423558875,
175.985484901271));
#27073=CARTESIAN_POINT('Ctrl Pts',(-54.3649468106533,-107.328201786851,
174.324310296203));
#27074=CARTESIAN_POINT('Ctrl Pts',(-55.5230181719417,-107.110462414228,
173.149682517375));
#27075=CARTESIAN_POINT('Ctrl Pts',(-56.6810895332303,-106.892723041605,
171.975054738546));
#27076=CARTESIAN_POINT('Ctrl Pts',(-58.3229661698874,-106.623406794376,
171.975054808055));
#27077=CARTESIAN_POINT('Ctrl Pts',(-59.9648428065445,-106.354090547146,
171.975054877564));
#27078=CARTESIAN_POINT('Ctrl Pts',(-61.1229140700869,-106.136351184943,
173.149682754692));
#27079=CARTESIAN_POINT('Ctrl Pts',(-62.2809853336293,-105.918611822741,
174.32431063182));
#27080=CARTESIAN_POINT('Ctrl Pts',(-62.2710472015954,-105.825390065454,
175.985485236888));
#27081=CARTESIAN_POINT('Ctrl Pts',(-62.2611090695615,-105.732168308167,
177.646659841956));
#27082=CARTESIAN_POINT('Ctrl Pts',(-61.0831615824389,-105.763464151479,
178.821287620784));
#27083=CARTESIAN_POINT('Ctrl Pts',(-59.9052140953164,-105.794759994792,
179.995915399612));
#27084=CARTESIAN_POINT('Ctrl Pts',(-58.2434613328252,-105.87763271271,179.995915330104));
#27085=CARTESIAN_POINT('Ctrl Pts',(-56.5817085703341,-105.960505430629,
179.995915260595));
#27086=CARTESIAN_POINT('Ctrl Pts',(-55.4037611809577,-105.991801263521,
178.821287383467));
#27087=CARTESIAN_POINT('Ctrl Pts',(-54.2258137915812,-106.023097096413,
177.646659506339));
#27088=CARTESIAN_POINT('Ctrl Pts',(-54.2158757977811,-105.929875324389,
175.985484901271));
#27089=CARTESIAN_POINT('Ctrl Pts',(-54.205937803981,-105.836653552366,174.324310296203));
#27090=CARTESIAN_POINT('Ctrl Pts',(-55.3640091652695,-105.618914179742,
173.149682517375));
#27091=CARTESIAN_POINT('Ctrl Pts',(-56.522080526558,-105.401174807119,171.975054738546));
#27092=CARTESIAN_POINT('Ctrl Pts',(-58.1639571632151,-105.13185855989,171.975054808055));
#27093=CARTESIAN_POINT('Ctrl Pts',(-59.8058337998722,-104.862542312661,
171.975054877564));
#27094=CARTESIAN_POINT('Ctrl Pts',(-60.9639050634147,-104.644802950458,
173.149682754692));
#27095=CARTESIAN_POINT('Ctrl Pts',(-62.1219763269571,-104.427063588255,
174.32431063182));
#27096=CARTESIAN_POINT('Ctrl Pts',(-62.1120381949232,-104.333841830968,
175.985485236888));
#27097=CARTESIAN_POINT('Ctrl Pts',(-62.1021000628892,-104.240620073681,
177.646659841956));
#27098=CARTESIAN_POINT('Ctrl Pts',(-60.9241525757667,-104.271915916993,
178.821287620784));
#27099=CARTESIAN_POINT('Ctrl Pts',(-59.7462050886442,-104.303211760306,
179.995915399612));
#27100=CARTESIAN_POINT('Ctrl Pts',(-58.084452326153,-104.386084478225,179.995915330104));
#27101=CARTESIAN_POINT('Ctrl Pts',(-56.4226995636619,-104.468957196143,
179.995915260595));
#27102=CARTESIAN_POINT('Ctrl Pts',(-55.2447521742854,-104.500253029035,
178.821287383467));
#27103=CARTESIAN_POINT('Ctrl Pts',(-54.066804784909,-104.531548861927,177.646659506339));
#27104=CARTESIAN_POINT('Ctrl Pts',(-54.0568667911089,-104.438327089904,
175.985484901271));
#27105=CARTESIAN_POINT('Ctrl Pts',(-54.0469287973088,-104.34510531788,174.324310296203));
#27106=CARTESIAN_POINT('Ctrl Pts',(-55.2050001585973,-104.127365945257,
173.149682517375));
#27107=CARTESIAN_POINT('Ctrl Pts',(-56.3630715198858,-103.909626572634,
171.975054738546));
#27108=CARTESIAN_POINT('Ctrl Pts',(-58.0049481565429,-103.640310325404,
171.975054808055));
#27109=CARTESIAN_POINT('Ctrl Pts',(-59.6468247932,-103.370994078175,171.975054877564));
#27110=CARTESIAN_POINT('Ctrl Pts',(-60.8048960567424,-103.153254715972,
173.149682754692));
#27111=CARTESIAN_POINT('Ctrl Pts',(-61.9629673202849,-102.93551535377,174.32431063182));
#27112=CARTESIAN_POINT('Ctrl Pts',(-61.9530291882509,-102.842293596483,
175.985485236888));
#27113=CARTESIAN_POINT('Ctrl Pts',(-61.943091056217,-102.749071839196,177.646659841956));
#27114=CARTESIAN_POINT('Ctrl Pts',(-60.7651435690945,-102.780367682508,
178.821287620784));
#27115=CARTESIAN_POINT('Ctrl Pts',(-59.587196081972,-102.81166352582,179.995915399612));
#27116=CARTESIAN_POINT('Ctrl Pts',(-57.9254433194808,-102.894536243739,
179.995915330104));
#27117=CARTESIAN_POINT('Ctrl Pts',(-56.2636905569897,-102.977408961658,
179.995915260595));
#27118=CARTESIAN_POINT('Ctrl Pts',(-55.0857431676132,-103.00870479455,178.821287383467));
#27119=CARTESIAN_POINT('Ctrl Pts',(-53.9077957782368,-103.040000627442,
177.646659506339));
#27120=CARTESIAN_POINT('Ctrl Pts',(-53.8978577844367,-102.946778855418,
175.985484901271));
#27121=CARTESIAN_POINT('Ctrl Pts',(-53.8879197906366,-102.853557083394,
174.324310296203));
#27122=CARTESIAN_POINT('Ctrl Pts',(-55.0459911519251,-102.635817710771,
173.149682517375));
#27123=CARTESIAN_POINT('Ctrl Pts',(-56.2040625132136,-102.418078338148,
171.975054738546));
#27124=CARTESIAN_POINT('Ctrl Pts',(-57.8459391498707,-102.148762090919,
171.975054808055));
#27125=CARTESIAN_POINT('Ctrl Pts',(-59.4878157865278,-101.879445843689,
171.975054877564));
#27126=CARTESIAN_POINT('Ctrl Pts',(-60.6458870500702,-101.661706481487,
173.149682754692));
#27127=CARTESIAN_POINT('Ctrl Pts',(-61.8039583136126,-101.443967119284,
174.32431063182));
#27128=CARTESIAN_POINT('Ctrl Pts',(-61.7940201815787,-101.350745361997,
175.985485236888));
#27129=CARTESIAN_POINT('Ctrl Pts',(-61.7840820495448,-101.25752360471,177.646659841956));
#27130=CARTESIAN_POINT('Ctrl Pts',(-60.6061345624222,-101.288819448022,
178.821287620784));
#27131=CARTESIAN_POINT('Ctrl Pts',(-59.4281870752997,-101.320115291335,
179.995915399612));
#27132=CARTESIAN_POINT('Ctrl Pts',(-57.7664343128086,-101.402988009253,
179.995915330104));
#27133=CARTESIAN_POINT('Ctrl Pts',(-56.1046815503175,-101.485860727172,
179.995915260595));
#27134=CARTESIAN_POINT('Ctrl Pts',(-54.926734160941,-101.517156560064,178.821287383467));
#27135=CARTESIAN_POINT('Ctrl Pts',(-53.7487867715645,-101.548452392956,
177.646659506339));
#27136=CARTESIAN_POINT('Ctrl Pts',(-53.7388487777644,-101.455230620932,
175.985484901271));
#27137=CARTESIAN_POINT('Ctrl Pts',(-53.7289107839643,-101.362008848909,
174.324310296203));
#27138=CARTESIAN_POINT('Ctrl Pts',(-54.8869821452528,-101.144269476286,
173.149682517375));
#27139=CARTESIAN_POINT('Ctrl Pts',(-56.0450535065414,-100.926530103662,
171.975054738546));
#27140=CARTESIAN_POINT('Ctrl Pts',(-57.6869301431984,-100.657213856433,
171.975054808055));
#27141=CARTESIAN_POINT('Ctrl Pts',(-59.3288067798556,-100.387897609204,
171.975054877564));
#27142=CARTESIAN_POINT('Ctrl Pts',(-60.486878043398,-100.170158247001,173.149682754692));
#27143=CARTESIAN_POINT('Ctrl Pts',(-61.6449493069404,-99.9524188847983,
174.32431063182));
#27144=CARTESIAN_POINT('Ctrl Pts',(-61.6350111749065,-99.8591971275113,
175.985485236888));
#27145=CARTESIAN_POINT('Ctrl Pts',(-61.6250730428726,-99.7659753702243,
177.646659841956));
#27146=CARTESIAN_POINT('Ctrl Pts',(-60.44712555575,-99.7972712135367,178.821287620784));
#27147=CARTESIAN_POINT('Ctrl Pts',(-59.2691780686275,-99.8285670568492,
179.995915399612));
#27148=CARTESIAN_POINT('Ctrl Pts',(-57.6074253061363,-99.9114397747677,
179.995915330104));
#27149=CARTESIAN_POINT('Ctrl Pts',(-55.9456725436452,-99.9943124926864,
179.995915260595));
#27150=CARTESIAN_POINT('Ctrl Pts',(-54.7677251542687,-100.025608325578,
178.821287383467));
#27151=CARTESIAN_POINT('Ctrl Pts',(-53.5897777648923,-100.05690415847,177.646659506339));
#27152=CARTESIAN_POINT('Ctrl Pts',(-53.5798397710922,-99.9636823864468,
175.985484901271));
#27153=CARTESIAN_POINT('Ctrl Pts',(-53.5699017772921,-99.8704606144232,
174.324310296203));
#27154=CARTESIAN_POINT('Ctrl Pts',(-54.7279731385806,-99.6527212418,173.149682517375));
#27155=CARTESIAN_POINT('Ctrl Pts',(-55.8860444998691,-99.4349818691769,
171.975054738546));
#27156=CARTESIAN_POINT('Ctrl Pts',(-57.5279211365262,-99.1656656219475,
171.975054808055));
#27157=CARTESIAN_POINT('Ctrl Pts',(-59.1697977731833,-98.8963493747183,
171.975054877564));
#27158=CARTESIAN_POINT('Ctrl Pts',(-60.3278690367257,-98.6786100125155,
173.149682754692));
#27159=CARTESIAN_POINT('Ctrl Pts',(-61.4859403002682,-98.4608706503128,
174.32431063182));
#27160=CARTESIAN_POINT('Ctrl Pts',(-61.4760021682342,-98.3676488930257,
175.985485236888));
#27161=CARTESIAN_POINT('Ctrl Pts',(-61.4660640362003,-98.2744271357387,
177.646659841956));
#27162=CARTESIAN_POINT('Ctrl Pts',(-60.2881165490778,-98.3057229790511,
178.821287620784));
#27163=CARTESIAN_POINT('Ctrl Pts',(-59.1101690619552,-98.3370188223636,
179.995915399612));
#27164=CARTESIAN_POINT('Ctrl Pts',(-57.4484162994641,-98.4198915402821,
179.995915330104));
#27165=CARTESIAN_POINT('Ctrl Pts',(-55.786663536973,-98.5027642582008,179.995915260595));
#27166=CARTESIAN_POINT('Ctrl Pts',(-54.6087161475965,-98.5340600910929,
178.821287383467));
#27167=CARTESIAN_POINT('Ctrl Pts',(-56.2237961054143,-113.614380048479,
178.813912075476));
#27168=CARTESIAN_POINT('Ctrl Pts',(-55.0488864554725,-113.645352038053,
177.6423391512));
#27169=CARTESIAN_POINT('Ctrl Pts',(-55.0389484614927,-113.552130266048,
175.985484901707));
#27170=CARTESIAN_POINT('Ctrl Pts',(-55.0290104675128,-113.458908494044,
174.328630652215));
#27171=CARTESIAN_POINT('Ctrl Pts',(-56.1840440891124,-113.241492964766,
173.157057825983));
#27172=CARTESIAN_POINT('Ctrl Pts',(-57.3390777107121,-113.024077435489,
171.985484999752));
#27173=CARTESIAN_POINT('Ctrl Pts',(-58.9766583348819,-112.755219171892,
171.985485069079));
#27174=CARTESIAN_POINT('Ctrl Pts',(-60.6142389590518,-112.486360908295,
171.985485138407));
#27175=CARTESIAN_POINT('Ctrl Pts',(-61.7692724831595,-112.268945389411,
173.157058062683));
#27176=CARTESIAN_POINT('Ctrl Pts',(-62.9243060072673,-112.051529870527,
174.328630986959));
#27177=CARTESIAN_POINT('Ctrl Pts',(-62.9143678754131,-111.95830811322,175.985485236451));
#27178=CARTESIAN_POINT('Ctrl Pts',(-62.9044297435589,-111.865086355914,
177.642339485944));
#27179=CARTESIAN_POINT('Ctrl Pts',(-61.7295199961253,-111.896058355881,
178.813912312176));
#27180=CARTESIAN_POINT('Ctrl Pts',(-60.5546102486917,-111.927030355848,
179.985485138407));
#27181=CARTESIAN_POINT('Ctrl Pts',(-58.8971534986878,-112.009445090134,
179.985485069079));
#27182=CARTESIAN_POINT('Ctrl Pts',(-57.2396967486839,-112.09185982442,179.985484999752));
#27183=CARTESIAN_POINT('Ctrl Pts',(-56.0647870987421,-112.122831813994,
178.813912075476));
#27184=CARTESIAN_POINT('Ctrl Pts',(-54.8898774488003,-112.153803803567,
177.6423391512));
#27185=CARTESIAN_POINT('Ctrl Pts',(-54.8799394548205,-112.060582031563,
175.985484901707));
#27186=CARTESIAN_POINT('Ctrl Pts',(-54.8700014608406,-111.967360259558,
174.328630652215));
#27187=CARTESIAN_POINT('Ctrl Pts',(-56.0250350824402,-111.749944730281,
173.157057825983));
#27188=CARTESIAN_POINT('Ctrl Pts',(-57.1800687040398,-111.532529201003,
171.985484999752));
#27189=CARTESIAN_POINT('Ctrl Pts',(-58.8176493282097,-111.263670937406,
171.985485069079));
#27190=CARTESIAN_POINT('Ctrl Pts',(-60.4552299523796,-110.994812673809,
171.985485138407));
#27191=CARTESIAN_POINT('Ctrl Pts',(-61.6102634764873,-110.777397154925,
173.157058062683));
#27192=CARTESIAN_POINT('Ctrl Pts',(-62.7652970005951,-110.559981636041,
174.328630986959));
#27193=CARTESIAN_POINT('Ctrl Pts',(-62.7553588687409,-110.466759878735,
175.985485236451));
#27194=CARTESIAN_POINT('Ctrl Pts',(-62.7454207368867,-110.373538121429,
177.642339485944));
#27195=CARTESIAN_POINT('Ctrl Pts',(-61.5705109894531,-110.404510121395,
178.813912312176));
#27196=CARTESIAN_POINT('Ctrl Pts',(-60.3956012420194,-110.435482121362,
179.985485138407));
#27197=CARTESIAN_POINT('Ctrl Pts',(-58.7381444920155,-110.517896855648,
179.985485069079));
#27198=CARTESIAN_POINT('Ctrl Pts',(-57.0806877420116,-110.600311589935,
179.985484999752));
#27199=CARTESIAN_POINT('Ctrl Pts',(-55.9057780920699,-110.631283579508,
178.813912075476));
#27200=CARTESIAN_POINT('Ctrl Pts',(-54.7308684421281,-110.662255569082,
177.6423391512));
#27201=CARTESIAN_POINT('Ctrl Pts',(-54.7209304481482,-110.569033797077,
175.985484901707));
#27202=CARTESIAN_POINT('Ctrl Pts',(-54.7109924541684,-110.475812025073,
174.328630652215));
#27203=CARTESIAN_POINT('Ctrl Pts',(-55.866026075768,-110.258396495795,173.157057825983));
#27204=CARTESIAN_POINT('Ctrl Pts',(-57.0210596973676,-110.040980966518,
171.985484999752));
#27205=CARTESIAN_POINT('Ctrl Pts',(-58.6586403215375,-109.772122702921,
171.985485069079));
#27206=CARTESIAN_POINT('Ctrl Pts',(-60.2962209457073,-109.503264439324,
171.985485138407));
#27207=CARTESIAN_POINT('Ctrl Pts',(-61.4512544698151,-109.28584892044,173.157058062683));
#27208=CARTESIAN_POINT('Ctrl Pts',(-62.6062879939228,-109.068433401555,
174.328630986959));
#27209=CARTESIAN_POINT('Ctrl Pts',(-62.5963498620687,-108.975211644249,
175.985485236451));
#27210=CARTESIAN_POINT('Ctrl Pts',(-62.5864117302145,-108.881989886943,
177.642339485944));
#27211=CARTESIAN_POINT('Ctrl Pts',(-61.4115019827808,-108.91296188691,178.813912312176));
#27212=CARTESIAN_POINT('Ctrl Pts',(-60.2365922353472,-108.943933886877,
179.985485138407));
#27213=CARTESIAN_POINT('Ctrl Pts',(-58.5791354853433,-109.026348621163,
179.985485069079));
#27214=CARTESIAN_POINT('Ctrl Pts',(-56.9216787353394,-109.108763355449,
179.985484999752));
#27215=CARTESIAN_POINT('Ctrl Pts',(-55.7467690853976,-109.139735345023,
178.813912075476));
#27216=CARTESIAN_POINT('Ctrl Pts',(-54.5718594354559,-109.170707334596,
177.6423391512));
#27217=CARTESIAN_POINT('Ctrl Pts',(-54.561921441476,-109.077485562592,175.985484901707));
#27218=CARTESIAN_POINT('Ctrl Pts',(-54.5519834474962,-108.984263790587,
174.328630652215));
#27219=CARTESIAN_POINT('Ctrl Pts',(-55.7070170690958,-108.76684826131,173.157057825983));
#27220=CARTESIAN_POINT('Ctrl Pts',(-56.8620506906954,-108.549432732032,
171.985484999752));
#27221=CARTESIAN_POINT('Ctrl Pts',(-58.4996313148652,-108.280574468435,
171.985485069079));
#27222=CARTESIAN_POINT('Ctrl Pts',(-60.1372119390351,-108.011716204838,
171.985485138407));
#27223=CARTESIAN_POINT('Ctrl Pts',(-61.2922454631428,-107.794300685954,
173.157058062683));
#27224=CARTESIAN_POINT('Ctrl Pts',(-62.4472789872506,-107.57688516707,174.328630986959));
#27225=CARTESIAN_POINT('Ctrl Pts',(-62.4373408553964,-107.483663409764,
175.985485236451));
#27226=CARTESIAN_POINT('Ctrl Pts',(-62.4274027235423,-107.390441652457,
177.642339485944));
#27227=CARTESIAN_POINT('Ctrl Pts',(-61.2524929761086,-107.421413652424,
178.813912312176));
#27228=CARTESIAN_POINT('Ctrl Pts',(-60.077583228675,-107.452385652391,179.985485138407));
#27229=CARTESIAN_POINT('Ctrl Pts',(-58.4201264786711,-107.534800386677,
179.985485069079));
#27230=CARTESIAN_POINT('Ctrl Pts',(-56.7626697286672,-107.617215120964,
179.985484999752));
#27231=CARTESIAN_POINT('Ctrl Pts',(-55.5877600787254,-107.648187110537,
178.813912075476));
#27232=CARTESIAN_POINT('Ctrl Pts',(-54.4128504287836,-107.67915910011,177.6423391512));
#27233=CARTESIAN_POINT('Ctrl Pts',(-54.4029124348038,-107.585937328106,
175.985484901707));
#27234=CARTESIAN_POINT('Ctrl Pts',(-54.3929744408239,-107.492715556102,
174.328630652215));
#27235=CARTESIAN_POINT('Ctrl Pts',(-55.5480080624235,-107.275300026824,
173.157057825983));
#27236=CARTESIAN_POINT('Ctrl Pts',(-56.7030416840231,-107.057884497547,
171.985484999752));
#27237=CARTESIAN_POINT('Ctrl Pts',(-58.340622308193,-106.78902623395,171.985485069079));
#27238=CARTESIAN_POINT('Ctrl Pts',(-59.9782029323629,-106.520167970353,
171.985485138407));
#27239=CARTESIAN_POINT('Ctrl Pts',(-61.1332364564706,-106.302752451468,
173.157058062683));
#27240=CARTESIAN_POINT('Ctrl Pts',(-62.2882699805784,-106.085336932584,
174.328630986959));
#27241=CARTESIAN_POINT('Ctrl Pts',(-62.2783318487242,-105.992115175278,
175.985485236451));
#27242=CARTESIAN_POINT('Ctrl Pts',(-62.26839371687,-105.898893417972,177.642339485944));
#27243=CARTESIAN_POINT('Ctrl Pts',(-61.0934839694364,-105.929865417939,
178.813912312176));
#27244=CARTESIAN_POINT('Ctrl Pts',(-59.9185742220028,-105.960837417905,
179.985485138407));
#27245=CARTESIAN_POINT('Ctrl Pts',(-58.2611174719989,-106.043252152192,
179.985485069079));
#27246=CARTESIAN_POINT('Ctrl Pts',(-56.603660721995,-106.125666886478,179.985484999752));
#27247=CARTESIAN_POINT('Ctrl Pts',(-55.4287510720532,-106.156638876051,
178.813912075476));
#27248=CARTESIAN_POINT('Ctrl Pts',(-54.2538414221114,-106.187610865625,
177.6423391512));
#27249=CARTESIAN_POINT('Ctrl Pts',(-54.2439034281315,-106.09438909362,175.985484901707));
#27250=CARTESIAN_POINT('Ctrl Pts',(-54.2339654341517,-106.001167321616,
174.328630652215));
#27251=CARTESIAN_POINT('Ctrl Pts',(-55.3889990557513,-105.783751792338,
173.157057825983));
#27252=CARTESIAN_POINT('Ctrl Pts',(-56.5440326773509,-105.566336263061,
171.985484999752));
#27253=CARTESIAN_POINT('Ctrl Pts',(-58.1816133015208,-105.297477999464,
171.985485069079));
#27254=CARTESIAN_POINT('Ctrl Pts',(-59.8191939256906,-105.028619735867,
171.985485138407));
#27255=CARTESIAN_POINT('Ctrl Pts',(-60.9742274497984,-104.811204216983,
173.157058062683));
#27256=CARTESIAN_POINT('Ctrl Pts',(-62.1292609739061,-104.593788698099,
174.328630986959));
#27257=CARTESIAN_POINT('Ctrl Pts',(-62.119322842052,-104.500566940792,175.985485236451));
#27258=CARTESIAN_POINT('Ctrl Pts',(-62.1093847101978,-104.407345183486,
177.642339485944));
#27259=CARTESIAN_POINT('Ctrl Pts',(-60.9344749627642,-104.438317183453,
178.813912312176));
#27260=CARTESIAN_POINT('Ctrl Pts',(-59.7595652153305,-104.46928918342,179.985485138407));
#27261=CARTESIAN_POINT('Ctrl Pts',(-58.1021084653266,-104.551703917706,
179.985485069079));
#27262=CARTESIAN_POINT('Ctrl Pts',(-56.4446517153227,-104.634118651992,
179.985484999752));
#27263=CARTESIAN_POINT('Ctrl Pts',(-55.269742065381,-104.665090641566,178.813912075476));
#27264=CARTESIAN_POINT('Ctrl Pts',(-54.0948324154392,-104.696062631139,
177.6423391512));
#27265=CARTESIAN_POINT('Ctrl Pts',(-54.0848944214593,-104.602840859135,
175.985484901707));
#27266=CARTESIAN_POINT('Ctrl Pts',(-54.0749564274795,-104.50961908713,174.328630652215));
#27267=CARTESIAN_POINT('Ctrl Pts',(-55.2299900490791,-104.292203557853,
173.157057825983));
#27268=CARTESIAN_POINT('Ctrl Pts',(-56.3850236706787,-104.074788028575,
171.985484999752));
#27269=CARTESIAN_POINT('Ctrl Pts',(-58.0226042948486,-103.805929764978,
171.985485069079));
#27270=CARTESIAN_POINT('Ctrl Pts',(-59.6601849190184,-103.537071501381,
171.985485138407));
#27271=CARTESIAN_POINT('Ctrl Pts',(-60.8152184431262,-103.319655982497,
173.157058062683));
#27272=CARTESIAN_POINT('Ctrl Pts',(-61.9702519672339,-103.102240463613,
174.328630986959));
#27273=CARTESIAN_POINT('Ctrl Pts',(-61.9603138353797,-103.009018706307,
175.985485236451));
#27274=CARTESIAN_POINT('Ctrl Pts',(-61.9503757035256,-102.915796949001,
177.642339485944));
#27275=CARTESIAN_POINT('Ctrl Pts',(-60.7754659560919,-102.946768948967,
178.813912312176));
#27276=CARTESIAN_POINT('Ctrl Pts',(-59.6005562086583,-102.977740948934,
179.985485138407));
#27277=CARTESIAN_POINT('Ctrl Pts',(-57.9430994586544,-103.06015568322,179.985485069079));
#27278=CARTESIAN_POINT('Ctrl Pts',(-56.2856427086505,-103.142570417507,
179.985484999752));
#27279=CARTESIAN_POINT('Ctrl Pts',(-55.1107330587087,-103.17354240708,178.813912075476));
#27280=CARTESIAN_POINT('Ctrl Pts',(-53.935823408767,-103.204514396654,177.6423391512));
#27281=CARTESIAN_POINT('Ctrl Pts',(-53.9258854147871,-103.111292624649,
175.985484901707));
#27282=CARTESIAN_POINT('Ctrl Pts',(-53.9159474208072,-103.018070852645,
174.328630652215));
#27283=CARTESIAN_POINT('Ctrl Pts',(-55.0709810424069,-102.800655323367,
173.157057825983));
#27284=CARTESIAN_POINT('Ctrl Pts',(-56.2260146640065,-102.58323979409,171.985484999752));
#27285=CARTESIAN_POINT('Ctrl Pts',(-57.8635952881763,-102.314381530493,
171.985485069079));
#27286=CARTESIAN_POINT('Ctrl Pts',(-59.5011759123462,-102.045523266896,
171.985485138407));
#27287=CARTESIAN_POINT('Ctrl Pts',(-60.6562094364539,-101.828107748012,
173.157058062683));
#27288=CARTESIAN_POINT('Ctrl Pts',(-61.8112429605617,-101.610692229127,
174.328630986959));
#27289=CARTESIAN_POINT('Ctrl Pts',(-61.8013048287075,-101.517470471821,
175.985485236451));
#27290=CARTESIAN_POINT('Ctrl Pts',(-61.7913666968533,-101.424248714515,
177.642339485944));
#27291=CARTESIAN_POINT('Ctrl Pts',(-60.6164569494197,-101.455220714482,
178.813912312176));
#27292=CARTESIAN_POINT('Ctrl Pts',(-59.4415472019861,-101.486192714449,
179.985485138407));
#27293=CARTESIAN_POINT('Ctrl Pts',(-57.7840904519822,-101.568607448735,
179.985485069079));
#27294=CARTESIAN_POINT('Ctrl Pts',(-56.1266337019783,-101.651022183021,
179.985484999752));
#27295=CARTESIAN_POINT('Ctrl Pts',(-54.9517240520365,-101.681994172595,
178.813912075476));
#27296=CARTESIAN_POINT('Ctrl Pts',(-53.7768144020947,-101.712966162168,
177.6423391512));
#27297=CARTESIAN_POINT('Ctrl Pts',(-53.7668764081149,-101.619744390164,
175.985484901707));
#27298=CARTESIAN_POINT('Ctrl Pts',(-53.756938414135,-101.526522618159,174.328630652215));
#27299=CARTESIAN_POINT('Ctrl Pts',(-54.9119720357346,-101.309107088882,
173.157057825983));
#27300=CARTESIAN_POINT('Ctrl Pts',(-56.0670056573342,-101.091691559604,
171.985484999752));
#27301=CARTESIAN_POINT('Ctrl Pts',(-57.7045862815041,-100.822833296007,
171.985485069079));
#27302=CARTESIAN_POINT('Ctrl Pts',(-59.342166905674,-100.55397503241,171.985485138407));
#27303=CARTESIAN_POINT('Ctrl Pts',(-60.4972004297817,-100.336559513526,
173.157058062683));
#27304=CARTESIAN_POINT('Ctrl Pts',(-61.6522339538895,-100.119143994642,
174.328630986959));
#27305=CARTESIAN_POINT('Ctrl Pts',(-61.6422958220353,-100.025922237336,
175.985485236451));
#27306=CARTESIAN_POINT('Ctrl Pts',(-61.6323576901811,-99.9327004800294,
177.642339485944));
#27307=CARTESIAN_POINT('Ctrl Pts',(-60.4574479427475,-99.9636724799962,
178.813912312176));
#27308=CARTESIAN_POINT('Ctrl Pts',(-59.2825381953138,-99.994644479963,179.985485138407));
#27309=CARTESIAN_POINT('Ctrl Pts',(-57.6250814453099,-100.077059214249,
179.985485069079));
#27310=CARTESIAN_POINT('Ctrl Pts',(-55.9676246953061,-100.159473948536,
179.985484999752));
#27311=CARTESIAN_POINT('Ctrl Pts',(-54.7927150453643,-100.190445938109,
178.813912075476));
#27312=CARTESIAN_POINT('Ctrl Pts',(-53.6178053954225,-100.221417927683,
177.6423391512));
#27313=CARTESIAN_POINT('Ctrl Pts',(-53.6078674014426,-100.128196155678,
175.985484901707));
#27314=CARTESIAN_POINT('Ctrl Pts',(-53.5979294074628,-100.034974383673,
174.328630652215));
#27315=CARTESIAN_POINT('Ctrl Pts',(-54.7529630290624,-99.817558854396,173.157057825983));
#27316=CARTESIAN_POINT('Ctrl Pts',(-55.907996650662,-99.6001433251185,171.985484999752));
#27317=CARTESIAN_POINT('Ctrl Pts',(-57.5455772748319,-99.3312850615215,
171.985485069079));
#27318=CARTESIAN_POINT('Ctrl Pts',(-59.1831578990017,-99.0624267979246,
171.985485138407));
#27319=CARTESIAN_POINT('Ctrl Pts',(-60.3381914231095,-98.8450112790404,
173.157058062683));
#27320=CARTESIAN_POINT('Ctrl Pts',(-61.4932249472172,-98.6275957601562,
174.328630986959));
#27321=CARTESIAN_POINT('Ctrl Pts',(-61.4832868153631,-98.53437400285,175.985485236451));
#27322=CARTESIAN_POINT('Ctrl Pts',(-61.4733486835089,-98.4411522455438,
177.642339485944));
#27323=CARTESIAN_POINT('Ctrl Pts',(-60.2984389360752,-98.4721242455106,
178.813912312176));
#27324=CARTESIAN_POINT('Ctrl Pts',(-59.1235291886416,-98.5030962454774,
179.985485138407));
#27325=CARTESIAN_POINT('Ctrl Pts',(-57.4660724386377,-98.5855109797636,
179.985485069079));
#27326=CARTESIAN_POINT('Ctrl Pts',(-55.8086156886338,-98.6679257140499,
179.985484999752));
#27327=CARTESIAN_POINT('Ctrl Pts',(-54.633706038692,-98.6988977036234,178.813912075476));
#27328=CARTESIAN_POINT('Ctrl Pts',(-56.2237961054143,-113.614380048479,
178.813912075476));
#27329=CARTESIAN_POINT('Ctrl Pts',(-55.0488864554725,-113.645352038053,
177.6423391512));
#27330=CARTESIAN_POINT('Ctrl Pts',(-55.0389484614927,-113.552130266048,
175.985484901707));
#27331=CARTESIAN_POINT('Ctrl Pts',(-55.0290104675128,-113.458908494044,
174.328630652215));
#27332=CARTESIAN_POINT('Ctrl Pts',(-56.1840440891124,-113.241492964766,
173.157057825983));
#27333=CARTESIAN_POINT('Ctrl Pts',(-57.3390777107121,-113.024077435489,
171.985484999752));
#27334=CARTESIAN_POINT('Ctrl Pts',(-58.9766583348819,-112.755219171892,
171.985485069079));
#27335=CARTESIAN_POINT('Ctrl Pts',(-60.6142389590518,-112.486360908295,
171.985485138407));
#27336=CARTESIAN_POINT('Ctrl Pts',(-61.7692724831595,-112.268945389411,
173.157058062683));
#27337=CARTESIAN_POINT('Ctrl Pts',(-62.9243060072673,-112.051529870527,
174.328630986959));
#27338=CARTESIAN_POINT('Ctrl Pts',(-62.9143678754131,-111.95830811322,175.985485236451));
#27339=CARTESIAN_POINT('Ctrl Pts',(-62.9044297435589,-111.865086355914,
177.642339485944));
#27340=CARTESIAN_POINT('Ctrl Pts',(-61.7295199961253,-111.896058355881,
178.813912312176));
#27341=CARTESIAN_POINT('Ctrl Pts',(-60.5546102486917,-111.927030355848,
179.985485138407));
#27342=CARTESIAN_POINT('Ctrl Pts',(-58.8971534986878,-112.009445090134,
179.985485069079));
#27343=CARTESIAN_POINT('Ctrl Pts',(-57.2396967486839,-112.09185982442,179.985484999752));
#27344=CARTESIAN_POINT('Ctrl Pts',(-56.0647870987421,-112.122831813994,
178.813912075476));
#27345=CARTESIAN_POINT('Ctrl Pts',(-54.8898774488003,-112.153803803567,
177.6423391512));
#27346=CARTESIAN_POINT('Ctrl Pts',(-54.8799394548205,-112.060582031563,
175.985484901707));
#27347=CARTESIAN_POINT('Ctrl Pts',(-54.8700014608406,-111.967360259558,
174.328630652215));
#27348=CARTESIAN_POINT('Ctrl Pts',(-56.0250350824402,-111.749944730281,
173.157057825983));
#27349=CARTESIAN_POINT('Ctrl Pts',(-57.1800687040398,-111.532529201003,
171.985484999752));
#27350=CARTESIAN_POINT('Ctrl Pts',(-58.8176493282097,-111.263670937406,
171.985485069079));
#27351=CARTESIAN_POINT('Ctrl Pts',(-60.4552299523796,-110.994812673809,
171.985485138407));
#27352=CARTESIAN_POINT('Ctrl Pts',(-61.6102634764873,-110.777397154925,
173.157058062683));
#27353=CARTESIAN_POINT('Ctrl Pts',(-62.7652970005951,-110.559981636041,
174.328630986959));
#27354=CARTESIAN_POINT('Ctrl Pts',(-62.7553588687409,-110.466759878735,
175.985485236451));
#27355=CARTESIAN_POINT('Ctrl Pts',(-62.7454207368867,-110.373538121429,
177.642339485944));
#27356=CARTESIAN_POINT('Ctrl Pts',(-61.5705109894531,-110.404510121395,
178.813912312176));
#27357=CARTESIAN_POINT('Ctrl Pts',(-60.3956012420194,-110.435482121362,
179.985485138407));
#27358=CARTESIAN_POINT('Ctrl Pts',(-58.7381444920155,-110.517896855648,
179.985485069079));
#27359=CARTESIAN_POINT('Ctrl Pts',(-57.0806877420116,-110.600311589935,
179.985484999752));
#27360=CARTESIAN_POINT('Ctrl Pts',(-55.9057780920699,-110.631283579508,
178.813912075476));
#27361=CARTESIAN_POINT('Ctrl Pts',(-54.7308684421281,-110.662255569082,
177.6423391512));
#27362=CARTESIAN_POINT('Ctrl Pts',(-54.7209304481482,-110.569033797077,
175.985484901707));
#27363=CARTESIAN_POINT('Ctrl Pts',(-54.7109924541684,-110.475812025073,
174.328630652215));
#27364=CARTESIAN_POINT('Ctrl Pts',(-55.866026075768,-110.258396495795,173.157057825983));
#27365=CARTESIAN_POINT('Ctrl Pts',(-57.0210596973676,-110.040980966518,
171.985484999752));
#27366=CARTESIAN_POINT('Ctrl Pts',(-58.6586403215375,-109.772122702921,
171.985485069079));
#27367=CARTESIAN_POINT('Ctrl Pts',(-60.2962209457073,-109.503264439324,
171.985485138407));
#27368=CARTESIAN_POINT('Ctrl Pts',(-61.4512544698151,-109.28584892044,173.157058062683));
#27369=CARTESIAN_POINT('Ctrl Pts',(-62.6062879939228,-109.068433401555,
174.328630986959));
#27370=CARTESIAN_POINT('Ctrl Pts',(-62.5963498620687,-108.975211644249,
175.985485236451));
#27371=CARTESIAN_POINT('Ctrl Pts',(-62.5864117302145,-108.881989886943,
177.642339485944));
#27372=CARTESIAN_POINT('Ctrl Pts',(-61.4115019827808,-108.91296188691,178.813912312176));
#27373=CARTESIAN_POINT('Ctrl Pts',(-60.2365922353472,-108.943933886877,
179.985485138407));
#27374=CARTESIAN_POINT('Ctrl Pts',(-58.5791354853433,-109.026348621163,
179.985485069079));
#27375=CARTESIAN_POINT('Ctrl Pts',(-56.9216787353394,-109.108763355449,
179.985484999752));
#27376=CARTESIAN_POINT('Ctrl Pts',(-55.7467690853976,-109.139735345023,
178.813912075476));
#27377=CARTESIAN_POINT('Ctrl Pts',(-54.5718594354559,-109.170707334596,
177.6423391512));
#27378=CARTESIAN_POINT('Ctrl Pts',(-54.561921441476,-109.077485562592,175.985484901707));
#27379=CARTESIAN_POINT('Ctrl Pts',(-54.5519834474962,-108.984263790587,
174.328630652215));
#27380=CARTESIAN_POINT('Ctrl Pts',(-55.7070170690958,-108.76684826131,173.157057825983));
#27381=CARTESIAN_POINT('Ctrl Pts',(-56.8620506906954,-108.549432732032,
171.985484999752));
#27382=CARTESIAN_POINT('Ctrl Pts',(-58.4996313148652,-108.280574468435,
171.985485069079));
#27383=CARTESIAN_POINT('Ctrl Pts',(-60.1372119390351,-108.011716204838,
171.985485138407));
#27384=CARTESIAN_POINT('Ctrl Pts',(-61.2922454631428,-107.794300685954,
173.157058062683));
#27385=CARTESIAN_POINT('Ctrl Pts',(-62.4472789872506,-107.57688516707,174.328630986959));
#27386=CARTESIAN_POINT('Ctrl Pts',(-62.4373408553964,-107.483663409764,
175.985485236451));
#27387=CARTESIAN_POINT('Ctrl Pts',(-62.4274027235423,-107.390441652457,
177.642339485944));
#27388=CARTESIAN_POINT('Ctrl Pts',(-61.2524929761086,-107.421413652424,
178.813912312176));
#27389=CARTESIAN_POINT('Ctrl Pts',(-60.077583228675,-107.452385652391,179.985485138407));
#27390=CARTESIAN_POINT('Ctrl Pts',(-58.4201264786711,-107.534800386677,
179.985485069079));
#27391=CARTESIAN_POINT('Ctrl Pts',(-56.7626697286672,-107.617215120964,
179.985484999752));
#27392=CARTESIAN_POINT('Ctrl Pts',(-55.5877600787254,-107.648187110537,
178.813912075476));
#27393=CARTESIAN_POINT('Ctrl Pts',(-54.4128504287836,-107.67915910011,177.6423391512));
#27394=CARTESIAN_POINT('Ctrl Pts',(-54.4029124348038,-107.585937328106,
175.985484901707));
#27395=CARTESIAN_POINT('Ctrl Pts',(-54.3929744408239,-107.492715556102,
174.328630652215));
#27396=CARTESIAN_POINT('Ctrl Pts',(-55.5480080624235,-107.275300026824,
173.157057825983));
#27397=CARTESIAN_POINT('Ctrl Pts',(-56.7030416840231,-107.057884497547,
171.985484999752));
#27398=CARTESIAN_POINT('Ctrl Pts',(-58.340622308193,-106.78902623395,171.985485069079));
#27399=CARTESIAN_POINT('Ctrl Pts',(-59.9782029323629,-106.520167970353,
171.985485138407));
#27400=CARTESIAN_POINT('Ctrl Pts',(-61.1332364564706,-106.302752451468,
173.157058062683));
#27401=CARTESIAN_POINT('Ctrl Pts',(-62.2882699805784,-106.085336932584,
174.328630986959));
#27402=CARTESIAN_POINT('Ctrl Pts',(-62.2783318487242,-105.992115175278,
175.985485236451));
#27403=CARTESIAN_POINT('Ctrl Pts',(-62.26839371687,-105.898893417972,177.642339485944));
#27404=CARTESIAN_POINT('Ctrl Pts',(-61.0934839694364,-105.929865417939,
178.813912312176));
#27405=CARTESIAN_POINT('Ctrl Pts',(-59.9185742220028,-105.960837417905,
179.985485138407));
#27406=CARTESIAN_POINT('Ctrl Pts',(-58.2611174719989,-106.043252152192,
179.985485069079));
#27407=CARTESIAN_POINT('Ctrl Pts',(-56.603660721995,-106.125666886478,179.985484999752));
#27408=CARTESIAN_POINT('Ctrl Pts',(-55.4287510720532,-106.156638876051,
178.813912075476));
#27409=CARTESIAN_POINT('Ctrl Pts',(-54.2538414221114,-106.187610865625,
177.6423391512));
#27410=CARTESIAN_POINT('Ctrl Pts',(-54.2439034281315,-106.09438909362,175.985484901707));
#27411=CARTESIAN_POINT('Ctrl Pts',(-54.2339654341517,-106.001167321616,
174.328630652215));
#27412=CARTESIAN_POINT('Ctrl Pts',(-55.3889990557513,-105.783751792338,
173.157057825983));
#27413=CARTESIAN_POINT('Ctrl Pts',(-56.5440326773509,-105.566336263061,
171.985484999752));
#27414=CARTESIAN_POINT('Ctrl Pts',(-58.1816133015208,-105.297477999464,
171.985485069079));
#27415=CARTESIAN_POINT('Ctrl Pts',(-59.8191939256906,-105.028619735867,
171.985485138407));
#27416=CARTESIAN_POINT('Ctrl Pts',(-60.9742274497984,-104.811204216983,
173.157058062683));
#27417=CARTESIAN_POINT('Ctrl Pts',(-62.1292609739061,-104.593788698099,
174.328630986959));
#27418=CARTESIAN_POINT('Ctrl Pts',(-62.119322842052,-104.500566940792,175.985485236451));
#27419=CARTESIAN_POINT('Ctrl Pts',(-62.1093847101978,-104.407345183486,
177.642339485944));
#27420=CARTESIAN_POINT('Ctrl Pts',(-60.9344749627642,-104.438317183453,
178.813912312176));
#27421=CARTESIAN_POINT('Ctrl Pts',(-59.7595652153305,-104.46928918342,179.985485138407));
#27422=CARTESIAN_POINT('Ctrl Pts',(-58.1021084653266,-104.551703917706,
179.985485069079));
#27423=CARTESIAN_POINT('Ctrl Pts',(-56.4446517153227,-104.634118651992,
179.985484999752));
#27424=CARTESIAN_POINT('Ctrl Pts',(-55.269742065381,-104.665090641566,178.813912075476));
#27425=CARTESIAN_POINT('Ctrl Pts',(-54.0948324154392,-104.696062631139,
177.6423391512));
#27426=CARTESIAN_POINT('Ctrl Pts',(-54.0848944214593,-104.602840859135,
175.985484901707));
#27427=CARTESIAN_POINT('Ctrl Pts',(-54.0749564274795,-104.50961908713,174.328630652215));
#27428=CARTESIAN_POINT('Ctrl Pts',(-55.2299900490791,-104.292203557853,
173.157057825983));
#27429=CARTESIAN_POINT('Ctrl Pts',(-56.3850236706787,-104.074788028575,
171.985484999752));
#27430=CARTESIAN_POINT('Ctrl Pts',(-58.0226042948486,-103.805929764978,
171.985485069079));
#27431=CARTESIAN_POINT('Ctrl Pts',(-59.6601849190184,-103.537071501381,
171.985485138407));
#27432=CARTESIAN_POINT('Ctrl Pts',(-60.8152184431262,-103.319655982497,
173.157058062683));
#27433=CARTESIAN_POINT('Ctrl Pts',(-61.9702519672339,-103.102240463613,
174.328630986959));
#27434=CARTESIAN_POINT('Ctrl Pts',(-61.9603138353797,-103.009018706307,
175.985485236451));
#27435=CARTESIAN_POINT('Ctrl Pts',(-61.9503757035256,-102.915796949001,
177.642339485944));
#27436=CARTESIAN_POINT('Ctrl Pts',(-60.7754659560919,-102.946768948967,
178.813912312176));
#27437=CARTESIAN_POINT('Ctrl Pts',(-59.6005562086583,-102.977740948934,
179.985485138407));
#27438=CARTESIAN_POINT('Ctrl Pts',(-57.9430994586544,-103.06015568322,179.985485069079));
#27439=CARTESIAN_POINT('Ctrl Pts',(-56.2856427086505,-103.142570417507,
179.985484999752));
#27440=CARTESIAN_POINT('Ctrl Pts',(-55.1107330587087,-103.17354240708,178.813912075476));
#27441=CARTESIAN_POINT('Ctrl Pts',(-53.935823408767,-103.204514396654,177.6423391512));
#27442=CARTESIAN_POINT('Ctrl Pts',(-53.9258854147871,-103.111292624649,
175.985484901707));
#27443=CARTESIAN_POINT('Ctrl Pts',(-53.9159474208072,-103.018070852645,
174.328630652215));
#27444=CARTESIAN_POINT('Ctrl Pts',(-55.0709810424069,-102.800655323367,
173.157057825983));
#27445=CARTESIAN_POINT('Ctrl Pts',(-56.2260146640065,-102.58323979409,171.985484999752));
#27446=CARTESIAN_POINT('Ctrl Pts',(-57.8635952881763,-102.314381530493,
171.985485069079));
#27447=CARTESIAN_POINT('Ctrl Pts',(-59.5011759123462,-102.045523266896,
171.985485138407));
#27448=CARTESIAN_POINT('Ctrl Pts',(-60.6562094364539,-101.828107748012,
173.157058062683));
#27449=CARTESIAN_POINT('Ctrl Pts',(-61.8112429605617,-101.610692229127,
174.328630986959));
#27450=CARTESIAN_POINT('Ctrl Pts',(-61.8013048287075,-101.517470471821,
175.985485236451));
#27451=CARTESIAN_POINT('Ctrl Pts',(-61.7913666968533,-101.424248714515,
177.642339485944));
#27452=CARTESIAN_POINT('Ctrl Pts',(-60.6164569494197,-101.455220714482,
178.813912312176));
#27453=CARTESIAN_POINT('Ctrl Pts',(-59.4415472019861,-101.486192714449,
179.985485138407));
#27454=CARTESIAN_POINT('Ctrl Pts',(-57.7840904519822,-101.568607448735,
179.985485069079));
#27455=CARTESIAN_POINT('Ctrl Pts',(-56.1266337019783,-101.651022183021,
179.985484999752));
#27456=CARTESIAN_POINT('Ctrl Pts',(-54.9517240520365,-101.681994172595,
178.813912075476));
#27457=CARTESIAN_POINT('Ctrl Pts',(-53.7768144020947,-101.712966162168,
177.6423391512));
#27458=CARTESIAN_POINT('Ctrl Pts',(-53.7668764081149,-101.619744390164,
175.985484901707));
#27459=CARTESIAN_POINT('Ctrl Pts',(-53.756938414135,-101.526522618159,174.328630652215));
#27460=CARTESIAN_POINT('Ctrl Pts',(-54.9119720357346,-101.309107088882,
173.157057825983));
#27461=CARTESIAN_POINT('Ctrl Pts',(-56.0670056573342,-101.091691559604,
171.985484999752));
#27462=CARTESIAN_POINT('Ctrl Pts',(-57.7045862815041,-100.822833296007,
171.985485069079));
#27463=CARTESIAN_POINT('Ctrl Pts',(-59.342166905674,-100.55397503241,171.985485138407));
#27464=CARTESIAN_POINT('Ctrl Pts',(-60.4972004297817,-100.336559513526,
173.157058062683));
#27465=CARTESIAN_POINT('Ctrl Pts',(-61.6522339538895,-100.119143994642,
174.328630986959));
#27466=CARTESIAN_POINT('Ctrl Pts',(-61.6422958220353,-100.025922237336,
175.985485236451));
#27467=CARTESIAN_POINT('Ctrl Pts',(-61.6323576901811,-99.9327004800294,
177.642339485944));
#27468=CARTESIAN_POINT('Ctrl Pts',(-60.4574479427475,-99.9636724799962,
178.813912312176));
#27469=CARTESIAN_POINT('Ctrl Pts',(-59.2825381953138,-99.994644479963,179.985485138407));
#27470=CARTESIAN_POINT('Ctrl Pts',(-57.6250814453099,-100.077059214249,
179.985485069079));
#27471=CARTESIAN_POINT('Ctrl Pts',(-55.9676246953061,-100.159473948536,
179.985484999752));
#27472=CARTESIAN_POINT('Ctrl Pts',(-54.7927150453643,-100.190445938109,
178.813912075476));
#27473=CARTESIAN_POINT('Ctrl Pts',(-53.6178053954225,-100.221417927683,
177.6423391512));
#27474=CARTESIAN_POINT('Ctrl Pts',(-53.6078674014426,-100.128196155678,
175.985484901707));
#27475=CARTESIAN_POINT('Ctrl Pts',(-53.5979294074628,-100.034974383673,
174.328630652215));
#27476=CARTESIAN_POINT('Ctrl Pts',(-54.7529630290624,-99.817558854396,173.157057825983));
#27477=CARTESIAN_POINT('Ctrl Pts',(-55.907996650662,-99.6001433251185,171.985484999752));
#27478=CARTESIAN_POINT('Ctrl Pts',(-57.5455772748319,-99.3312850615215,
171.985485069079));
#27479=CARTESIAN_POINT('Ctrl Pts',(-59.1831578990017,-99.0624267979246,
171.985485138407));
#27480=CARTESIAN_POINT('Ctrl Pts',(-60.3381914231095,-98.8450112790404,
173.157058062683));
#27481=CARTESIAN_POINT('Ctrl Pts',(-61.4932249472172,-98.6275957601562,
174.328630986959));
#27482=CARTESIAN_POINT('Ctrl Pts',(-61.4832868153631,-98.53437400285,175.985485236451));
#27483=CARTESIAN_POINT('Ctrl Pts',(-61.4733486835089,-98.4411522455438,
177.642339485944));
#27484=CARTESIAN_POINT('Ctrl Pts',(-60.2984389360752,-98.4721242455106,
178.813912312176));
#27485=CARTESIAN_POINT('Ctrl Pts',(-59.1235291886416,-98.5030962454774,
179.985485138407));
#27486=CARTESIAN_POINT('Ctrl Pts',(-57.4660724386377,-98.5855109797636,
179.985485069079));
#27487=CARTESIAN_POINT('Ctrl Pts',(-55.8086156886338,-98.6679257140499,
179.985484999752));
#27488=CARTESIAN_POINT('Ctrl Pts',(-54.633706038692,-98.6988977036234,178.813912075476));
#27489=CARTESIAN_POINT('Ctrl Pts',(-56.9964983346804,-113.864655531781,
178.072094410988));
#27490=CARTESIAN_POINT('Ctrl Pts',(-56.1271283009022,-113.863054956993,
177.207792449865));
#27491=CARTESIAN_POINT('Ctrl Pts',(-56.117190288842,-113.769833186916,175.985484945604));
#27492=CARTESIAN_POINT('Ctrl Pts',(-56.1072522767819,-113.676611416839,
174.763177441344));
#27493=CARTESIAN_POINT('Ctrl Pts',(-56.9567462566485,-113.491768454648,
173.89887555255));
#27494=CARTESIAN_POINT('Ctrl Pts',(-57.8062402365152,-113.306925492458,
173.034573663757));
#27495=CARTESIAN_POINT('Ctrl Pts',(-59.011722573584,-113.084131793069,173.034573714903));
#27496=CARTESIAN_POINT('Ctrl Pts',(-60.2172049106529,-112.86133809368,173.034573766048));
#27497=CARTESIAN_POINT('Ctrl Pts',(-61.0666988185971,-112.676495139156,
173.898875727171));
#27498=CARTESIAN_POINT('Ctrl Pts',(-61.9161927265413,-112.491652184633,
174.763177688294));
#27499=CARTESIAN_POINT('Ctrl Pts',(-61.9062546127674,-112.398430425399,
175.985485192554));
#27500=CARTESIAN_POINT('Ctrl Pts',(-61.8963164989935,-112.305208666166,
177.207792696815));
#27501=CARTESIAN_POINT('Ctrl Pts',(-61.0269463932928,-112.303608099046,
178.072094585608));
#27502=CARTESIAN_POINT('Ctrl Pts',(-60.1575762875921,-112.302007531926,
178.936396474401));
#27503=CARTESIAN_POINT('Ctrl Pts',(-58.9322178246893,-112.338357702004,
178.936396423256));
#27504=CARTESIAN_POINT('Ctrl Pts',(-57.7068593617864,-112.374707872082,
178.936396372111));
#27505=CARTESIAN_POINT('Ctrl Pts',(-56.8374893280082,-112.373107297295,
178.072094410988));
#27506=CARTESIAN_POINT('Ctrl Pts',(-55.9681192942299,-112.371506722508,
177.207792449865));
#27507=CARTESIAN_POINT('Ctrl Pts',(-55.9581812821698,-112.278284952431,
175.985484945604));
#27508=CARTESIAN_POINT('Ctrl Pts',(-55.9482432701096,-112.185063182354,
174.763177441344));
#27509=CARTESIAN_POINT('Ctrl Pts',(-56.7977372499763,-112.000220220163,
173.89887555255));
#27510=CARTESIAN_POINT('Ctrl Pts',(-57.647231229843,-111.815377257972,173.034573663757));
#27511=CARTESIAN_POINT('Ctrl Pts',(-58.8527135669118,-111.592583558583,
173.034573714903));
#27512=CARTESIAN_POINT('Ctrl Pts',(-60.0581959039807,-111.369789859194,
173.034573766048));
#27513=CARTESIAN_POINT('Ctrl Pts',(-60.9076898119249,-111.184946904671,
173.898875727171));
#27514=CARTESIAN_POINT('Ctrl Pts',(-61.7571837198691,-111.000103950148,
174.763177688294));
#27515=CARTESIAN_POINT('Ctrl Pts',(-61.7472456060952,-110.906882190914,
175.985485192554));
#27516=CARTESIAN_POINT('Ctrl Pts',(-61.7373074923213,-110.81366043168,177.207792696815));
#27517=CARTESIAN_POINT('Ctrl Pts',(-60.8679373866206,-110.81205986456,178.072094585608));
#27518=CARTESIAN_POINT('Ctrl Pts',(-59.9985672809199,-110.81045929744,178.936396474401));
#27519=CARTESIAN_POINT('Ctrl Pts',(-58.7732088180171,-110.846809467519,
178.936396423256));
#27520=CARTESIAN_POINT('Ctrl Pts',(-57.5478503551142,-110.883159637597,
178.936396372111));
#27521=CARTESIAN_POINT('Ctrl Pts',(-56.6784803213359,-110.881559062809,
178.072094410988));
#27522=CARTESIAN_POINT('Ctrl Pts',(-55.8091102875577,-110.879958488022,
177.207792449865));
#27523=CARTESIAN_POINT('Ctrl Pts',(-55.7991722754976,-110.786736717945,
175.985484945604));
#27524=CARTESIAN_POINT('Ctrl Pts',(-55.7892342634374,-110.693514947868,
174.763177441344));
#27525=CARTESIAN_POINT('Ctrl Pts',(-56.6387282433041,-110.508671985677,
173.89887555255));
#27526=CARTESIAN_POINT('Ctrl Pts',(-57.4882222231708,-110.323829023487,
173.034573663757));
#27527=CARTESIAN_POINT('Ctrl Pts',(-58.6937045602396,-110.101035324098,
173.034573714903));
#27528=CARTESIAN_POINT('Ctrl Pts',(-59.8991868973084,-109.878241624709,
173.034573766048));
#27529=CARTESIAN_POINT('Ctrl Pts',(-60.7486808052526,-109.693398670185,
173.898875727171));
#27530=CARTESIAN_POINT('Ctrl Pts',(-61.5981747131968,-109.508555715662,
174.763177688294));
#27531=CARTESIAN_POINT('Ctrl Pts',(-61.588236599423,-109.415333956428,175.985485192554));
#27532=CARTESIAN_POINT('Ctrl Pts',(-61.5782984856491,-109.322112197195,
177.207792696815));
#27533=CARTESIAN_POINT('Ctrl Pts',(-60.7089283799484,-109.320511630075,
178.072094585608));
#27534=CARTESIAN_POINT('Ctrl Pts',(-59.8395582742477,-109.318911062955,
178.936396474401));
#27535=CARTESIAN_POINT('Ctrl Pts',(-58.6141998113448,-109.355261233033,
178.936396423256));
#27536=CARTESIAN_POINT('Ctrl Pts',(-57.388841348442,-109.391611403111,178.936396372111));
#27537=CARTESIAN_POINT('Ctrl Pts',(-56.5194713146637,-109.390010828324,
178.072094410988));
#27538=CARTESIAN_POINT('Ctrl Pts',(-55.6501012808855,-109.388410253536,
177.207792449865));
#27539=CARTESIAN_POINT('Ctrl Pts',(-55.6401632688253,-109.295188483459,
175.985484945604));
#27540=CARTESIAN_POINT('Ctrl Pts',(-55.6302252567652,-109.201966713382,
174.763177441344));
#27541=CARTESIAN_POINT('Ctrl Pts',(-56.4797192366319,-109.017123751192,
173.89887555255));
#27542=CARTESIAN_POINT('Ctrl Pts',(-57.3292132164985,-108.832280789001,
173.034573663757));
#27543=CARTESIAN_POINT('Ctrl Pts',(-58.5346955535674,-108.609487089612,
173.034573714903));
#27544=CARTESIAN_POINT('Ctrl Pts',(-59.7401778906362,-108.386693390223,
173.034573766048));
#27545=CARTESIAN_POINT('Ctrl Pts',(-60.5896717985804,-108.2018504357,173.898875727171));
#27546=CARTESIAN_POINT('Ctrl Pts',(-61.4391657065246,-108.017007481176,
174.763177688294));
#27547=CARTESIAN_POINT('Ctrl Pts',(-61.4292275927507,-107.923785721943,
175.985485192554));
#27548=CARTESIAN_POINT('Ctrl Pts',(-61.4192894789769,-107.830563962709,
177.207792696815));
#27549=CARTESIAN_POINT('Ctrl Pts',(-60.5499193732762,-107.828963395589,
178.072094585608));
#27550=CARTESIAN_POINT('Ctrl Pts',(-59.6805492675755,-107.827362828469,
178.936396474401));
#27551=CARTESIAN_POINT('Ctrl Pts',(-58.4551908046726,-107.863712998547,
178.936396423256));
#27552=CARTESIAN_POINT('Ctrl Pts',(-57.2298323417698,-107.900063168626,
178.936396372111));
#27553=CARTESIAN_POINT('Ctrl Pts',(-56.3604623079915,-107.898462593838,
178.072094410988));
#27554=CARTESIAN_POINT('Ctrl Pts',(-55.4910922742133,-107.896862019051,
177.207792449865));
#27555=CARTESIAN_POINT('Ctrl Pts',(-55.4811542621531,-107.803640248974,
175.985484945604));
#27556=CARTESIAN_POINT('Ctrl Pts',(-55.471216250093,-107.710418478897,174.763177441344));
#27557=CARTESIAN_POINT('Ctrl Pts',(-56.3207102299596,-107.525575516706,
173.89887555255));
#27558=CARTESIAN_POINT('Ctrl Pts',(-57.1702042098263,-107.340732554515,
173.034573663757));
#27559=CARTESIAN_POINT('Ctrl Pts',(-58.3756865468951,-107.117938855126,
173.034573714903));
#27560=CARTESIAN_POINT('Ctrl Pts',(-59.581168883964,-106.895145155737,173.034573766048));
#27561=CARTESIAN_POINT('Ctrl Pts',(-60.4306627919082,-106.710302201214,
173.898875727171));
#27562=CARTESIAN_POINT('Ctrl Pts',(-61.2801566998524,-106.525459246691,
174.763177688294));
#27563=CARTESIAN_POINT('Ctrl Pts',(-61.2702185860785,-106.432237487457,
175.985485192554));
#27564=CARTESIAN_POINT('Ctrl Pts',(-61.2602804723046,-106.339015728223,
177.207792696815));
#27565=CARTESIAN_POINT('Ctrl Pts',(-60.3909103666039,-106.337415161103,
178.072094585608));
#27566=CARTESIAN_POINT('Ctrl Pts',(-59.5215402609032,-106.335814593983,
178.936396474401));
#27567=CARTESIAN_POINT('Ctrl Pts',(-58.2961817980004,-106.372164764062,
178.936396423256));
#27568=CARTESIAN_POINT('Ctrl Pts',(-57.0708233350975,-106.40851493414,178.936396372111));
#27569=CARTESIAN_POINT('Ctrl Pts',(-56.2014533013193,-106.406914359353,
178.072094410988));
#27570=CARTESIAN_POINT('Ctrl Pts',(-55.332083267541,-106.405313784565,177.207792449865));
#27571=CARTESIAN_POINT('Ctrl Pts',(-55.3221452554809,-106.312092014488,
175.985484945604));
#27572=CARTESIAN_POINT('Ctrl Pts',(-55.3122072434207,-106.218870244411,
174.763177441344));
#27573=CARTESIAN_POINT('Ctrl Pts',(-56.1617012232874,-106.034027282221,
173.89887555255));
#27574=CARTESIAN_POINT('Ctrl Pts',(-57.0111952031541,-105.84918432003,173.034573663757));
#27575=CARTESIAN_POINT('Ctrl Pts',(-58.2166775402229,-105.626390620641,
173.034573714903));
#27576=CARTESIAN_POINT('Ctrl Pts',(-59.4221598772917,-105.403596921252,
173.034573766048));
#27577=CARTESIAN_POINT('Ctrl Pts',(-60.2716537852359,-105.218753966728,
173.898875727171));
#27578=CARTESIAN_POINT('Ctrl Pts',(-61.1211476931802,-105.033911012205,
174.763177688294));
#27579=CARTESIAN_POINT('Ctrl Pts',(-61.1112095794063,-104.940689252971,
175.985485192554));
#27580=CARTESIAN_POINT('Ctrl Pts',(-61.1012714656324,-104.847467493738,
177.207792696815));
#27581=CARTESIAN_POINT('Ctrl Pts',(-60.2319013599317,-104.845866926618,
178.072094585608));
#27582=CARTESIAN_POINT('Ctrl Pts',(-59.362531254231,-104.844266359498,178.936396474401));
#27583=CARTESIAN_POINT('Ctrl Pts',(-58.1371727913281,-104.880616529576,
178.936396423256));
#27584=CARTESIAN_POINT('Ctrl Pts',(-56.9118143284253,-104.916966699654,
178.936396372111));
#27585=CARTESIAN_POINT('Ctrl Pts',(-56.042444294647,-104.915366124867,178.072094410988));
#27586=CARTESIAN_POINT('Ctrl Pts',(-55.1730742608688,-104.91376555008,177.207792449865));
#27587=CARTESIAN_POINT('Ctrl Pts',(-55.1631362488087,-104.820543780003,
175.985484945604));
#27588=CARTESIAN_POINT('Ctrl Pts',(-55.1531982367485,-104.727322009926,
174.763177441344));
#27589=CARTESIAN_POINT('Ctrl Pts',(-56.0026922166152,-104.542479047735,
173.89887555255));
#27590=CARTESIAN_POINT('Ctrl Pts',(-56.8521861964818,-104.357636085544,
173.034573663757));
#27591=CARTESIAN_POINT('Ctrl Pts',(-58.0576685335507,-104.134842386155,
173.034573714903));
#27592=CARTESIAN_POINT('Ctrl Pts',(-59.2631508706195,-103.912048686766,
173.034573766048));
#27593=CARTESIAN_POINT('Ctrl Pts',(-60.1126447785637,-103.727205732243,
173.898875727171));
#27594=CARTESIAN_POINT('Ctrl Pts',(-60.9621386865079,-103.54236277772,174.763177688294));
#27595=CARTESIAN_POINT('Ctrl Pts',(-60.952200572734,-103.449141018486,175.985485192554));
#27596=CARTESIAN_POINT('Ctrl Pts',(-60.9422624589602,-103.355919259252,
177.207792696815));
#27597=CARTESIAN_POINT('Ctrl Pts',(-60.0728923532595,-103.354318692132,
178.072094585608));
#27598=CARTESIAN_POINT('Ctrl Pts',(-59.2035222475588,-103.352718125012,
178.936396474401));
#27599=CARTESIAN_POINT('Ctrl Pts',(-57.9781637846559,-103.389068295091,
178.936396423256));
#27600=CARTESIAN_POINT('Ctrl Pts',(-56.7528053217531,-103.425418465169,
178.936396372111));
#27601=CARTESIAN_POINT('Ctrl Pts',(-55.8834352879748,-103.423817890381,
178.072094410988));
#27602=CARTESIAN_POINT('Ctrl Pts',(-55.0140652541966,-103.422217315594,
177.207792449865));
#27603=CARTESIAN_POINT('Ctrl Pts',(-55.0041272421364,-103.328995545517,
175.985484945604));
#27604=CARTESIAN_POINT('Ctrl Pts',(-54.9941892300763,-103.23577377544,174.763177441344));
#27605=CARTESIAN_POINT('Ctrl Pts',(-55.8436832099429,-103.050930813249,
173.89887555255));
#27606=CARTESIAN_POINT('Ctrl Pts',(-56.6931771898096,-102.866087851059,
173.034573663757));
#27607=CARTESIAN_POINT('Ctrl Pts',(-57.8986595268784,-102.64329415167,173.034573714903));
#27608=CARTESIAN_POINT('Ctrl Pts',(-59.1041418639473,-102.420500452281,
173.034573766048));
#27609=CARTESIAN_POINT('Ctrl Pts',(-59.9536357718915,-102.235657497757,
173.898875727171));
#27610=CARTESIAN_POINT('Ctrl Pts',(-60.8031296798357,-102.050814543234,
174.763177688294));
#27611=CARTESIAN_POINT('Ctrl Pts',(-60.7931915660618,-101.957592784,175.985485192554));
#27612=CARTESIAN_POINT('Ctrl Pts',(-60.783253452288,-101.864371024767,177.207792696815));
#27613=CARTESIAN_POINT('Ctrl Pts',(-59.9138833465873,-101.862770457647,
178.072094585608));
#27614=CARTESIAN_POINT('Ctrl Pts',(-59.0445132408866,-101.861169890527,
178.936396474401));
#27615=CARTESIAN_POINT('Ctrl Pts',(-57.8191547779837,-101.897520060605,
178.936396423256));
#27616=CARTESIAN_POINT('Ctrl Pts',(-56.5937963150808,-101.933870230683,
178.936396372111));
#27617=CARTESIAN_POINT('Ctrl Pts',(-55.7244262813026,-101.932269655896,
178.072094410988));
#27618=CARTESIAN_POINT('Ctrl Pts',(-54.8550562475244,-101.930669081108,
177.207792449865));
#27619=CARTESIAN_POINT('Ctrl Pts',(-54.8451182354642,-101.837447311031,
175.985484945604));
#27620=CARTESIAN_POINT('Ctrl Pts',(-54.8351802234041,-101.744225540954,
174.763177441344));
#27621=CARTESIAN_POINT('Ctrl Pts',(-55.6846742032707,-101.559382578764,
173.89887555255));
#27622=CARTESIAN_POINT('Ctrl Pts',(-56.5341681831374,-101.374539616573,
173.034573663757));
#27623=CARTESIAN_POINT('Ctrl Pts',(-57.7396505202062,-101.151745917184,
173.034573714903));
#27624=CARTESIAN_POINT('Ctrl Pts',(-58.9451328572751,-100.928952217795,
173.034573766048));
#27625=CARTESIAN_POINT('Ctrl Pts',(-59.7946267652193,-100.744109263272,
173.898875727171));
#27626=CARTESIAN_POINT('Ctrl Pts',(-60.6441206731635,-100.559266308748,
174.763177688294));
#27627=CARTESIAN_POINT('Ctrl Pts',(-60.6341825593896,-100.466044549515,
175.985485192554));
#27628=CARTESIAN_POINT('Ctrl Pts',(-60.6242444456157,-100.372822790281,
177.207792696815));
#27629=CARTESIAN_POINT('Ctrl Pts',(-59.754874339915,-100.371222223161,178.072094585608));
#27630=CARTESIAN_POINT('Ctrl Pts',(-58.8855042342143,-100.369621656041,
178.936396474401));
#27631=CARTESIAN_POINT('Ctrl Pts',(-57.6601457713115,-100.405971826119,
178.936396423256));
#27632=CARTESIAN_POINT('Ctrl Pts',(-56.4347873084086,-100.442321996198,
178.936396372111));
#27633=CARTESIAN_POINT('Ctrl Pts',(-55.5654172746304,-100.44072142141,178.072094410988));
#27634=CARTESIAN_POINT('Ctrl Pts',(-54.6960472408521,-100.439120846623,
177.207792449865));
#27635=CARTESIAN_POINT('Ctrl Pts',(-54.686109228792,-100.345899076546,175.985484945604));
#27636=CARTESIAN_POINT('Ctrl Pts',(-54.6761712167318,-100.252677306469,
174.763177441344));
#27637=CARTESIAN_POINT('Ctrl Pts',(-55.5256651965985,-100.067834344278,
173.89887555255));
#27638=CARTESIAN_POINT('Ctrl Pts',(-56.3751591764652,-99.8829913820874,
173.034573663757));
#27639=CARTESIAN_POINT('Ctrl Pts',(-57.580641513534,-99.6601976826983,173.034573714903));
#27640=CARTESIAN_POINT('Ctrl Pts',(-58.7861238506028,-99.4374039833093,
173.034573766048));
#27641=CARTESIAN_POINT('Ctrl Pts',(-59.635617758547,-99.252561028786,173.898875727171));
#27642=CARTESIAN_POINT('Ctrl Pts',(-60.4851116664912,-99.0677180742627,
174.763177688294));
#27643=CARTESIAN_POINT('Ctrl Pts',(-60.4751735527174,-98.9744963150291,
175.985485192554));
#27644=CARTESIAN_POINT('Ctrl Pts',(-60.4652354389435,-98.8812745557954,
177.207792696815));
#27645=CARTESIAN_POINT('Ctrl Pts',(-59.5958653332428,-98.8796739886754,
178.072094585608));
#27646=CARTESIAN_POINT('Ctrl Pts',(-58.7264952275421,-98.8780734215554,
178.936396474401));
#27647=CARTESIAN_POINT('Ctrl Pts',(-57.5011367646392,-98.9144235916337,
178.936396423256));
#27648=CARTESIAN_POINT('Ctrl Pts',(-56.2757783017364,-98.9507737617121,
178.936396372111));
#27649=CARTESIAN_POINT('Ctrl Pts',(-55.4064082679581,-98.9491731869247,
178.072094410988));
#27650=CARTESIAN_POINT('Ctrl Pts',(-61.5476086001415,-107.415572466264,
178.485485069079));
#27651=CARTESIAN_POINT('Ctrl Pts',(-61.4090363957847,-107.417286984142,
178.657813499464));
#27652=CARTESIAN_POINT('Ctrl Pts',(-61.2524929761086,-107.421413652424,
178.813912312176));
#27653=CARTESIAN_POINT('Ctrl Pts',(-60.077583228675,-107.452385652391,179.985485138407));
#27654=CARTESIAN_POINT('Ctrl Pts',(-58.4201264786711,-107.534800386677,
179.985485069079));
#27655=CARTESIAN_POINT('Ctrl Pts',(-56.7626697286672,-107.617215120964,
179.985484999752));
#27656=CARTESIAN_POINT('Ctrl Pts',(-55.5877600787254,-107.648187110537,
178.813912075476));
#27657=CARTESIAN_POINT('Ctrl Pts',(-54.4128504287836,-107.67915910011,177.6423391512));
#27658=CARTESIAN_POINT('Ctrl Pts',(-54.4029124348038,-107.585937328106,
175.985484901707));
#27659=CARTESIAN_POINT('Ctrl Pts',(-54.3929744408239,-107.492715556101,
174.328630652215));
#27660=CARTESIAN_POINT('Ctrl Pts',(-55.5480080624235,-107.275300026824,
173.157057825983));
#27661=CARTESIAN_POINT('Ctrl Pts',(-56.7030416840231,-107.057884497547,
171.985484999752));
#27662=CARTESIAN_POINT('Ctrl Pts',(-58.340622308193,-106.78902623395,171.985485069079));
#27663=CARTESIAN_POINT('Ctrl Pts',(-59.9782029323629,-106.520167970353,
171.985485138407));
#27664=CARTESIAN_POINT('Ctrl Pts',(-61.1332364564706,-106.302752451468,
173.157058062683));
#27665=CARTESIAN_POINT('Ctrl Pts',(-61.2871314774238,-106.273784317526,
173.313156769748));
#27666=CARTESIAN_POINT('Ctrl Pts',(-61.4229506813946,-106.246246888344,
173.485485069079));
#27667=CARTESIAN_POINT('Ctrl Pts',(-56.8733667677527,-112.709647553905,
178.072094410988));
#27668=CARTESIAN_POINT('Ctrl Pts',(-56.0039967339745,-112.708046979118,
177.207792449865));
#27669=CARTESIAN_POINT('Ctrl Pts',(-55.9940587219143,-112.614825209041,
175.985484945604));
#27670=CARTESIAN_POINT('Ctrl Pts',(-55.9841207098542,-112.521603438964,
174.763177441344));
#27671=CARTESIAN_POINT('Ctrl Pts',(-56.8336146897208,-112.336760476773,
173.89887555255));
#27672=CARTESIAN_POINT('Ctrl Pts',(-57.6831086695875,-112.151917514582,
173.034573663757));
#27673=CARTESIAN_POINT('Ctrl Pts',(-58.8885910066563,-111.929123815193,
173.034573714903));
#27674=CARTESIAN_POINT('Ctrl Pts',(-60.0940733437252,-111.706330115804,
173.034573766048));
#27675=CARTESIAN_POINT('Ctrl Pts',(-60.9435672516694,-111.521487161281,
173.898875727171));
#27676=CARTESIAN_POINT('Ctrl Pts',(-61.7930611596136,-111.336644206758,
174.763177688294));
#27677=CARTESIAN_POINT('Ctrl Pts',(-61.7831230458397,-111.243422447524,
175.985485192554));
#27678=CARTESIAN_POINT('Ctrl Pts',(-61.7731849320658,-111.15020068829,177.207792696815));
#27679=CARTESIAN_POINT('Ctrl Pts',(-60.9038148263651,-111.14860012117,178.072094585608));
#27680=CARTESIAN_POINT('Ctrl Pts',(-60.0344447206644,-111.14699955405,178.936396474401));
#27681=CARTESIAN_POINT('Ctrl Pts',(-58.8090862577616,-111.183349724129,
178.936396423256));
#27682=CARTESIAN_POINT('Ctrl Pts',(-57.5837277948587,-111.219699894207,
178.936396372111));
#27683=CARTESIAN_POINT('Ctrl Pts',(-56.7143577610805,-111.21809931942,178.072094410988));
#27684=CARTESIAN_POINT('Ctrl Pts',(-55.8449877273022,-111.216498744632,
177.207792449865));
#27685=CARTESIAN_POINT('Ctrl Pts',(-55.8350497152421,-111.123276974555,
175.985484945604));
#27686=CARTESIAN_POINT('Ctrl Pts',(-55.8251117031819,-111.030055204478,
174.763177441344));
#27687=CARTESIAN_POINT('Ctrl Pts',(-56.6746056830486,-110.845212242287,
173.89887555255));
#27688=CARTESIAN_POINT('Ctrl Pts',(-57.5240996629153,-110.660369280097,
173.034573663757));
#27689=CARTESIAN_POINT('Ctrl Pts',(-58.7295819999841,-110.437575580708,
173.034573714903));
#27690=CARTESIAN_POINT('Ctrl Pts',(-59.9350643370529,-110.214781881319,
173.034573766048));
#27691=CARTESIAN_POINT('Ctrl Pts',(-60.7845582449971,-110.029938926795,
173.898875727171));
#27692=CARTESIAN_POINT('Ctrl Pts',(-61.6340521529414,-109.845095972272,
174.763177688294));
#27693=CARTESIAN_POINT('Ctrl Pts',(-61.6241140391675,-109.751874213038,
175.985485192554));
#27694=CARTESIAN_POINT('Ctrl Pts',(-61.6141759253936,-109.658652453805,
177.207792696815));
#27695=CARTESIAN_POINT('Ctrl Pts',(-60.7448058196929,-109.657051886685,
178.072094585608));
#27696=CARTESIAN_POINT('Ctrl Pts',(-59.8754357139922,-109.655451319565,
178.936396474401));
#27697=CARTESIAN_POINT('Ctrl Pts',(-58.6500772510893,-109.691801489643,
178.936396423256));
#27698=CARTESIAN_POINT('Ctrl Pts',(-57.4247187881865,-109.728151659721,
178.936396372111));
#27699=CARTESIAN_POINT('Ctrl Pts',(-56.5553487544082,-109.726551084934,
178.072094410988));
#27700=CARTESIAN_POINT('Ctrl Pts',(-55.68597872063,-109.724950510147,177.207792449865));
#27701=CARTESIAN_POINT('Ctrl Pts',(-55.6760407085698,-109.63172874007,175.985484945604));
#27702=CARTESIAN_POINT('Ctrl Pts',(-55.6661026965097,-109.538506969993,
174.763177441344));
#27703=CARTESIAN_POINT('Ctrl Pts',(-56.5155966763764,-109.353664007802,
173.89887555255));
#27704=CARTESIAN_POINT('Ctrl Pts',(-57.365090656243,-109.168821045611,173.034573663757));
#27705=CARTESIAN_POINT('Ctrl Pts',(-58.5705729933119,-108.946027346222,
173.034573714903));
#27706=CARTESIAN_POINT('Ctrl Pts',(-59.7760553303807,-108.723233646833,
173.034573766048));
#27707=CARTESIAN_POINT('Ctrl Pts',(-60.6255492383249,-108.53839069231,173.898875727171));
#27708=CARTESIAN_POINT('Ctrl Pts',(-61.4750431462691,-108.353547737786,
174.763177688294));
#27709=CARTESIAN_POINT('Ctrl Pts',(-61.4651050324952,-108.260325978553,
175.985485192554));
#27710=CARTESIAN_POINT('Ctrl Pts',(-61.4551669187214,-108.167104219319,
177.207792696815));
#27711=CARTESIAN_POINT('Ctrl Pts',(-60.5857968130207,-108.165503652199,
178.072094585608));
#27712=CARTESIAN_POINT('Ctrl Pts',(-59.71642670732,-108.163903085079,178.936396474401));
#27713=CARTESIAN_POINT('Ctrl Pts',(-58.4910682444171,-108.200253255158,
178.936396423256));
#27714=CARTESIAN_POINT('Ctrl Pts',(-57.2657097815143,-108.236603425236,
178.936396372111));
#27715=CARTESIAN_POINT('Ctrl Pts',(-56.396339747736,-108.235002850448,178.072094410988));
#27716=CARTESIAN_POINT('Ctrl Pts',(-55.5269697139578,-108.233402275661,
177.207792449865));
#27717=CARTESIAN_POINT('Ctrl Pts',(-55.5170317018976,-108.140180505584,
175.985484945604));
#27718=CARTESIAN_POINT('Ctrl Pts',(-55.5070936898375,-108.046958735507,
174.763177441344));
#27719=CARTESIAN_POINT('Ctrl Pts',(-56.3565876697041,-107.862115773316,
173.89887555255));
#27720=CARTESIAN_POINT('Ctrl Pts',(-57.2060816495708,-107.677272811126,
173.034573663757));
#27721=CARTESIAN_POINT('Ctrl Pts',(-58.4115639866396,-107.454479111736,
173.034573714903));
#27722=CARTESIAN_POINT('Ctrl Pts',(-59.6170463237085,-107.231685412347,
173.034573766048));
#27723=CARTESIAN_POINT('Ctrl Pts',(-60.4665402316527,-107.046842457824,
173.898875727171));
#27724=CARTESIAN_POINT('Ctrl Pts',(-61.3160341395969,-106.861999503301,
174.763177688294));
#27725=CARTESIAN_POINT('Ctrl Pts',(-61.306096025823,-106.768777744067,175.985485192554));
#27726=CARTESIAN_POINT('Ctrl Pts',(-61.2961579120492,-106.675555984834,
177.207792696815));
#27727=CARTESIAN_POINT('Ctrl Pts',(-60.4267878063484,-106.673955417714,
178.072094585608));
#27728=CARTESIAN_POINT('Ctrl Pts',(-59.5574177006478,-106.672354850594,
178.936396474401));
#27729=CARTESIAN_POINT('Ctrl Pts',(-58.3320592377449,-106.708705020672,
178.936396423256));
#27730=CARTESIAN_POINT('Ctrl Pts',(-57.106700774842,-106.74505519075,178.936396372111));
#27731=CARTESIAN_POINT('Ctrl Pts',(-56.2373307410638,-106.743454615963,
178.072094410988));
#27732=CARTESIAN_POINT('Ctrl Pts',(-55.3679607072856,-106.741854041175,
177.207792449865));
#27733=CARTESIAN_POINT('Ctrl Pts',(-55.3580226952254,-106.648632271098,
175.985484945604));
#27734=CARTESIAN_POINT('Ctrl Pts',(-55.3480846831652,-106.555410501021,
174.763177441344));
#27735=CARTESIAN_POINT('Ctrl Pts',(-56.1975786630319,-106.370567538831,
173.89887555255));
#27736=CARTESIAN_POINT('Ctrl Pts',(-57.0470726428986,-106.18572457664,173.034573663757));
#27737=CARTESIAN_POINT('Ctrl Pts',(-58.2525549799674,-105.962930877251,
173.034573714903));
#27738=CARTESIAN_POINT('Ctrl Pts',(-59.4580373170363,-105.740137177862,
173.034573766048));
#27739=CARTESIAN_POINT('Ctrl Pts',(-60.3075312249805,-105.555294223339,
173.898875727171));
#27740=CARTESIAN_POINT('Ctrl Pts',(-61.1570251329247,-105.370451268815,
174.763177688294));
#27741=CARTESIAN_POINT('Ctrl Pts',(-61.1470870191508,-105.277229509582,
175.985485192554));
#27742=CARTESIAN_POINT('Ctrl Pts',(-61.1371489053769,-105.184007750348,
177.207792696815));
#27743=CARTESIAN_POINT('Ctrl Pts',(-60.2677787996762,-105.182407183228,
178.072094585608));
#27744=CARTESIAN_POINT('Ctrl Pts',(-59.3984086939755,-105.180806616108,
178.936396474401));
#27745=CARTESIAN_POINT('Ctrl Pts',(-58.1730502310727,-105.217156786186,
178.936396423256));
#27746=CARTESIAN_POINT('Ctrl Pts',(-56.9476917681698,-105.253506956265,
178.936396372111));
#27747=CARTESIAN_POINT('Ctrl Pts',(-56.0783217343916,-105.251906381477,
178.072094410988));
#27748=CARTESIAN_POINT('Ctrl Pts',(-55.2089517006133,-105.25030580669,177.207792449865));
#27749=CARTESIAN_POINT('Ctrl Pts',(-55.1990136885532,-105.157084036613,
175.985484945604));
#27750=CARTESIAN_POINT('Ctrl Pts',(-55.189075676493,-105.063862266536,174.763177441344));
#27751=CARTESIAN_POINT('Ctrl Pts',(-56.0385696563597,-104.879019304345,
173.89887555255));
#27752=CARTESIAN_POINT('Ctrl Pts',(-56.8880636362264,-104.694176342154,
173.034573663757));
#27753=CARTESIAN_POINT('Ctrl Pts',(-58.0935459732952,-104.471382642765,
173.034573714903));
#27754=CARTESIAN_POINT('Ctrl Pts',(-59.299028310364,-104.248588943376,173.034573766048));
#27755=CARTESIAN_POINT('Ctrl Pts',(-60.1485222183082,-104.063745988853,
173.898875727171));
#27756=CARTESIAN_POINT('Ctrl Pts',(-60.9980161262524,-103.87890303433,174.763177688294));
#27757=CARTESIAN_POINT('Ctrl Pts',(-60.9880780124786,-103.785681275096,
175.985485192554));
#27758=CARTESIAN_POINT('Ctrl Pts',(-60.9781398987047,-103.692459515862,
177.207792696815));
#27759=CARTESIAN_POINT('Ctrl Pts',(-60.108769793004,-103.690858948742,178.072094585608));
#27760=CARTESIAN_POINT('Ctrl Pts',(-59.2393996873033,-103.689258381622,
178.936396474401));
#27761=CARTESIAN_POINT('Ctrl Pts',(-58.0140412244004,-103.725608551701,
178.936396423256));
#27762=CARTESIAN_POINT('Ctrl Pts',(-56.7886827614976,-103.761958721779,
178.936396372111));
#27763=CARTESIAN_POINT('Ctrl Pts',(-55.9193127277193,-103.760358146992,
178.072094410988));
#27764=CARTESIAN_POINT('Ctrl Pts',(-55.0499426939411,-103.758757572204,
177.207792449865));
#27765=CARTESIAN_POINT('Ctrl Pts',(-55.0400046818809,-103.665535802127,
175.985484945604));
#27766=CARTESIAN_POINT('Ctrl Pts',(-55.0300666698208,-103.57231403205,174.763177441344));
#27767=CARTESIAN_POINT('Ctrl Pts',(-55.8795606496874,-103.387471069859,
173.89887555255));
#27768=CARTESIAN_POINT('Ctrl Pts',(-56.7290546295541,-103.202628107669,
173.034573663757));
#27769=CARTESIAN_POINT('Ctrl Pts',(-57.934536966623,-102.97983440828,173.034573714903));
#27770=CARTESIAN_POINT('Ctrl Pts',(-59.1400193036918,-102.757040708891,
173.034573766048));
#27771=CARTESIAN_POINT('Ctrl Pts',(-59.989513211636,-102.572197754367,173.898875727171));
#27772=CARTESIAN_POINT('Ctrl Pts',(-60.8390071195802,-102.387354799844,
174.763177688294));
#27773=CARTESIAN_POINT('Ctrl Pts',(-60.8290690058063,-102.29413304061,175.985485192554));
#27774=CARTESIAN_POINT('Ctrl Pts',(-60.8191308920325,-102.200911281377,
177.207792696815));
#27775=CARTESIAN_POINT('Ctrl Pts',(-59.9497607863318,-102.199310714257,
178.072094585608));
#27776=CARTESIAN_POINT('Ctrl Pts',(-59.0803906806311,-102.197710147137,
178.936396474401));
#27777=CARTESIAN_POINT('Ctrl Pts',(-57.8550322177282,-102.234060317215,
178.936396423256));
#27778=CARTESIAN_POINT('Ctrl Pts',(-56.6296737548253,-102.270410487293,
178.936396372111));
#27779=CARTESIAN_POINT('Ctrl Pts',(-55.7603037210471,-102.268809912506,
178.072094410988));
#27780=CARTESIAN_POINT('Ctrl Pts',(-54.8909336872689,-102.267209337719,
177.207792449865));
#27781=CARTESIAN_POINT('Ctrl Pts',(-54.8809956752087,-102.173987567642,
175.985484945604));
#27782=CARTESIAN_POINT('Ctrl Pts',(-54.8710576631486,-102.080765797565,
174.763177441344));
#27783=CARTESIAN_POINT('Ctrl Pts',(-55.7205516430152,-101.895922835374,
173.89887555255));
#27784=CARTESIAN_POINT('Ctrl Pts',(-56.5700456228819,-101.711079873183,
173.034573663757));
#27785=CARTESIAN_POINT('Ctrl Pts',(-57.7755279599507,-101.488286173794,
173.034573714903));
#27786=CARTESIAN_POINT('Ctrl Pts',(-58.9810102970196,-101.265492474405,
173.034573766048));
#27787=CARTESIAN_POINT('Ctrl Pts',(-59.8305042049638,-101.080649519882,
173.898875727171));
#27788=CARTESIAN_POINT('Ctrl Pts',(-60.679998112908,-100.895806565358,174.763177688294));
#27789=CARTESIAN_POINT('Ctrl Pts',(-60.6700599991341,-100.802584806125,
175.985485192554));
#27790=CARTESIAN_POINT('Ctrl Pts',(-60.6601218853602,-100.709363046891,
177.207792696815));
#27791=CARTESIAN_POINT('Ctrl Pts',(-59.7907517796595,-100.707762479771,
178.072094585608));
#27792=CARTESIAN_POINT('Ctrl Pts',(-58.9213816739588,-100.706161912651,
178.936396474401));
#27793=CARTESIAN_POINT('Ctrl Pts',(-57.696023211056,-100.742512082729,178.936396423256));
#27794=CARTESIAN_POINT('Ctrl Pts',(-56.4706647481531,-100.778862252808,
178.936396372111));
#27795=CARTESIAN_POINT('Ctrl Pts',(-55.6012947143749,-100.77726167802,178.072094410988));
#27796=CARTESIAN_POINT('Ctrl Pts',(-54.7319246805966,-100.775661103233,
177.207792449865));
#27797=CARTESIAN_POINT('Ctrl Pts',(-54.7219866685365,-100.682439333156,
175.985484945604));
#27798=CARTESIAN_POINT('Ctrl Pts',(-54.7120486564763,-100.589217563079,
174.763177441344));
#27799=CARTESIAN_POINT('Ctrl Pts',(-55.561542636343,-100.404374600888,173.89887555255));
#27800=CARTESIAN_POINT('Ctrl Pts',(-56.4110366162097,-100.219531638698,
173.034573663757));
#27801=CARTESIAN_POINT('Ctrl Pts',(-57.6165189532785,-99.9967379393085,
173.034573714903));
#27802=CARTESIAN_POINT('Ctrl Pts',(-58.8220012903473,-99.7739442399195,
173.034573766048));
#27803=CARTESIAN_POINT('Ctrl Pts',(-59.6714951982915,-99.5891012853962,
173.898875727171));
#27804=CARTESIAN_POINT('Ctrl Pts',(-60.5209891062358,-99.4042583308729,
174.763177688294));
#27805=CARTESIAN_POINT('Ctrl Pts',(-60.5110509924619,-99.3110365716392,
175.985485192554));
#27806=CARTESIAN_POINT('Ctrl Pts',(-60.501112878688,-99.2178148124055,177.207792696815));
#27807=CARTESIAN_POINT('Ctrl Pts',(-59.6317427729873,-99.2162142452855,
178.072094585608));
#27808=CARTESIAN_POINT('Ctrl Pts',(-58.7623726672866,-99.2146136781656,
178.936396474401));
#27809=CARTESIAN_POINT('Ctrl Pts',(-57.5370142043838,-99.2509638482439,
178.936396423256));
#27810=CARTESIAN_POINT('Ctrl Pts',(-56.3116557414809,-99.2873140183222,
178.936396372111));
#27811=CARTESIAN_POINT('Ctrl Pts',(-55.4422857077027,-99.2857134435348,
178.072094410988));
#27812=CARTESIAN_POINT('Ctrl Pts',(-54.5729156739244,-99.2841128687474,
177.207792449865));
#27813=CARTESIAN_POINT('Ctrl Pts',(-54.5629776618643,-99.1908910986704,
175.985484945604));
#27814=CARTESIAN_POINT('Ctrl Pts',(-54.5530396498041,-99.0976693285933,
174.763177441344));
#27815=CARTESIAN_POINT('Ctrl Pts',(-55.4025336296708,-98.9128263664026,
173.89887555255));
#27816=CARTESIAN_POINT('Ctrl Pts',(-56.2520276095374,-98.727983404212,173.034573663757));
#27817=CARTESIAN_POINT('Ctrl Pts',(-57.4575099466063,-98.5051897048229,
173.034573714903));
#27818=CARTESIAN_POINT('Ctrl Pts',(-58.6629922836751,-98.2823960054338,
173.034573766048));
#27819=CARTESIAN_POINT('Ctrl Pts',(-59.5124861916193,-98.0975530509106,
173.898875727171));
#27820=CARTESIAN_POINT('Ctrl Pts',(-60.3619800995635,-97.9127100963873,
174.763177688294));
#27821=CARTESIAN_POINT('Ctrl Pts',(-60.3520419857897,-97.8194883371536,
175.985485192554));
#27822=CARTESIAN_POINT('Ctrl Pts',(-60.3421038720158,-97.7262665779199,
177.207792696815));
#27823=CARTESIAN_POINT('Ctrl Pts',(-59.4727337663151,-97.7246660108,178.072094585608));
#27824=CARTESIAN_POINT('Ctrl Pts',(-58.6033636606144,-97.72306544368,178.936396474401));
#27825=CARTESIAN_POINT('Ctrl Pts',(-57.3780051977115,-97.7594156137583,
178.936396423256));
#27826=CARTESIAN_POINT('Ctrl Pts',(-56.1526467348087,-97.7957657838366,
178.936396372111));
#27827=CARTESIAN_POINT('Ctrl Pts',(-55.2832767010304,-97.7941652090492,
178.072094410988));
#27828=CARTESIAN_POINT('Ctrl Pts',(-56.1707931031902,-113.117197303651,
178.813912075476));
#27829=CARTESIAN_POINT('Ctrl Pts',(-54.9958834532485,-113.148169293224,
177.6423391512));
#27830=CARTESIAN_POINT('Ctrl Pts',(-54.9859454592686,-113.05494752122,175.985484901707));
#27831=CARTESIAN_POINT('Ctrl Pts',(-54.9760074652888,-112.961725749215,
174.328630652215));
#27832=CARTESIAN_POINT('Ctrl Pts',(-56.1310410868884,-112.744310219938,
173.157057825983));
#27833=CARTESIAN_POINT('Ctrl Pts',(-57.286074708488,-112.52689469066,171.985484999752));
#27834=CARTESIAN_POINT('Ctrl Pts',(-58.9236553326579,-112.258036427063,
171.985485069079));
#27835=CARTESIAN_POINT('Ctrl Pts',(-60.5612359568277,-111.989178163466,
171.985485138407));
#27836=CARTESIAN_POINT('Ctrl Pts',(-61.7162694809355,-111.771762644582,
173.157058062683));
#27837=CARTESIAN_POINT('Ctrl Pts',(-62.8713030050432,-111.554347125698,
174.328630986959));
#27838=CARTESIAN_POINT('Ctrl Pts',(-62.861364873189,-111.461125368392,175.985485236451));
#27839=CARTESIAN_POINT('Ctrl Pts',(-62.8514267413349,-111.367903611086,
177.642339485944));
#27840=CARTESIAN_POINT('Ctrl Pts',(-61.6765169939012,-111.398875611052,
178.813912312176));
#27841=CARTESIAN_POINT('Ctrl Pts',(-60.5016072464676,-111.429847611019,
179.985485138407));
#27842=CARTESIAN_POINT('Ctrl Pts',(-58.8441504964637,-111.512262345305,
179.985485069079));
#27843=CARTESIAN_POINT('Ctrl Pts',(-57.1866937464598,-111.594677079592,
179.985484999752));
#27844=CARTESIAN_POINT('Ctrl Pts',(-56.011784096518,-111.625649069165,178.813912075476));
#27845=CARTESIAN_POINT('Ctrl Pts',(-54.8368744465762,-111.656621058739,
177.6423391512));
#27846=CARTESIAN_POINT('Ctrl Pts',(-54.8269364525964,-111.563399286734,
175.985484901707));
#27847=CARTESIAN_POINT('Ctrl Pts',(-54.8169984586165,-111.47017751473,174.328630652215));
#27848=CARTESIAN_POINT('Ctrl Pts',(-55.9720320802161,-111.252761985452,
173.157057825983));
#27849=CARTESIAN_POINT('Ctrl Pts',(-57.1270657018158,-111.035346456175,
171.985484999752));
#27850=CARTESIAN_POINT('Ctrl Pts',(-58.7646463259856,-110.766488192578,
171.985485069079));
#27851=CARTESIAN_POINT('Ctrl Pts',(-60.4022269501555,-110.497629928981,
171.985485138407));
#27852=CARTESIAN_POINT('Ctrl Pts',(-61.5572604742632,-110.280214410097,
173.157058062683));
#27853=CARTESIAN_POINT('Ctrl Pts',(-62.712293998371,-110.062798891212,174.328630986959));
#27854=CARTESIAN_POINT('Ctrl Pts',(-62.7023558665168,-109.969577133906,
175.985485236451));
#27855=CARTESIAN_POINT('Ctrl Pts',(-62.6924177346626,-109.8763553766,177.642339485944));
#27856=CARTESIAN_POINT('Ctrl Pts',(-61.517507987229,-109.907327376567,178.813912312176));
#27857=CARTESIAN_POINT('Ctrl Pts',(-60.3425982397954,-109.938299376534,
179.985485138407));
#27858=CARTESIAN_POINT('Ctrl Pts',(-58.6851414897915,-110.02071411082,179.985485069079));
#27859=CARTESIAN_POINT('Ctrl Pts',(-57.0276847397876,-110.103128845106,
179.985484999752));
#27860=CARTESIAN_POINT('Ctrl Pts',(-55.8527750898458,-110.13410083468,178.813912075476));
#27861=CARTESIAN_POINT('Ctrl Pts',(-54.677865439904,-110.165072824253,177.6423391512));
#27862=CARTESIAN_POINT('Ctrl Pts',(-54.6679274459242,-110.071851052249,
175.985484901707));
#27863=CARTESIAN_POINT('Ctrl Pts',(-54.6579894519443,-109.978629280244,
174.328630652215));
#27864=CARTESIAN_POINT('Ctrl Pts',(-55.8130230735439,-109.761213750967,
173.157057825983));
#27865=CARTESIAN_POINT('Ctrl Pts',(-56.9680566951435,-109.543798221689,
171.985484999752));
#27866=CARTESIAN_POINT('Ctrl Pts',(-58.6056373193134,-109.274939958092,
171.985485069079));
#27867=CARTESIAN_POINT('Ctrl Pts',(-60.2432179434833,-109.006081694495,
171.985485138407));
#27868=CARTESIAN_POINT('Ctrl Pts',(-61.398251467591,-108.788666175611,173.157058062683));
#27869=CARTESIAN_POINT('Ctrl Pts',(-62.5532849916988,-108.571250656727,
174.328630986959));
#27870=CARTESIAN_POINT('Ctrl Pts',(-62.5433468598446,-108.478028899421,
175.985485236451));
#27871=CARTESIAN_POINT('Ctrl Pts',(-62.5334087279904,-108.384807142114,
177.642339485944));
#27872=CARTESIAN_POINT('Ctrl Pts',(-61.3584989805568,-108.415779142081,
178.813912312176));
#27873=CARTESIAN_POINT('Ctrl Pts',(-60.1835892331231,-108.446751142048,
179.985485138407));
#27874=CARTESIAN_POINT('Ctrl Pts',(-58.5261324831192,-108.529165876334,
179.985485069079));
#27875=CARTESIAN_POINT('Ctrl Pts',(-56.8686757331153,-108.611580610621,
179.985484999752));
#27876=CARTESIAN_POINT('Ctrl Pts',(-55.6937660831736,-108.642552600194,
178.813912075476));
#27877=CARTESIAN_POINT('Ctrl Pts',(-54.5188564332318,-108.673524589768,
177.6423391512));
#27878=CARTESIAN_POINT('Ctrl Pts',(-54.5089184392519,-108.580302817763,
175.985484901707));
#27879=CARTESIAN_POINT('Ctrl Pts',(-54.4989804452721,-108.487081045759,
174.328630652215));
#27880=CARTESIAN_POINT('Ctrl Pts',(-55.6540140668717,-108.269665516481,
173.157057825983));
#27881=CARTESIAN_POINT('Ctrl Pts',(-56.8090476884713,-108.052249987204,
171.985484999752));
#27882=CARTESIAN_POINT('Ctrl Pts',(-58.4466283126412,-107.783391723607,
171.985485069079));
#27883=CARTESIAN_POINT('Ctrl Pts',(-60.084208936811,-107.51453346001,171.985485138407));
#27884=CARTESIAN_POINT('Ctrl Pts',(-61.2392424609188,-107.297117941125,
173.157058062683));
#27885=CARTESIAN_POINT('Ctrl Pts',(-62.3942759850265,-107.079702422241,
174.328630986959));
#27886=CARTESIAN_POINT('Ctrl Pts',(-62.3843378531723,-106.986480664935,
175.985485236451));
#27887=CARTESIAN_POINT('Ctrl Pts',(-62.3743997213182,-106.893258907629,
177.642339485944));
#27888=CARTESIAN_POINT('Ctrl Pts',(-61.1994899738845,-106.924230907596,
178.813912312176));
#27889=CARTESIAN_POINT('Ctrl Pts',(-60.0245802264509,-106.955202907562,
179.985485138407));
#27890=CARTESIAN_POINT('Ctrl Pts',(-58.367123476447,-107.037617641849,179.985485069079));
#27891=CARTESIAN_POINT('Ctrl Pts',(-56.7096667264431,-107.120032376135,
179.985484999752));
#27892=CARTESIAN_POINT('Ctrl Pts',(-55.5347570765013,-107.151004365708,
178.813912075476));
#27893=CARTESIAN_POINT('Ctrl Pts',(-54.3598474265596,-107.181976355282,
177.6423391512));
#27894=CARTESIAN_POINT('Ctrl Pts',(-54.3499094325797,-107.088754583277,
175.985484901707));
#27895=CARTESIAN_POINT('Ctrl Pts',(-54.3399714385998,-106.995532811273,
174.328630652215));
#27896=CARTESIAN_POINT('Ctrl Pts',(-55.4950050601995,-106.778117281995,
173.157057825983));
#27897=CARTESIAN_POINT('Ctrl Pts',(-56.6500386817991,-106.560701752718,
171.985484999752));
#27898=CARTESIAN_POINT('Ctrl Pts',(-58.2876193059689,-106.291843489121,
171.985485069079));
#27899=CARTESIAN_POINT('Ctrl Pts',(-59.9251999301388,-106.022985225524,
171.985485138407));
#27900=CARTESIAN_POINT('Ctrl Pts',(-61.0802334542465,-105.80556970664,173.157058062683));
#27901=CARTESIAN_POINT('Ctrl Pts',(-62.2352669783543,-105.588154187756,
174.328630986959));
#27902=CARTESIAN_POINT('Ctrl Pts',(-62.2253288465001,-105.494932430449,
175.985485236451));
#27903=CARTESIAN_POINT('Ctrl Pts',(-62.2153907146459,-105.401710673143,
177.642339485944));
#27904=CARTESIAN_POINT('Ctrl Pts',(-61.0404809672123,-105.43268267311,178.813912312176));
#27905=CARTESIAN_POINT('Ctrl Pts',(-59.8655712197787,-105.463654673077,
179.985485138407));
#27906=CARTESIAN_POINT('Ctrl Pts',(-58.2081144697748,-105.546069407363,
179.985485069079));
#27907=CARTESIAN_POINT('Ctrl Pts',(-56.5506577197709,-105.628484141649,
179.985484999752));
#27908=CARTESIAN_POINT('Ctrl Pts',(-55.3757480698291,-105.659456131223,
178.813912075476));
#27909=CARTESIAN_POINT('Ctrl Pts',(-54.2008384198873,-105.690428120796,
177.6423391512));
#27910=CARTESIAN_POINT('Ctrl Pts',(-54.1909004259075,-105.597206348792,
175.985484901707));
#27911=CARTESIAN_POINT('Ctrl Pts',(-54.1809624319276,-105.503984576787,
174.328630652215));
#27912=CARTESIAN_POINT('Ctrl Pts',(-55.3359960535272,-105.28656904751,173.157057825983));
#27913=CARTESIAN_POINT('Ctrl Pts',(-56.4910296751268,-105.069153518232,
171.985484999752));
#27914=CARTESIAN_POINT('Ctrl Pts',(-58.1286102992967,-104.800295254635,
171.985485069079));
#27915=CARTESIAN_POINT('Ctrl Pts',(-59.7661909234666,-104.531436991038,
171.985485138407));
#27916=CARTESIAN_POINT('Ctrl Pts',(-60.9212244475743,-104.314021472154,
173.157058062683));
#27917=CARTESIAN_POINT('Ctrl Pts',(-62.0762579716821,-104.09660595327,174.328630986959));
#27918=CARTESIAN_POINT('Ctrl Pts',(-62.0663198398279,-104.003384195964,
175.985485236451));
#27919=CARTESIAN_POINT('Ctrl Pts',(-62.0563817079737,-103.910162438658,
177.642339485944));
#27920=CARTESIAN_POINT('Ctrl Pts',(-60.8814719605401,-103.941134438624,
178.813912312176));
#27921=CARTESIAN_POINT('Ctrl Pts',(-59.7065622131064,-103.972106438591,
179.985485138407));
#27922=CARTESIAN_POINT('Ctrl Pts',(-58.0491054631025,-104.054521172878,
179.985485069079));
#27923=CARTESIAN_POINT('Ctrl Pts',(-56.3916487130987,-104.136935907164,
179.985484999752));
#27924=CARTESIAN_POINT('Ctrl Pts',(-55.2167390631569,-104.167907896737,
178.813912075476));
#27925=CARTESIAN_POINT('Ctrl Pts',(-54.0418294132151,-104.198879886311,
177.6423391512));
#27926=CARTESIAN_POINT('Ctrl Pts',(-54.0318914192353,-104.105658114306,
175.985484901707));
#27927=CARTESIAN_POINT('Ctrl Pts',(-54.0219534252554,-104.012436342302,
174.328630652215));
#27928=CARTESIAN_POINT('Ctrl Pts',(-55.176987046855,-103.795020813024,173.157057825983));
#27929=CARTESIAN_POINT('Ctrl Pts',(-56.3320206684546,-103.577605283747,
171.985484999752));
#27930=CARTESIAN_POINT('Ctrl Pts',(-57.9696012926245,-103.30874702015,171.985485069079));
#27931=CARTESIAN_POINT('Ctrl Pts',(-59.6071819167943,-103.039888756553,
171.985485138407));
#27932=CARTESIAN_POINT('Ctrl Pts',(-60.7622154409021,-102.822473237669,
173.157058062683));
#27933=CARTESIAN_POINT('Ctrl Pts',(-61.9172489650099,-102.605057718784,
174.328630986959));
#27934=CARTESIAN_POINT('Ctrl Pts',(-61.9073108331557,-102.511835961478,
175.985485236451));
#27935=CARTESIAN_POINT('Ctrl Pts',(-61.8973727013015,-102.418614204172,
177.642339485944));
#27936=CARTESIAN_POINT('Ctrl Pts',(-60.7224629538678,-102.449586204139,
178.813912312176));
#27937=CARTESIAN_POINT('Ctrl Pts',(-59.5475532064342,-102.480558204106,
179.985485138407));
#27938=CARTESIAN_POINT('Ctrl Pts',(-57.8900964564303,-102.562972938392,
179.985485069079));
#27939=CARTESIAN_POINT('Ctrl Pts',(-56.2326397064264,-102.645387672678,
179.985484999752));
#27940=CARTESIAN_POINT('Ctrl Pts',(-55.0577300564847,-102.676359662252,
178.813912075476));
#27941=CARTESIAN_POINT('Ctrl Pts',(-53.8828204065429,-102.707331651825,
177.6423391512));
#27942=CARTESIAN_POINT('Ctrl Pts',(-53.872882412563,-102.614109879821,175.985484901707));
#27943=CARTESIAN_POINT('Ctrl Pts',(-53.8629444185832,-102.520888107816,
174.328630652215));
#27944=CARTESIAN_POINT('Ctrl Pts',(-55.0179780401828,-102.303472578539,
173.157057825983));
#27945=CARTESIAN_POINT('Ctrl Pts',(-56.1730116617824,-102.086057049261,
171.985484999752));
#27946=CARTESIAN_POINT('Ctrl Pts',(-57.8105922859523,-101.817198785664,
171.985485069079));
#27947=CARTESIAN_POINT('Ctrl Pts',(-59.4481729101221,-101.548340522067,
171.985485138407));
#27948=CARTESIAN_POINT('Ctrl Pts',(-60.6032064342299,-101.330925003183,
173.157058062683));
#27949=CARTESIAN_POINT('Ctrl Pts',(-61.7582399583376,-101.113509484299,
174.328630986959));
#27950=CARTESIAN_POINT('Ctrl Pts',(-61.7483018264834,-101.020287726993,
175.985485236451));
#27951=CARTESIAN_POINT('Ctrl Pts',(-61.7383636946293,-100.927065969686,
177.642339485944));
#27952=CARTESIAN_POINT('Ctrl Pts',(-60.5634539471956,-100.958037969653,
178.813912312176));
#27953=CARTESIAN_POINT('Ctrl Pts',(-59.388544199762,-100.98900996962,179.985485138407));
#27954=CARTESIAN_POINT('Ctrl Pts',(-57.7310874497581,-101.071424703906,
179.985485069079));
#27955=CARTESIAN_POINT('Ctrl Pts',(-56.0736306997542,-101.153839438193,
179.985484999752));
#27956=CARTESIAN_POINT('Ctrl Pts',(-54.8987210498124,-101.184811427766,
178.813912075476));
#27957=CARTESIAN_POINT('Ctrl Pts',(-53.7238113998707,-101.21578341734,177.6423391512));
#27958=CARTESIAN_POINT('Ctrl Pts',(-53.7138734058908,-101.122561645335,
175.985484901707));
#27959=CARTESIAN_POINT('Ctrl Pts',(-53.7039354119109,-101.029339873331,
174.328630652215));
#27960=CARTESIAN_POINT('Ctrl Pts',(-54.8589690335105,-100.811924344053,
173.157057825983));
#27961=CARTESIAN_POINT('Ctrl Pts',(-56.0140026551102,-100.594508814776,
171.985484999752));
#27962=CARTESIAN_POINT('Ctrl Pts',(-57.65158327928,-100.325650551179,171.985485069079));
#27963=CARTESIAN_POINT('Ctrl Pts',(-59.2891639034499,-100.056792287582,
171.985485138407));
#27964=CARTESIAN_POINT('Ctrl Pts',(-60.4441974275576,-99.8393767686974,
173.157058062683));
#27965=CARTESIAN_POINT('Ctrl Pts',(-61.5992309516654,-99.6219612498133,
174.328630986959));
#27966=CARTESIAN_POINT('Ctrl Pts',(-61.5892928198112,-99.528739492507,175.985485236451));
#27967=CARTESIAN_POINT('Ctrl Pts',(-61.579354687957,-99.4355177352008,177.642339485944));
#27968=CARTESIAN_POINT('Ctrl Pts',(-60.4044449405234,-99.4664897351676,
178.813912312176));
#27969=CARTESIAN_POINT('Ctrl Pts',(-59.2295351930898,-99.4974617351344,
179.985485138407));
#27970=CARTESIAN_POINT('Ctrl Pts',(-57.5720784430859,-99.5798764694207,
179.985485069079));
#27971=CARTESIAN_POINT('Ctrl Pts',(-55.914621693082,-99.662291203707,179.985484999752));
#27972=CARTESIAN_POINT('Ctrl Pts',(-54.7397120431402,-99.6932631932805,
178.813912075476));
#27973=CARTESIAN_POINT('Ctrl Pts',(-53.5648023931984,-99.724235182854,177.6423391512));
#27974=CARTESIAN_POINT('Ctrl Pts',(-53.5548643992186,-99.6310134108495,
175.985484901707));
#27975=CARTESIAN_POINT('Ctrl Pts',(-53.5449264052387,-99.5377916388449,
174.328630652215));
#27976=CARTESIAN_POINT('Ctrl Pts',(-54.6999600268383,-99.3203761095675,
173.157057825983));
#27977=CARTESIAN_POINT('Ctrl Pts',(-55.8549936484379,-99.10296058029,171.985484999752));
#27978=CARTESIAN_POINT('Ctrl Pts',(-57.4925742726078,-98.834102316693,171.985485069079));
#27979=CARTESIAN_POINT('Ctrl Pts',(-59.1301548967777,-98.565244053096,171.985485138407));
#27980=CARTESIAN_POINT('Ctrl Pts',(-60.2851884208854,-98.3478285342118,
173.157058062683));
#27981=CARTESIAN_POINT('Ctrl Pts',(-61.4402219449932,-98.1304130153276,
174.328630986959));
#27982=CARTESIAN_POINT('Ctrl Pts',(-61.430283813139,-98.0371912580215,175.985485236451));
#27983=CARTESIAN_POINT('Ctrl Pts',(-61.4203456812848,-97.9439695007152,
177.642339485944));
#27984=CARTESIAN_POINT('Ctrl Pts',(-60.2454359338512,-97.974941500682,178.813912312176));
#27985=CARTESIAN_POINT('Ctrl Pts',(-59.0705261864175,-98.0059135006488,
179.985485138407));
#27986=CARTESIAN_POINT('Ctrl Pts',(-57.4130694364136,-98.0883282349351,
179.985485069079));
#27987=CARTESIAN_POINT('Ctrl Pts',(-55.7556126864097,-98.1707429692214,
179.985484999752));
#27988=CARTESIAN_POINT('Ctrl Pts',(-54.580703036468,-98.2017149587949,178.813912075476));
#27989=CARTESIAN_POINT('Ctrl Pts',(-61.4946055979174,-106.918389721436,
178.485485069079));
#27990=CARTESIAN_POINT('Ctrl Pts',(-61.3560333935607,-106.920104239314,
178.657813499464));
#27991=CARTESIAN_POINT('Ctrl Pts',(-61.1994899738845,-106.924230907596,
178.813912312176));
#27992=CARTESIAN_POINT('Ctrl Pts',(-60.0245802264509,-106.955202907562,
179.985485138407));
#27993=CARTESIAN_POINT('Ctrl Pts',(-58.367123476447,-107.037617641849,179.985485069079));
#27994=CARTESIAN_POINT('Ctrl Pts',(-56.7096667264431,-107.120032376135,
179.985484999752));
#27995=CARTESIAN_POINT('Ctrl Pts',(-55.5347570765013,-107.151004365708,
178.813912075476));
#27996=CARTESIAN_POINT('Ctrl Pts',(-54.3598474265596,-107.181976355282,
177.6423391512));
#27997=CARTESIAN_POINT('Ctrl Pts',(-54.3499094325797,-107.088754583277,
175.985484901707));
#27998=CARTESIAN_POINT('Ctrl Pts',(-54.3399714385999,-106.995532811273,
174.328630652215));
#27999=CARTESIAN_POINT('Ctrl Pts',(-55.4950050601995,-106.778117281995,
173.157057825983));
#28000=CARTESIAN_POINT('Ctrl Pts',(-56.6500386817991,-106.560701752718,
171.985484999752));
#28001=CARTESIAN_POINT('Ctrl Pts',(-58.2876193059689,-106.291843489121,
171.985485069079));
#28002=CARTESIAN_POINT('Ctrl Pts',(-59.9251999301388,-106.022985225524,
171.985485138407));
#28003=CARTESIAN_POINT('Ctrl Pts',(-61.0802334542465,-105.80556970664,173.157058062683));
#28004=CARTESIAN_POINT('Ctrl Pts',(-61.2341284751997,-105.776601572697,
173.313156769748));
#28005=CARTESIAN_POINT('Ctrl Pts',(-61.3699476791705,-105.749064143515,
173.485485069079));
#28006=CARTESIAN_POINT('Ctrl Pts',(-56.1707931031902,-113.117197303651,
178.813912075476));
#28007=CARTESIAN_POINT('Ctrl Pts',(-54.9958834532485,-113.148169293224,
177.6423391512));
#28008=CARTESIAN_POINT('Ctrl Pts',(-54.9859454592686,-113.05494752122,175.985484901707));
#28009=CARTESIAN_POINT('Ctrl Pts',(-54.9760074652888,-112.961725749215,
174.328630652215));
#28010=CARTESIAN_POINT('Ctrl Pts',(-56.1310410868884,-112.744310219938,
173.157057825983));
#28011=CARTESIAN_POINT('Ctrl Pts',(-57.286074708488,-112.52689469066,171.985484999752));
#28012=CARTESIAN_POINT('Ctrl Pts',(-58.9236553326578,-112.258036427063,
171.985485069079));
#28013=CARTESIAN_POINT('Ctrl Pts',(-60.5612359568277,-111.989178163466,
171.985485138407));
#28014=CARTESIAN_POINT('Ctrl Pts',(-61.7162694809355,-111.771762644582,
173.157058062683));
#28015=CARTESIAN_POINT('Ctrl Pts',(-62.8713030050432,-111.554347125698,
174.328630986959));
#28016=CARTESIAN_POINT('Ctrl Pts',(-62.861364873189,-111.461125368392,175.985485236451));
#28017=CARTESIAN_POINT('Ctrl Pts',(-62.8514267413349,-111.367903611086,
177.642339485944));
#28018=CARTESIAN_POINT('Ctrl Pts',(-61.6765169939012,-111.398875611052,
178.813912312176));
#28019=CARTESIAN_POINT('Ctrl Pts',(-60.5016072464676,-111.429847611019,
179.985485138407));
#28020=CARTESIAN_POINT('Ctrl Pts',(-58.8441504964637,-111.512262345305,
179.985485069079));
#28021=CARTESIAN_POINT('Ctrl Pts',(-57.1866937464598,-111.594677079592,
179.985484999752));
#28022=CARTESIAN_POINT('Ctrl Pts',(-56.011784096518,-111.625649069165,178.813912075476));
#28023=CARTESIAN_POINT('Ctrl Pts',(-54.8368744465763,-111.656621058739,
177.6423391512));
#28024=CARTESIAN_POINT('Ctrl Pts',(-54.8269364525964,-111.563399286734,
175.985484901707));
#28025=CARTESIAN_POINT('Ctrl Pts',(-54.8169984586165,-111.47017751473,174.328630652215));
#28026=CARTESIAN_POINT('Ctrl Pts',(-55.9720320802161,-111.252761985452,
173.157057825983));
#28027=CARTESIAN_POINT('Ctrl Pts',(-57.1270657018158,-111.035346456175,
171.985484999752));
#28028=CARTESIAN_POINT('Ctrl Pts',(-58.7646463259856,-110.766488192578,
171.985485069079));
#28029=CARTESIAN_POINT('Ctrl Pts',(-60.4022269501555,-110.497629928981,
171.985485138407));
#28030=CARTESIAN_POINT('Ctrl Pts',(-61.5572604742632,-110.280214410097,
173.157058062683));
#28031=CARTESIAN_POINT('Ctrl Pts',(-62.712293998371,-110.062798891212,174.328630986959));
#28032=CARTESIAN_POINT('Ctrl Pts',(-62.7023558665168,-109.969577133906,
175.985485236451));
#28033=CARTESIAN_POINT('Ctrl Pts',(-62.6924177346626,-109.8763553766,177.642339485944));
#28034=CARTESIAN_POINT('Ctrl Pts',(-61.517507987229,-109.907327376567,178.813912312176));
#28035=CARTESIAN_POINT('Ctrl Pts',(-60.3425982397954,-109.938299376534,
179.985485138407));
#28036=CARTESIAN_POINT('Ctrl Pts',(-58.6851414897915,-110.02071411082,179.985485069079));
#28037=CARTESIAN_POINT('Ctrl Pts',(-57.0276847397876,-110.103128845106,
179.985484999752));
#28038=CARTESIAN_POINT('Ctrl Pts',(-55.8527750898458,-110.13410083468,178.813912075476));
#28039=CARTESIAN_POINT('Ctrl Pts',(-54.677865439904,-110.165072824253,177.6423391512));
#28040=CARTESIAN_POINT('Ctrl Pts',(-54.6679274459242,-110.071851052249,
175.985484901707));
#28041=CARTESIAN_POINT('Ctrl Pts',(-54.6579894519443,-109.978629280244,
174.328630652215));
#28042=CARTESIAN_POINT('Ctrl Pts',(-55.8130230735439,-109.761213750967,
173.157057825983));
#28043=CARTESIAN_POINT('Ctrl Pts',(-56.9680566951435,-109.543798221689,
171.985484999752));
#28044=CARTESIAN_POINT('Ctrl Pts',(-58.6056373193134,-109.274939958092,
171.985485069079));
#28045=CARTESIAN_POINT('Ctrl Pts',(-60.2432179434833,-109.006081694495,
171.985485138407));
#28046=CARTESIAN_POINT('Ctrl Pts',(-61.398251467591,-108.788666175611,173.157058062683));
#28047=CARTESIAN_POINT('Ctrl Pts',(-62.5532849916988,-108.571250656727,
174.328630986959));
#28048=CARTESIAN_POINT('Ctrl Pts',(-62.5433468598446,-108.478028899421,
175.985485236451));
#28049=CARTESIAN_POINT('Ctrl Pts',(-62.5334087279904,-108.384807142114,
177.642339485944));
#28050=CARTESIAN_POINT('Ctrl Pts',(-61.3584989805568,-108.415779142081,
178.813912312176));
#28051=CARTESIAN_POINT('Ctrl Pts',(-60.1835892331231,-108.446751142048,
179.985485138407));
#28052=CARTESIAN_POINT('Ctrl Pts',(-58.5261324831192,-108.529165876334,
179.985485069079));
#28053=CARTESIAN_POINT('Ctrl Pts',(-56.8686757331153,-108.611580610621,
179.985484999752));
#28054=CARTESIAN_POINT('Ctrl Pts',(-55.6937660831736,-108.642552600194,
178.813912075476));
#28055=CARTESIAN_POINT('Ctrl Pts',(-54.5188564332318,-108.673524589768,
177.6423391512));
#28056=CARTESIAN_POINT('Ctrl Pts',(-54.5089184392519,-108.580302817763,
175.985484901707));
#28057=CARTESIAN_POINT('Ctrl Pts',(-54.4989804452721,-108.487081045759,
174.328630652215));
#28058=CARTESIAN_POINT('Ctrl Pts',(-55.6540140668717,-108.269665516481,
173.157057825983));
#28059=CARTESIAN_POINT('Ctrl Pts',(-56.8090476884713,-108.052249987204,
171.985484999752));
#28060=CARTESIAN_POINT('Ctrl Pts',(-58.4466283126412,-107.783391723607,
171.985485069079));
#28061=CARTESIAN_POINT('Ctrl Pts',(-60.084208936811,-107.51453346001,171.985485138407));
#28062=CARTESIAN_POINT('Ctrl Pts',(-61.2392424609188,-107.297117941125,
173.157058062683));
#28063=CARTESIAN_POINT('Ctrl Pts',(-62.3942759850265,-107.079702422241,
174.328630986959));
#28064=CARTESIAN_POINT('Ctrl Pts',(-62.3843378531723,-106.986480664935,
175.985485236451));
#28065=CARTESIAN_POINT('Ctrl Pts',(-62.3743997213182,-106.893258907629,
177.642339485944));
#28066=CARTESIAN_POINT('Ctrl Pts',(-61.1994899738845,-106.924230907596,
178.813912312176));
#28067=CARTESIAN_POINT('Ctrl Pts',(-60.0245802264509,-106.955202907562,
179.985485138407));
#28068=CARTESIAN_POINT('Ctrl Pts',(-58.367123476447,-107.037617641849,179.985485069079));
#28069=CARTESIAN_POINT('Ctrl Pts',(-56.7096667264431,-107.120032376135,
179.985484999752));
#28070=CARTESIAN_POINT('Ctrl Pts',(-55.5347570765013,-107.151004365708,
178.813912075476));
#28071=CARTESIAN_POINT('Ctrl Pts',(-54.3598474265596,-107.181976355282,
177.6423391512));
#28072=CARTESIAN_POINT('Ctrl Pts',(-54.3499094325797,-107.088754583277,
175.985484901707));
#28073=CARTESIAN_POINT('Ctrl Pts',(-54.3399714385998,-106.995532811273,
174.328630652215));
#28074=CARTESIAN_POINT('Ctrl Pts',(-55.4950050601995,-106.778117281995,
173.157057825983));
#28075=CARTESIAN_POINT('Ctrl Pts',(-56.6500386817991,-106.560701752718,
171.985484999752));
#28076=CARTESIAN_POINT('Ctrl Pts',(-58.2876193059689,-106.291843489121,
171.985485069079));
#28077=CARTESIAN_POINT('Ctrl Pts',(-59.9251999301388,-106.022985225524,
171.985485138407));
#28078=CARTESIAN_POINT('Ctrl Pts',(-61.0802334542465,-105.80556970664,173.157058062683));
#28079=CARTESIAN_POINT('Ctrl Pts',(-62.2352669783543,-105.588154187756,
174.328630986959));
#28080=CARTESIAN_POINT('Ctrl Pts',(-62.2253288465001,-105.494932430449,
175.985485236451));
#28081=CARTESIAN_POINT('Ctrl Pts',(-62.2153907146459,-105.401710673143,
177.642339485944));
#28082=CARTESIAN_POINT('Ctrl Pts',(-61.0404809672123,-105.43268267311,178.813912312176));
#28083=CARTESIAN_POINT('Ctrl Pts',(-59.8655712197787,-105.463654673077,
179.985485138407));
#28084=CARTESIAN_POINT('Ctrl Pts',(-58.2081144697748,-105.546069407363,
179.985485069079));
#28085=CARTESIAN_POINT('Ctrl Pts',(-56.5506577197709,-105.628484141649,
179.985484999752));
#28086=CARTESIAN_POINT('Ctrl Pts',(-55.3757480698291,-105.659456131223,
178.813912075476));
#28087=CARTESIAN_POINT('Ctrl Pts',(-54.2008384198873,-105.690428120796,
177.6423391512));
#28088=CARTESIAN_POINT('Ctrl Pts',(-54.1909004259075,-105.597206348792,
175.985484901707));
#28089=CARTESIAN_POINT('Ctrl Pts',(-54.1809624319276,-105.503984576787,
174.328630652215));
#28090=CARTESIAN_POINT('Ctrl Pts',(-55.3359960535272,-105.28656904751,173.157057825983));
#28091=CARTESIAN_POINT('Ctrl Pts',(-56.4910296751268,-105.069153518232,
171.985484999752));
#28092=CARTESIAN_POINT('Ctrl Pts',(-58.1286102992967,-104.800295254635,
171.985485069079));
#28093=CARTESIAN_POINT('Ctrl Pts',(-59.7661909234666,-104.531436991038,
171.985485138407));
#28094=CARTESIAN_POINT('Ctrl Pts',(-60.9212244475743,-104.314021472154,
173.157058062683));
#28095=CARTESIAN_POINT('Ctrl Pts',(-62.0762579716821,-104.09660595327,174.328630986959));
#28096=CARTESIAN_POINT('Ctrl Pts',(-62.0663198398279,-104.003384195964,
175.985485236451));
#28097=CARTESIAN_POINT('Ctrl Pts',(-62.0563817079737,-103.910162438658,
177.642339485944));
#28098=CARTESIAN_POINT('Ctrl Pts',(-60.8814719605401,-103.941134438624,
178.813912312176));
#28099=CARTESIAN_POINT('Ctrl Pts',(-59.7065622131064,-103.972106438591,
179.985485138407));
#28100=CARTESIAN_POINT('Ctrl Pts',(-58.0491054631025,-104.054521172878,
179.985485069079));
#28101=CARTESIAN_POINT('Ctrl Pts',(-56.3916487130987,-104.136935907164,
179.985484999752));
#28102=CARTESIAN_POINT('Ctrl Pts',(-55.2167390631569,-104.167907896737,
178.813912075476));
#28103=CARTESIAN_POINT('Ctrl Pts',(-54.0418294132151,-104.198879886311,
177.6423391512));
#28104=CARTESIAN_POINT('Ctrl Pts',(-54.0318914192353,-104.105658114306,
175.985484901707));
#28105=CARTESIAN_POINT('Ctrl Pts',(-54.0219534252554,-104.012436342302,
174.328630652215));
#28106=CARTESIAN_POINT('Ctrl Pts',(-55.176987046855,-103.795020813024,173.157057825983));
#28107=CARTESIAN_POINT('Ctrl Pts',(-56.3320206684546,-103.577605283747,
171.985484999752));
#28108=CARTESIAN_POINT('Ctrl Pts',(-57.9696012926245,-103.30874702015,171.985485069079));
#28109=CARTESIAN_POINT('Ctrl Pts',(-59.6071819167943,-103.039888756553,
171.985485138407));
#28110=CARTESIAN_POINT('Ctrl Pts',(-60.7622154409021,-102.822473237669,
173.157058062683));
#28111=CARTESIAN_POINT('Ctrl Pts',(-61.9172489650099,-102.605057718784,
174.328630986959));
#28112=CARTESIAN_POINT('Ctrl Pts',(-61.9073108331557,-102.511835961478,
175.985485236451));
#28113=CARTESIAN_POINT('Ctrl Pts',(-61.8973727013015,-102.418614204172,
177.642339485944));
#28114=CARTESIAN_POINT('Ctrl Pts',(-60.7224629538678,-102.449586204139,
178.813912312176));
#28115=CARTESIAN_POINT('Ctrl Pts',(-59.5475532064342,-102.480558204106,
179.985485138407));
#28116=CARTESIAN_POINT('Ctrl Pts',(-57.8900964564303,-102.562972938392,
179.985485069079));
#28117=CARTESIAN_POINT('Ctrl Pts',(-56.2326397064264,-102.645387672678,
179.985484999752));
#28118=CARTESIAN_POINT('Ctrl Pts',(-55.0577300564847,-102.676359662252,
178.813912075476));
#28119=CARTESIAN_POINT('Ctrl Pts',(-53.8828204065429,-102.707331651825,
177.6423391512));
#28120=CARTESIAN_POINT('Ctrl Pts',(-53.872882412563,-102.614109879821,175.985484901707));
#28121=CARTESIAN_POINT('Ctrl Pts',(-53.8629444185832,-102.520888107816,
174.328630652215));
#28122=CARTESIAN_POINT('Ctrl Pts',(-55.0179780401828,-102.303472578539,
173.157057825983));
#28123=CARTESIAN_POINT('Ctrl Pts',(-56.1730116617824,-102.086057049261,
171.985484999752));
#28124=CARTESIAN_POINT('Ctrl Pts',(-57.8105922859523,-101.817198785664,
171.985485069079));
#28125=CARTESIAN_POINT('Ctrl Pts',(-59.4481729101221,-101.548340522067,
171.985485138407));
#28126=CARTESIAN_POINT('Ctrl Pts',(-60.6032064342299,-101.330925003183,
173.157058062683));
#28127=CARTESIAN_POINT('Ctrl Pts',(-61.7582399583376,-101.113509484299,
174.328630986959));
#28128=CARTESIAN_POINT('Ctrl Pts',(-61.7483018264834,-101.020287726993,
175.985485236451));
#28129=CARTESIAN_POINT('Ctrl Pts',(-61.7383636946293,-100.927065969686,
177.642339485944));
#28130=CARTESIAN_POINT('Ctrl Pts',(-60.5634539471956,-100.958037969653,
178.813912312176));
#28131=CARTESIAN_POINT('Ctrl Pts',(-59.388544199762,-100.98900996962,179.985485138407));
#28132=CARTESIAN_POINT('Ctrl Pts',(-57.7310874497581,-101.071424703906,
179.985485069079));
#28133=CARTESIAN_POINT('Ctrl Pts',(-56.0736306997542,-101.153839438193,
179.985484999752));
#28134=CARTESIAN_POINT('Ctrl Pts',(-54.8987210498124,-101.184811427766,
178.813912075476));
#28135=CARTESIAN_POINT('Ctrl Pts',(-53.7238113998707,-101.21578341734,177.6423391512));
#28136=CARTESIAN_POINT('Ctrl Pts',(-53.7138734058908,-101.122561645335,
175.985484901707));
#28137=CARTESIAN_POINT('Ctrl Pts',(-53.7039354119109,-101.029339873331,
174.328630652215));
#28138=CARTESIAN_POINT('Ctrl Pts',(-54.8589690335105,-100.811924344053,
173.157057825983));
#28139=CARTESIAN_POINT('Ctrl Pts',(-56.0140026551102,-100.594508814776,
171.985484999752));
#28140=CARTESIAN_POINT('Ctrl Pts',(-57.65158327928,-100.325650551179,171.985485069079));
#28141=CARTESIAN_POINT('Ctrl Pts',(-59.2891639034499,-100.056792287582,
171.985485138407));
#28142=CARTESIAN_POINT('Ctrl Pts',(-60.4441974275576,-99.8393767686974,
173.157058062683));
#28143=CARTESIAN_POINT('Ctrl Pts',(-61.5992309516654,-99.6219612498133,
174.328630986959));
#28144=CARTESIAN_POINT('Ctrl Pts',(-61.5892928198112,-99.528739492507,175.985485236451));
#28145=CARTESIAN_POINT('Ctrl Pts',(-61.579354687957,-99.4355177352008,177.642339485944));
#28146=CARTESIAN_POINT('Ctrl Pts',(-60.4044449405234,-99.4664897351676,
178.813912312176));
#28147=CARTESIAN_POINT('Ctrl Pts',(-59.2295351930898,-99.4974617351344,
179.985485138407));
#28148=CARTESIAN_POINT('Ctrl Pts',(-57.5720784430859,-99.5798764694207,
179.985485069079));
#28149=CARTESIAN_POINT('Ctrl Pts',(-55.914621693082,-99.662291203707,179.985484999752));
#28150=CARTESIAN_POINT('Ctrl Pts',(-54.7397120431402,-99.6932631932805,
178.813912075476));
#28151=CARTESIAN_POINT('Ctrl Pts',(-53.5648023931984,-99.724235182854,177.6423391512));
#28152=CARTESIAN_POINT('Ctrl Pts',(-53.5548643992186,-99.6310134108495,
175.985484901707));
#28153=CARTESIAN_POINT('Ctrl Pts',(-53.5449264052387,-99.5377916388449,
174.328630652215));
#28154=CARTESIAN_POINT('Ctrl Pts',(-54.6999600268383,-99.3203761095675,
173.157057825983));
#28155=CARTESIAN_POINT('Ctrl Pts',(-55.8549936484379,-99.10296058029,171.985484999752));
#28156=CARTESIAN_POINT('Ctrl Pts',(-57.4925742726078,-98.834102316693,171.985485069079));
#28157=CARTESIAN_POINT('Ctrl Pts',(-59.1301548967777,-98.5652440530961,
171.985485138407));
#28158=CARTESIAN_POINT('Ctrl Pts',(-60.2851884208854,-98.3478285342118,
173.157058062683));
#28159=CARTESIAN_POINT('Ctrl Pts',(-61.4402219449932,-98.1304130153276,
174.328630986959));
#28160=CARTESIAN_POINT('Ctrl Pts',(-61.430283813139,-98.0371912580215,175.985485236451));
#28161=CARTESIAN_POINT('Ctrl Pts',(-61.4203456812848,-97.9439695007152,
177.642339485944));
#28162=CARTESIAN_POINT('Ctrl Pts',(-60.2454359338512,-97.974941500682,178.813912312176));
#28163=CARTESIAN_POINT('Ctrl Pts',(-59.0705261864175,-98.0059135006488,
179.985485138407));
#28164=CARTESIAN_POINT('Ctrl Pts',(-57.4130694364136,-98.0883282349351,
179.985485069079));
#28165=CARTESIAN_POINT('Ctrl Pts',(-55.7556126864097,-98.1707429692214,
179.985484999752));
#28166=CARTESIAN_POINT('Ctrl Pts',(-54.580703036468,-98.2017149587949,178.813912075476));
#28167=CARTESIAN_POINT('Ctrl Pts',(-56.181115489574,-113.283598570176,178.821287383467));
#28168=CARTESIAN_POINT('Ctrl Pts',(-55.0031681001975,-113.314894403068,
177.646659506339));
#28169=CARTESIAN_POINT('Ctrl Pts',(-54.9932301063974,-113.221672631044,
175.985484901271));
#28170=CARTESIAN_POINT('Ctrl Pts',(-54.9832921125973,-113.12845085902,174.324310296203));
#28171=CARTESIAN_POINT('Ctrl Pts',(-56.1413634738858,-112.910711486397,
173.149682517375));
#28172=CARTESIAN_POINT('Ctrl Pts',(-57.2994348351743,-112.692972113774,
171.975054738546));
#28173=CARTESIAN_POINT('Ctrl Pts',(-58.9413114718314,-112.423655866545,
171.975054808055));
#28174=CARTESIAN_POINT('Ctrl Pts',(-60.5831881084886,-112.154339619316,
171.975054877564));
#28175=CARTESIAN_POINT('Ctrl Pts',(-61.741259372031,-111.936600257113,173.149682754692));
#28176=CARTESIAN_POINT('Ctrl Pts',(-62.8993306355734,-111.71886089491,174.32431063182));
#28177=CARTESIAN_POINT('Ctrl Pts',(-62.8893925035395,-111.625639137623,
175.985485236888));
#28178=CARTESIAN_POINT('Ctrl Pts',(-62.8794543715055,-111.532417380336,
177.646659841956));
#28179=CARTESIAN_POINT('Ctrl Pts',(-61.701506884383,-111.563713223648,178.821287620784));
#28180=CARTESIAN_POINT('Ctrl Pts',(-60.5235593972605,-111.595009066961,
179.995915399612));
#28181=CARTESIAN_POINT('Ctrl Pts',(-58.8618066347693,-111.677881784879,
179.995915330104));
#28182=CARTESIAN_POINT('Ctrl Pts',(-57.2000538722782,-111.760754502798,
179.995915260595));
#28183=CARTESIAN_POINT('Ctrl Pts',(-56.0221064829017,-111.79205033569,178.821287383467));
#28184=CARTESIAN_POINT('Ctrl Pts',(-54.8441590935253,-111.823346168582,
177.646659506339));
#28185=CARTESIAN_POINT('Ctrl Pts',(-54.8342210997252,-111.730124396559,
175.985484901271));
#28186=CARTESIAN_POINT('Ctrl Pts',(-54.8242831059251,-111.636902624535,
174.324310296203));
#28187=CARTESIAN_POINT('Ctrl Pts',(-55.9823544672136,-111.419163251912,
173.149682517375));
#28188=CARTESIAN_POINT('Ctrl Pts',(-57.1404258285021,-111.201423879289,
171.975054738546));
#28189=CARTESIAN_POINT('Ctrl Pts',(-58.7823024651592,-110.932107632059,
171.975054808055));
#28190=CARTESIAN_POINT('Ctrl Pts',(-60.4241791018163,-110.66279138483,171.975054877564));
#28191=CARTESIAN_POINT('Ctrl Pts',(-61.5822503653587,-110.445052022627,
173.149682754692));
#28192=CARTESIAN_POINT('Ctrl Pts',(-62.7403216289012,-110.227312660424,
174.32431063182));
#28193=CARTESIAN_POINT('Ctrl Pts',(-62.7303834968672,-110.134090903137,
175.985485236888));
#28194=CARTESIAN_POINT('Ctrl Pts',(-62.7204453648333,-110.04086914585,177.646659841956));
#28195=CARTESIAN_POINT('Ctrl Pts',(-61.5424978777108,-110.072164989163,
178.821287620784));
#28196=CARTESIAN_POINT('Ctrl Pts',(-60.3645503905882,-110.103460832475,
179.995915399612));
#28197=CARTESIAN_POINT('Ctrl Pts',(-58.7027976280971,-110.186333550394,
179.995915330104));
#28198=CARTESIAN_POINT('Ctrl Pts',(-57.041044865606,-110.269206268313,179.995915260595));
#28199=CARTESIAN_POINT('Ctrl Pts',(-55.8630974762295,-110.300502101205,
178.821287383467));
#28200=CARTESIAN_POINT('Ctrl Pts',(-54.6851500868531,-110.331797934097,
177.646659506339));
#28201=CARTESIAN_POINT('Ctrl Pts',(-54.675212093053,-110.238576162073,175.985484901271));
#28202=CARTESIAN_POINT('Ctrl Pts',(-54.6652740992529,-110.145354390049,
174.324310296203));
#28203=CARTESIAN_POINT('Ctrl Pts',(-55.8233454605414,-109.927615017426,
173.149682517375));
#28204=CARTESIAN_POINT('Ctrl Pts',(-56.9814168218299,-109.709875644803,
171.975054738546));
#28205=CARTESIAN_POINT('Ctrl Pts',(-58.623293458487,-109.440559397574,171.975054808055));
#28206=CARTESIAN_POINT('Ctrl Pts',(-60.2651700951441,-109.171243150344,
171.975054877564));
#28207=CARTESIAN_POINT('Ctrl Pts',(-61.4232413586865,-108.953503788142,
173.149682754692));
#28208=CARTESIAN_POINT('Ctrl Pts',(-62.581312622229,-108.735764425939,174.32431063182));
#28209=CARTESIAN_POINT('Ctrl Pts',(-62.571374490195,-108.642542668652,175.985485236888));
#28210=CARTESIAN_POINT('Ctrl Pts',(-62.5614363581611,-108.549320911365,
177.646659841956));
#28211=CARTESIAN_POINT('Ctrl Pts',(-61.3834888710385,-108.580616754677,
178.821287620784));
#28212=CARTESIAN_POINT('Ctrl Pts',(-60.205541383916,-108.61191259799,179.995915399612));
#28213=CARTESIAN_POINT('Ctrl Pts',(-58.5437886214249,-108.694785315908,
179.995915330104));
#28214=CARTESIAN_POINT('Ctrl Pts',(-56.8820358589338,-108.777658033827,
179.995915260595));
#28215=CARTESIAN_POINT('Ctrl Pts',(-55.7040884695573,-108.808953866719,
178.821287383467));
#28216=CARTESIAN_POINT('Ctrl Pts',(-54.5261410801808,-108.840249699611,
177.646659506339));
#28217=CARTESIAN_POINT('Ctrl Pts',(-54.5162030863807,-108.747027927587,
175.985484901271));
#28218=CARTESIAN_POINT('Ctrl Pts',(-54.5062650925806,-108.653806155564,
174.324310296203));
#28219=CARTESIAN_POINT('Ctrl Pts',(-55.6643364538691,-108.436066782941,
173.149682517375));
#28220=CARTESIAN_POINT('Ctrl Pts',(-56.8224078151577,-108.218327410317,
171.975054738546));
#28221=CARTESIAN_POINT('Ctrl Pts',(-58.4642844518147,-107.949011163088,
171.975054808055));
#28222=CARTESIAN_POINT('Ctrl Pts',(-60.1061610884719,-107.679694915859,
171.975054877564));
#28223=CARTESIAN_POINT('Ctrl Pts',(-61.2642323520143,-107.461955553656,
173.149682754692));
#28224=CARTESIAN_POINT('Ctrl Pts',(-62.4223036155567,-107.244216191453,
174.32431063182));
#28225=CARTESIAN_POINT('Ctrl Pts',(-62.4123654835228,-107.150994434166,
175.985485236888));
#28226=CARTESIAN_POINT('Ctrl Pts',(-62.4024273514889,-107.057772676879,
177.646659841956));
#28227=CARTESIAN_POINT('Ctrl Pts',(-61.2244798643663,-107.089068520192,
178.821287620784));
#28228=CARTESIAN_POINT('Ctrl Pts',(-60.0465323772438,-107.120364363504,
179.995915399612));
#28229=CARTESIAN_POINT('Ctrl Pts',(-58.3847796147526,-107.203237081423,
179.995915330104));
#28230=CARTESIAN_POINT('Ctrl Pts',(-56.7230268522615,-107.286109799341,
179.995915260595));
#28231=CARTESIAN_POINT('Ctrl Pts',(-55.5450794628851,-107.317405632233,
178.821287383467));
#28232=CARTESIAN_POINT('Ctrl Pts',(-54.3671320735086,-107.348701465125,
177.646659506339));
#28233=CARTESIAN_POINT('Ctrl Pts',(-54.3571940797085,-107.255479693102,
175.985484901271));
#28234=CARTESIAN_POINT('Ctrl Pts',(-54.3472560859084,-107.162257921078,
174.324310296203));
#28235=CARTESIAN_POINT('Ctrl Pts',(-55.5053274471969,-106.944518548455,
173.149682517375));
#28236=CARTESIAN_POINT('Ctrl Pts',(-56.6633988084854,-106.726779175832,
171.975054738546));
#28237=CARTESIAN_POINT('Ctrl Pts',(-58.3052754451425,-106.457462928602,
171.975054808055));
#28238=CARTESIAN_POINT('Ctrl Pts',(-59.9471520817997,-106.188146681373,
171.975054877564));
#28239=CARTESIAN_POINT('Ctrl Pts',(-61.1052233453421,-105.97040731917,173.149682754692));
#28240=CARTESIAN_POINT('Ctrl Pts',(-62.2632946088845,-105.752667956968,
174.32431063182));
#28241=CARTESIAN_POINT('Ctrl Pts',(-62.2533564768505,-105.659446199681,
175.985485236888));
#28242=CARTESIAN_POINT('Ctrl Pts',(-62.2434183448166,-105.566224442394,
177.646659841956));
#28243=CARTESIAN_POINT('Ctrl Pts',(-61.0654708576941,-105.597520285706,
178.821287620784));
#28244=CARTESIAN_POINT('Ctrl Pts',(-59.8875233705716,-105.628816129018,
179.995915399612));
#28245=CARTESIAN_POINT('Ctrl Pts',(-58.2257706080804,-105.711688846937,
179.995915330104));
#28246=CARTESIAN_POINT('Ctrl Pts',(-56.5640178455893,-105.794561564856,
179.995915260595));
#28247=CARTESIAN_POINT('Ctrl Pts',(-55.3860704562128,-105.825857397748,
178.821287383467));
#28248=CARTESIAN_POINT('Ctrl Pts',(-54.2081230668364,-105.85715323064,177.646659506339));
#28249=CARTESIAN_POINT('Ctrl Pts',(-54.1981850730363,-105.763931458616,
175.985484901271));
#28250=CARTESIAN_POINT('Ctrl Pts',(-54.1882470792362,-105.670709686593,
174.324310296203));
#28251=CARTESIAN_POINT('Ctrl Pts',(-55.3463184405247,-105.452970313969,
173.149682517375));
#28252=CARTESIAN_POINT('Ctrl Pts',(-56.5043898018132,-105.235230941346,
171.975054738546));
#28253=CARTESIAN_POINT('Ctrl Pts',(-58.1462664384703,-104.965914694117,
171.975054808055));
#28254=CARTESIAN_POINT('Ctrl Pts',(-59.7881430751274,-104.696598446888,
171.975054877564));
#28255=CARTESIAN_POINT('Ctrl Pts',(-60.9462143386698,-104.478859084685,
173.149682754692));
#28256=CARTESIAN_POINT('Ctrl Pts',(-62.1042856022123,-104.261119722482,
174.32431063182));
#28257=CARTESIAN_POINT('Ctrl Pts',(-62.0943474701783,-104.167897965195,
175.985485236888));
#28258=CARTESIAN_POINT('Ctrl Pts',(-62.0844093381444,-104.074676207908,
177.646659841956));
#28259=CARTESIAN_POINT('Ctrl Pts',(-60.9064618510219,-104.10597205122,178.821287620784));
#28260=CARTESIAN_POINT('Ctrl Pts',(-59.7285143638993,-104.137267894533,
179.995915399612));
#28261=CARTESIAN_POINT('Ctrl Pts',(-58.0667616014082,-104.220140612451,
179.995915330104));
#28262=CARTESIAN_POINT('Ctrl Pts',(-56.4050088389171,-104.30301333037,179.995915260595));
#28263=CARTESIAN_POINT('Ctrl Pts',(-55.2270614495406,-104.334309163262,
178.821287383467));
#28264=CARTESIAN_POINT('Ctrl Pts',(-54.0491140601642,-104.365604996154,
177.646659506339));
#28265=CARTESIAN_POINT('Ctrl Pts',(-54.039176066364,-104.272383224131,175.985484901271));
#28266=CARTESIAN_POINT('Ctrl Pts',(-54.029238072564,-104.179161452107,174.324310296203));
#28267=CARTESIAN_POINT('Ctrl Pts',(-55.1873094338524,-103.961422079484,
173.149682517375));
#28268=CARTESIAN_POINT('Ctrl Pts',(-56.345380795141,-103.743682706861,171.975054738546));
#28269=CARTESIAN_POINT('Ctrl Pts',(-57.9872574317981,-103.474366459631,
171.975054808055));
#28270=CARTESIAN_POINT('Ctrl Pts',(-59.6291340684552,-103.205050212402,
171.975054877564));
#28271=CARTESIAN_POINT('Ctrl Pts',(-60.7872053319976,-102.987310850199,
173.149682754692));
#28272=CARTESIAN_POINT('Ctrl Pts',(-61.94527659554,-102.769571487996,174.32431063182));
#28273=CARTESIAN_POINT('Ctrl Pts',(-61.9353384635061,-102.676349730709,
175.985485236888));
#28274=CARTESIAN_POINT('Ctrl Pts',(-61.9254003314722,-102.583127973422,
177.646659841956));
#28275=CARTESIAN_POINT('Ctrl Pts',(-60.7474528443496,-102.614423816735,
178.821287620784));
#28276=CARTESIAN_POINT('Ctrl Pts',(-59.5695053572271,-102.645719660047,
179.995915399612));
#28277=CARTESIAN_POINT('Ctrl Pts',(-57.907752594736,-102.728592377966,179.995915330104));
#28278=CARTESIAN_POINT('Ctrl Pts',(-56.2459998322448,-102.811465095885,
179.995915260595));
#28279=CARTESIAN_POINT('Ctrl Pts',(-55.0680524428684,-102.842760928777,
178.821287383467));
#28280=CARTESIAN_POINT('Ctrl Pts',(-53.8901050534919,-102.874056761669,
177.646659506339));
#28281=CARTESIAN_POINT('Ctrl Pts',(-53.8801670596918,-102.780834989645,
175.985484901271));
#28282=CARTESIAN_POINT('Ctrl Pts',(-53.8702290658917,-102.687613217621,
174.324310296203));
#28283=CARTESIAN_POINT('Ctrl Pts',(-55.0283004271802,-102.469873844998,
173.149682517375));
#28284=CARTESIAN_POINT('Ctrl Pts',(-56.1863717884687,-102.252134472375,
171.975054738546));
#28285=CARTESIAN_POINT('Ctrl Pts',(-57.8282484251258,-101.982818225146,
171.975054808055));
#28286=CARTESIAN_POINT('Ctrl Pts',(-59.470125061783,-101.713501977916,171.975054877564));
#28287=CARTESIAN_POINT('Ctrl Pts',(-60.6281963253254,-101.495762615714,
173.149682754692));
#28288=CARTESIAN_POINT('Ctrl Pts',(-61.7862675888678,-101.278023253511,
174.32431063182));
#28289=CARTESIAN_POINT('Ctrl Pts',(-61.7763294568339,-101.184801496224,
175.985485236888));
#28290=CARTESIAN_POINT('Ctrl Pts',(-61.7663913247999,-101.091579738937,
177.646659841956));
#28291=CARTESIAN_POINT('Ctrl Pts',(-60.5884438376774,-101.122875582249,
178.821287620784));
#28292=CARTESIAN_POINT('Ctrl Pts',(-59.4104963505549,-101.154171425562,
179.995915399612));
#28293=CARTESIAN_POINT('Ctrl Pts',(-57.7487435880637,-101.23704414348,179.995915330104));
#28294=CARTESIAN_POINT('Ctrl Pts',(-56.0869908255726,-101.319916861399,
179.995915260595));
#28295=CARTESIAN_POINT('Ctrl Pts',(-54.9090434361961,-101.351212694291,
178.821287383467));
#28296=CARTESIAN_POINT('Ctrl Pts',(-53.7310960468197,-101.382508527183,
177.646659506339));
#28297=CARTESIAN_POINT('Ctrl Pts',(-53.7211580530196,-101.289286755159,
175.985484901271));
#28298=CARTESIAN_POINT('Ctrl Pts',(-53.7112200592195,-101.196064983136,
174.324310296203));
#28299=CARTESIAN_POINT('Ctrl Pts',(-54.869291420508,-100.978325610513,173.149682517375));
#28300=CARTESIAN_POINT('Ctrl Pts',(-56.0273627817965,-100.760586237889,
171.975054738546));
#28301=CARTESIAN_POINT('Ctrl Pts',(-57.6692394184536,-100.49126999066,171.975054808055));
#28302=CARTESIAN_POINT('Ctrl Pts',(-59.3111160551107,-100.221953743431,
171.975054877564));
#28303=CARTESIAN_POINT('Ctrl Pts',(-60.4691873186531,-100.004214381228,
173.149682754692));
#28304=CARTESIAN_POINT('Ctrl Pts',(-61.6272585821956,-99.7864750190253,
174.32431063182));
#28305=CARTESIAN_POINT('Ctrl Pts',(-61.6173204501616,-99.6932532617382,
175.985485236888));
#28306=CARTESIAN_POINT('Ctrl Pts',(-61.6073823181277,-99.6000315044512,
177.646659841956));
#28307=CARTESIAN_POINT('Ctrl Pts',(-60.4294348310052,-99.6313273477637,
178.821287620784));
#28308=CARTESIAN_POINT('Ctrl Pts',(-59.2514873438827,-99.6626231910761,
179.995915399612));
#28309=CARTESIAN_POINT('Ctrl Pts',(-57.5897345813915,-99.7454959089947,
179.995915330104));
#28310=CARTESIAN_POINT('Ctrl Pts',(-55.9279818189004,-99.8283686269133,
179.995915260595));
#28311=CARTESIAN_POINT('Ctrl Pts',(-54.7500344295239,-99.8596644598054,
178.821287383467));
#28312=CARTESIAN_POINT('Ctrl Pts',(-53.5720870401475,-99.8909602926975,
177.646659506339));
#28313=CARTESIAN_POINT('Ctrl Pts',(-53.5621490463474,-99.7977385206737,
175.985484901271));
#28314=CARTESIAN_POINT('Ctrl Pts',(-53.5522110525473,-99.7045167486501,
174.324310296203));
#28315=CARTESIAN_POINT('Ctrl Pts',(-54.7102824138358,-99.4867773760269,
173.149682517375));
#28316=CARTESIAN_POINT('Ctrl Pts',(-55.8683537751243,-99.2690380034038,
171.975054738546));
#28317=CARTESIAN_POINT('Ctrl Pts',(-57.5102304117814,-98.9997217561745,
171.975054808055));
#28318=CARTESIAN_POINT('Ctrl Pts',(-59.1521070484385,-98.7304055089452,
171.975054877564));
#28319=CARTESIAN_POINT('Ctrl Pts',(-60.3101783119809,-98.5126661467424,
173.149682754692));
#28320=CARTESIAN_POINT('Ctrl Pts',(-61.4682495755234,-98.2949267845397,
174.32431063182));
#28321=CARTESIAN_POINT('Ctrl Pts',(-61.4583114434894,-98.2017050272526,
175.985485236888));
#28322=CARTESIAN_POINT('Ctrl Pts',(-61.4483733114555,-98.1084832699656,
177.646659841956));
#28323=CARTESIAN_POINT('Ctrl Pts',(-60.2704258243329,-98.139779113278,178.821287620784));
#28324=CARTESIAN_POINT('Ctrl Pts',(-59.0924783372104,-98.1710749565905,
179.995915399612));
#28325=CARTESIAN_POINT('Ctrl Pts',(-57.4307255747193,-98.2539476745091,
179.995915330104));
#28326=CARTESIAN_POINT('Ctrl Pts',(-55.7689728122282,-98.3368203924277,
179.995915260595));
#28327=CARTESIAN_POINT('Ctrl Pts',(-54.5910254228517,-98.3681162253198,
178.821287383467));
#28328=CARTESIAN_POINT('Ctrl Pts',(-56.1988062143188,-113.449542435949,
178.821287383467));
#28329=CARTESIAN_POINT('Ctrl Pts',(-55.0208588249424,-113.480838268841,
177.646659506339));
#28330=CARTESIAN_POINT('Ctrl Pts',(-55.0109208311422,-113.387616496817,
175.985484901271));
#28331=CARTESIAN_POINT('Ctrl Pts',(-55.0009828373422,-113.294394724794,
174.324310296203));
#28332=CARTESIAN_POINT('Ctrl Pts',(-56.1590541986307,-113.07665535217,173.149682517375));
#28333=CARTESIAN_POINT('Ctrl Pts',(-57.3171255599192,-112.858915979547,
171.975054738546));
#28334=CARTESIAN_POINT('Ctrl Pts',(-58.9590021965763,-112.589599732318,
171.975054808055));
#28335=CARTESIAN_POINT('Ctrl Pts',(-60.6008788332334,-112.320283485089,
171.975054877564));
#28336=CARTESIAN_POINT('Ctrl Pts',(-61.7589500967758,-112.102544122886,
173.149682754692));
#28337=CARTESIAN_POINT('Ctrl Pts',(-62.9170213603182,-111.884804760683,
174.32431063182));
#28338=CARTESIAN_POINT('Ctrl Pts',(-62.9070832282843,-111.791583003396,
175.985485236888));
#28339=CARTESIAN_POINT('Ctrl Pts',(-62.8971450962504,-111.698361246109,
177.646659841956));
#28340=CARTESIAN_POINT('Ctrl Pts',(-61.7191976091278,-111.729657089422,
178.821287620784));
#28341=CARTESIAN_POINT('Ctrl Pts',(-60.5412501220053,-111.760952932734,
179.995915399612));
#28342=CARTESIAN_POINT('Ctrl Pts',(-58.8794973595142,-111.843825650653,
179.995915330104));
#28343=CARTESIAN_POINT('Ctrl Pts',(-57.217744597023,-111.926698368571,179.995915260595));
#28344=CARTESIAN_POINT('Ctrl Pts',(-56.0397972076466,-111.957994201463,
178.821287383467));
#28345=CARTESIAN_POINT('Ctrl Pts',(-54.8618498182701,-111.989290034355,
177.646659506339));
#28346=CARTESIAN_POINT('Ctrl Pts',(-54.85191182447,-111.896068262332,175.985484901271));
#28347=CARTESIAN_POINT('Ctrl Pts',(-54.8419738306699,-111.802846490308,
174.324310296203));
#28348=CARTESIAN_POINT('Ctrl Pts',(-56.0000451919584,-111.585107117685,
173.149682517375));
#28349=CARTESIAN_POINT('Ctrl Pts',(-57.158116553247,-111.367367745062,171.975054738546));
#28350=CARTESIAN_POINT('Ctrl Pts',(-58.799993189904,-111.098051497832,171.975054808055));
#28351=CARTESIAN_POINT('Ctrl Pts',(-60.4418698265612,-110.828735250603,
171.975054877564));
#28352=CARTESIAN_POINT('Ctrl Pts',(-61.5999410901036,-110.6109958884,173.149682754692));
#28353=CARTESIAN_POINT('Ctrl Pts',(-62.758012353646,-110.393256526198,174.32431063182));
#28354=CARTESIAN_POINT('Ctrl Pts',(-62.7480742216121,-110.30003476891,175.985485236888));
#28355=CARTESIAN_POINT('Ctrl Pts',(-62.7381360895782,-110.206813011623,
177.646659841956));
#28356=CARTESIAN_POINT('Ctrl Pts',(-61.5601886024556,-110.238108854936,
178.821287620784));
#28357=CARTESIAN_POINT('Ctrl Pts',(-60.3822411153331,-110.269404698248,
179.995915399612));
#28358=CARTESIAN_POINT('Ctrl Pts',(-58.7204883528419,-110.352277416167,
179.995915330104));
#28359=CARTESIAN_POINT('Ctrl Pts',(-57.0587355903508,-110.435150134086,
179.995915260595));
#28360=CARTESIAN_POINT('Ctrl Pts',(-55.8807882009743,-110.466445966978,
178.821287383467));
#28361=CARTESIAN_POINT('Ctrl Pts',(-54.7028408115979,-110.49774179987,177.646659506339));
#28362=CARTESIAN_POINT('Ctrl Pts',(-54.6929028177978,-110.404520027846,
175.985484901271));
#28363=CARTESIAN_POINT('Ctrl Pts',(-54.6829648239977,-110.311298255822,
174.324310296203));
#28364=CARTESIAN_POINT('Ctrl Pts',(-55.8410361852862,-110.093558883199,
173.149682517375));
#28365=CARTESIAN_POINT('Ctrl Pts',(-56.9991075465747,-109.875819510576,
171.975054738546));
#28366=CARTESIAN_POINT('Ctrl Pts',(-58.6409841832318,-109.606503263347,
171.975054808055));
#28367=CARTESIAN_POINT('Ctrl Pts',(-60.2828608198889,-109.337187016117,
171.975054877564));
#28368=CARTESIAN_POINT('Ctrl Pts',(-61.4409320834313,-109.119447653915,
173.149682754692));
#28369=CARTESIAN_POINT('Ctrl Pts',(-62.5990033469738,-108.901708291712,
174.32431063182));
#28370=CARTESIAN_POINT('Ctrl Pts',(-62.5890652149398,-108.808486534425,
175.985485236888));
#28371=CARTESIAN_POINT('Ctrl Pts',(-62.5791270829059,-108.715264777138,
177.646659841956));
#28372=CARTESIAN_POINT('Ctrl Pts',(-61.4011795957834,-108.74656062045,178.821287620784));
#28373=CARTESIAN_POINT('Ctrl Pts',(-60.2232321086609,-108.777856463763,
179.995915399612));
#28374=CARTESIAN_POINT('Ctrl Pts',(-58.5614793461697,-108.860729181681,
179.995915330104));
#28375=CARTESIAN_POINT('Ctrl Pts',(-56.8997265836786,-108.9436018996,179.995915260595));
#28376=CARTESIAN_POINT('Ctrl Pts',(-55.7217791943021,-108.974897732492,
178.821287383467));
#28377=CARTESIAN_POINT('Ctrl Pts',(-54.5438318049257,-109.006193565384,
177.646659506339));
#28378=CARTESIAN_POINT('Ctrl Pts',(-54.5338938111256,-108.91297179336,175.985484901271));
#28379=CARTESIAN_POINT('Ctrl Pts',(-54.5239558173255,-108.819750021337,
174.324310296203));
#28380=CARTESIAN_POINT('Ctrl Pts',(-55.682027178614,-108.602010648714,173.149682517375));
#28381=CARTESIAN_POINT('Ctrl Pts',(-56.8400985399025,-108.384271276091,
171.975054738546));
#28382=CARTESIAN_POINT('Ctrl Pts',(-58.4819751765596,-108.114955028861,
171.975054808055));
#28383=CARTESIAN_POINT('Ctrl Pts',(-60.1238518132167,-107.845638781632,
171.975054877564));
#28384=CARTESIAN_POINT('Ctrl Pts',(-61.2819230767591,-107.627899419429,
173.149682754692));
#28385=CARTESIAN_POINT('Ctrl Pts',(-62.4399943403016,-107.410160057226,
174.32431063182));
#28386=CARTESIAN_POINT('Ctrl Pts',(-62.4300562082676,-107.316938299939,
175.985485236888));
#28387=CARTESIAN_POINT('Ctrl Pts',(-62.4201180762337,-107.223716542652,
177.646659841956));
#28388=CARTESIAN_POINT('Ctrl Pts',(-61.2421705891111,-107.255012385965,
178.821287620784));
#28389=CARTESIAN_POINT('Ctrl Pts',(-60.0642231019886,-107.286308229277,
179.995915399612));
#28390=CARTESIAN_POINT('Ctrl Pts',(-58.4024703394975,-107.369180947196,
179.995915330104));
#28391=CARTESIAN_POINT('Ctrl Pts',(-56.7407175770064,-107.452053665114,
179.995915260595));
#28392=CARTESIAN_POINT('Ctrl Pts',(-55.5627701876299,-107.483349498006,
178.821287383467));
#28393=CARTESIAN_POINT('Ctrl Pts',(-54.3848227982534,-107.514645330899,
177.646659506339));
#28394=CARTESIAN_POINT('Ctrl Pts',(-54.3748848044533,-107.421423558875,
175.985484901271));
#28395=CARTESIAN_POINT('Ctrl Pts',(-54.3649468106533,-107.328201786851,
174.324310296203));
#28396=CARTESIAN_POINT('Ctrl Pts',(-55.5230181719417,-107.110462414228,
173.149682517375));
#28397=CARTESIAN_POINT('Ctrl Pts',(-56.6810895332303,-106.892723041605,
171.975054738546));
#28398=CARTESIAN_POINT('Ctrl Pts',(-58.3229661698874,-106.623406794376,
171.975054808055));
#28399=CARTESIAN_POINT('Ctrl Pts',(-59.9648428065445,-106.354090547146,
171.975054877564));
#28400=CARTESIAN_POINT('Ctrl Pts',(-61.1229140700869,-106.136351184943,
173.149682754692));
#28401=CARTESIAN_POINT('Ctrl Pts',(-62.2809853336293,-105.918611822741,
174.32431063182));
#28402=CARTESIAN_POINT('Ctrl Pts',(-62.2710472015954,-105.825390065454,
175.985485236888));
#28403=CARTESIAN_POINT('Ctrl Pts',(-62.2611090695615,-105.732168308167,
177.646659841956));
#28404=CARTESIAN_POINT('Ctrl Pts',(-61.0831615824389,-105.763464151479,
178.821287620784));
#28405=CARTESIAN_POINT('Ctrl Pts',(-59.9052140953164,-105.794759994792,
179.995915399612));
#28406=CARTESIAN_POINT('Ctrl Pts',(-58.2434613328252,-105.87763271271,179.995915330104));
#28407=CARTESIAN_POINT('Ctrl Pts',(-56.5817085703341,-105.960505430629,
179.995915260595));
#28408=CARTESIAN_POINT('Ctrl Pts',(-55.4037611809577,-105.991801263521,
178.821287383467));
#28409=CARTESIAN_POINT('Ctrl Pts',(-54.2258137915812,-106.023097096413,
177.646659506339));
#28410=CARTESIAN_POINT('Ctrl Pts',(-54.2158757977811,-105.929875324389,
175.985484901271));
#28411=CARTESIAN_POINT('Ctrl Pts',(-54.205937803981,-105.836653552366,174.324310296203));
#28412=CARTESIAN_POINT('Ctrl Pts',(-55.3640091652695,-105.618914179742,
173.149682517375));
#28413=CARTESIAN_POINT('Ctrl Pts',(-56.522080526558,-105.401174807119,171.975054738546));
#28414=CARTESIAN_POINT('Ctrl Pts',(-58.1639571632151,-105.13185855989,171.975054808055));
#28415=CARTESIAN_POINT('Ctrl Pts',(-59.8058337998722,-104.862542312661,
171.975054877564));
#28416=CARTESIAN_POINT('Ctrl Pts',(-60.9639050634147,-104.644802950458,
173.149682754692));
#28417=CARTESIAN_POINT('Ctrl Pts',(-62.1219763269571,-104.427063588255,
174.32431063182));
#28418=CARTESIAN_POINT('Ctrl Pts',(-62.1120381949232,-104.333841830968,
175.985485236888));
#28419=CARTESIAN_POINT('Ctrl Pts',(-62.1021000628892,-104.240620073681,
177.646659841956));
#28420=CARTESIAN_POINT('Ctrl Pts',(-60.9241525757667,-104.271915916993,
178.821287620784));
#28421=CARTESIAN_POINT('Ctrl Pts',(-59.7462050886442,-104.303211760306,
179.995915399612));
#28422=CARTESIAN_POINT('Ctrl Pts',(-58.084452326153,-104.386084478225,179.995915330104));
#28423=CARTESIAN_POINT('Ctrl Pts',(-56.4226995636619,-104.468957196143,
179.995915260595));
#28424=CARTESIAN_POINT('Ctrl Pts',(-55.2447521742854,-104.500253029035,
178.821287383467));
#28425=CARTESIAN_POINT('Ctrl Pts',(-54.066804784909,-104.531548861927,177.646659506339));
#28426=CARTESIAN_POINT('Ctrl Pts',(-54.0568667911089,-104.438327089904,
175.985484901271));
#28427=CARTESIAN_POINT('Ctrl Pts',(-54.0469287973088,-104.34510531788,174.324310296203));
#28428=CARTESIAN_POINT('Ctrl Pts',(-55.2050001585973,-104.127365945257,
173.149682517375));
#28429=CARTESIAN_POINT('Ctrl Pts',(-56.3630715198858,-103.909626572634,
171.975054738546));
#28430=CARTESIAN_POINT('Ctrl Pts',(-58.0049481565429,-103.640310325404,
171.975054808055));
#28431=CARTESIAN_POINT('Ctrl Pts',(-59.6468247932,-103.370994078175,171.975054877564));
#28432=CARTESIAN_POINT('Ctrl Pts',(-60.8048960567424,-103.153254715972,
173.149682754692));
#28433=CARTESIAN_POINT('Ctrl Pts',(-61.9629673202849,-102.93551535377,174.32431063182));
#28434=CARTESIAN_POINT('Ctrl Pts',(-61.9530291882509,-102.842293596483,
175.985485236888));
#28435=CARTESIAN_POINT('Ctrl Pts',(-61.943091056217,-102.749071839196,177.646659841956));
#28436=CARTESIAN_POINT('Ctrl Pts',(-60.7651435690945,-102.780367682508,
178.821287620784));
#28437=CARTESIAN_POINT('Ctrl Pts',(-59.587196081972,-102.81166352582,179.995915399612));
#28438=CARTESIAN_POINT('Ctrl Pts',(-57.9254433194808,-102.894536243739,
179.995915330104));
#28439=CARTESIAN_POINT('Ctrl Pts',(-56.2636905569897,-102.977408961658,
179.995915260595));
#28440=CARTESIAN_POINT('Ctrl Pts',(-55.0857431676132,-103.00870479455,178.821287383467));
#28441=CARTESIAN_POINT('Ctrl Pts',(-53.9077957782368,-103.040000627442,
177.646659506339));
#28442=CARTESIAN_POINT('Ctrl Pts',(-53.8978577844367,-102.946778855418,
175.985484901271));
#28443=CARTESIAN_POINT('Ctrl Pts',(-53.8879197906366,-102.853557083394,
174.324310296203));
#28444=CARTESIAN_POINT('Ctrl Pts',(-55.0459911519251,-102.635817710771,
173.149682517375));
#28445=CARTESIAN_POINT('Ctrl Pts',(-56.2040625132136,-102.418078338148,
171.975054738546));
#28446=CARTESIAN_POINT('Ctrl Pts',(-57.8459391498707,-102.148762090919,
171.975054808055));
#28447=CARTESIAN_POINT('Ctrl Pts',(-59.4878157865278,-101.879445843689,
171.975054877564));
#28448=CARTESIAN_POINT('Ctrl Pts',(-60.6458870500702,-101.661706481487,
173.149682754692));
#28449=CARTESIAN_POINT('Ctrl Pts',(-61.8039583136126,-101.443967119284,
174.32431063182));
#28450=CARTESIAN_POINT('Ctrl Pts',(-61.7940201815787,-101.350745361997,
175.985485236888));
#28451=CARTESIAN_POINT('Ctrl Pts',(-61.7840820495448,-101.25752360471,177.646659841956));
#28452=CARTESIAN_POINT('Ctrl Pts',(-60.6061345624222,-101.288819448022,
178.821287620784));
#28453=CARTESIAN_POINT('Ctrl Pts',(-59.4281870752997,-101.320115291335,
179.995915399612));
#28454=CARTESIAN_POINT('Ctrl Pts',(-57.7664343128086,-101.402988009253,
179.995915330104));
#28455=CARTESIAN_POINT('Ctrl Pts',(-56.1046815503175,-101.485860727172,
179.995915260595));
#28456=CARTESIAN_POINT('Ctrl Pts',(-54.926734160941,-101.517156560064,178.821287383467));
#28457=CARTESIAN_POINT('Ctrl Pts',(-53.7487867715645,-101.548452392956,
177.646659506339));
#28458=CARTESIAN_POINT('Ctrl Pts',(-53.7388487777644,-101.455230620932,
175.985484901271));
#28459=CARTESIAN_POINT('Ctrl Pts',(-53.7289107839643,-101.362008848909,
174.324310296203));
#28460=CARTESIAN_POINT('Ctrl Pts',(-54.8869821452528,-101.144269476286,
173.149682517375));
#28461=CARTESIAN_POINT('Ctrl Pts',(-56.0450535065414,-100.926530103662,
171.975054738546));
#28462=CARTESIAN_POINT('Ctrl Pts',(-57.6869301431984,-100.657213856433,
171.975054808055));
#28463=CARTESIAN_POINT('Ctrl Pts',(-59.3288067798556,-100.387897609204,
171.975054877564));
#28464=CARTESIAN_POINT('Ctrl Pts',(-60.486878043398,-100.170158247001,173.149682754692));
#28465=CARTESIAN_POINT('Ctrl Pts',(-61.6449493069404,-99.9524188847983,
174.32431063182));
#28466=CARTESIAN_POINT('Ctrl Pts',(-61.6350111749065,-99.8591971275113,
175.985485236888));
#28467=CARTESIAN_POINT('Ctrl Pts',(-61.6250730428726,-99.7659753702243,
177.646659841956));
#28468=CARTESIAN_POINT('Ctrl Pts',(-60.44712555575,-99.7972712135367,178.821287620784));
#28469=CARTESIAN_POINT('Ctrl Pts',(-59.2691780686275,-99.8285670568492,
179.995915399612));
#28470=CARTESIAN_POINT('Ctrl Pts',(-57.6074253061363,-99.9114397747677,
179.995915330104));
#28471=CARTESIAN_POINT('Ctrl Pts',(-55.9456725436452,-99.9943124926864,
179.995915260595));
#28472=CARTESIAN_POINT('Ctrl Pts',(-54.7677251542687,-100.025608325578,
178.821287383467));
#28473=CARTESIAN_POINT('Ctrl Pts',(-53.5897777648923,-100.05690415847,177.646659506339));
#28474=CARTESIAN_POINT('Ctrl Pts',(-53.5798397710922,-99.9636823864468,
175.985484901271));
#28475=CARTESIAN_POINT('Ctrl Pts',(-53.5699017772921,-99.8704606144232,
174.324310296203));
#28476=CARTESIAN_POINT('Ctrl Pts',(-54.7279731385806,-99.6527212418,173.149682517375));
#28477=CARTESIAN_POINT('Ctrl Pts',(-55.8860444998691,-99.4349818691769,
171.975054738546));
#28478=CARTESIAN_POINT('Ctrl Pts',(-57.5279211365262,-99.1656656219475,
171.975054808055));
#28479=CARTESIAN_POINT('Ctrl Pts',(-59.1697977731833,-98.8963493747183,
171.975054877564));
#28480=CARTESIAN_POINT('Ctrl Pts',(-60.3278690367257,-98.6786100125155,
173.149682754692));
#28481=CARTESIAN_POINT('Ctrl Pts',(-61.4859403002682,-98.4608706503128,
174.32431063182));
#28482=CARTESIAN_POINT('Ctrl Pts',(-61.4760021682342,-98.3676488930257,
175.985485236888));
#28483=CARTESIAN_POINT('Ctrl Pts',(-61.4660640362003,-98.2744271357387,
177.646659841956));
#28484=CARTESIAN_POINT('Ctrl Pts',(-60.2881165490778,-98.3057229790511,
178.821287620784));
#28485=CARTESIAN_POINT('Ctrl Pts',(-59.1101690619552,-98.3370188223636,
179.995915399612));
#28486=CARTESIAN_POINT('Ctrl Pts',(-57.4484162994641,-98.4198915402821,
179.995915330104));
#28487=CARTESIAN_POINT('Ctrl Pts',(-55.786663536973,-98.5027642582008,179.995915260595));
#28488=CARTESIAN_POINT('Ctrl Pts',(-54.6087161475965,-98.5340600910929,
178.821287383467));
#28489=CARTESIAN_POINT('Ctrl Pts',(-56.2237961054143,-113.614380048479,
178.813912075476));
#28490=CARTESIAN_POINT('Ctrl Pts',(-55.0488864554725,-113.645352038053,
177.6423391512));
#28491=CARTESIAN_POINT('Ctrl Pts',(-55.0389484614927,-113.552130266048,
175.985484901707));
#28492=CARTESIAN_POINT('Ctrl Pts',(-55.0290104675128,-113.458908494044,
174.328630652215));
#28493=CARTESIAN_POINT('Ctrl Pts',(-56.1840440891124,-113.241492964766,
173.157057825983));
#28494=CARTESIAN_POINT('Ctrl Pts',(-57.3390777107121,-113.024077435489,
171.985484999752));
#28495=CARTESIAN_POINT('Ctrl Pts',(-58.9766583348819,-112.755219171892,
171.985485069079));
#28496=CARTESIAN_POINT('Ctrl Pts',(-60.6142389590518,-112.486360908295,
171.985485138407));
#28497=CARTESIAN_POINT('Ctrl Pts',(-61.7692724831595,-112.268945389411,
173.157058062683));
#28498=CARTESIAN_POINT('Ctrl Pts',(-62.9243060072673,-112.051529870527,
174.328630986959));
#28499=CARTESIAN_POINT('Ctrl Pts',(-62.9143678754131,-111.95830811322,175.985485236451));
#28500=CARTESIAN_POINT('Ctrl Pts',(-62.9044297435589,-111.865086355914,
177.642339485944));
#28501=CARTESIAN_POINT('Ctrl Pts',(-61.7295199961253,-111.896058355881,
178.813912312176));
#28502=CARTESIAN_POINT('Ctrl Pts',(-60.5546102486917,-111.927030355848,
179.985485138407));
#28503=CARTESIAN_POINT('Ctrl Pts',(-58.8971534986878,-112.009445090134,
179.985485069079));
#28504=CARTESIAN_POINT('Ctrl Pts',(-57.2396967486839,-112.09185982442,179.985484999752));
#28505=CARTESIAN_POINT('Ctrl Pts',(-56.0647870987421,-112.122831813994,
178.813912075476));
#28506=CARTESIAN_POINT('Ctrl Pts',(-54.8898774488003,-112.153803803567,
177.6423391512));
#28507=CARTESIAN_POINT('Ctrl Pts',(-54.8799394548205,-112.060582031563,
175.985484901707));
#28508=CARTESIAN_POINT('Ctrl Pts',(-54.8700014608406,-111.967360259558,
174.328630652215));
#28509=CARTESIAN_POINT('Ctrl Pts',(-56.0250350824402,-111.749944730281,
173.157057825983));
#28510=CARTESIAN_POINT('Ctrl Pts',(-57.1800687040398,-111.532529201003,
171.985484999752));
#28511=CARTESIAN_POINT('Ctrl Pts',(-58.8176493282097,-111.263670937406,
171.985485069079));
#28512=CARTESIAN_POINT('Ctrl Pts',(-60.4552299523796,-110.994812673809,
171.985485138407));
#28513=CARTESIAN_POINT('Ctrl Pts',(-61.6102634764873,-110.777397154925,
173.157058062683));
#28514=CARTESIAN_POINT('Ctrl Pts',(-62.7652970005951,-110.559981636041,
174.328630986959));
#28515=CARTESIAN_POINT('Ctrl Pts',(-62.7553588687409,-110.466759878735,
175.985485236451));
#28516=CARTESIAN_POINT('Ctrl Pts',(-62.7454207368867,-110.373538121429,
177.642339485944));
#28517=CARTESIAN_POINT('Ctrl Pts',(-61.5705109894531,-110.404510121395,
178.813912312176));
#28518=CARTESIAN_POINT('Ctrl Pts',(-60.3956012420194,-110.435482121362,
179.985485138407));
#28519=CARTESIAN_POINT('Ctrl Pts',(-58.7381444920155,-110.517896855648,
179.985485069079));
#28520=CARTESIAN_POINT('Ctrl Pts',(-57.0806877420116,-110.600311589935,
179.985484999752));
#28521=CARTESIAN_POINT('Ctrl Pts',(-55.9057780920699,-110.631283579508,
178.813912075476));
#28522=CARTESIAN_POINT('Ctrl Pts',(-54.7308684421281,-110.662255569082,
177.6423391512));
#28523=CARTESIAN_POINT('Ctrl Pts',(-54.7209304481482,-110.569033797077,
175.985484901707));
#28524=CARTESIAN_POINT('Ctrl Pts',(-54.7109924541684,-110.475812025073,
174.328630652215));
#28525=CARTESIAN_POINT('Ctrl Pts',(-55.866026075768,-110.258396495795,173.157057825983));
#28526=CARTESIAN_POINT('Ctrl Pts',(-57.0210596973676,-110.040980966518,
171.985484999752));
#28527=CARTESIAN_POINT('Ctrl Pts',(-58.6586403215375,-109.772122702921,
171.985485069079));
#28528=CARTESIAN_POINT('Ctrl Pts',(-60.2962209457073,-109.503264439324,
171.985485138407));
#28529=CARTESIAN_POINT('Ctrl Pts',(-61.4512544698151,-109.28584892044,173.157058062683));
#28530=CARTESIAN_POINT('Ctrl Pts',(-62.6062879939228,-109.068433401555,
174.328630986959));
#28531=CARTESIAN_POINT('Ctrl Pts',(-62.5963498620687,-108.975211644249,
175.985485236451));
#28532=CARTESIAN_POINT('Ctrl Pts',(-62.5864117302145,-108.881989886943,
177.642339485944));
#28533=CARTESIAN_POINT('Ctrl Pts',(-61.4115019827808,-108.91296188691,178.813912312176));
#28534=CARTESIAN_POINT('Ctrl Pts',(-60.2365922353472,-108.943933886877,
179.985485138407));
#28535=CARTESIAN_POINT('Ctrl Pts',(-58.5791354853433,-109.026348621163,
179.985485069079));
#28536=CARTESIAN_POINT('Ctrl Pts',(-56.9216787353394,-109.108763355449,
179.985484999752));
#28537=CARTESIAN_POINT('Ctrl Pts',(-55.7467690853976,-109.139735345023,
178.813912075476));
#28538=CARTESIAN_POINT('Ctrl Pts',(-54.5718594354559,-109.170707334596,
177.6423391512));
#28539=CARTESIAN_POINT('Ctrl Pts',(-54.561921441476,-109.077485562592,175.985484901707));
#28540=CARTESIAN_POINT('Ctrl Pts',(-54.5519834474962,-108.984263790587,
174.328630652215));
#28541=CARTESIAN_POINT('Ctrl Pts',(-55.7070170690958,-108.76684826131,173.157057825983));
#28542=CARTESIAN_POINT('Ctrl Pts',(-56.8620506906954,-108.549432732032,
171.985484999752));
#28543=CARTESIAN_POINT('Ctrl Pts',(-58.4996313148652,-108.280574468435,
171.985485069079));
#28544=CARTESIAN_POINT('Ctrl Pts',(-60.1372119390351,-108.011716204838,
171.985485138407));
#28545=CARTESIAN_POINT('Ctrl Pts',(-61.2922454631428,-107.794300685954,
173.157058062683));
#28546=CARTESIAN_POINT('Ctrl Pts',(-62.4472789872506,-107.57688516707,174.328630986959));
#28547=CARTESIAN_POINT('Ctrl Pts',(-62.4373408553964,-107.483663409764,
175.985485236451));
#28548=CARTESIAN_POINT('Ctrl Pts',(-62.4274027235423,-107.390441652457,
177.642339485944));
#28549=CARTESIAN_POINT('Ctrl Pts',(-61.2524929761086,-107.421413652424,
178.813912312176));
#28550=CARTESIAN_POINT('Ctrl Pts',(-60.077583228675,-107.452385652391,179.985485138407));
#28551=CARTESIAN_POINT('Ctrl Pts',(-58.4201264786711,-107.534800386677,
179.985485069079));
#28552=CARTESIAN_POINT('Ctrl Pts',(-56.7626697286672,-107.617215120964,
179.985484999752));
#28553=CARTESIAN_POINT('Ctrl Pts',(-55.5877600787254,-107.648187110537,
178.813912075476));
#28554=CARTESIAN_POINT('Ctrl Pts',(-54.4128504287836,-107.67915910011,177.6423391512));
#28555=CARTESIAN_POINT('Ctrl Pts',(-54.4029124348038,-107.585937328106,
175.985484901707));
#28556=CARTESIAN_POINT('Ctrl Pts',(-54.3929744408239,-107.492715556102,
174.328630652215));
#28557=CARTESIAN_POINT('Ctrl Pts',(-55.5480080624235,-107.275300026824,
173.157057825983));
#28558=CARTESIAN_POINT('Ctrl Pts',(-56.7030416840231,-107.057884497547,
171.985484999752));
#28559=CARTESIAN_POINT('Ctrl Pts',(-58.340622308193,-106.78902623395,171.985485069079));
#28560=CARTESIAN_POINT('Ctrl Pts',(-59.9782029323629,-106.520167970353,
171.985485138407));
#28561=CARTESIAN_POINT('Ctrl Pts',(-61.1332364564706,-106.302752451468,
173.157058062683));
#28562=CARTESIAN_POINT('Ctrl Pts',(-62.2882699805784,-106.085336932584,
174.328630986959));
#28563=CARTESIAN_POINT('Ctrl Pts',(-62.2783318487242,-105.992115175278,
175.985485236451));
#28564=CARTESIAN_POINT('Ctrl Pts',(-62.26839371687,-105.898893417972,177.642339485944));
#28565=CARTESIAN_POINT('Ctrl Pts',(-61.0934839694364,-105.929865417939,
178.813912312176));
#28566=CARTESIAN_POINT('Ctrl Pts',(-59.9185742220028,-105.960837417905,
179.985485138407));
#28567=CARTESIAN_POINT('Ctrl Pts',(-58.2611174719989,-106.043252152192,
179.985485069079));
#28568=CARTESIAN_POINT('Ctrl Pts',(-56.603660721995,-106.125666886478,179.985484999752));
#28569=CARTESIAN_POINT('Ctrl Pts',(-55.4287510720532,-106.156638876051,
178.813912075476));
#28570=CARTESIAN_POINT('Ctrl Pts',(-54.2538414221114,-106.187610865625,
177.6423391512));
#28571=CARTESIAN_POINT('Ctrl Pts',(-54.2439034281315,-106.09438909362,175.985484901707));
#28572=CARTESIAN_POINT('Ctrl Pts',(-54.2339654341517,-106.001167321616,
174.328630652215));
#28573=CARTESIAN_POINT('Ctrl Pts',(-55.3889990557513,-105.783751792338,
173.157057825983));
#28574=CARTESIAN_POINT('Ctrl Pts',(-56.5440326773509,-105.566336263061,
171.985484999752));
#28575=CARTESIAN_POINT('Ctrl Pts',(-58.1816133015208,-105.297477999464,
171.985485069079));
#28576=CARTESIAN_POINT('Ctrl Pts',(-59.8191939256906,-105.028619735867,
171.985485138407));
#28577=CARTESIAN_POINT('Ctrl Pts',(-60.9742274497984,-104.811204216983,
173.157058062683));
#28578=CARTESIAN_POINT('Ctrl Pts',(-62.1292609739061,-104.593788698099,
174.328630986959));
#28579=CARTESIAN_POINT('Ctrl Pts',(-62.119322842052,-104.500566940792,175.985485236451));
#28580=CARTESIAN_POINT('Ctrl Pts',(-62.1093847101978,-104.407345183486,
177.642339485944));
#28581=CARTESIAN_POINT('Ctrl Pts',(-60.9344749627642,-104.438317183453,
178.813912312176));
#28582=CARTESIAN_POINT('Ctrl Pts',(-59.7595652153305,-104.46928918342,179.985485138407));
#28583=CARTESIAN_POINT('Ctrl Pts',(-58.1021084653266,-104.551703917706,
179.985485069079));
#28584=CARTESIAN_POINT('Ctrl Pts',(-56.4446517153227,-104.634118651992,
179.985484999752));
#28585=CARTESIAN_POINT('Ctrl Pts',(-55.269742065381,-104.665090641566,178.813912075476));
#28586=CARTESIAN_POINT('Ctrl Pts',(-54.0948324154392,-104.696062631139,
177.6423391512));
#28587=CARTESIAN_POINT('Ctrl Pts',(-54.0848944214593,-104.602840859135,
175.985484901707));
#28588=CARTESIAN_POINT('Ctrl Pts',(-54.0749564274795,-104.50961908713,174.328630652215));
#28589=CARTESIAN_POINT('Ctrl Pts',(-55.2299900490791,-104.292203557853,
173.157057825983));
#28590=CARTESIAN_POINT('Ctrl Pts',(-56.3850236706787,-104.074788028575,
171.985484999752));
#28591=CARTESIAN_POINT('Ctrl Pts',(-58.0226042948486,-103.805929764978,
171.985485069079));
#28592=CARTESIAN_POINT('Ctrl Pts',(-59.6601849190184,-103.537071501381,
171.985485138407));
#28593=CARTESIAN_POINT('Ctrl Pts',(-60.8152184431262,-103.319655982497,
173.157058062683));
#28594=CARTESIAN_POINT('Ctrl Pts',(-61.9702519672339,-103.102240463613,
174.328630986959));
#28595=CARTESIAN_POINT('Ctrl Pts',(-61.9603138353797,-103.009018706307,
175.985485236451));
#28596=CARTESIAN_POINT('Ctrl Pts',(-61.9503757035256,-102.915796949001,
177.642339485944));
#28597=CARTESIAN_POINT('Ctrl Pts',(-60.7754659560919,-102.946768948967,
178.813912312176));
#28598=CARTESIAN_POINT('Ctrl Pts',(-59.6005562086583,-102.977740948934,
179.985485138407));
#28599=CARTESIAN_POINT('Ctrl Pts',(-57.9430994586544,-103.06015568322,179.985485069079));
#28600=CARTESIAN_POINT('Ctrl Pts',(-56.2856427086505,-103.142570417507,
179.985484999752));
#28601=CARTESIAN_POINT('Ctrl Pts',(-55.1107330587087,-103.17354240708,178.813912075476));
#28602=CARTESIAN_POINT('Ctrl Pts',(-53.935823408767,-103.204514396654,177.6423391512));
#28603=CARTESIAN_POINT('Ctrl Pts',(-53.9258854147871,-103.111292624649,
175.985484901707));
#28604=CARTESIAN_POINT('Ctrl Pts',(-53.9159474208072,-103.018070852645,
174.328630652215));
#28605=CARTESIAN_POINT('Ctrl Pts',(-55.0709810424069,-102.800655323367,
173.157057825983));
#28606=CARTESIAN_POINT('Ctrl Pts',(-56.2260146640065,-102.58323979409,171.985484999752));
#28607=CARTESIAN_POINT('Ctrl Pts',(-57.8635952881763,-102.314381530493,
171.985485069079));
#28608=CARTESIAN_POINT('Ctrl Pts',(-59.5011759123462,-102.045523266896,
171.985485138407));
#28609=CARTESIAN_POINT('Ctrl Pts',(-60.6562094364539,-101.828107748012,
173.157058062683));
#28610=CARTESIAN_POINT('Ctrl Pts',(-61.8112429605617,-101.610692229127,
174.328630986959));
#28611=CARTESIAN_POINT('Ctrl Pts',(-61.8013048287075,-101.517470471821,
175.985485236451));
#28612=CARTESIAN_POINT('Ctrl Pts',(-61.7913666968533,-101.424248714515,
177.642339485944));
#28613=CARTESIAN_POINT('Ctrl Pts',(-60.6164569494197,-101.455220714482,
178.813912312176));
#28614=CARTESIAN_POINT('Ctrl Pts',(-59.4415472019861,-101.486192714449,
179.985485138407));
#28615=CARTESIAN_POINT('Ctrl Pts',(-57.7840904519822,-101.568607448735,
179.985485069079));
#28616=CARTESIAN_POINT('Ctrl Pts',(-56.1266337019783,-101.651022183021,
179.985484999752));
#28617=CARTESIAN_POINT('Ctrl Pts',(-54.9517240520365,-101.681994172595,
178.813912075476));
#28618=CARTESIAN_POINT('Ctrl Pts',(-53.7768144020947,-101.712966162168,
177.6423391512));
#28619=CARTESIAN_POINT('Ctrl Pts',(-53.7668764081149,-101.619744390164,
175.985484901707));
#28620=CARTESIAN_POINT('Ctrl Pts',(-53.756938414135,-101.526522618159,174.328630652215));
#28621=CARTESIAN_POINT('Ctrl Pts',(-54.9119720357346,-101.309107088882,
173.157057825983));
#28622=CARTESIAN_POINT('Ctrl Pts',(-56.0670056573342,-101.091691559604,
171.985484999752));
#28623=CARTESIAN_POINT('Ctrl Pts',(-57.7045862815041,-100.822833296007,
171.985485069079));
#28624=CARTESIAN_POINT('Ctrl Pts',(-59.342166905674,-100.55397503241,171.985485138407));
#28625=CARTESIAN_POINT('Ctrl Pts',(-60.4972004297817,-100.336559513526,
173.157058062683));
#28626=CARTESIAN_POINT('Ctrl Pts',(-61.6522339538895,-100.119143994642,
174.328630986959));
#28627=CARTESIAN_POINT('Ctrl Pts',(-61.6422958220353,-100.025922237336,
175.985485236451));
#28628=CARTESIAN_POINT('Ctrl Pts',(-61.6323576901811,-99.9327004800294,
177.642339485944));
#28629=CARTESIAN_POINT('Ctrl Pts',(-60.4574479427475,-99.9636724799962,
178.813912312176));
#28630=CARTESIAN_POINT('Ctrl Pts',(-59.2825381953138,-99.994644479963,179.985485138407));
#28631=CARTESIAN_POINT('Ctrl Pts',(-57.6250814453099,-100.077059214249,
179.985485069079));
#28632=CARTESIAN_POINT('Ctrl Pts',(-55.9676246953061,-100.159473948536,
179.985484999752));
#28633=CARTESIAN_POINT('Ctrl Pts',(-54.7927150453643,-100.190445938109,
178.813912075476));
#28634=CARTESIAN_POINT('Ctrl Pts',(-53.6178053954225,-100.221417927683,
177.6423391512));
#28635=CARTESIAN_POINT('Ctrl Pts',(-53.6078674014426,-100.128196155678,
175.985484901707));
#28636=CARTESIAN_POINT('Ctrl Pts',(-53.5979294074628,-100.034974383673,
174.328630652215));
#28637=CARTESIAN_POINT('Ctrl Pts',(-54.7529630290624,-99.817558854396,173.157057825983));
#28638=CARTESIAN_POINT('Ctrl Pts',(-55.907996650662,-99.6001433251185,171.985484999752));
#28639=CARTESIAN_POINT('Ctrl Pts',(-57.5455772748319,-99.3312850615215,
171.985485069079));
#28640=CARTESIAN_POINT('Ctrl Pts',(-59.1831578990017,-99.0624267979246,
171.985485138407));
#28641=CARTESIAN_POINT('Ctrl Pts',(-60.3381914231095,-98.8450112790404,
173.157058062683));
#28642=CARTESIAN_POINT('Ctrl Pts',(-61.4932249472172,-98.6275957601562,
174.328630986959));
#28643=CARTESIAN_POINT('Ctrl Pts',(-61.4832868153631,-98.53437400285,175.985485236451));
#28644=CARTESIAN_POINT('Ctrl Pts',(-61.4733486835089,-98.4411522455438,
177.642339485944));
#28645=CARTESIAN_POINT('Ctrl Pts',(-60.2984389360752,-98.4721242455106,
178.813912312176));
#28646=CARTESIAN_POINT('Ctrl Pts',(-59.1235291886416,-98.5030962454774,
179.985485138407));
#28647=CARTESIAN_POINT('Ctrl Pts',(-57.4660724386377,-98.5855109797636,
179.985485069079));
#28648=CARTESIAN_POINT('Ctrl Pts',(-55.8086156886338,-98.6679257140499,
179.985484999752));
#28649=CARTESIAN_POINT('Ctrl Pts',(-54.633706038692,-98.6988977036234,178.813912075476));
#28650=CARTESIAN_POINT('Ctrl Pts',(-56.2237961054143,-113.614380048479,
178.813912075476));
#28651=CARTESIAN_POINT('Ctrl Pts',(-55.0488864554725,-113.645352038053,
177.6423391512));
#28652=CARTESIAN_POINT('Ctrl Pts',(-55.0389484614927,-113.552130266048,
175.985484901707));
#28653=CARTESIAN_POINT('Ctrl Pts',(-55.0290104675128,-113.458908494044,
174.328630652215));
#28654=CARTESIAN_POINT('Ctrl Pts',(-56.1840440891124,-113.241492964766,
173.157057825983));
#28655=CARTESIAN_POINT('Ctrl Pts',(-57.3390777107121,-113.024077435489,
171.985484999752));
#28656=CARTESIAN_POINT('Ctrl Pts',(-58.9766583348819,-112.755219171892,
171.985485069079));
#28657=CARTESIAN_POINT('Ctrl Pts',(-60.6142389590518,-112.486360908295,
171.985485138407));
#28658=CARTESIAN_POINT('Ctrl Pts',(-61.7692724831595,-112.268945389411,
173.157058062683));
#28659=CARTESIAN_POINT('Ctrl Pts',(-62.9243060072673,-112.051529870527,
174.328630986959));
#28660=CARTESIAN_POINT('Ctrl Pts',(-62.9143678754131,-111.95830811322,175.985485236451));
#28661=CARTESIAN_POINT('Ctrl Pts',(-62.9044297435589,-111.865086355914,
177.642339485944));
#28662=CARTESIAN_POINT('Ctrl Pts',(-61.7295199961253,-111.896058355881,
178.813912312176));
#28663=CARTESIAN_POINT('Ctrl Pts',(-60.5546102486917,-111.927030355848,
179.985485138407));
#28664=CARTESIAN_POINT('Ctrl Pts',(-58.8971534986878,-112.009445090134,
179.985485069079));
#28665=CARTESIAN_POINT('Ctrl Pts',(-57.2396967486839,-112.09185982442,179.985484999752));
#28666=CARTESIAN_POINT('Ctrl Pts',(-56.0647870987421,-112.122831813994,
178.813912075476));
#28667=CARTESIAN_POINT('Ctrl Pts',(-54.8898774488003,-112.153803803567,
177.6423391512));
#28668=CARTESIAN_POINT('Ctrl Pts',(-54.8799394548205,-112.060582031563,
175.985484901707));
#28669=CARTESIAN_POINT('Ctrl Pts',(-54.8700014608406,-111.967360259558,
174.328630652215));
#28670=CARTESIAN_POINT('Ctrl Pts',(-56.0250350824402,-111.749944730281,
173.157057825983));
#28671=CARTESIAN_POINT('Ctrl Pts',(-57.1800687040398,-111.532529201003,
171.985484999752));
#28672=CARTESIAN_POINT('Ctrl Pts',(-58.8176493282097,-111.263670937406,
171.985485069079));
#28673=CARTESIAN_POINT('Ctrl Pts',(-60.4552299523796,-110.994812673809,
171.985485138407));
#28674=CARTESIAN_POINT('Ctrl Pts',(-61.6102634764873,-110.777397154925,
173.157058062683));
#28675=CARTESIAN_POINT('Ctrl Pts',(-62.7652970005951,-110.559981636041,
174.328630986959));
#28676=CARTESIAN_POINT('Ctrl Pts',(-62.7553588687409,-110.466759878735,
175.985485236451));
#28677=CARTESIAN_POINT('Ctrl Pts',(-62.7454207368867,-110.373538121429,
177.642339485944));
#28678=CARTESIAN_POINT('Ctrl Pts',(-61.5705109894531,-110.404510121395,
178.813912312176));
#28679=CARTESIAN_POINT('Ctrl Pts',(-60.3956012420194,-110.435482121362,
179.985485138407));
#28680=CARTESIAN_POINT('Ctrl Pts',(-58.7381444920155,-110.517896855648,
179.985485069079));
#28681=CARTESIAN_POINT('Ctrl Pts',(-57.0806877420116,-110.600311589935,
179.985484999752));
#28682=CARTESIAN_POINT('Ctrl Pts',(-55.9057780920699,-110.631283579508,
178.813912075476));
#28683=CARTESIAN_POINT('Ctrl Pts',(-54.7308684421281,-110.662255569082,
177.6423391512));
#28684=CARTESIAN_POINT('Ctrl Pts',(-54.7209304481482,-110.569033797077,
175.985484901707));
#28685=CARTESIAN_POINT('Ctrl Pts',(-54.7109924541684,-110.475812025073,
174.328630652215));
#28686=CARTESIAN_POINT('Ctrl Pts',(-55.866026075768,-110.258396495795,173.157057825983));
#28687=CARTESIAN_POINT('Ctrl Pts',(-57.0210596973676,-110.040980966518,
171.985484999752));
#28688=CARTESIAN_POINT('Ctrl Pts',(-58.6586403215375,-109.772122702921,
171.985485069079));
#28689=CARTESIAN_POINT('Ctrl Pts',(-60.2962209457073,-109.503264439324,
171.985485138407));
#28690=CARTESIAN_POINT('Ctrl Pts',(-61.4512544698151,-109.28584892044,173.157058062683));
#28691=CARTESIAN_POINT('Ctrl Pts',(-62.6062879939228,-109.068433401555,
174.328630986959));
#28692=CARTESIAN_POINT('Ctrl Pts',(-62.5963498620687,-108.975211644249,
175.985485236451));
#28693=CARTESIAN_POINT('Ctrl Pts',(-62.5864117302145,-108.881989886943,
177.642339485944));
#28694=CARTESIAN_POINT('Ctrl Pts',(-61.4115019827808,-108.91296188691,178.813912312176));
#28695=CARTESIAN_POINT('Ctrl Pts',(-60.2365922353472,-108.943933886877,
179.985485138407));
#28696=CARTESIAN_POINT('Ctrl Pts',(-58.5791354853433,-109.026348621163,
179.985485069079));
#28697=CARTESIAN_POINT('Ctrl Pts',(-56.9216787353394,-109.108763355449,
179.985484999752));
#28698=CARTESIAN_POINT('Ctrl Pts',(-55.7467690853976,-109.139735345023,
178.813912075476));
#28699=CARTESIAN_POINT('Ctrl Pts',(-54.5718594354559,-109.170707334596,
177.6423391512));
#28700=CARTESIAN_POINT('Ctrl Pts',(-54.561921441476,-109.077485562592,175.985484901707));
#28701=CARTESIAN_POINT('Ctrl Pts',(-54.5519834474962,-108.984263790587,
174.328630652215));
#28702=CARTESIAN_POINT('Ctrl Pts',(-55.7070170690958,-108.76684826131,173.157057825983));
#28703=CARTESIAN_POINT('Ctrl Pts',(-56.8620506906954,-108.549432732032,
171.985484999752));
#28704=CARTESIAN_POINT('Ctrl Pts',(-58.4996313148652,-108.280574468435,
171.985485069079));
#28705=CARTESIAN_POINT('Ctrl Pts',(-60.1372119390351,-108.011716204838,
171.985485138407));
#28706=CARTESIAN_POINT('Ctrl Pts',(-61.2922454631428,-107.794300685954,
173.157058062683));
#28707=CARTESIAN_POINT('Ctrl Pts',(-62.4472789872506,-107.57688516707,174.328630986959));
#28708=CARTESIAN_POINT('Ctrl Pts',(-62.4373408553964,-107.483663409764,
175.985485236451));
#28709=CARTESIAN_POINT('Ctrl Pts',(-62.4274027235423,-107.390441652457,
177.642339485944));
#28710=CARTESIAN_POINT('Ctrl Pts',(-61.2524929761086,-107.421413652424,
178.813912312176));
#28711=CARTESIAN_POINT('Ctrl Pts',(-60.077583228675,-107.452385652391,179.985485138407));
#28712=CARTESIAN_POINT('Ctrl Pts',(-58.4201264786711,-107.534800386677,
179.985485069079));
#28713=CARTESIAN_POINT('Ctrl Pts',(-56.7626697286672,-107.617215120964,
179.985484999752));
#28714=CARTESIAN_POINT('Ctrl Pts',(-55.5877600787254,-107.648187110537,
178.813912075476));
#28715=CARTESIAN_POINT('Ctrl Pts',(-54.4128504287836,-107.67915910011,177.6423391512));
#28716=CARTESIAN_POINT('Ctrl Pts',(-54.4029124348038,-107.585937328106,
175.985484901707));
#28717=CARTESIAN_POINT('Ctrl Pts',(-54.3929744408239,-107.492715556102,
174.328630652215));
#28718=CARTESIAN_POINT('Ctrl Pts',(-55.5480080624235,-107.275300026824,
173.157057825983));
#28719=CARTESIAN_POINT('Ctrl Pts',(-56.7030416840231,-107.057884497547,
171.985484999752));
#28720=CARTESIAN_POINT('Ctrl Pts',(-58.340622308193,-106.78902623395,171.985485069079));
#28721=CARTESIAN_POINT('Ctrl Pts',(-59.9782029323629,-106.520167970353,
171.985485138407));
#28722=CARTESIAN_POINT('Ctrl Pts',(-61.1332364564706,-106.302752451468,
173.157058062683));
#28723=CARTESIAN_POINT('Ctrl Pts',(-62.2882699805784,-106.085336932584,
174.328630986959));
#28724=CARTESIAN_POINT('Ctrl Pts',(-62.2783318487242,-105.992115175278,
175.985485236451));
#28725=CARTESIAN_POINT('Ctrl Pts',(-62.26839371687,-105.898893417972,177.642339485944));
#28726=CARTESIAN_POINT('Ctrl Pts',(-61.0934839694364,-105.929865417939,
178.813912312176));
#28727=CARTESIAN_POINT('Ctrl Pts',(-59.9185742220028,-105.960837417905,
179.985485138407));
#28728=CARTESIAN_POINT('Ctrl Pts',(-58.2611174719989,-106.043252152192,
179.985485069079));
#28729=CARTESIAN_POINT('Ctrl Pts',(-56.603660721995,-106.125666886478,179.985484999752));
#28730=CARTESIAN_POINT('Ctrl Pts',(-55.4287510720532,-106.156638876051,
178.813912075476));
#28731=CARTESIAN_POINT('Ctrl Pts',(-54.2538414221114,-106.187610865625,
177.6423391512));
#28732=CARTESIAN_POINT('Ctrl Pts',(-54.2439034281315,-106.09438909362,175.985484901707));
#28733=CARTESIAN_POINT('Ctrl Pts',(-54.2339654341517,-106.001167321616,
174.328630652215));
#28734=CARTESIAN_POINT('Ctrl Pts',(-55.3889990557513,-105.783751792338,
173.157057825983));
#28735=CARTESIAN_POINT('Ctrl Pts',(-56.5440326773509,-105.566336263061,
171.985484999752));
#28736=CARTESIAN_POINT('Ctrl Pts',(-58.1816133015208,-105.297477999464,
171.985485069079));
#28737=CARTESIAN_POINT('Ctrl Pts',(-59.8191939256906,-105.028619735867,
171.985485138407));
#28738=CARTESIAN_POINT('Ctrl Pts',(-60.9742274497984,-104.811204216983,
173.157058062683));
#28739=CARTESIAN_POINT('Ctrl Pts',(-62.1292609739061,-104.593788698099,
174.328630986959));
#28740=CARTESIAN_POINT('Ctrl Pts',(-62.119322842052,-104.500566940792,175.985485236451));
#28741=CARTESIAN_POINT('Ctrl Pts',(-62.1093847101978,-104.407345183486,
177.642339485944));
#28742=CARTESIAN_POINT('Ctrl Pts',(-60.9344749627642,-104.438317183453,
178.813912312176));
#28743=CARTESIAN_POINT('Ctrl Pts',(-59.7595652153305,-104.46928918342,179.985485138407));
#28744=CARTESIAN_POINT('Ctrl Pts',(-58.1021084653266,-104.551703917706,
179.985485069079));
#28745=CARTESIAN_POINT('Ctrl Pts',(-56.4446517153227,-104.634118651992,
179.985484999752));
#28746=CARTESIAN_POINT('Ctrl Pts',(-55.269742065381,-104.665090641566,178.813912075476));
#28747=CARTESIAN_POINT('Ctrl Pts',(-54.0948324154392,-104.696062631139,
177.6423391512));
#28748=CARTESIAN_POINT('Ctrl Pts',(-54.0848944214593,-104.602840859135,
175.985484901707));
#28749=CARTESIAN_POINT('Ctrl Pts',(-54.0749564274795,-104.50961908713,174.328630652215));
#28750=CARTESIAN_POINT('Ctrl Pts',(-55.2299900490791,-104.292203557853,
173.157057825983));
#28751=CARTESIAN_POINT('Ctrl Pts',(-56.3850236706787,-104.074788028575,
171.985484999752));
#28752=CARTESIAN_POINT('Ctrl Pts',(-58.0226042948486,-103.805929764978,
171.985485069079));
#28753=CARTESIAN_POINT('Ctrl Pts',(-59.6601849190184,-103.537071501381,
171.985485138407));
#28754=CARTESIAN_POINT('Ctrl Pts',(-60.8152184431262,-103.319655982497,
173.157058062683));
#28755=CARTESIAN_POINT('Ctrl Pts',(-61.9702519672339,-103.102240463613,
174.328630986959));
#28756=CARTESIAN_POINT('Ctrl Pts',(-61.9603138353797,-103.009018706307,
175.985485236451));
#28757=CARTESIAN_POINT('Ctrl Pts',(-61.9503757035256,-102.915796949001,
177.642339485944));
#28758=CARTESIAN_POINT('Ctrl Pts',(-60.7754659560919,-102.946768948967,
178.813912312176));
#28759=CARTESIAN_POINT('Ctrl Pts',(-59.6005562086583,-102.977740948934,
179.985485138407));
#28760=CARTESIAN_POINT('Ctrl Pts',(-57.9430994586544,-103.06015568322,179.985485069079));
#28761=CARTESIAN_POINT('Ctrl Pts',(-56.2856427086505,-103.142570417507,
179.985484999752));
#28762=CARTESIAN_POINT('Ctrl Pts',(-55.1107330587087,-103.17354240708,178.813912075476));
#28763=CARTESIAN_POINT('Ctrl Pts',(-53.935823408767,-103.204514396654,177.6423391512));
#28764=CARTESIAN_POINT('Ctrl Pts',(-53.9258854147871,-103.111292624649,
175.985484901707));
#28765=CARTESIAN_POINT('Ctrl Pts',(-53.9159474208072,-103.018070852645,
174.328630652215));
#28766=CARTESIAN_POINT('Ctrl Pts',(-55.0709810424069,-102.800655323367,
173.157057825983));
#28767=CARTESIAN_POINT('Ctrl Pts',(-56.2260146640065,-102.58323979409,171.985484999752));
#28768=CARTESIAN_POINT('Ctrl Pts',(-57.8635952881763,-102.314381530493,
171.985485069079));
#28769=CARTESIAN_POINT('Ctrl Pts',(-59.5011759123462,-102.045523266896,
171.985485138407));
#28770=CARTESIAN_POINT('Ctrl Pts',(-60.6562094364539,-101.828107748012,
173.157058062683));
#28771=CARTESIAN_POINT('Ctrl Pts',(-61.8112429605617,-101.610692229127,
174.328630986959));
#28772=CARTESIAN_POINT('Ctrl Pts',(-61.8013048287075,-101.517470471821,
175.985485236451));
#28773=CARTESIAN_POINT('Ctrl Pts',(-61.7913666968533,-101.424248714515,
177.642339485944));
#28774=CARTESIAN_POINT('Ctrl Pts',(-60.6164569494197,-101.455220714482,
178.813912312176));
#28775=CARTESIAN_POINT('Ctrl Pts',(-59.4415472019861,-101.486192714449,
179.985485138407));
#28776=CARTESIAN_POINT('Ctrl Pts',(-57.7840904519822,-101.568607448735,
179.985485069079));
#28777=CARTESIAN_POINT('Ctrl Pts',(-56.1266337019783,-101.651022183021,
179.985484999752));
#28778=CARTESIAN_POINT('Ctrl Pts',(-54.9517240520365,-101.681994172595,
178.813912075476));
#28779=CARTESIAN_POINT('Ctrl Pts',(-53.7768144020947,-101.712966162168,
177.6423391512));
#28780=CARTESIAN_POINT('Ctrl Pts',(-53.7668764081149,-101.619744390164,
175.985484901707));
#28781=CARTESIAN_POINT('Ctrl Pts',(-53.756938414135,-101.526522618159,174.328630652215));
#28782=CARTESIAN_POINT('Ctrl Pts',(-54.9119720357346,-101.309107088882,
173.157057825983));
#28783=CARTESIAN_POINT('Ctrl Pts',(-56.0670056573342,-101.091691559604,
171.985484999752));
#28784=CARTESIAN_POINT('Ctrl Pts',(-57.7045862815041,-100.822833296007,
171.985485069079));
#28785=CARTESIAN_POINT('Ctrl Pts',(-59.342166905674,-100.55397503241,171.985485138407));
#28786=CARTESIAN_POINT('Ctrl Pts',(-60.4972004297817,-100.336559513526,
173.157058062683));
#28787=CARTESIAN_POINT('Ctrl Pts',(-61.6522339538895,-100.119143994642,
174.328630986959));
#28788=CARTESIAN_POINT('Ctrl Pts',(-61.6422958220353,-100.025922237336,
175.985485236451));
#28789=CARTESIAN_POINT('Ctrl Pts',(-61.6323576901811,-99.9327004800294,
177.642339485944));
#28790=CARTESIAN_POINT('Ctrl Pts',(-60.4574479427475,-99.9636724799962,
178.813912312176));
#28791=CARTESIAN_POINT('Ctrl Pts',(-59.2825381953138,-99.994644479963,179.985485138407));
#28792=CARTESIAN_POINT('Ctrl Pts',(-57.6250814453099,-100.077059214249,
179.985485069079));
#28793=CARTESIAN_POINT('Ctrl Pts',(-55.9676246953061,-100.159473948536,
179.985484999752));
#28794=CARTESIAN_POINT('Ctrl Pts',(-54.7927150453643,-100.190445938109,
178.813912075476));
#28795=CARTESIAN_POINT('Ctrl Pts',(-53.6178053954225,-100.221417927683,
177.6423391512));
#28796=CARTESIAN_POINT('Ctrl Pts',(-53.6078674014426,-100.128196155678,
175.985484901707));
#28797=CARTESIAN_POINT('Ctrl Pts',(-53.5979294074628,-100.034974383673,
174.328630652215));
#28798=CARTESIAN_POINT('Ctrl Pts',(-54.7529630290624,-99.817558854396,173.157057825983));
#28799=CARTESIAN_POINT('Ctrl Pts',(-55.907996650662,-99.6001433251185,171.985484999752));
#28800=CARTESIAN_POINT('Ctrl Pts',(-57.5455772748319,-99.3312850615215,
171.985485069079));
#28801=CARTESIAN_POINT('Ctrl Pts',(-59.1831578990017,-99.0624267979246,
171.985485138407));
#28802=CARTESIAN_POINT('Ctrl Pts',(-60.3381914231095,-98.8450112790404,
173.157058062683));
#28803=CARTESIAN_POINT('Ctrl Pts',(-61.4932249472172,-98.6275957601562,
174.328630986959));
#28804=CARTESIAN_POINT('Ctrl Pts',(-61.4832868153631,-98.53437400285,175.985485236451));
#28805=CARTESIAN_POINT('Ctrl Pts',(-61.4733486835089,-98.4411522455438,
177.642339485944));
#28806=CARTESIAN_POINT('Ctrl Pts',(-60.2984389360752,-98.4721242455106,
178.813912312176));
#28807=CARTESIAN_POINT('Ctrl Pts',(-59.1235291886416,-98.5030962454774,
179.985485138407));
#28808=CARTESIAN_POINT('Ctrl Pts',(-57.4660724386377,-98.5855109797636,
179.985485069079));
#28809=CARTESIAN_POINT('Ctrl Pts',(-55.8086156886338,-98.6679257140499,
179.985484999752));
#28810=CARTESIAN_POINT('Ctrl Pts',(-54.633706038692,-98.6988977036234,178.813912075476));
#28811=CARTESIAN_POINT('Ctrl Pts',(-56.9964983346804,-113.864655531781,
178.072094410988));
#28812=CARTESIAN_POINT('Ctrl Pts',(-56.1271283009022,-113.863054956993,
177.207792449865));
#28813=CARTESIAN_POINT('Ctrl Pts',(-56.117190288842,-113.769833186916,175.985484945604));
#28814=CARTESIAN_POINT('Ctrl Pts',(-56.1072522767819,-113.676611416839,
174.763177441344));
#28815=CARTESIAN_POINT('Ctrl Pts',(-56.9567462566485,-113.491768454648,
173.89887555255));
#28816=CARTESIAN_POINT('Ctrl Pts',(-57.8062402365152,-113.306925492458,
173.034573663757));
#28817=CARTESIAN_POINT('Ctrl Pts',(-59.011722573584,-113.084131793069,173.034573714903));
#28818=CARTESIAN_POINT('Ctrl Pts',(-60.2172049106529,-112.86133809368,173.034573766048));
#28819=CARTESIAN_POINT('Ctrl Pts',(-61.0666988185971,-112.676495139156,
173.898875727171));
#28820=CARTESIAN_POINT('Ctrl Pts',(-61.9161927265413,-112.491652184633,
174.763177688294));
#28821=CARTESIAN_POINT('Ctrl Pts',(-61.9062546127674,-112.398430425399,
175.985485192554));
#28822=CARTESIAN_POINT('Ctrl Pts',(-61.8963164989935,-112.305208666166,
177.207792696815));
#28823=CARTESIAN_POINT('Ctrl Pts',(-61.0269463932928,-112.303608099046,
178.072094585608));
#28824=CARTESIAN_POINT('Ctrl Pts',(-60.1575762875921,-112.302007531926,
178.936396474401));
#28825=CARTESIAN_POINT('Ctrl Pts',(-58.9322178246893,-112.338357702004,
178.936396423256));
#28826=CARTESIAN_POINT('Ctrl Pts',(-57.7068593617864,-112.374707872082,
178.936396372111));
#28827=CARTESIAN_POINT('Ctrl Pts',(-56.8374893280082,-112.373107297295,
178.072094410988));
#28828=CARTESIAN_POINT('Ctrl Pts',(-55.9681192942299,-112.371506722508,
177.207792449865));
#28829=CARTESIAN_POINT('Ctrl Pts',(-55.9581812821698,-112.278284952431,
175.985484945604));
#28830=CARTESIAN_POINT('Ctrl Pts',(-55.9482432701096,-112.185063182354,
174.763177441344));
#28831=CARTESIAN_POINT('Ctrl Pts',(-56.7977372499763,-112.000220220163,
173.89887555255));
#28832=CARTESIAN_POINT('Ctrl Pts',(-57.647231229843,-111.815377257972,173.034573663757));
#28833=CARTESIAN_POINT('Ctrl Pts',(-58.8527135669118,-111.592583558583,
173.034573714903));
#28834=CARTESIAN_POINT('Ctrl Pts',(-60.0581959039807,-111.369789859194,
173.034573766048));
#28835=CARTESIAN_POINT('Ctrl Pts',(-60.9076898119249,-111.184946904671,
173.898875727171));
#28836=CARTESIAN_POINT('Ctrl Pts',(-61.7571837198691,-111.000103950148,
174.763177688294));
#28837=CARTESIAN_POINT('Ctrl Pts',(-61.7472456060952,-110.906882190914,
175.985485192554));
#28838=CARTESIAN_POINT('Ctrl Pts',(-61.7373074923213,-110.81366043168,177.207792696815));
#28839=CARTESIAN_POINT('Ctrl Pts',(-60.8679373866206,-110.81205986456,178.072094585608));
#28840=CARTESIAN_POINT('Ctrl Pts',(-59.9985672809199,-110.81045929744,178.936396474401));
#28841=CARTESIAN_POINT('Ctrl Pts',(-58.7732088180171,-110.846809467519,
178.936396423256));
#28842=CARTESIAN_POINT('Ctrl Pts',(-57.5478503551142,-110.883159637597,
178.936396372111));
#28843=CARTESIAN_POINT('Ctrl Pts',(-56.6784803213359,-110.881559062809,
178.072094410988));
#28844=CARTESIAN_POINT('Ctrl Pts',(-55.8091102875577,-110.879958488022,
177.207792449865));
#28845=CARTESIAN_POINT('Ctrl Pts',(-55.7991722754976,-110.786736717945,
175.985484945604));
#28846=CARTESIAN_POINT('Ctrl Pts',(-55.7892342634374,-110.693514947868,
174.763177441344));
#28847=CARTESIAN_POINT('Ctrl Pts',(-56.6387282433041,-110.508671985677,
173.89887555255));
#28848=CARTESIAN_POINT('Ctrl Pts',(-57.4882222231708,-110.323829023487,
173.034573663757));
#28849=CARTESIAN_POINT('Ctrl Pts',(-58.6937045602396,-110.101035324098,
173.034573714903));
#28850=CARTESIAN_POINT('Ctrl Pts',(-59.8991868973084,-109.878241624709,
173.034573766048));
#28851=CARTESIAN_POINT('Ctrl Pts',(-60.7486808052526,-109.693398670185,
173.898875727171));
#28852=CARTESIAN_POINT('Ctrl Pts',(-61.5981747131968,-109.508555715662,
174.763177688294));
#28853=CARTESIAN_POINT('Ctrl Pts',(-61.588236599423,-109.415333956428,175.985485192554));
#28854=CARTESIAN_POINT('Ctrl Pts',(-61.5782984856491,-109.322112197195,
177.207792696815));
#28855=CARTESIAN_POINT('Ctrl Pts',(-60.7089283799484,-109.320511630075,
178.072094585608));
#28856=CARTESIAN_POINT('Ctrl Pts',(-59.8395582742477,-109.318911062955,
178.936396474401));
#28857=CARTESIAN_POINT('Ctrl Pts',(-58.6141998113448,-109.355261233033,
178.936396423256));
#28858=CARTESIAN_POINT('Ctrl Pts',(-57.388841348442,-109.391611403111,178.936396372111));
#28859=CARTESIAN_POINT('Ctrl Pts',(-56.5194713146637,-109.390010828324,
178.072094410988));
#28860=CARTESIAN_POINT('Ctrl Pts',(-55.6501012808855,-109.388410253536,
177.207792449865));
#28861=CARTESIAN_POINT('Ctrl Pts',(-55.6401632688253,-109.295188483459,
175.985484945604));
#28862=CARTESIAN_POINT('Ctrl Pts',(-55.6302252567652,-109.201966713382,
174.763177441344));
#28863=CARTESIAN_POINT('Ctrl Pts',(-56.4797192366319,-109.017123751192,
173.89887555255));
#28864=CARTESIAN_POINT('Ctrl Pts',(-57.3292132164985,-108.832280789001,
173.034573663757));
#28865=CARTESIAN_POINT('Ctrl Pts',(-58.5346955535674,-108.609487089612,
173.034573714903));
#28866=CARTESIAN_POINT('Ctrl Pts',(-59.7401778906362,-108.386693390223,
173.034573766048));
#28867=CARTESIAN_POINT('Ctrl Pts',(-60.5896717985804,-108.2018504357,173.898875727171));
#28868=CARTESIAN_POINT('Ctrl Pts',(-61.4391657065246,-108.017007481176,
174.763177688294));
#28869=CARTESIAN_POINT('Ctrl Pts',(-61.4292275927507,-107.923785721943,
175.985485192554));
#28870=CARTESIAN_POINT('Ctrl Pts',(-61.4192894789769,-107.830563962709,
177.207792696815));
#28871=CARTESIAN_POINT('Ctrl Pts',(-60.5499193732762,-107.828963395589,
178.072094585608));
#28872=CARTESIAN_POINT('Ctrl Pts',(-59.6805492675755,-107.827362828469,
178.936396474401));
#28873=CARTESIAN_POINT('Ctrl Pts',(-58.4551908046726,-107.863712998547,
178.936396423256));
#28874=CARTESIAN_POINT('Ctrl Pts',(-57.2298323417698,-107.900063168626,
178.936396372111));
#28875=CARTESIAN_POINT('Ctrl Pts',(-56.3604623079915,-107.898462593838,
178.072094410988));
#28876=CARTESIAN_POINT('Ctrl Pts',(-55.4910922742133,-107.896862019051,
177.207792449865));
#28877=CARTESIAN_POINT('Ctrl Pts',(-55.4811542621531,-107.803640248974,
175.985484945604));
#28878=CARTESIAN_POINT('Ctrl Pts',(-55.471216250093,-107.710418478897,174.763177441344));
#28879=CARTESIAN_POINT('Ctrl Pts',(-56.3207102299596,-107.525575516706,
173.89887555255));
#28880=CARTESIAN_POINT('Ctrl Pts',(-57.1702042098263,-107.340732554515,
173.034573663757));
#28881=CARTESIAN_POINT('Ctrl Pts',(-58.3756865468951,-107.117938855126,
173.034573714903));
#28882=CARTESIAN_POINT('Ctrl Pts',(-59.581168883964,-106.895145155737,173.034573766048));
#28883=CARTESIAN_POINT('Ctrl Pts',(-60.4306627919082,-106.710302201214,
173.898875727171));
#28884=CARTESIAN_POINT('Ctrl Pts',(-61.2801566998524,-106.525459246691,
174.763177688294));
#28885=CARTESIAN_POINT('Ctrl Pts',(-61.2702185860785,-106.432237487457,
175.985485192554));
#28886=CARTESIAN_POINT('Ctrl Pts',(-61.2602804723046,-106.339015728223,
177.207792696815));
#28887=CARTESIAN_POINT('Ctrl Pts',(-60.3909103666039,-106.337415161103,
178.072094585608));
#28888=CARTESIAN_POINT('Ctrl Pts',(-59.5215402609032,-106.335814593983,
178.936396474401));
#28889=CARTESIAN_POINT('Ctrl Pts',(-58.2961817980004,-106.372164764062,
178.936396423256));
#28890=CARTESIAN_POINT('Ctrl Pts',(-57.0708233350975,-106.40851493414,178.936396372111));
#28891=CARTESIAN_POINT('Ctrl Pts',(-56.2014533013193,-106.406914359353,
178.072094410988));
#28892=CARTESIAN_POINT('Ctrl Pts',(-55.332083267541,-106.405313784565,177.207792449865));
#28893=CARTESIAN_POINT('Ctrl Pts',(-55.3221452554809,-106.312092014488,
175.985484945604));
#28894=CARTESIAN_POINT('Ctrl Pts',(-55.3122072434207,-106.218870244411,
174.763177441344));
#28895=CARTESIAN_POINT('Ctrl Pts',(-56.1617012232874,-106.034027282221,
173.89887555255));
#28896=CARTESIAN_POINT('Ctrl Pts',(-57.0111952031541,-105.84918432003,173.034573663757));
#28897=CARTESIAN_POINT('Ctrl Pts',(-58.2166775402229,-105.626390620641,
173.034573714903));
#28898=CARTESIAN_POINT('Ctrl Pts',(-59.4221598772917,-105.403596921252,
173.034573766048));
#28899=CARTESIAN_POINT('Ctrl Pts',(-60.2716537852359,-105.218753966728,
173.898875727171));
#28900=CARTESIAN_POINT('Ctrl Pts',(-61.1211476931802,-105.033911012205,
174.763177688294));
#28901=CARTESIAN_POINT('Ctrl Pts',(-61.1112095794063,-104.940689252971,
175.985485192554));
#28902=CARTESIAN_POINT('Ctrl Pts',(-61.1012714656324,-104.847467493738,
177.207792696815));
#28903=CARTESIAN_POINT('Ctrl Pts',(-60.2319013599317,-104.845866926618,
178.072094585608));
#28904=CARTESIAN_POINT('Ctrl Pts',(-59.362531254231,-104.844266359498,178.936396474401));
#28905=CARTESIAN_POINT('Ctrl Pts',(-58.1371727913281,-104.880616529576,
178.936396423256));
#28906=CARTESIAN_POINT('Ctrl Pts',(-56.9118143284253,-104.916966699654,
178.936396372111));
#28907=CARTESIAN_POINT('Ctrl Pts',(-56.042444294647,-104.915366124867,178.072094410988));
#28908=CARTESIAN_POINT('Ctrl Pts',(-55.1730742608688,-104.91376555008,177.207792449865));
#28909=CARTESIAN_POINT('Ctrl Pts',(-55.1631362488087,-104.820543780003,
175.985484945604));
#28910=CARTESIAN_POINT('Ctrl Pts',(-55.1531982367485,-104.727322009926,
174.763177441344));
#28911=CARTESIAN_POINT('Ctrl Pts',(-56.0026922166152,-104.542479047735,
173.89887555255));
#28912=CARTESIAN_POINT('Ctrl Pts',(-56.8521861964818,-104.357636085544,
173.034573663757));
#28913=CARTESIAN_POINT('Ctrl Pts',(-58.0576685335507,-104.134842386155,
173.034573714903));
#28914=CARTESIAN_POINT('Ctrl Pts',(-59.2631508706195,-103.912048686766,
173.034573766048));
#28915=CARTESIAN_POINT('Ctrl Pts',(-60.1126447785637,-103.727205732243,
173.898875727171));
#28916=CARTESIAN_POINT('Ctrl Pts',(-60.9621386865079,-103.54236277772,174.763177688294));
#28917=CARTESIAN_POINT('Ctrl Pts',(-60.952200572734,-103.449141018486,175.985485192554));
#28918=CARTESIAN_POINT('Ctrl Pts',(-60.9422624589602,-103.355919259252,
177.207792696815));
#28919=CARTESIAN_POINT('Ctrl Pts',(-60.0728923532595,-103.354318692132,
178.072094585608));
#28920=CARTESIAN_POINT('Ctrl Pts',(-59.2035222475588,-103.352718125012,
178.936396474401));
#28921=CARTESIAN_POINT('Ctrl Pts',(-57.9781637846559,-103.389068295091,
178.936396423256));
#28922=CARTESIAN_POINT('Ctrl Pts',(-56.7528053217531,-103.425418465169,
178.936396372111));
#28923=CARTESIAN_POINT('Ctrl Pts',(-55.8834352879748,-103.423817890381,
178.072094410988));
#28924=CARTESIAN_POINT('Ctrl Pts',(-55.0140652541966,-103.422217315594,
177.207792449865));
#28925=CARTESIAN_POINT('Ctrl Pts',(-55.0041272421364,-103.328995545517,
175.985484945604));
#28926=CARTESIAN_POINT('Ctrl Pts',(-54.9941892300763,-103.23577377544,174.763177441344));
#28927=CARTESIAN_POINT('Ctrl Pts',(-55.8436832099429,-103.050930813249,
173.89887555255));
#28928=CARTESIAN_POINT('Ctrl Pts',(-56.6931771898096,-102.866087851059,
173.034573663757));
#28929=CARTESIAN_POINT('Ctrl Pts',(-57.8986595268784,-102.64329415167,173.034573714903));
#28930=CARTESIAN_POINT('Ctrl Pts',(-59.1041418639473,-102.420500452281,
173.034573766048));
#28931=CARTESIAN_POINT('Ctrl Pts',(-59.9536357718915,-102.235657497757,
173.898875727171));
#28932=CARTESIAN_POINT('Ctrl Pts',(-60.8031296798357,-102.050814543234,
174.763177688294));
#28933=CARTESIAN_POINT('Ctrl Pts',(-60.7931915660618,-101.957592784,175.985485192554));
#28934=CARTESIAN_POINT('Ctrl Pts',(-60.783253452288,-101.864371024767,177.207792696815));
#28935=CARTESIAN_POINT('Ctrl Pts',(-59.9138833465873,-101.862770457647,
178.072094585608));
#28936=CARTESIAN_POINT('Ctrl Pts',(-59.0445132408866,-101.861169890527,
178.936396474401));
#28937=CARTESIAN_POINT('Ctrl Pts',(-57.8191547779837,-101.897520060605,
178.936396423256));
#28938=CARTESIAN_POINT('Ctrl Pts',(-56.5937963150808,-101.933870230683,
178.936396372111));
#28939=CARTESIAN_POINT('Ctrl Pts',(-55.7244262813026,-101.932269655896,
178.072094410988));
#28940=CARTESIAN_POINT('Ctrl Pts',(-54.8550562475244,-101.930669081108,
177.207792449865));
#28941=CARTESIAN_POINT('Ctrl Pts',(-54.8451182354642,-101.837447311031,
175.985484945604));
#28942=CARTESIAN_POINT('Ctrl Pts',(-54.8351802234041,-101.744225540954,
174.763177441344));
#28943=CARTESIAN_POINT('Ctrl Pts',(-55.6846742032707,-101.559382578764,
173.89887555255));
#28944=CARTESIAN_POINT('Ctrl Pts',(-56.5341681831374,-101.374539616573,
173.034573663757));
#28945=CARTESIAN_POINT('Ctrl Pts',(-57.7396505202062,-101.151745917184,
173.034573714903));
#28946=CARTESIAN_POINT('Ctrl Pts',(-58.9451328572751,-100.928952217795,
173.034573766048));
#28947=CARTESIAN_POINT('Ctrl Pts',(-59.7946267652193,-100.744109263272,
173.898875727171));
#28948=CARTESIAN_POINT('Ctrl Pts',(-60.6441206731635,-100.559266308748,
174.763177688294));
#28949=CARTESIAN_POINT('Ctrl Pts',(-60.6341825593896,-100.466044549515,
175.985485192554));
#28950=CARTESIAN_POINT('Ctrl Pts',(-60.6242444456157,-100.372822790281,
177.207792696815));
#28951=CARTESIAN_POINT('Ctrl Pts',(-59.754874339915,-100.371222223161,178.072094585608));
#28952=CARTESIAN_POINT('Ctrl Pts',(-58.8855042342143,-100.369621656041,
178.936396474401));
#28953=CARTESIAN_POINT('Ctrl Pts',(-57.6601457713115,-100.405971826119,
178.936396423256));
#28954=CARTESIAN_POINT('Ctrl Pts',(-56.4347873084086,-100.442321996198,
178.936396372111));
#28955=CARTESIAN_POINT('Ctrl Pts',(-55.5654172746304,-100.44072142141,178.072094410988));
#28956=CARTESIAN_POINT('Ctrl Pts',(-54.6960472408521,-100.439120846623,
177.207792449865));
#28957=CARTESIAN_POINT('Ctrl Pts',(-54.686109228792,-100.345899076546,175.985484945604));
#28958=CARTESIAN_POINT('Ctrl Pts',(-54.6761712167318,-100.252677306469,
174.763177441344));
#28959=CARTESIAN_POINT('Ctrl Pts',(-55.5256651965985,-100.067834344278,
173.89887555255));
#28960=CARTESIAN_POINT('Ctrl Pts',(-56.3751591764652,-99.8829913820874,
173.034573663757));
#28961=CARTESIAN_POINT('Ctrl Pts',(-57.580641513534,-99.6601976826983,173.034573714903));
#28962=CARTESIAN_POINT('Ctrl Pts',(-58.7861238506028,-99.4374039833093,
173.034573766048));
#28963=CARTESIAN_POINT('Ctrl Pts',(-59.635617758547,-99.252561028786,173.898875727171));
#28964=CARTESIAN_POINT('Ctrl Pts',(-60.4851116664912,-99.0677180742627,
174.763177688294));
#28965=CARTESIAN_POINT('Ctrl Pts',(-60.4751735527174,-98.9744963150291,
175.985485192554));
#28966=CARTESIAN_POINT('Ctrl Pts',(-60.4652354389435,-98.8812745557954,
177.207792696815));
#28967=CARTESIAN_POINT('Ctrl Pts',(-59.5958653332428,-98.8796739886754,
178.072094585608));
#28968=CARTESIAN_POINT('Ctrl Pts',(-58.7264952275421,-98.8780734215554,
178.936396474401));
#28969=CARTESIAN_POINT('Ctrl Pts',(-57.5011367646392,-98.9144235916337,
178.936396423256));
#28970=CARTESIAN_POINT('Ctrl Pts',(-56.2757783017364,-98.9507737617121,
178.936396372111));
#28971=CARTESIAN_POINT('Ctrl Pts',(-55.4064082679581,-98.9491731869247,
178.072094410988));
#28972=CARTESIAN_POINT('Ctrl Pts',(-61.3885995934693,-105.924024231779,
178.485485069079));
#28973=CARTESIAN_POINT('Ctrl Pts',(-61.2500273891125,-105.925738749657,
178.657813499464));
#28974=CARTESIAN_POINT('Ctrl Pts',(-61.0934839694364,-105.929865417939,
178.813912312176));
#28975=CARTESIAN_POINT('Ctrl Pts',(-59.9185742220028,-105.960837417905,
179.985485138407));
#28976=CARTESIAN_POINT('Ctrl Pts',(-58.2611174719989,-106.043252152192,
179.985485069079));
#28977=CARTESIAN_POINT('Ctrl Pts',(-56.603660721995,-106.125666886478,179.985484999752));
#28978=CARTESIAN_POINT('Ctrl Pts',(-55.4287510720532,-106.156638876051,
178.813912075476));
#28979=CARTESIAN_POINT('Ctrl Pts',(-54.2538414221114,-106.187610865625,
177.6423391512));
#28980=CARTESIAN_POINT('Ctrl Pts',(-54.2439034281315,-106.09438909362,175.985484901707));
#28981=CARTESIAN_POINT('Ctrl Pts',(-54.2339654341517,-106.001167321616,
174.328630652215));
#28982=CARTESIAN_POINT('Ctrl Pts',(-55.3889990557513,-105.783751792338,
173.157057825983));
#28983=CARTESIAN_POINT('Ctrl Pts',(-56.5440326773509,-105.566336263061,
171.985484999752));
#28984=CARTESIAN_POINT('Ctrl Pts',(-58.1816133015208,-105.297477999464,
171.985485069079));
#28985=CARTESIAN_POINT('Ctrl Pts',(-59.8191939256906,-105.028619735867,
171.985485138407));
#28986=CARTESIAN_POINT('Ctrl Pts',(-60.9742274497984,-104.811204216983,
173.157058062683));
#28987=CARTESIAN_POINT('Ctrl Pts',(-61.1281224707516,-104.78223608304,173.313156769748));
#28988=CARTESIAN_POINT('Ctrl Pts',(-61.2639416747223,-104.754698653858,
173.485485069079));
#28989=CARTESIAN_POINT('Ctrl Pts',(-56.8733667677527,-112.709647553905,
178.072094410988));
#28990=CARTESIAN_POINT('Ctrl Pts',(-56.0039967339745,-112.708046979118,
177.207792449865));
#28991=CARTESIAN_POINT('Ctrl Pts',(-55.9940587219143,-112.614825209041,
175.985484945604));
#28992=CARTESIAN_POINT('Ctrl Pts',(-55.9841207098542,-112.521603438964,
174.763177441344));
#28993=CARTESIAN_POINT('Ctrl Pts',(-56.8336146897208,-112.336760476773,
173.89887555255));
#28994=CARTESIAN_POINT('Ctrl Pts',(-57.6831086695875,-112.151917514582,
173.034573663757));
#28995=CARTESIAN_POINT('Ctrl Pts',(-58.8885910066563,-111.929123815193,
173.034573714903));
#28996=CARTESIAN_POINT('Ctrl Pts',(-60.0940733437252,-111.706330115804,
173.034573766048));
#28997=CARTESIAN_POINT('Ctrl Pts',(-60.9435672516694,-111.521487161281,
173.898875727171));
#28998=CARTESIAN_POINT('Ctrl Pts',(-61.7930611596136,-111.336644206758,
174.763177688294));
#28999=CARTESIAN_POINT('Ctrl Pts',(-61.7831230458397,-111.243422447524,
175.985485192554));
#29000=CARTESIAN_POINT('Ctrl Pts',(-61.7731849320658,-111.15020068829,177.207792696815));
#29001=CARTESIAN_POINT('Ctrl Pts',(-60.9038148263651,-111.14860012117,178.072094585608));
#29002=CARTESIAN_POINT('Ctrl Pts',(-60.0344447206644,-111.14699955405,178.936396474401));
#29003=CARTESIAN_POINT('Ctrl Pts',(-58.8090862577616,-111.183349724129,
178.936396423256));
#29004=CARTESIAN_POINT('Ctrl Pts',(-57.5837277948587,-111.219699894207,
178.936396372111));
#29005=CARTESIAN_POINT('Ctrl Pts',(-56.7143577610805,-111.21809931942,178.072094410988));
#29006=CARTESIAN_POINT('Ctrl Pts',(-55.8449877273022,-111.216498744632,
177.207792449865));
#29007=CARTESIAN_POINT('Ctrl Pts',(-55.8350497152421,-111.123276974555,
175.985484945604));
#29008=CARTESIAN_POINT('Ctrl Pts',(-55.8251117031819,-111.030055204478,
174.763177441344));
#29009=CARTESIAN_POINT('Ctrl Pts',(-56.6746056830486,-110.845212242287,
173.89887555255));
#29010=CARTESIAN_POINT('Ctrl Pts',(-57.5240996629153,-110.660369280097,
173.034573663757));
#29011=CARTESIAN_POINT('Ctrl Pts',(-58.7295819999841,-110.437575580708,
173.034573714903));
#29012=CARTESIAN_POINT('Ctrl Pts',(-59.9350643370529,-110.214781881319,
173.034573766048));
#29013=CARTESIAN_POINT('Ctrl Pts',(-60.7845582449971,-110.029938926795,
173.898875727171));
#29014=CARTESIAN_POINT('Ctrl Pts',(-61.6340521529414,-109.845095972272,
174.763177688294));
#29015=CARTESIAN_POINT('Ctrl Pts',(-61.6241140391675,-109.751874213038,
175.985485192554));
#29016=CARTESIAN_POINT('Ctrl Pts',(-61.6141759253936,-109.658652453805,
177.207792696815));
#29017=CARTESIAN_POINT('Ctrl Pts',(-60.7448058196929,-109.657051886685,
178.072094585608));
#29018=CARTESIAN_POINT('Ctrl Pts',(-59.8754357139922,-109.655451319565,
178.936396474401));
#29019=CARTESIAN_POINT('Ctrl Pts',(-58.6500772510893,-109.691801489643,
178.936396423256));
#29020=CARTESIAN_POINT('Ctrl Pts',(-57.4247187881865,-109.728151659721,
178.936396372111));
#29021=CARTESIAN_POINT('Ctrl Pts',(-56.5553487544082,-109.726551084934,
178.072094410988));
#29022=CARTESIAN_POINT('Ctrl Pts',(-55.68597872063,-109.724950510147,177.207792449865));
#29023=CARTESIAN_POINT('Ctrl Pts',(-55.6760407085698,-109.63172874007,175.985484945604));
#29024=CARTESIAN_POINT('Ctrl Pts',(-55.6661026965097,-109.538506969993,
174.763177441344));
#29025=CARTESIAN_POINT('Ctrl Pts',(-56.5155966763764,-109.353664007802,
173.89887555255));
#29026=CARTESIAN_POINT('Ctrl Pts',(-57.365090656243,-109.168821045611,173.034573663757));
#29027=CARTESIAN_POINT('Ctrl Pts',(-58.5705729933119,-108.946027346222,
173.034573714903));
#29028=CARTESIAN_POINT('Ctrl Pts',(-59.7760553303807,-108.723233646833,
173.034573766048));
#29029=CARTESIAN_POINT('Ctrl Pts',(-60.6255492383249,-108.53839069231,173.898875727171));
#29030=CARTESIAN_POINT('Ctrl Pts',(-61.4750431462691,-108.353547737786,
174.763177688294));
#29031=CARTESIAN_POINT('Ctrl Pts',(-61.4651050324952,-108.260325978553,
175.985485192554));
#29032=CARTESIAN_POINT('Ctrl Pts',(-61.4551669187214,-108.167104219319,
177.207792696815));
#29033=CARTESIAN_POINT('Ctrl Pts',(-60.5857968130207,-108.165503652199,
178.072094585608));
#29034=CARTESIAN_POINT('Ctrl Pts',(-59.71642670732,-108.163903085079,178.936396474401));
#29035=CARTESIAN_POINT('Ctrl Pts',(-58.4910682444171,-108.200253255158,
178.936396423256));
#29036=CARTESIAN_POINT('Ctrl Pts',(-57.2657097815143,-108.236603425236,
178.936396372111));
#29037=CARTESIAN_POINT('Ctrl Pts',(-56.396339747736,-108.235002850448,178.072094410988));
#29038=CARTESIAN_POINT('Ctrl Pts',(-55.5269697139578,-108.233402275661,
177.207792449865));
#29039=CARTESIAN_POINT('Ctrl Pts',(-55.5170317018976,-108.140180505584,
175.985484945604));
#29040=CARTESIAN_POINT('Ctrl Pts',(-55.5070936898375,-108.046958735507,
174.763177441344));
#29041=CARTESIAN_POINT('Ctrl Pts',(-56.3565876697041,-107.862115773316,
173.89887555255));
#29042=CARTESIAN_POINT('Ctrl Pts',(-57.2060816495708,-107.677272811126,
173.034573663757));
#29043=CARTESIAN_POINT('Ctrl Pts',(-58.4115639866396,-107.454479111736,
173.034573714903));
#29044=CARTESIAN_POINT('Ctrl Pts',(-59.6170463237085,-107.231685412347,
173.034573766048));
#29045=CARTESIAN_POINT('Ctrl Pts',(-60.4665402316527,-107.046842457824,
173.898875727171));
#29046=CARTESIAN_POINT('Ctrl Pts',(-61.3160341395969,-106.861999503301,
174.763177688294));
#29047=CARTESIAN_POINT('Ctrl Pts',(-61.306096025823,-106.768777744067,175.985485192554));
#29048=CARTESIAN_POINT('Ctrl Pts',(-61.2961579120492,-106.675555984834,
177.207792696815));
#29049=CARTESIAN_POINT('Ctrl Pts',(-60.4267878063484,-106.673955417714,
178.072094585608));
#29050=CARTESIAN_POINT('Ctrl Pts',(-59.5574177006478,-106.672354850594,
178.936396474401));
#29051=CARTESIAN_POINT('Ctrl Pts',(-58.3320592377449,-106.708705020672,
178.936396423256));
#29052=CARTESIAN_POINT('Ctrl Pts',(-57.106700774842,-106.74505519075,178.936396372111));
#29053=CARTESIAN_POINT('Ctrl Pts',(-56.2373307410638,-106.743454615963,
178.072094410988));
#29054=CARTESIAN_POINT('Ctrl Pts',(-55.3679607072856,-106.741854041175,
177.207792449865));
#29055=CARTESIAN_POINT('Ctrl Pts',(-55.3580226952254,-106.648632271098,
175.985484945604));
#29056=CARTESIAN_POINT('Ctrl Pts',(-55.3480846831652,-106.555410501021,
174.763177441344));
#29057=CARTESIAN_POINT('Ctrl Pts',(-56.1975786630319,-106.370567538831,
173.89887555255));
#29058=CARTESIAN_POINT('Ctrl Pts',(-57.0470726428986,-106.18572457664,173.034573663757));
#29059=CARTESIAN_POINT('Ctrl Pts',(-58.2525549799674,-105.962930877251,
173.034573714903));
#29060=CARTESIAN_POINT('Ctrl Pts',(-59.4580373170363,-105.740137177862,
173.034573766048));
#29061=CARTESIAN_POINT('Ctrl Pts',(-60.3075312249805,-105.555294223339,
173.898875727171));
#29062=CARTESIAN_POINT('Ctrl Pts',(-61.1570251329247,-105.370451268815,
174.763177688294));
#29063=CARTESIAN_POINT('Ctrl Pts',(-61.1470870191508,-105.277229509582,
175.985485192554));
#29064=CARTESIAN_POINT('Ctrl Pts',(-61.1371489053769,-105.184007750348,
177.207792696815));
#29065=CARTESIAN_POINT('Ctrl Pts',(-60.2677787996762,-105.182407183228,
178.072094585608));
#29066=CARTESIAN_POINT('Ctrl Pts',(-59.3984086939755,-105.180806616108,
178.936396474401));
#29067=CARTESIAN_POINT('Ctrl Pts',(-58.1730502310727,-105.217156786186,
178.936396423256));
#29068=CARTESIAN_POINT('Ctrl Pts',(-56.9476917681698,-105.253506956265,
178.936396372111));
#29069=CARTESIAN_POINT('Ctrl Pts',(-56.0783217343916,-105.251906381477,
178.072094410988));
#29070=CARTESIAN_POINT('Ctrl Pts',(-55.2089517006133,-105.25030580669,177.207792449865));
#29071=CARTESIAN_POINT('Ctrl Pts',(-55.1990136885532,-105.157084036613,
175.985484945604));
#29072=CARTESIAN_POINT('Ctrl Pts',(-55.189075676493,-105.063862266536,174.763177441344));
#29073=CARTESIAN_POINT('Ctrl Pts',(-56.0385696563597,-104.879019304345,
173.89887555255));
#29074=CARTESIAN_POINT('Ctrl Pts',(-56.8880636362264,-104.694176342154,
173.034573663757));
#29075=CARTESIAN_POINT('Ctrl Pts',(-58.0935459732952,-104.471382642765,
173.034573714903));
#29076=CARTESIAN_POINT('Ctrl Pts',(-59.299028310364,-104.248588943376,173.034573766048));
#29077=CARTESIAN_POINT('Ctrl Pts',(-60.1485222183082,-104.063745988853,
173.898875727171));
#29078=CARTESIAN_POINT('Ctrl Pts',(-60.9980161262524,-103.87890303433,174.763177688294));
#29079=CARTESIAN_POINT('Ctrl Pts',(-60.9880780124786,-103.785681275096,
175.985485192554));
#29080=CARTESIAN_POINT('Ctrl Pts',(-60.9781398987047,-103.692459515862,
177.207792696815));
#29081=CARTESIAN_POINT('Ctrl Pts',(-60.108769793004,-103.690858948742,178.072094585608));
#29082=CARTESIAN_POINT('Ctrl Pts',(-59.2393996873033,-103.689258381622,
178.936396474401));
#29083=CARTESIAN_POINT('Ctrl Pts',(-58.0140412244004,-103.725608551701,
178.936396423256));
#29084=CARTESIAN_POINT('Ctrl Pts',(-56.7886827614976,-103.761958721779,
178.936396372111));
#29085=CARTESIAN_POINT('Ctrl Pts',(-55.9193127277193,-103.760358146992,
178.072094410988));
#29086=CARTESIAN_POINT('Ctrl Pts',(-55.0499426939411,-103.758757572204,
177.207792449865));
#29087=CARTESIAN_POINT('Ctrl Pts',(-55.0400046818809,-103.665535802127,
175.985484945604));
#29088=CARTESIAN_POINT('Ctrl Pts',(-55.0300666698208,-103.57231403205,174.763177441344));
#29089=CARTESIAN_POINT('Ctrl Pts',(-55.8795606496874,-103.387471069859,
173.89887555255));
#29090=CARTESIAN_POINT('Ctrl Pts',(-56.7290546295541,-103.202628107669,
173.034573663757));
#29091=CARTESIAN_POINT('Ctrl Pts',(-57.934536966623,-102.97983440828,173.034573714903));
#29092=CARTESIAN_POINT('Ctrl Pts',(-59.1400193036918,-102.757040708891,
173.034573766048));
#29093=CARTESIAN_POINT('Ctrl Pts',(-59.989513211636,-102.572197754367,173.898875727171));
#29094=CARTESIAN_POINT('Ctrl Pts',(-60.8390071195802,-102.387354799844,
174.763177688294));
#29095=CARTESIAN_POINT('Ctrl Pts',(-60.8290690058063,-102.29413304061,175.985485192554));
#29096=CARTESIAN_POINT('Ctrl Pts',(-60.8191308920325,-102.200911281377,
177.207792696815));
#29097=CARTESIAN_POINT('Ctrl Pts',(-59.9497607863318,-102.199310714257,
178.072094585608));
#29098=CARTESIAN_POINT('Ctrl Pts',(-59.0803906806311,-102.197710147137,
178.936396474401));
#29099=CARTESIAN_POINT('Ctrl Pts',(-57.8550322177282,-102.234060317215,
178.936396423256));
#29100=CARTESIAN_POINT('Ctrl Pts',(-56.6296737548253,-102.270410487293,
178.936396372111));
#29101=CARTESIAN_POINT('Ctrl Pts',(-55.7603037210471,-102.268809912506,
178.072094410988));
#29102=CARTESIAN_POINT('Ctrl Pts',(-54.8909336872689,-102.267209337719,
177.207792449865));
#29103=CARTESIAN_POINT('Ctrl Pts',(-54.8809956752087,-102.173987567642,
175.985484945604));
#29104=CARTESIAN_POINT('Ctrl Pts',(-54.8710576631486,-102.080765797565,
174.763177441344));
#29105=CARTESIAN_POINT('Ctrl Pts',(-55.7205516430152,-101.895922835374,
173.89887555255));
#29106=CARTESIAN_POINT('Ctrl Pts',(-56.5700456228819,-101.711079873183,
173.034573663757));
#29107=CARTESIAN_POINT('Ctrl Pts',(-57.7755279599507,-101.488286173794,
173.034573714903));
#29108=CARTESIAN_POINT('Ctrl Pts',(-58.9810102970196,-101.265492474405,
173.034573766048));
#29109=CARTESIAN_POINT('Ctrl Pts',(-59.8305042049638,-101.080649519882,
173.898875727171));
#29110=CARTESIAN_POINT('Ctrl Pts',(-60.679998112908,-100.895806565358,174.763177688294));
#29111=CARTESIAN_POINT('Ctrl Pts',(-60.6700599991341,-100.802584806125,
175.985485192554));
#29112=CARTESIAN_POINT('Ctrl Pts',(-60.6601218853602,-100.709363046891,
177.207792696815));
#29113=CARTESIAN_POINT('Ctrl Pts',(-59.7907517796595,-100.707762479771,
178.072094585608));
#29114=CARTESIAN_POINT('Ctrl Pts',(-58.9213816739588,-100.706161912651,
178.936396474401));
#29115=CARTESIAN_POINT('Ctrl Pts',(-57.696023211056,-100.742512082729,178.936396423256));
#29116=CARTESIAN_POINT('Ctrl Pts',(-56.4706647481531,-100.778862252808,
178.936396372111));
#29117=CARTESIAN_POINT('Ctrl Pts',(-55.6012947143749,-100.77726167802,178.072094410988));
#29118=CARTESIAN_POINT('Ctrl Pts',(-54.7319246805966,-100.775661103233,
177.207792449865));
#29119=CARTESIAN_POINT('Ctrl Pts',(-54.7219866685365,-100.682439333156,
175.985484945604));
#29120=CARTESIAN_POINT('Ctrl Pts',(-54.7120486564763,-100.589217563079,
174.763177441344));
#29121=CARTESIAN_POINT('Ctrl Pts',(-55.561542636343,-100.404374600888,173.89887555255));
#29122=CARTESIAN_POINT('Ctrl Pts',(-56.4110366162097,-100.219531638698,
173.034573663757));
#29123=CARTESIAN_POINT('Ctrl Pts',(-57.6165189532785,-99.9967379393085,
173.034573714903));
#29124=CARTESIAN_POINT('Ctrl Pts',(-58.8220012903473,-99.7739442399195,
173.034573766048));
#29125=CARTESIAN_POINT('Ctrl Pts',(-59.6714951982915,-99.5891012853962,
173.898875727171));
#29126=CARTESIAN_POINT('Ctrl Pts',(-60.5209891062358,-99.4042583308729,
174.763177688294));
#29127=CARTESIAN_POINT('Ctrl Pts',(-60.5110509924619,-99.3110365716392,
175.985485192554));
#29128=CARTESIAN_POINT('Ctrl Pts',(-60.501112878688,-99.2178148124055,177.207792696815));
#29129=CARTESIAN_POINT('Ctrl Pts',(-59.6317427729873,-99.2162142452855,
178.072094585608));
#29130=CARTESIAN_POINT('Ctrl Pts',(-58.7623726672866,-99.2146136781656,
178.936396474401));
#29131=CARTESIAN_POINT('Ctrl Pts',(-57.5370142043838,-99.2509638482439,
178.936396423256));
#29132=CARTESIAN_POINT('Ctrl Pts',(-56.3116557414809,-99.2873140183222,
178.936396372111));
#29133=CARTESIAN_POINT('Ctrl Pts',(-55.4422857077027,-99.2857134435348,
178.072094410988));
#29134=CARTESIAN_POINT('Ctrl Pts',(-54.5729156739244,-99.2841128687474,
177.207792449865));
#29135=CARTESIAN_POINT('Ctrl Pts',(-54.5629776618643,-99.1908910986704,
175.985484945604));
#29136=CARTESIAN_POINT('Ctrl Pts',(-54.5530396498041,-99.0976693285933,
174.763177441344));
#29137=CARTESIAN_POINT('Ctrl Pts',(-55.4025336296708,-98.9128263664026,
173.89887555255));
#29138=CARTESIAN_POINT('Ctrl Pts',(-56.2520276095374,-98.727983404212,173.034573663757));
#29139=CARTESIAN_POINT('Ctrl Pts',(-57.4575099466063,-98.5051897048229,
173.034573714903));
#29140=CARTESIAN_POINT('Ctrl Pts',(-58.6629922836751,-98.2823960054338,
173.034573766048));
#29141=CARTESIAN_POINT('Ctrl Pts',(-59.5124861916193,-98.0975530509106,
173.898875727171));
#29142=CARTESIAN_POINT('Ctrl Pts',(-60.3619800995635,-97.9127100963873,
174.763177688294));
#29143=CARTESIAN_POINT('Ctrl Pts',(-60.3520419857897,-97.8194883371536,
175.985485192554));
#29144=CARTESIAN_POINT('Ctrl Pts',(-60.3421038720158,-97.7262665779199,
177.207792696815));
#29145=CARTESIAN_POINT('Ctrl Pts',(-59.4727337663151,-97.7246660108,178.072094585608));
#29146=CARTESIAN_POINT('Ctrl Pts',(-58.6033636606144,-97.72306544368,178.936396474401));
#29147=CARTESIAN_POINT('Ctrl Pts',(-57.3780051977115,-97.7594156137583,
178.936396423256));
#29148=CARTESIAN_POINT('Ctrl Pts',(-56.1526467348087,-97.7957657838366,
178.936396372111));
#29149=CARTESIAN_POINT('Ctrl Pts',(-55.2832767010304,-97.7941652090492,
178.072094410988));
#29150=CARTESIAN_POINT('Ctrl Pts',(-56.1707931031902,-113.117197303651,
178.813912075476));
#29151=CARTESIAN_POINT('Ctrl Pts',(-54.9958834532485,-113.148169293224,
177.6423391512));
#29152=CARTESIAN_POINT('Ctrl Pts',(-54.9859454592686,-113.05494752122,175.985484901707));
#29153=CARTESIAN_POINT('Ctrl Pts',(-54.9760074652888,-112.961725749215,
174.328630652215));
#29154=CARTESIAN_POINT('Ctrl Pts',(-56.1310410868884,-112.744310219938,
173.157057825983));
#29155=CARTESIAN_POINT('Ctrl Pts',(-57.286074708488,-112.52689469066,171.985484999752));
#29156=CARTESIAN_POINT('Ctrl Pts',(-58.9236553326579,-112.258036427063,
171.985485069079));
#29157=CARTESIAN_POINT('Ctrl Pts',(-60.5612359568277,-111.989178163466,
171.985485138407));
#29158=CARTESIAN_POINT('Ctrl Pts',(-61.7162694809355,-111.771762644582,
173.157058062683));
#29159=CARTESIAN_POINT('Ctrl Pts',(-62.8713030050432,-111.554347125698,
174.328630986959));
#29160=CARTESIAN_POINT('Ctrl Pts',(-62.861364873189,-111.461125368392,175.985485236451));
#29161=CARTESIAN_POINT('Ctrl Pts',(-62.8514267413349,-111.367903611086,
177.642339485944));
#29162=CARTESIAN_POINT('Ctrl Pts',(-61.6765169939012,-111.398875611052,
178.813912312176));
#29163=CARTESIAN_POINT('Ctrl Pts',(-60.5016072464676,-111.429847611019,
179.985485138407));
#29164=CARTESIAN_POINT('Ctrl Pts',(-58.8441504964637,-111.512262345305,
179.985485069079));
#29165=CARTESIAN_POINT('Ctrl Pts',(-57.1866937464598,-111.594677079592,
179.985484999752));
#29166=CARTESIAN_POINT('Ctrl Pts',(-56.011784096518,-111.625649069165,178.813912075476));
#29167=CARTESIAN_POINT('Ctrl Pts',(-54.8368744465762,-111.656621058739,
177.6423391512));
#29168=CARTESIAN_POINT('Ctrl Pts',(-54.8269364525964,-111.563399286734,
175.985484901707));
#29169=CARTESIAN_POINT('Ctrl Pts',(-54.8169984586165,-111.47017751473,174.328630652215));
#29170=CARTESIAN_POINT('Ctrl Pts',(-55.9720320802161,-111.252761985452,
173.157057825983));
#29171=CARTESIAN_POINT('Ctrl Pts',(-57.1270657018158,-111.035346456175,
171.985484999752));
#29172=CARTESIAN_POINT('Ctrl Pts',(-58.7646463259856,-110.766488192578,
171.985485069079));
#29173=CARTESIAN_POINT('Ctrl Pts',(-60.4022269501555,-110.497629928981,
171.985485138407));
#29174=CARTESIAN_POINT('Ctrl Pts',(-61.5572604742632,-110.280214410097,
173.157058062683));
#29175=CARTESIAN_POINT('Ctrl Pts',(-62.712293998371,-110.062798891212,174.328630986959));
#29176=CARTESIAN_POINT('Ctrl Pts',(-62.7023558665168,-109.969577133906,
175.985485236451));
#29177=CARTESIAN_POINT('Ctrl Pts',(-62.6924177346626,-109.8763553766,177.642339485944));
#29178=CARTESIAN_POINT('Ctrl Pts',(-61.517507987229,-109.907327376567,178.813912312176));
#29179=CARTESIAN_POINT('Ctrl Pts',(-60.3425982397954,-109.938299376534,
179.985485138407));
#29180=CARTESIAN_POINT('Ctrl Pts',(-58.6851414897915,-110.02071411082,179.985485069079));
#29181=CARTESIAN_POINT('Ctrl Pts',(-57.0276847397876,-110.103128845106,
179.985484999752));
#29182=CARTESIAN_POINT('Ctrl Pts',(-55.8527750898458,-110.13410083468,178.813912075476));
#29183=CARTESIAN_POINT('Ctrl Pts',(-54.677865439904,-110.165072824253,177.6423391512));
#29184=CARTESIAN_POINT('Ctrl Pts',(-54.6679274459242,-110.071851052249,
175.985484901707));
#29185=CARTESIAN_POINT('Ctrl Pts',(-54.6579894519443,-109.978629280244,
174.328630652215));
#29186=CARTESIAN_POINT('Ctrl Pts',(-55.8130230735439,-109.761213750967,
173.157057825983));
#29187=CARTESIAN_POINT('Ctrl Pts',(-56.9680566951435,-109.543798221689,
171.985484999752));
#29188=CARTESIAN_POINT('Ctrl Pts',(-58.6056373193134,-109.274939958092,
171.985485069079));
#29189=CARTESIAN_POINT('Ctrl Pts',(-60.2432179434833,-109.006081694495,
171.985485138407));
#29190=CARTESIAN_POINT('Ctrl Pts',(-61.398251467591,-108.788666175611,173.157058062683));
#29191=CARTESIAN_POINT('Ctrl Pts',(-62.5532849916988,-108.571250656727,
174.328630986959));
#29192=CARTESIAN_POINT('Ctrl Pts',(-62.5433468598446,-108.478028899421,
175.985485236451));
#29193=CARTESIAN_POINT('Ctrl Pts',(-62.5334087279904,-108.384807142114,
177.642339485944));
#29194=CARTESIAN_POINT('Ctrl Pts',(-61.3584989805568,-108.415779142081,
178.813912312176));
#29195=CARTESIAN_POINT('Ctrl Pts',(-60.1835892331231,-108.446751142048,
179.985485138407));
#29196=CARTESIAN_POINT('Ctrl Pts',(-58.5261324831192,-108.529165876334,
179.985485069079));
#29197=CARTESIAN_POINT('Ctrl Pts',(-56.8686757331153,-108.611580610621,
179.985484999752));
#29198=CARTESIAN_POINT('Ctrl Pts',(-55.6937660831736,-108.642552600194,
178.813912075476));
#29199=CARTESIAN_POINT('Ctrl Pts',(-54.5188564332318,-108.673524589768,
177.6423391512));
#29200=CARTESIAN_POINT('Ctrl Pts',(-54.5089184392519,-108.580302817763,
175.985484901707));
#29201=CARTESIAN_POINT('Ctrl Pts',(-54.4989804452721,-108.487081045759,
174.328630652215));
#29202=CARTESIAN_POINT('Ctrl Pts',(-55.6540140668717,-108.269665516481,
173.157057825983));
#29203=CARTESIAN_POINT('Ctrl Pts',(-56.8090476884713,-108.052249987204,
171.985484999752));
#29204=CARTESIAN_POINT('Ctrl Pts',(-58.4466283126412,-107.783391723607,
171.985485069079));
#29205=CARTESIAN_POINT('Ctrl Pts',(-60.084208936811,-107.51453346001,171.985485138407));
#29206=CARTESIAN_POINT('Ctrl Pts',(-61.2392424609188,-107.297117941125,
173.157058062683));
#29207=CARTESIAN_POINT('Ctrl Pts',(-62.3942759850265,-107.079702422241,
174.328630986959));
#29208=CARTESIAN_POINT('Ctrl Pts',(-62.3843378531723,-106.986480664935,
175.985485236451));
#29209=CARTESIAN_POINT('Ctrl Pts',(-62.3743997213182,-106.893258907629,
177.642339485944));
#29210=CARTESIAN_POINT('Ctrl Pts',(-61.1994899738845,-106.924230907596,
178.813912312176));
#29211=CARTESIAN_POINT('Ctrl Pts',(-60.0245802264509,-106.955202907562,
179.985485138407));
#29212=CARTESIAN_POINT('Ctrl Pts',(-58.367123476447,-107.037617641849,179.985485069079));
#29213=CARTESIAN_POINT('Ctrl Pts',(-56.7096667264431,-107.120032376135,
179.985484999752));
#29214=CARTESIAN_POINT('Ctrl Pts',(-55.5347570765013,-107.151004365708,
178.813912075476));
#29215=CARTESIAN_POINT('Ctrl Pts',(-54.3598474265596,-107.181976355282,
177.6423391512));
#29216=CARTESIAN_POINT('Ctrl Pts',(-54.3499094325797,-107.088754583277,
175.985484901707));
#29217=CARTESIAN_POINT('Ctrl Pts',(-54.3399714385998,-106.995532811273,
174.328630652215));
#29218=CARTESIAN_POINT('Ctrl Pts',(-55.4950050601995,-106.778117281995,
173.157057825983));
#29219=CARTESIAN_POINT('Ctrl Pts',(-56.6500386817991,-106.560701752718,
171.985484999752));
#29220=CARTESIAN_POINT('Ctrl Pts',(-58.2876193059689,-106.291843489121,
171.985485069079));
#29221=CARTESIAN_POINT('Ctrl Pts',(-59.9251999301388,-106.022985225524,
171.985485138407));
#29222=CARTESIAN_POINT('Ctrl Pts',(-61.0802334542465,-105.80556970664,173.157058062683));
#29223=CARTESIAN_POINT('Ctrl Pts',(-62.2352669783543,-105.588154187756,
174.328630986959));
#29224=CARTESIAN_POINT('Ctrl Pts',(-62.2253288465001,-105.494932430449,
175.985485236451));
#29225=CARTESIAN_POINT('Ctrl Pts',(-62.2153907146459,-105.401710673143,
177.642339485944));
#29226=CARTESIAN_POINT('Ctrl Pts',(-61.0404809672123,-105.43268267311,178.813912312176));
#29227=CARTESIAN_POINT('Ctrl Pts',(-59.8655712197787,-105.463654673077,
179.985485138407));
#29228=CARTESIAN_POINT('Ctrl Pts',(-58.2081144697748,-105.546069407363,
179.985485069079));
#29229=CARTESIAN_POINT('Ctrl Pts',(-56.5506577197709,-105.628484141649,
179.985484999752));
#29230=CARTESIAN_POINT('Ctrl Pts',(-55.3757480698291,-105.659456131223,
178.813912075476));
#29231=CARTESIAN_POINT('Ctrl Pts',(-54.2008384198873,-105.690428120796,
177.6423391512));
#29232=CARTESIAN_POINT('Ctrl Pts',(-54.1909004259075,-105.597206348792,
175.985484901707));
#29233=CARTESIAN_POINT('Ctrl Pts',(-54.1809624319276,-105.503984576787,
174.328630652215));
#29234=CARTESIAN_POINT('Ctrl Pts',(-55.3359960535272,-105.28656904751,173.157057825983));
#29235=CARTESIAN_POINT('Ctrl Pts',(-56.4910296751268,-105.069153518232,
171.985484999752));
#29236=CARTESIAN_POINT('Ctrl Pts',(-58.1286102992967,-104.800295254635,
171.985485069079));
#29237=CARTESIAN_POINT('Ctrl Pts',(-59.7661909234666,-104.531436991038,
171.985485138407));
#29238=CARTESIAN_POINT('Ctrl Pts',(-60.9212244475743,-104.314021472154,
173.157058062683));
#29239=CARTESIAN_POINT('Ctrl Pts',(-62.0762579716821,-104.09660595327,174.328630986959));
#29240=CARTESIAN_POINT('Ctrl Pts',(-62.0663198398279,-104.003384195964,
175.985485236451));
#29241=CARTESIAN_POINT('Ctrl Pts',(-62.0563817079737,-103.910162438658,
177.642339485944));
#29242=CARTESIAN_POINT('Ctrl Pts',(-60.8814719605401,-103.941134438624,
178.813912312176));
#29243=CARTESIAN_POINT('Ctrl Pts',(-59.7065622131064,-103.972106438591,
179.985485138407));
#29244=CARTESIAN_POINT('Ctrl Pts',(-58.0491054631025,-104.054521172878,
179.985485069079));
#29245=CARTESIAN_POINT('Ctrl Pts',(-56.3916487130987,-104.136935907164,
179.985484999752));
#29246=CARTESIAN_POINT('Ctrl Pts',(-55.2167390631569,-104.167907896737,
178.813912075476));
#29247=CARTESIAN_POINT('Ctrl Pts',(-54.0418294132151,-104.198879886311,
177.6423391512));
#29248=CARTESIAN_POINT('Ctrl Pts',(-54.0318914192353,-104.105658114306,
175.985484901707));
#29249=CARTESIAN_POINT('Ctrl Pts',(-54.0219534252554,-104.012436342302,
174.328630652215));
#29250=CARTESIAN_POINT('Ctrl Pts',(-55.176987046855,-103.795020813024,173.157057825983));
#29251=CARTESIAN_POINT('Ctrl Pts',(-56.3320206684546,-103.577605283747,
171.985484999752));
#29252=CARTESIAN_POINT('Ctrl Pts',(-57.9696012926245,-103.30874702015,171.985485069079));
#29253=CARTESIAN_POINT('Ctrl Pts',(-59.6071819167943,-103.039888756553,
171.985485138407));
#29254=CARTESIAN_POINT('Ctrl Pts',(-60.7622154409021,-102.822473237669,
173.157058062683));
#29255=CARTESIAN_POINT('Ctrl Pts',(-61.9172489650099,-102.605057718784,
174.328630986959));
#29256=CARTESIAN_POINT('Ctrl Pts',(-61.9073108331557,-102.511835961478,
175.985485236451));
#29257=CARTESIAN_POINT('Ctrl Pts',(-61.8973727013015,-102.418614204172,
177.642339485944));
#29258=CARTESIAN_POINT('Ctrl Pts',(-60.7224629538678,-102.449586204139,
178.813912312176));
#29259=CARTESIAN_POINT('Ctrl Pts',(-59.5475532064342,-102.480558204106,
179.985485138407));
#29260=CARTESIAN_POINT('Ctrl Pts',(-57.8900964564303,-102.562972938392,
179.985485069079));
#29261=CARTESIAN_POINT('Ctrl Pts',(-56.2326397064264,-102.645387672678,
179.985484999752));
#29262=CARTESIAN_POINT('Ctrl Pts',(-55.0577300564847,-102.676359662252,
178.813912075476));
#29263=CARTESIAN_POINT('Ctrl Pts',(-53.8828204065429,-102.707331651825,
177.6423391512));
#29264=CARTESIAN_POINT('Ctrl Pts',(-53.872882412563,-102.614109879821,175.985484901707));
#29265=CARTESIAN_POINT('Ctrl Pts',(-53.8629444185832,-102.520888107816,
174.328630652215));
#29266=CARTESIAN_POINT('Ctrl Pts',(-55.0179780401828,-102.303472578539,
173.157057825983));
#29267=CARTESIAN_POINT('Ctrl Pts',(-56.1730116617824,-102.086057049261,
171.985484999752));
#29268=CARTESIAN_POINT('Ctrl Pts',(-57.8105922859523,-101.817198785664,
171.985485069079));
#29269=CARTESIAN_POINT('Ctrl Pts',(-59.4481729101221,-101.548340522067,
171.985485138407));
#29270=CARTESIAN_POINT('Ctrl Pts',(-60.6032064342299,-101.330925003183,
173.157058062683));
#29271=CARTESIAN_POINT('Ctrl Pts',(-61.7582399583376,-101.113509484299,
174.328630986959));
#29272=CARTESIAN_POINT('Ctrl Pts',(-61.7483018264834,-101.020287726993,
175.985485236451));
#29273=CARTESIAN_POINT('Ctrl Pts',(-61.7383636946293,-100.927065969686,
177.642339485944));
#29274=CARTESIAN_POINT('Ctrl Pts',(-60.5634539471956,-100.958037969653,
178.813912312176));
#29275=CARTESIAN_POINT('Ctrl Pts',(-59.388544199762,-100.98900996962,179.985485138407));
#29276=CARTESIAN_POINT('Ctrl Pts',(-57.7310874497581,-101.071424703906,
179.985485069079));
#29277=CARTESIAN_POINT('Ctrl Pts',(-56.0736306997542,-101.153839438193,
179.985484999752));
#29278=CARTESIAN_POINT('Ctrl Pts',(-54.8987210498124,-101.184811427766,
178.813912075476));
#29279=CARTESIAN_POINT('Ctrl Pts',(-53.7238113998707,-101.21578341734,177.6423391512));
#29280=CARTESIAN_POINT('Ctrl Pts',(-53.7138734058908,-101.122561645335,
175.985484901707));
#29281=CARTESIAN_POINT('Ctrl Pts',(-53.7039354119109,-101.029339873331,
174.328630652215));
#29282=CARTESIAN_POINT('Ctrl Pts',(-54.8589690335105,-100.811924344053,
173.157057825983));
#29283=CARTESIAN_POINT('Ctrl Pts',(-56.0140026551102,-100.594508814776,
171.985484999752));
#29284=CARTESIAN_POINT('Ctrl Pts',(-57.65158327928,-100.325650551179,171.985485069079));
#29285=CARTESIAN_POINT('Ctrl Pts',(-59.2891639034499,-100.056792287582,
171.985485138407));
#29286=CARTESIAN_POINT('Ctrl Pts',(-60.4441974275576,-99.8393767686974,
173.157058062683));
#29287=CARTESIAN_POINT('Ctrl Pts',(-61.5992309516654,-99.6219612498133,
174.328630986959));
#29288=CARTESIAN_POINT('Ctrl Pts',(-61.5892928198112,-99.528739492507,175.985485236451));
#29289=CARTESIAN_POINT('Ctrl Pts',(-61.579354687957,-99.4355177352008,177.642339485944));
#29290=CARTESIAN_POINT('Ctrl Pts',(-60.4044449405234,-99.4664897351676,
178.813912312176));
#29291=CARTESIAN_POINT('Ctrl Pts',(-59.2295351930898,-99.4974617351344,
179.985485138407));
#29292=CARTESIAN_POINT('Ctrl Pts',(-57.5720784430859,-99.5798764694207,
179.985485069079));
#29293=CARTESIAN_POINT('Ctrl Pts',(-55.914621693082,-99.662291203707,179.985484999752));
#29294=CARTESIAN_POINT('Ctrl Pts',(-54.7397120431402,-99.6932631932805,
178.813912075476));
#29295=CARTESIAN_POINT('Ctrl Pts',(-53.5648023931984,-99.724235182854,177.6423391512));
#29296=CARTESIAN_POINT('Ctrl Pts',(-53.5548643992186,-99.6310134108495,
175.985484901707));
#29297=CARTESIAN_POINT('Ctrl Pts',(-53.5449264052387,-99.5377916388449,
174.328630652215));
#29298=CARTESIAN_POINT('Ctrl Pts',(-54.6999600268383,-99.3203761095675,
173.157057825983));
#29299=CARTESIAN_POINT('Ctrl Pts',(-55.8549936484379,-99.10296058029,171.985484999752));
#29300=CARTESIAN_POINT('Ctrl Pts',(-57.4925742726078,-98.834102316693,171.985485069079));
#29301=CARTESIAN_POINT('Ctrl Pts',(-59.1301548967777,-98.565244053096,171.985485138407));
#29302=CARTESIAN_POINT('Ctrl Pts',(-60.2851884208854,-98.3478285342118,
173.157058062683));
#29303=CARTESIAN_POINT('Ctrl Pts',(-61.4402219449932,-98.1304130153276,
174.328630986959));
#29304=CARTESIAN_POINT('Ctrl Pts',(-61.430283813139,-98.0371912580215,175.985485236451));
#29305=CARTESIAN_POINT('Ctrl Pts',(-61.4203456812848,-97.9439695007152,
177.642339485944));
#29306=CARTESIAN_POINT('Ctrl Pts',(-60.2454359338512,-97.974941500682,178.813912312176));
#29307=CARTESIAN_POINT('Ctrl Pts',(-59.0705261864175,-98.0059135006488,
179.985485138407));
#29308=CARTESIAN_POINT('Ctrl Pts',(-57.4130694364136,-98.0883282349351,
179.985485069079));
#29309=CARTESIAN_POINT('Ctrl Pts',(-55.7556126864097,-98.1707429692214,
179.985484999752));
#29310=CARTESIAN_POINT('Ctrl Pts',(-54.580703036468,-98.2017149587949,178.813912075476));
#29311=CARTESIAN_POINT('Ctrl Pts',(-61.3355965912452,-105.42684148695,178.485485069079));
#29312=CARTESIAN_POINT('Ctrl Pts',(-61.1970243868884,-105.428556004828,
178.657813499464));
#29313=CARTESIAN_POINT('Ctrl Pts',(-61.0404809672123,-105.43268267311,178.813912312176));
#29314=CARTESIAN_POINT('Ctrl Pts',(-59.8655712197787,-105.463654673077,
179.985485138407));
#29315=CARTESIAN_POINT('Ctrl Pts',(-58.2081144697748,-105.546069407363,
179.985485069079));
#29316=CARTESIAN_POINT('Ctrl Pts',(-56.5506577197709,-105.628484141649,
179.985484999752));
#29317=CARTESIAN_POINT('Ctrl Pts',(-55.3757480698291,-105.659456131223,
178.813912075476));
#29318=CARTESIAN_POINT('Ctrl Pts',(-54.2008384198873,-105.690428120796,
177.6423391512));
#29319=CARTESIAN_POINT('Ctrl Pts',(-54.1909004259075,-105.597206348792,
175.985484901707));
#29320=CARTESIAN_POINT('Ctrl Pts',(-54.1809624319276,-105.503984576787,
174.328630652215));
#29321=CARTESIAN_POINT('Ctrl Pts',(-55.3359960535272,-105.28656904751,173.157057825983));
#29322=CARTESIAN_POINT('Ctrl Pts',(-56.4910296751268,-105.069153518232,
171.985484999752));
#29323=CARTESIAN_POINT('Ctrl Pts',(-58.1286102992967,-104.800295254635,
171.985485069079));
#29324=CARTESIAN_POINT('Ctrl Pts',(-59.7661909234666,-104.531436991038,
171.985485138407));
#29325=CARTESIAN_POINT('Ctrl Pts',(-60.9212244475743,-104.314021472154,
173.157058062683));
#29326=CARTESIAN_POINT('Ctrl Pts',(-61.0751194685275,-104.285053338212,
173.313156769748));
#29327=CARTESIAN_POINT('Ctrl Pts',(-61.2109386724983,-104.25751590903,173.485485069079));
#29328=CARTESIAN_POINT('Ctrl Pts',(-56.1707931031902,-113.117197303651,
178.813912075476));
#29329=CARTESIAN_POINT('Ctrl Pts',(-54.9958834532485,-113.148169293224,
177.6423391512));
#29330=CARTESIAN_POINT('Ctrl Pts',(-54.9859454592686,-113.05494752122,175.985484901707));
#29331=CARTESIAN_POINT('Ctrl Pts',(-54.9760074652888,-112.961725749215,
174.328630652215));
#29332=CARTESIAN_POINT('Ctrl Pts',(-56.1310410868884,-112.744310219938,
173.157057825983));
#29333=CARTESIAN_POINT('Ctrl Pts',(-57.286074708488,-112.52689469066,171.985484999752));
#29334=CARTESIAN_POINT('Ctrl Pts',(-58.9236553326578,-112.258036427063,
171.985485069079));
#29335=CARTESIAN_POINT('Ctrl Pts',(-60.5612359568277,-111.989178163466,
171.985485138407));
#29336=CARTESIAN_POINT('Ctrl Pts',(-61.7162694809355,-111.771762644582,
173.157058062683));
#29337=CARTESIAN_POINT('Ctrl Pts',(-62.8713030050432,-111.554347125698,
174.328630986959));
#29338=CARTESIAN_POINT('Ctrl Pts',(-62.861364873189,-111.461125368392,175.985485236451));
#29339=CARTESIAN_POINT('Ctrl Pts',(-62.8514267413349,-111.367903611086,
177.642339485944));
#29340=CARTESIAN_POINT('Ctrl Pts',(-61.6765169939012,-111.398875611052,
178.813912312176));
#29341=CARTESIAN_POINT('Ctrl Pts',(-60.5016072464676,-111.429847611019,
179.985485138407));
#29342=CARTESIAN_POINT('Ctrl Pts',(-58.8441504964637,-111.512262345305,
179.985485069079));
#29343=CARTESIAN_POINT('Ctrl Pts',(-57.1866937464598,-111.594677079592,
179.985484999752));
#29344=CARTESIAN_POINT('Ctrl Pts',(-56.011784096518,-111.625649069165,178.813912075476));
#29345=CARTESIAN_POINT('Ctrl Pts',(-54.8368744465763,-111.656621058739,
177.6423391512));
#29346=CARTESIAN_POINT('Ctrl Pts',(-54.8269364525964,-111.563399286734,
175.985484901707));
#29347=CARTESIAN_POINT('Ctrl Pts',(-54.8169984586165,-111.47017751473,174.328630652215));
#29348=CARTESIAN_POINT('Ctrl Pts',(-55.9720320802161,-111.252761985452,
173.157057825983));
#29349=CARTESIAN_POINT('Ctrl Pts',(-57.1270657018158,-111.035346456175,
171.985484999752));
#29350=CARTESIAN_POINT('Ctrl Pts',(-58.7646463259856,-110.766488192578,
171.985485069079));
#29351=CARTESIAN_POINT('Ctrl Pts',(-60.4022269501555,-110.497629928981,
171.985485138407));
#29352=CARTESIAN_POINT('Ctrl Pts',(-61.5572604742632,-110.280214410097,
173.157058062683));
#29353=CARTESIAN_POINT('Ctrl Pts',(-62.712293998371,-110.062798891212,174.328630986959));
#29354=CARTESIAN_POINT('Ctrl Pts',(-62.7023558665168,-109.969577133906,
175.985485236451));
#29355=CARTESIAN_POINT('Ctrl Pts',(-62.6924177346626,-109.8763553766,177.642339485944));
#29356=CARTESIAN_POINT('Ctrl Pts',(-61.517507987229,-109.907327376567,178.813912312176));
#29357=CARTESIAN_POINT('Ctrl Pts',(-60.3425982397954,-109.938299376534,
179.985485138407));
#29358=CARTESIAN_POINT('Ctrl Pts',(-58.6851414897915,-110.02071411082,179.985485069079));
#29359=CARTESIAN_POINT('Ctrl Pts',(-57.0276847397876,-110.103128845106,
179.985484999752));
#29360=CARTESIAN_POINT('Ctrl Pts',(-55.8527750898458,-110.13410083468,178.813912075476));
#29361=CARTESIAN_POINT('Ctrl Pts',(-54.677865439904,-110.165072824253,177.6423391512));
#29362=CARTESIAN_POINT('Ctrl Pts',(-54.6679274459242,-110.071851052249,
175.985484901707));
#29363=CARTESIAN_POINT('Ctrl Pts',(-54.6579894519443,-109.978629280244,
174.328630652215));
#29364=CARTESIAN_POINT('Ctrl Pts',(-55.8130230735439,-109.761213750967,
173.157057825983));
#29365=CARTESIAN_POINT('Ctrl Pts',(-56.9680566951435,-109.543798221689,
171.985484999752));
#29366=CARTESIAN_POINT('Ctrl Pts',(-58.6056373193134,-109.274939958092,
171.985485069079));
#29367=CARTESIAN_POINT('Ctrl Pts',(-60.2432179434833,-109.006081694495,
171.985485138407));
#29368=CARTESIAN_POINT('Ctrl Pts',(-61.398251467591,-108.788666175611,173.157058062683));
#29369=CARTESIAN_POINT('Ctrl Pts',(-62.5532849916988,-108.571250656727,
174.328630986959));
#29370=CARTESIAN_POINT('Ctrl Pts',(-62.5433468598446,-108.478028899421,
175.985485236451));
#29371=CARTESIAN_POINT('Ctrl Pts',(-62.5334087279904,-108.384807142114,
177.642339485944));
#29372=CARTESIAN_POINT('Ctrl Pts',(-61.3584989805568,-108.415779142081,
178.813912312176));
#29373=CARTESIAN_POINT('Ctrl Pts',(-60.1835892331231,-108.446751142048,
179.985485138407));
#29374=CARTESIAN_POINT('Ctrl Pts',(-58.5261324831192,-108.529165876334,
179.985485069079));
#29375=CARTESIAN_POINT('Ctrl Pts',(-56.8686757331153,-108.611580610621,
179.985484999752));
#29376=CARTESIAN_POINT('Ctrl Pts',(-55.6937660831736,-108.642552600194,
178.813912075476));
#29377=CARTESIAN_POINT('Ctrl Pts',(-54.5188564332318,-108.673524589768,
177.6423391512));
#29378=CARTESIAN_POINT('Ctrl Pts',(-54.5089184392519,-108.580302817763,
175.985484901707));
#29379=CARTESIAN_POINT('Ctrl Pts',(-54.4989804452721,-108.487081045759,
174.328630652215));
#29380=CARTESIAN_POINT('Ctrl Pts',(-55.6540140668717,-108.269665516481,
173.157057825983));
#29381=CARTESIAN_POINT('Ctrl Pts',(-56.8090476884713,-108.052249987204,
171.985484999752));
#29382=CARTESIAN_POINT('Ctrl Pts',(-58.4466283126412,-107.783391723607,
171.985485069079));
#29383=CARTESIAN_POINT('Ctrl Pts',(-60.084208936811,-107.51453346001,171.985485138407));
#29384=CARTESIAN_POINT('Ctrl Pts',(-61.2392424609188,-107.297117941125,
173.157058062683));
#29385=CARTESIAN_POINT('Ctrl Pts',(-62.3942759850265,-107.079702422241,
174.328630986959));
#29386=CARTESIAN_POINT('Ctrl Pts',(-62.3843378531723,-106.986480664935,
175.985485236451));
#29387=CARTESIAN_POINT('Ctrl Pts',(-62.3743997213182,-106.893258907629,
177.642339485944));
#29388=CARTESIAN_POINT('Ctrl Pts',(-61.1994899738845,-106.924230907596,
178.813912312176));
#29389=CARTESIAN_POINT('Ctrl Pts',(-60.0245802264509,-106.955202907562,
179.985485138407));
#29390=CARTESIAN_POINT('Ctrl Pts',(-58.367123476447,-107.037617641849,179.985485069079));
#29391=CARTESIAN_POINT('Ctrl Pts',(-56.7096667264431,-107.120032376135,
179.985484999752));
#29392=CARTESIAN_POINT('Ctrl Pts',(-55.5347570765013,-107.151004365708,
178.813912075476));
#29393=CARTESIAN_POINT('Ctrl Pts',(-54.3598474265596,-107.181976355282,
177.6423391512));
#29394=CARTESIAN_POINT('Ctrl Pts',(-54.3499094325797,-107.088754583277,
175.985484901707));
#29395=CARTESIAN_POINT('Ctrl Pts',(-54.3399714385998,-106.995532811273,
174.328630652215));
#29396=CARTESIAN_POINT('Ctrl Pts',(-55.4950050601995,-106.778117281995,
173.157057825983));
#29397=CARTESIAN_POINT('Ctrl Pts',(-56.6500386817991,-106.560701752718,
171.985484999752));
#29398=CARTESIAN_POINT('Ctrl Pts',(-58.2876193059689,-106.291843489121,
171.985485069079));
#29399=CARTESIAN_POINT('Ctrl Pts',(-59.9251999301388,-106.022985225524,
171.985485138407));
#29400=CARTESIAN_POINT('Ctrl Pts',(-61.0802334542465,-105.80556970664,173.157058062683));
#29401=CARTESIAN_POINT('Ctrl Pts',(-62.2352669783543,-105.588154187756,
174.328630986959));
#29402=CARTESIAN_POINT('Ctrl Pts',(-62.2253288465001,-105.494932430449,
175.985485236451));
#29403=CARTESIAN_POINT('Ctrl Pts',(-62.2153907146459,-105.401710673143,
177.642339485944));
#29404=CARTESIAN_POINT('Ctrl Pts',(-61.0404809672123,-105.43268267311,178.813912312176));
#29405=CARTESIAN_POINT('Ctrl Pts',(-59.8655712197787,-105.463654673077,
179.985485138407));
#29406=CARTESIAN_POINT('Ctrl Pts',(-58.2081144697748,-105.546069407363,
179.985485069079));
#29407=CARTESIAN_POINT('Ctrl Pts',(-56.5506577197709,-105.628484141649,
179.985484999752));
#29408=CARTESIAN_POINT('Ctrl Pts',(-55.3757480698291,-105.659456131223,
178.813912075476));
#29409=CARTESIAN_POINT('Ctrl Pts',(-54.2008384198873,-105.690428120796,
177.6423391512));
#29410=CARTESIAN_POINT('Ctrl Pts',(-54.1909004259075,-105.597206348792,
175.985484901707));
#29411=CARTESIAN_POINT('Ctrl Pts',(-54.1809624319276,-105.503984576787,
174.328630652215));
#29412=CARTESIAN_POINT('Ctrl Pts',(-55.3359960535272,-105.28656904751,173.157057825983));
#29413=CARTESIAN_POINT('Ctrl Pts',(-56.4910296751268,-105.069153518232,
171.985484999752));
#29414=CARTESIAN_POINT('Ctrl Pts',(-58.1286102992967,-104.800295254635,
171.985485069079));
#29415=CARTESIAN_POINT('Ctrl Pts',(-59.7661909234666,-104.531436991038,
171.985485138407));
#29416=CARTESIAN_POINT('Ctrl Pts',(-60.9212244475743,-104.314021472154,
173.157058062683));
#29417=CARTESIAN_POINT('Ctrl Pts',(-62.0762579716821,-104.09660595327,174.328630986959));
#29418=CARTESIAN_POINT('Ctrl Pts',(-62.0663198398279,-104.003384195964,
175.985485236451));
#29419=CARTESIAN_POINT('Ctrl Pts',(-62.0563817079737,-103.910162438658,
177.642339485944));
#29420=CARTESIAN_POINT('Ctrl Pts',(-60.8814719605401,-103.941134438624,
178.813912312176));
#29421=CARTESIAN_POINT('Ctrl Pts',(-59.7065622131064,-103.972106438591,
179.985485138407));
#29422=CARTESIAN_POINT('Ctrl Pts',(-58.0491054631025,-104.054521172878,
179.985485069079));
#29423=CARTESIAN_POINT('Ctrl Pts',(-56.3916487130987,-104.136935907164,
179.985484999752));
#29424=CARTESIAN_POINT('Ctrl Pts',(-55.2167390631569,-104.167907896737,
178.813912075476));
#29425=CARTESIAN_POINT('Ctrl Pts',(-54.0418294132151,-104.198879886311,
177.6423391512));
#29426=CARTESIAN_POINT('Ctrl Pts',(-54.0318914192353,-104.105658114306,
175.985484901707));
#29427=CARTESIAN_POINT('Ctrl Pts',(-54.0219534252554,-104.012436342302,
174.328630652215));
#29428=CARTESIAN_POINT('Ctrl Pts',(-55.176987046855,-103.795020813024,173.157057825983));
#29429=CARTESIAN_POINT('Ctrl Pts',(-56.3320206684546,-103.577605283747,
171.985484999752));
#29430=CARTESIAN_POINT('Ctrl Pts',(-57.9696012926245,-103.30874702015,171.985485069079));
#29431=CARTESIAN_POINT('Ctrl Pts',(-59.6071819167943,-103.039888756553,
171.985485138407));
#29432=CARTESIAN_POINT('Ctrl Pts',(-60.7622154409021,-102.822473237669,
173.157058062683));
#29433=CARTESIAN_POINT('Ctrl Pts',(-61.9172489650099,-102.605057718784,
174.328630986959));
#29434=CARTESIAN_POINT('Ctrl Pts',(-61.9073108331557,-102.511835961478,
175.985485236451));
#29435=CARTESIAN_POINT('Ctrl Pts',(-61.8973727013015,-102.418614204172,
177.642339485944));
#29436=CARTESIAN_POINT('Ctrl Pts',(-60.7224629538678,-102.449586204139,
178.813912312176));
#29437=CARTESIAN_POINT('Ctrl Pts',(-59.5475532064342,-102.480558204106,
179.985485138407));
#29438=CARTESIAN_POINT('Ctrl Pts',(-57.8900964564303,-102.562972938392,
179.985485069079));
#29439=CARTESIAN_POINT('Ctrl Pts',(-56.2326397064264,-102.645387672678,
179.985484999752));
#29440=CARTESIAN_POINT('Ctrl Pts',(-55.0577300564847,-102.676359662252,
178.813912075476));
#29441=CARTESIAN_POINT('Ctrl Pts',(-53.8828204065429,-102.707331651825,
177.6423391512));
#29442=CARTESIAN_POINT('Ctrl Pts',(-53.872882412563,-102.614109879821,175.985484901707));
#29443=CARTESIAN_POINT('Ctrl Pts',(-53.8629444185832,-102.520888107816,
174.328630652215));
#29444=CARTESIAN_POINT('Ctrl Pts',(-55.0179780401828,-102.303472578539,
173.157057825983));
#29445=CARTESIAN_POINT('Ctrl Pts',(-56.1730116617824,-102.086057049261,
171.985484999752));
#29446=CARTESIAN_POINT('Ctrl Pts',(-57.8105922859523,-101.817198785664,
171.985485069079));
#29447=CARTESIAN_POINT('Ctrl Pts',(-59.4481729101221,-101.548340522067,
171.985485138407));
#29448=CARTESIAN_POINT('Ctrl Pts',(-60.6032064342299,-101.330925003183,
173.157058062683));
#29449=CARTESIAN_POINT('Ctrl Pts',(-61.7582399583376,-101.113509484299,
174.328630986959));
#29450=CARTESIAN_POINT('Ctrl Pts',(-61.7483018264834,-101.020287726993,
175.985485236451));
#29451=CARTESIAN_POINT('Ctrl Pts',(-61.7383636946293,-100.927065969686,
177.642339485944));
#29452=CARTESIAN_POINT('Ctrl Pts',(-60.5634539471956,-100.958037969653,
178.813912312176));
#29453=CARTESIAN_POINT('Ctrl Pts',(-59.388544199762,-100.98900996962,179.985485138407));
#29454=CARTESIAN_POINT('Ctrl Pts',(-57.7310874497581,-101.071424703906,
179.985485069079));
#29455=CARTESIAN_POINT('Ctrl Pts',(-56.0736306997542,-101.153839438193,
179.985484999752));
#29456=CARTESIAN_POINT('Ctrl Pts',(-54.8987210498124,-101.184811427766,
178.813912075476));
#29457=CARTESIAN_POINT('Ctrl Pts',(-53.7238113998707,-101.21578341734,177.6423391512));
#29458=CARTESIAN_POINT('Ctrl Pts',(-53.7138734058908,-101.122561645335,
175.985484901707));
#29459=CARTESIAN_POINT('Ctrl Pts',(-53.7039354119109,-101.029339873331,
174.328630652215));
#29460=CARTESIAN_POINT('Ctrl Pts',(-54.8589690335105,-100.811924344053,
173.157057825983));
#29461=CARTESIAN_POINT('Ctrl Pts',(-56.0140026551102,-100.594508814776,
171.985484999752));
#29462=CARTESIAN_POINT('Ctrl Pts',(-57.65158327928,-100.325650551179,171.985485069079));
#29463=CARTESIAN_POINT('Ctrl Pts',(-59.2891639034499,-100.056792287582,
171.985485138407));
#29464=CARTESIAN_POINT('Ctrl Pts',(-60.4441974275576,-99.8393767686974,
173.157058062683));
#29465=CARTESIAN_POINT('Ctrl Pts',(-61.5992309516654,-99.6219612498133,
174.328630986959));
#29466=CARTESIAN_POINT('Ctrl Pts',(-61.5892928198112,-99.528739492507,175.985485236451));
#29467=CARTESIAN_POINT('Ctrl Pts',(-61.579354687957,-99.4355177352008,177.642339485944));
#29468=CARTESIAN_POINT('Ctrl Pts',(-60.4044449405234,-99.4664897351676,
178.813912312176));
#29469=CARTESIAN_POINT('Ctrl Pts',(-59.2295351930898,-99.4974617351344,
179.985485138407));
#29470=CARTESIAN_POINT('Ctrl Pts',(-57.5720784430859,-99.5798764694207,
179.985485069079));
#29471=CARTESIAN_POINT('Ctrl Pts',(-55.914621693082,-99.662291203707,179.985484999752));
#29472=CARTESIAN_POINT('Ctrl Pts',(-54.7397120431402,-99.6932631932805,
178.813912075476));
#29473=CARTESIAN_POINT('Ctrl Pts',(-53.5648023931984,-99.724235182854,177.6423391512));
#29474=CARTESIAN_POINT('Ctrl Pts',(-53.5548643992186,-99.6310134108495,
175.985484901707));
#29475=CARTESIAN_POINT('Ctrl Pts',(-53.5449264052387,-99.5377916388449,
174.328630652215));
#29476=CARTESIAN_POINT('Ctrl Pts',(-54.6999600268383,-99.3203761095675,
173.157057825983));
#29477=CARTESIAN_POINT('Ctrl Pts',(-55.8549936484379,-99.10296058029,171.985484999752));
#29478=CARTESIAN_POINT('Ctrl Pts',(-57.4925742726078,-98.834102316693,171.985485069079));
#29479=CARTESIAN_POINT('Ctrl Pts',(-59.1301548967777,-98.5652440530961,
171.985485138407));
#29480=CARTESIAN_POINT('Ctrl Pts',(-60.2851884208854,-98.3478285342118,
173.157058062683));
#29481=CARTESIAN_POINT('Ctrl Pts',(-61.4402219449932,-98.1304130153276,
174.328630986959));
#29482=CARTESIAN_POINT('Ctrl Pts',(-61.430283813139,-98.0371912580215,175.985485236451));
#29483=CARTESIAN_POINT('Ctrl Pts',(-61.4203456812848,-97.9439695007152,
177.642339485944));
#29484=CARTESIAN_POINT('Ctrl Pts',(-60.2454359338512,-97.974941500682,178.813912312176));
#29485=CARTESIAN_POINT('Ctrl Pts',(-59.0705261864175,-98.0059135006488,
179.985485138407));
#29486=CARTESIAN_POINT('Ctrl Pts',(-57.4130694364136,-98.0883282349351,
179.985485069079));
#29487=CARTESIAN_POINT('Ctrl Pts',(-55.7556126864097,-98.1707429692214,
179.985484999752));
#29488=CARTESIAN_POINT('Ctrl Pts',(-54.580703036468,-98.2017149587949,178.813912075476));
#29489=CARTESIAN_POINT('Ctrl Pts',(-56.181115489574,-113.283598570176,178.821287383467));
#29490=CARTESIAN_POINT('Ctrl Pts',(-55.0031681001975,-113.314894403068,
177.646659506339));
#29491=CARTESIAN_POINT('Ctrl Pts',(-54.9932301063974,-113.221672631044,
175.985484901271));
#29492=CARTESIAN_POINT('Ctrl Pts',(-54.9832921125973,-113.12845085902,174.324310296203));
#29493=CARTESIAN_POINT('Ctrl Pts',(-56.1413634738858,-112.910711486397,
173.149682517375));
#29494=CARTESIAN_POINT('Ctrl Pts',(-57.2994348351743,-112.692972113774,
171.975054738546));
#29495=CARTESIAN_POINT('Ctrl Pts',(-58.9413114718314,-112.423655866545,
171.975054808055));
#29496=CARTESIAN_POINT('Ctrl Pts',(-60.5831881084886,-112.154339619316,
171.975054877564));
#29497=CARTESIAN_POINT('Ctrl Pts',(-61.741259372031,-111.936600257113,173.149682754692));
#29498=CARTESIAN_POINT('Ctrl Pts',(-62.8993306355734,-111.71886089491,174.32431063182));
#29499=CARTESIAN_POINT('Ctrl Pts',(-62.8893925035395,-111.625639137623,
175.985485236888));
#29500=CARTESIAN_POINT('Ctrl Pts',(-62.8794543715055,-111.532417380336,
177.646659841956));
#29501=CARTESIAN_POINT('Ctrl Pts',(-61.701506884383,-111.563713223648,178.821287620784));
#29502=CARTESIAN_POINT('Ctrl Pts',(-60.5235593972605,-111.595009066961,
179.995915399612));
#29503=CARTESIAN_POINT('Ctrl Pts',(-58.8618066347693,-111.677881784879,
179.995915330104));
#29504=CARTESIAN_POINT('Ctrl Pts',(-57.2000538722782,-111.760754502798,
179.995915260595));
#29505=CARTESIAN_POINT('Ctrl Pts',(-56.0221064829017,-111.79205033569,178.821287383467));
#29506=CARTESIAN_POINT('Ctrl Pts',(-54.8441590935253,-111.823346168582,
177.646659506339));
#29507=CARTESIAN_POINT('Ctrl Pts',(-54.8342210997252,-111.730124396559,
175.985484901271));
#29508=CARTESIAN_POINT('Ctrl Pts',(-54.8242831059251,-111.636902624535,
174.324310296203));
#29509=CARTESIAN_POINT('Ctrl Pts',(-55.9823544672136,-111.419163251912,
173.149682517375));
#29510=CARTESIAN_POINT('Ctrl Pts',(-57.1404258285021,-111.201423879289,
171.975054738546));
#29511=CARTESIAN_POINT('Ctrl Pts',(-58.7823024651592,-110.932107632059,
171.975054808055));
#29512=CARTESIAN_POINT('Ctrl Pts',(-60.4241791018163,-110.66279138483,171.975054877564));
#29513=CARTESIAN_POINT('Ctrl Pts',(-61.5822503653587,-110.445052022627,
173.149682754692));
#29514=CARTESIAN_POINT('Ctrl Pts',(-62.7403216289012,-110.227312660424,
174.32431063182));
#29515=CARTESIAN_POINT('Ctrl Pts',(-62.7303834968672,-110.134090903137,
175.985485236888));
#29516=CARTESIAN_POINT('Ctrl Pts',(-62.7204453648333,-110.04086914585,177.646659841956));
#29517=CARTESIAN_POINT('Ctrl Pts',(-61.5424978777108,-110.072164989163,
178.821287620784));
#29518=CARTESIAN_POINT('Ctrl Pts',(-60.3645503905882,-110.103460832475,
179.995915399612));
#29519=CARTESIAN_POINT('Ctrl Pts',(-58.7027976280971,-110.186333550394,
179.995915330104));
#29520=CARTESIAN_POINT('Ctrl Pts',(-57.041044865606,-110.269206268313,179.995915260595));
#29521=CARTESIAN_POINT('Ctrl Pts',(-55.8630974762295,-110.300502101205,
178.821287383467));
#29522=CARTESIAN_POINT('Ctrl Pts',(-54.6851500868531,-110.331797934097,
177.646659506339));
#29523=CARTESIAN_POINT('Ctrl Pts',(-54.675212093053,-110.238576162073,175.985484901271));
#29524=CARTESIAN_POINT('Ctrl Pts',(-54.6652740992529,-110.145354390049,
174.324310296203));
#29525=CARTESIAN_POINT('Ctrl Pts',(-55.8233454605414,-109.927615017426,
173.149682517375));
#29526=CARTESIAN_POINT('Ctrl Pts',(-56.9814168218299,-109.709875644803,
171.975054738546));
#29527=CARTESIAN_POINT('Ctrl Pts',(-58.623293458487,-109.440559397574,171.975054808055));
#29528=CARTESIAN_POINT('Ctrl Pts',(-60.2651700951441,-109.171243150344,
171.975054877564));
#29529=CARTESIAN_POINT('Ctrl Pts',(-61.4232413586865,-108.953503788142,
173.149682754692));
#29530=CARTESIAN_POINT('Ctrl Pts',(-62.581312622229,-108.735764425939,174.32431063182));
#29531=CARTESIAN_POINT('Ctrl Pts',(-62.571374490195,-108.642542668652,175.985485236888));
#29532=CARTESIAN_POINT('Ctrl Pts',(-62.5614363581611,-108.549320911365,
177.646659841956));
#29533=CARTESIAN_POINT('Ctrl Pts',(-61.3834888710385,-108.580616754677,
178.821287620784));
#29534=CARTESIAN_POINT('Ctrl Pts',(-60.205541383916,-108.61191259799,179.995915399612));
#29535=CARTESIAN_POINT('Ctrl Pts',(-58.5437886214249,-108.694785315908,
179.995915330104));
#29536=CARTESIAN_POINT('Ctrl Pts',(-56.8820358589338,-108.777658033827,
179.995915260595));
#29537=CARTESIAN_POINT('Ctrl Pts',(-55.7040884695573,-108.808953866719,
178.821287383467));
#29538=CARTESIAN_POINT('Ctrl Pts',(-54.5261410801808,-108.840249699611,
177.646659506339));
#29539=CARTESIAN_POINT('Ctrl Pts',(-54.5162030863807,-108.747027927587,
175.985484901271));
#29540=CARTESIAN_POINT('Ctrl Pts',(-54.5062650925806,-108.653806155564,
174.324310296203));
#29541=CARTESIAN_POINT('Ctrl Pts',(-55.6643364538691,-108.436066782941,
173.149682517375));
#29542=CARTESIAN_POINT('Ctrl Pts',(-56.8224078151577,-108.218327410317,
171.975054738546));
#29543=CARTESIAN_POINT('Ctrl Pts',(-58.4642844518147,-107.949011163088,
171.975054808055));
#29544=CARTESIAN_POINT('Ctrl Pts',(-60.1061610884719,-107.679694915859,
171.975054877564));
#29545=CARTESIAN_POINT('Ctrl Pts',(-61.2642323520143,-107.461955553656,
173.149682754692));
#29546=CARTESIAN_POINT('Ctrl Pts',(-62.4223036155567,-107.244216191453,
174.32431063182));
#29547=CARTESIAN_POINT('Ctrl Pts',(-62.4123654835228,-107.150994434166,
175.985485236888));
#29548=CARTESIAN_POINT('Ctrl Pts',(-62.4024273514889,-107.057772676879,
177.646659841956));
#29549=CARTESIAN_POINT('Ctrl Pts',(-61.2244798643663,-107.089068520192,
178.821287620784));
#29550=CARTESIAN_POINT('Ctrl Pts',(-60.0465323772438,-107.120364363504,
179.995915399612));
#29551=CARTESIAN_POINT('Ctrl Pts',(-58.3847796147526,-107.203237081423,
179.995915330104));
#29552=CARTESIAN_POINT('Ctrl Pts',(-56.7230268522615,-107.286109799341,
179.995915260595));
#29553=CARTESIAN_POINT('Ctrl Pts',(-55.5450794628851,-107.317405632233,
178.821287383467));
#29554=CARTESIAN_POINT('Ctrl Pts',(-54.3671320735086,-107.348701465125,
177.646659506339));
#29555=CARTESIAN_POINT('Ctrl Pts',(-54.3571940797085,-107.255479693102,
175.985484901271));
#29556=CARTESIAN_POINT('Ctrl Pts',(-54.3472560859084,-107.162257921078,
174.324310296203));
#29557=CARTESIAN_POINT('Ctrl Pts',(-55.5053274471969,-106.944518548455,
173.149682517375));
#29558=CARTESIAN_POINT('Ctrl Pts',(-56.6633988084854,-106.726779175832,
171.975054738546));
#29559=CARTESIAN_POINT('Ctrl Pts',(-58.3052754451425,-106.457462928602,
171.975054808055));
#29560=CARTESIAN_POINT('Ctrl Pts',(-59.9471520817997,-106.188146681373,
171.975054877564));
#29561=CARTESIAN_POINT('Ctrl Pts',(-61.1052233453421,-105.97040731917,173.149682754692));
#29562=CARTESIAN_POINT('Ctrl Pts',(-62.2632946088845,-105.752667956968,
174.32431063182));
#29563=CARTESIAN_POINT('Ctrl Pts',(-62.2533564768505,-105.659446199681,
175.985485236888));
#29564=CARTESIAN_POINT('Ctrl Pts',(-62.2434183448166,-105.566224442394,
177.646659841956));
#29565=CARTESIAN_POINT('Ctrl Pts',(-61.0654708576941,-105.597520285706,
178.821287620784));
#29566=CARTESIAN_POINT('Ctrl Pts',(-59.8875233705716,-105.628816129018,
179.995915399612));
#29567=CARTESIAN_POINT('Ctrl Pts',(-58.2257706080804,-105.711688846937,
179.995915330104));
#29568=CARTESIAN_POINT('Ctrl Pts',(-56.5640178455893,-105.794561564856,
179.995915260595));
#29569=CARTESIAN_POINT('Ctrl Pts',(-55.3860704562128,-105.825857397748,
178.821287383467));
#29570=CARTESIAN_POINT('Ctrl Pts',(-54.2081230668364,-105.85715323064,177.646659506339));
#29571=CARTESIAN_POINT('Ctrl Pts',(-54.1981850730363,-105.763931458616,
175.985484901271));
#29572=CARTESIAN_POINT('Ctrl Pts',(-54.1882470792362,-105.670709686593,
174.324310296203));
#29573=CARTESIAN_POINT('Ctrl Pts',(-55.3463184405247,-105.452970313969,
173.149682517375));
#29574=CARTESIAN_POINT('Ctrl Pts',(-56.5043898018132,-105.235230941346,
171.975054738546));
#29575=CARTESIAN_POINT('Ctrl Pts',(-58.1462664384703,-104.965914694117,
171.975054808055));
#29576=CARTESIAN_POINT('Ctrl Pts',(-59.7881430751274,-104.696598446888,
171.975054877564));
#29577=CARTESIAN_POINT('Ctrl Pts',(-60.9462143386698,-104.478859084685,
173.149682754692));
#29578=CARTESIAN_POINT('Ctrl Pts',(-62.1042856022123,-104.261119722482,
174.32431063182));
#29579=CARTESIAN_POINT('Ctrl Pts',(-62.0943474701783,-104.167897965195,
175.985485236888));
#29580=CARTESIAN_POINT('Ctrl Pts',(-62.0844093381444,-104.074676207908,
177.646659841956));
#29581=CARTESIAN_POINT('Ctrl Pts',(-60.9064618510219,-104.10597205122,178.821287620784));
#29582=CARTESIAN_POINT('Ctrl Pts',(-59.7285143638993,-104.137267894533,
179.995915399612));
#29583=CARTESIAN_POINT('Ctrl Pts',(-58.0667616014082,-104.220140612451,
179.995915330104));
#29584=CARTESIAN_POINT('Ctrl Pts',(-56.4050088389171,-104.30301333037,179.995915260595));
#29585=CARTESIAN_POINT('Ctrl Pts',(-55.2270614495406,-104.334309163262,
178.821287383467));
#29586=CARTESIAN_POINT('Ctrl Pts',(-54.0491140601642,-104.365604996154,
177.646659506339));
#29587=CARTESIAN_POINT('Ctrl Pts',(-54.039176066364,-104.272383224131,175.985484901271));
#29588=CARTESIAN_POINT('Ctrl Pts',(-54.029238072564,-104.179161452107,174.324310296203));
#29589=CARTESIAN_POINT('Ctrl Pts',(-55.1873094338524,-103.961422079484,
173.149682517375));
#29590=CARTESIAN_POINT('Ctrl Pts',(-56.345380795141,-103.743682706861,171.975054738546));
#29591=CARTESIAN_POINT('Ctrl Pts',(-57.9872574317981,-103.474366459631,
171.975054808055));
#29592=CARTESIAN_POINT('Ctrl Pts',(-59.6291340684552,-103.205050212402,
171.975054877564));
#29593=CARTESIAN_POINT('Ctrl Pts',(-60.7872053319976,-102.987310850199,
173.149682754692));
#29594=CARTESIAN_POINT('Ctrl Pts',(-61.94527659554,-102.769571487996,174.32431063182));
#29595=CARTESIAN_POINT('Ctrl Pts',(-61.9353384635061,-102.676349730709,
175.985485236888));
#29596=CARTESIAN_POINT('Ctrl Pts',(-61.9254003314722,-102.583127973422,
177.646659841956));
#29597=CARTESIAN_POINT('Ctrl Pts',(-60.7474528443496,-102.614423816735,
178.821287620784));
#29598=CARTESIAN_POINT('Ctrl Pts',(-59.5695053572271,-102.645719660047,
179.995915399612));
#29599=CARTESIAN_POINT('Ctrl Pts',(-57.907752594736,-102.728592377966,179.995915330104));
#29600=CARTESIAN_POINT('Ctrl Pts',(-56.2459998322448,-102.811465095885,
179.995915260595));
#29601=CARTESIAN_POINT('Ctrl Pts',(-55.0680524428684,-102.842760928777,
178.821287383467));
#29602=CARTESIAN_POINT('Ctrl Pts',(-53.8901050534919,-102.874056761669,
177.646659506339));
#29603=CARTESIAN_POINT('Ctrl Pts',(-53.8801670596918,-102.780834989645,
175.985484901271));
#29604=CARTESIAN_POINT('Ctrl Pts',(-53.8702290658917,-102.687613217621,
174.324310296203));
#29605=CARTESIAN_POINT('Ctrl Pts',(-55.0283004271802,-102.469873844998,
173.149682517375));
#29606=CARTESIAN_POINT('Ctrl Pts',(-56.1863717884687,-102.252134472375,
171.975054738546));
#29607=CARTESIAN_POINT('Ctrl Pts',(-57.8282484251258,-101.982818225146,
171.975054808055));
#29608=CARTESIAN_POINT('Ctrl Pts',(-59.470125061783,-101.713501977916,171.975054877564));
#29609=CARTESIAN_POINT('Ctrl Pts',(-60.6281963253254,-101.495762615714,
173.149682754692));
#29610=CARTESIAN_POINT('Ctrl Pts',(-61.7862675888678,-101.278023253511,
174.32431063182));
#29611=CARTESIAN_POINT('Ctrl Pts',(-61.7763294568339,-101.184801496224,
175.985485236888));
#29612=CARTESIAN_POINT('Ctrl Pts',(-61.7663913247999,-101.091579738937,
177.646659841956));
#29613=CARTESIAN_POINT('Ctrl Pts',(-60.5884438376774,-101.122875582249,
178.821287620784));
#29614=CARTESIAN_POINT('Ctrl Pts',(-59.4104963505549,-101.154171425562,
179.995915399612));
#29615=CARTESIAN_POINT('Ctrl Pts',(-57.7487435880637,-101.23704414348,179.995915330104));
#29616=CARTESIAN_POINT('Ctrl Pts',(-56.0869908255726,-101.319916861399,
179.995915260595));
#29617=CARTESIAN_POINT('Ctrl Pts',(-54.9090434361961,-101.351212694291,
178.821287383467));
#29618=CARTESIAN_POINT('Ctrl Pts',(-53.7310960468197,-101.382508527183,
177.646659506339));
#29619=CARTESIAN_POINT('Ctrl Pts',(-53.7211580530196,-101.289286755159,
175.985484901271));
#29620=CARTESIAN_POINT('Ctrl Pts',(-53.7112200592195,-101.196064983136,
174.324310296203));
#29621=CARTESIAN_POINT('Ctrl Pts',(-54.869291420508,-100.978325610513,173.149682517375));
#29622=CARTESIAN_POINT('Ctrl Pts',(-56.0273627817965,-100.760586237889,
171.975054738546));
#29623=CARTESIAN_POINT('Ctrl Pts',(-57.6692394184536,-100.49126999066,171.975054808055));
#29624=CARTESIAN_POINT('Ctrl Pts',(-59.3111160551107,-100.221953743431,
171.975054877564));
#29625=CARTESIAN_POINT('Ctrl Pts',(-60.4691873186531,-100.004214381228,
173.149682754692));
#29626=CARTESIAN_POINT('Ctrl Pts',(-61.6272585821956,-99.7864750190253,
174.32431063182));
#29627=CARTESIAN_POINT('Ctrl Pts',(-61.6173204501616,-99.6932532617382,
175.985485236888));
#29628=CARTESIAN_POINT('Ctrl Pts',(-61.6073823181277,-99.6000315044512,
177.646659841956));
#29629=CARTESIAN_POINT('Ctrl Pts',(-60.4294348310052,-99.6313273477637,
178.821287620784));
#29630=CARTESIAN_POINT('Ctrl Pts',(-59.2514873438827,-99.6626231910761,
179.995915399612));
#29631=CARTESIAN_POINT('Ctrl Pts',(-57.5897345813915,-99.7454959089947,
179.995915330104));
#29632=CARTESIAN_POINT('Ctrl Pts',(-55.9279818189004,-99.8283686269133,
179.995915260595));
#29633=CARTESIAN_POINT('Ctrl Pts',(-54.7500344295239,-99.8596644598054,
178.821287383467));
#29634=CARTESIAN_POINT('Ctrl Pts',(-53.5720870401475,-99.8909602926975,
177.646659506339));
#29635=CARTESIAN_POINT('Ctrl Pts',(-53.5621490463474,-99.7977385206737,
175.985484901271));
#29636=CARTESIAN_POINT('Ctrl Pts',(-53.5522110525473,-99.7045167486501,
174.324310296203));
#29637=CARTESIAN_POINT('Ctrl Pts',(-54.7102824138358,-99.4867773760269,
173.149682517375));
#29638=CARTESIAN_POINT('Ctrl Pts',(-55.8683537751243,-99.2690380034038,
171.975054738546));
#29639=CARTESIAN_POINT('Ctrl Pts',(-57.5102304117814,-98.9997217561745,
171.975054808055));
#29640=CARTESIAN_POINT('Ctrl Pts',(-59.1521070484385,-98.7304055089452,
171.975054877564));
#29641=CARTESIAN_POINT('Ctrl Pts',(-60.3101783119809,-98.5126661467424,
173.149682754692));
#29642=CARTESIAN_POINT('Ctrl Pts',(-61.4682495755234,-98.2949267845397,
174.32431063182));
#29643=CARTESIAN_POINT('Ctrl Pts',(-61.4583114434894,-98.2017050272526,
175.985485236888));
#29644=CARTESIAN_POINT('Ctrl Pts',(-61.4483733114555,-98.1084832699656,
177.646659841956));
#29645=CARTESIAN_POINT('Ctrl Pts',(-60.2704258243329,-98.139779113278,178.821287620784));
#29646=CARTESIAN_POINT('Ctrl Pts',(-59.0924783372104,-98.1710749565905,
179.995915399612));
#29647=CARTESIAN_POINT('Ctrl Pts',(-57.4307255747193,-98.2539476745091,
179.995915330104));
#29648=CARTESIAN_POINT('Ctrl Pts',(-55.7689728122282,-98.3368203924277,
179.995915260595));
#29649=CARTESIAN_POINT('Ctrl Pts',(-54.5910254228517,-98.3681162253198,
178.821287383467));
#29650=CARTESIAN_POINT('Ctrl Pts',(-56.1988062143188,-113.449542435949,
178.821287383467));
#29651=CARTESIAN_POINT('Ctrl Pts',(-55.0208588249424,-113.480838268841,
177.646659506339));
#29652=CARTESIAN_POINT('Ctrl Pts',(-55.0109208311422,-113.387616496817,
175.985484901271));
#29653=CARTESIAN_POINT('Ctrl Pts',(-55.0009828373422,-113.294394724794,
174.324310296203));
#29654=CARTESIAN_POINT('Ctrl Pts',(-56.1590541986307,-113.07665535217,173.149682517375));
#29655=CARTESIAN_POINT('Ctrl Pts',(-57.3171255599192,-112.858915979547,
171.975054738546));
#29656=CARTESIAN_POINT('Ctrl Pts',(-58.9590021965763,-112.589599732318,
171.975054808055));
#29657=CARTESIAN_POINT('Ctrl Pts',(-60.6008788332334,-112.320283485089,
171.975054877564));
#29658=CARTESIAN_POINT('Ctrl Pts',(-61.7589500967758,-112.102544122886,
173.149682754692));
#29659=CARTESIAN_POINT('Ctrl Pts',(-62.9170213603182,-111.884804760683,
174.32431063182));
#29660=CARTESIAN_POINT('Ctrl Pts',(-62.9070832282843,-111.791583003396,
175.985485236888));
#29661=CARTESIAN_POINT('Ctrl Pts',(-62.8971450962504,-111.698361246109,
177.646659841956));
#29662=CARTESIAN_POINT('Ctrl Pts',(-61.7191976091278,-111.729657089422,
178.821287620784));
#29663=CARTESIAN_POINT('Ctrl Pts',(-60.5412501220053,-111.760952932734,
179.995915399612));
#29664=CARTESIAN_POINT('Ctrl Pts',(-58.8794973595142,-111.843825650653,
179.995915330104));
#29665=CARTESIAN_POINT('Ctrl Pts',(-57.217744597023,-111.926698368571,179.995915260595));
#29666=CARTESIAN_POINT('Ctrl Pts',(-56.0397972076466,-111.957994201463,
178.821287383467));
#29667=CARTESIAN_POINT('Ctrl Pts',(-54.8618498182701,-111.989290034355,
177.646659506339));
#29668=CARTESIAN_POINT('Ctrl Pts',(-54.85191182447,-111.896068262332,175.985484901271));
#29669=CARTESIAN_POINT('Ctrl Pts',(-54.8419738306699,-111.802846490308,
174.324310296203));
#29670=CARTESIAN_POINT('Ctrl Pts',(-56.0000451919584,-111.585107117685,
173.149682517375));
#29671=CARTESIAN_POINT('Ctrl Pts',(-57.158116553247,-111.367367745062,171.975054738546));
#29672=CARTESIAN_POINT('Ctrl Pts',(-58.799993189904,-111.098051497832,171.975054808055));
#29673=CARTESIAN_POINT('Ctrl Pts',(-60.4418698265612,-110.828735250603,
171.975054877564));
#29674=CARTESIAN_POINT('Ctrl Pts',(-61.5999410901036,-110.6109958884,173.149682754692));
#29675=CARTESIAN_POINT('Ctrl Pts',(-62.758012353646,-110.393256526198,174.32431063182));
#29676=CARTESIAN_POINT('Ctrl Pts',(-62.7480742216121,-110.30003476891,175.985485236888));
#29677=CARTESIAN_POINT('Ctrl Pts',(-62.7381360895782,-110.206813011623,
177.646659841956));
#29678=CARTESIAN_POINT('Ctrl Pts',(-61.5601886024556,-110.238108854936,
178.821287620784));
#29679=CARTESIAN_POINT('Ctrl Pts',(-60.3822411153331,-110.269404698248,
179.995915399612));
#29680=CARTESIAN_POINT('Ctrl Pts',(-58.7204883528419,-110.352277416167,
179.995915330104));
#29681=CARTESIAN_POINT('Ctrl Pts',(-57.0587355903508,-110.435150134086,
179.995915260595));
#29682=CARTESIAN_POINT('Ctrl Pts',(-55.8807882009743,-110.466445966978,
178.821287383467));
#29683=CARTESIAN_POINT('Ctrl Pts',(-54.7028408115979,-110.49774179987,177.646659506339));
#29684=CARTESIAN_POINT('Ctrl Pts',(-54.6929028177978,-110.404520027846,
175.985484901271));
#29685=CARTESIAN_POINT('Ctrl Pts',(-54.6829648239977,-110.311298255822,
174.324310296203));
#29686=CARTESIAN_POINT('Ctrl Pts',(-55.8410361852862,-110.093558883199,
173.149682517375));
#29687=CARTESIAN_POINT('Ctrl Pts',(-56.9991075465747,-109.875819510576,
171.975054738546));
#29688=CARTESIAN_POINT('Ctrl Pts',(-58.6409841832318,-109.606503263347,
171.975054808055));
#29689=CARTESIAN_POINT('Ctrl Pts',(-60.2828608198889,-109.337187016117,
171.975054877564));
#29690=CARTESIAN_POINT('Ctrl Pts',(-61.4409320834313,-109.119447653915,
173.149682754692));
#29691=CARTESIAN_POINT('Ctrl Pts',(-62.5990033469738,-108.901708291712,
174.32431063182));
#29692=CARTESIAN_POINT('Ctrl Pts',(-62.5890652149398,-108.808486534425,
175.985485236888));
#29693=CARTESIAN_POINT('Ctrl Pts',(-62.5791270829059,-108.715264777138,
177.646659841956));
#29694=CARTESIAN_POINT('Ctrl Pts',(-61.4011795957834,-108.74656062045,178.821287620784));
#29695=CARTESIAN_POINT('Ctrl Pts',(-60.2232321086609,-108.777856463763,
179.995915399612));
#29696=CARTESIAN_POINT('Ctrl Pts',(-58.5614793461697,-108.860729181681,
179.995915330104));
#29697=CARTESIAN_POINT('Ctrl Pts',(-56.8997265836786,-108.9436018996,179.995915260595));
#29698=CARTESIAN_POINT('Ctrl Pts',(-55.7217791943021,-108.974897732492,
178.821287383467));
#29699=CARTESIAN_POINT('Ctrl Pts',(-54.5438318049257,-109.006193565384,
177.646659506339));
#29700=CARTESIAN_POINT('Ctrl Pts',(-54.5338938111256,-108.91297179336,175.985484901271));
#29701=CARTESIAN_POINT('Ctrl Pts',(-54.5239558173255,-108.819750021337,
174.324310296203));
#29702=CARTESIAN_POINT('Ctrl Pts',(-55.682027178614,-108.602010648714,173.149682517375));
#29703=CARTESIAN_POINT('Ctrl Pts',(-56.8400985399025,-108.384271276091,
171.975054738546));
#29704=CARTESIAN_POINT('Ctrl Pts',(-58.4819751765596,-108.114955028861,
171.975054808055));
#29705=CARTESIAN_POINT('Ctrl Pts',(-60.1238518132167,-107.845638781632,
171.975054877564));
#29706=CARTESIAN_POINT('Ctrl Pts',(-61.2819230767591,-107.627899419429,
173.149682754692));
#29707=CARTESIAN_POINT('Ctrl Pts',(-62.4399943403016,-107.410160057226,
174.32431063182));
#29708=CARTESIAN_POINT('Ctrl Pts',(-62.4300562082676,-107.316938299939,
175.985485236888));
#29709=CARTESIAN_POINT('Ctrl Pts',(-62.4201180762337,-107.223716542652,
177.646659841956));
#29710=CARTESIAN_POINT('Ctrl Pts',(-61.2421705891111,-107.255012385965,
178.821287620784));
#29711=CARTESIAN_POINT('Ctrl Pts',(-60.0642231019886,-107.286308229277,
179.995915399612));
#29712=CARTESIAN_POINT('Ctrl Pts',(-58.4024703394975,-107.369180947196,
179.995915330104));
#29713=CARTESIAN_POINT('Ctrl Pts',(-56.7407175770064,-107.452053665114,
179.995915260595));
#29714=CARTESIAN_POINT('Ctrl Pts',(-55.5627701876299,-107.483349498006,
178.821287383467));
#29715=CARTESIAN_POINT('Ctrl Pts',(-54.3848227982534,-107.514645330899,
177.646659506339));
#29716=CARTESIAN_POINT('Ctrl Pts',(-54.3748848044533,-107.421423558875,
175.985484901271));
#29717=CARTESIAN_POINT('Ctrl Pts',(-54.3649468106533,-107.328201786851,
174.324310296203));
#29718=CARTESIAN_POINT('Ctrl Pts',(-55.5230181719417,-107.110462414228,
173.149682517375));
#29719=CARTESIAN_POINT('Ctrl Pts',(-56.6810895332303,-106.892723041605,
171.975054738546));
#29720=CARTESIAN_POINT('Ctrl Pts',(-58.3229661698874,-106.623406794376,
171.975054808055));
#29721=CARTESIAN_POINT('Ctrl Pts',(-59.9648428065445,-106.354090547146,
171.975054877564));
#29722=CARTESIAN_POINT('Ctrl Pts',(-61.1229140700869,-106.136351184943,
173.149682754692));
#29723=CARTESIAN_POINT('Ctrl Pts',(-62.2809853336293,-105.918611822741,
174.32431063182));
#29724=CARTESIAN_POINT('Ctrl Pts',(-62.2710472015954,-105.825390065454,
175.985485236888));
#29725=CARTESIAN_POINT('Ctrl Pts',(-62.2611090695615,-105.732168308167,
177.646659841956));
#29726=CARTESIAN_POINT('Ctrl Pts',(-61.0831615824389,-105.763464151479,
178.821287620784));
#29727=CARTESIAN_POINT('Ctrl Pts',(-59.9052140953164,-105.794759994792,
179.995915399612));
#29728=CARTESIAN_POINT('Ctrl Pts',(-58.2434613328252,-105.87763271271,179.995915330104));
#29729=CARTESIAN_POINT('Ctrl Pts',(-56.5817085703341,-105.960505430629,
179.995915260595));
#29730=CARTESIAN_POINT('Ctrl Pts',(-55.4037611809577,-105.991801263521,
178.821287383467));
#29731=CARTESIAN_POINT('Ctrl Pts',(-54.2258137915812,-106.023097096413,
177.646659506339));
#29732=CARTESIAN_POINT('Ctrl Pts',(-54.2158757977811,-105.929875324389,
175.985484901271));
#29733=CARTESIAN_POINT('Ctrl Pts',(-54.205937803981,-105.836653552366,174.324310296203));
#29734=CARTESIAN_POINT('Ctrl Pts',(-55.3640091652695,-105.618914179742,
173.149682517375));
#29735=CARTESIAN_POINT('Ctrl Pts',(-56.522080526558,-105.401174807119,171.975054738546));
#29736=CARTESIAN_POINT('Ctrl Pts',(-58.1639571632151,-105.13185855989,171.975054808055));
#29737=CARTESIAN_POINT('Ctrl Pts',(-59.8058337998722,-104.862542312661,
171.975054877564));
#29738=CARTESIAN_POINT('Ctrl Pts',(-60.9639050634147,-104.644802950458,
173.149682754692));
#29739=CARTESIAN_POINT('Ctrl Pts',(-62.1219763269571,-104.427063588255,
174.32431063182));
#29740=CARTESIAN_POINT('Ctrl Pts',(-62.1120381949232,-104.333841830968,
175.985485236888));
#29741=CARTESIAN_POINT('Ctrl Pts',(-62.1021000628892,-104.240620073681,
177.646659841956));
#29742=CARTESIAN_POINT('Ctrl Pts',(-60.9241525757667,-104.271915916993,
178.821287620784));
#29743=CARTESIAN_POINT('Ctrl Pts',(-59.7462050886442,-104.303211760306,
179.995915399612));
#29744=CARTESIAN_POINT('Ctrl Pts',(-58.084452326153,-104.386084478225,179.995915330104));
#29745=CARTESIAN_POINT('Ctrl Pts',(-56.4226995636619,-104.468957196143,
179.995915260595));
#29746=CARTESIAN_POINT('Ctrl Pts',(-55.2447521742854,-104.500253029035,
178.821287383467));
#29747=CARTESIAN_POINT('Ctrl Pts',(-54.066804784909,-104.531548861927,177.646659506339));
#29748=CARTESIAN_POINT('Ctrl Pts',(-54.0568667911089,-104.438327089904,
175.985484901271));
#29749=CARTESIAN_POINT('Ctrl Pts',(-54.0469287973088,-104.34510531788,174.324310296203));
#29750=CARTESIAN_POINT('Ctrl Pts',(-55.2050001585973,-104.127365945257,
173.149682517375));
#29751=CARTESIAN_POINT('Ctrl Pts',(-56.3630715198858,-103.909626572634,
171.975054738546));
#29752=CARTESIAN_POINT('Ctrl Pts',(-58.0049481565429,-103.640310325404,
171.975054808055));
#29753=CARTESIAN_POINT('Ctrl Pts',(-59.6468247932,-103.370994078175,171.975054877564));
#29754=CARTESIAN_POINT('Ctrl Pts',(-60.8048960567424,-103.153254715972,
173.149682754692));
#29755=CARTESIAN_POINT('Ctrl Pts',(-61.9629673202849,-102.93551535377,174.32431063182));
#29756=CARTESIAN_POINT('Ctrl Pts',(-61.9530291882509,-102.842293596483,
175.985485236888));
#29757=CARTESIAN_POINT('Ctrl Pts',(-61.943091056217,-102.749071839196,177.646659841956));
#29758=CARTESIAN_POINT('Ctrl Pts',(-60.7651435690945,-102.780367682508,
178.821287620784));
#29759=CARTESIAN_POINT('Ctrl Pts',(-59.587196081972,-102.81166352582,179.995915399612));
#29760=CARTESIAN_POINT('Ctrl Pts',(-57.9254433194808,-102.894536243739,
179.995915330104));
#29761=CARTESIAN_POINT('Ctrl Pts',(-56.2636905569897,-102.977408961658,
179.995915260595));
#29762=CARTESIAN_POINT('Ctrl Pts',(-55.0857431676132,-103.00870479455,178.821287383467));
#29763=CARTESIAN_POINT('Ctrl Pts',(-53.9077957782368,-103.040000627442,
177.646659506339));
#29764=CARTESIAN_POINT('Ctrl Pts',(-53.8978577844367,-102.946778855418,
175.985484901271));
#29765=CARTESIAN_POINT('Ctrl Pts',(-53.8879197906366,-102.853557083394,
174.324310296203));
#29766=CARTESIAN_POINT('Ctrl Pts',(-55.0459911519251,-102.635817710771,
173.149682517375));
#29767=CARTESIAN_POINT('Ctrl Pts',(-56.2040625132136,-102.418078338148,
171.975054738546));
#29768=CARTESIAN_POINT('Ctrl Pts',(-57.8459391498707,-102.148762090919,
171.975054808055));
#29769=CARTESIAN_POINT('Ctrl Pts',(-59.4878157865278,-101.879445843689,
171.975054877564));
#29770=CARTESIAN_POINT('Ctrl Pts',(-60.6458870500702,-101.661706481487,
173.149682754692));
#29771=CARTESIAN_POINT('Ctrl Pts',(-61.8039583136126,-101.443967119284,
174.32431063182));
#29772=CARTESIAN_POINT('Ctrl Pts',(-61.7940201815787,-101.350745361997,
175.985485236888));
#29773=CARTESIAN_POINT('Ctrl Pts',(-61.7840820495448,-101.25752360471,177.646659841956));
#29774=CARTESIAN_POINT('Ctrl Pts',(-60.6061345624222,-101.288819448022,
178.821287620784));
#29775=CARTESIAN_POINT('Ctrl Pts',(-59.4281870752997,-101.320115291335,
179.995915399612));
#29776=CARTESIAN_POINT('Ctrl Pts',(-57.7664343128086,-101.402988009253,
179.995915330104));
#29777=CARTESIAN_POINT('Ctrl Pts',(-56.1046815503175,-101.485860727172,
179.995915260595));
#29778=CARTESIAN_POINT('Ctrl Pts',(-54.926734160941,-101.517156560064,178.821287383467));
#29779=CARTESIAN_POINT('Ctrl Pts',(-53.7487867715645,-101.548452392956,
177.646659506339));
#29780=CARTESIAN_POINT('Ctrl Pts',(-53.7388487777644,-101.455230620932,
175.985484901271));
#29781=CARTESIAN_POINT('Ctrl Pts',(-53.7289107839643,-101.362008848909,
174.324310296203));
#29782=CARTESIAN_POINT('Ctrl Pts',(-54.8869821452528,-101.144269476286,
173.149682517375));
#29783=CARTESIAN_POINT('Ctrl Pts',(-56.0450535065414,-100.926530103662,
171.975054738546));
#29784=CARTESIAN_POINT('Ctrl Pts',(-57.6869301431984,-100.657213856433,
171.975054808055));
#29785=CARTESIAN_POINT('Ctrl Pts',(-59.3288067798556,-100.387897609204,
171.975054877564));
#29786=CARTESIAN_POINT('Ctrl Pts',(-60.486878043398,-100.170158247001,173.149682754692));
#29787=CARTESIAN_POINT('Ctrl Pts',(-61.6449493069404,-99.9524188847983,
174.32431063182));
#29788=CARTESIAN_POINT('Ctrl Pts',(-61.6350111749065,-99.8591971275113,
175.985485236888));
#29789=CARTESIAN_POINT('Ctrl Pts',(-61.6250730428726,-99.7659753702243,
177.646659841956));
#29790=CARTESIAN_POINT('Ctrl Pts',(-60.44712555575,-99.7972712135367,178.821287620784));
#29791=CARTESIAN_POINT('Ctrl Pts',(-59.2691780686275,-99.8285670568492,
179.995915399612));
#29792=CARTESIAN_POINT('Ctrl Pts',(-57.6074253061363,-99.9114397747677,
179.995915330104));
#29793=CARTESIAN_POINT('Ctrl Pts',(-55.9456725436452,-99.9943124926864,
179.995915260595));
#29794=CARTESIAN_POINT('Ctrl Pts',(-54.7677251542687,-100.025608325578,
178.821287383467));
#29795=CARTESIAN_POINT('Ctrl Pts',(-53.5897777648923,-100.05690415847,177.646659506339));
#29796=CARTESIAN_POINT('Ctrl Pts',(-53.5798397710922,-99.9636823864468,
175.985484901271));
#29797=CARTESIAN_POINT('Ctrl Pts',(-53.5699017772921,-99.8704606144232,
174.324310296203));
#29798=CARTESIAN_POINT('Ctrl Pts',(-54.7279731385806,-99.6527212418,173.149682517375));
#29799=CARTESIAN_POINT('Ctrl Pts',(-55.8860444998691,-99.4349818691769,
171.975054738546));
#29800=CARTESIAN_POINT('Ctrl Pts',(-57.5279211365262,-99.1656656219475,
171.975054808055));
#29801=CARTESIAN_POINT('Ctrl Pts',(-59.1697977731833,-98.8963493747183,
171.975054877564));
#29802=CARTESIAN_POINT('Ctrl Pts',(-60.3278690367257,-98.6786100125155,
173.149682754692));
#29803=CARTESIAN_POINT('Ctrl Pts',(-61.4859403002682,-98.4608706503128,
174.32431063182));
#29804=CARTESIAN_POINT('Ctrl Pts',(-61.4760021682342,-98.3676488930257,
175.985485236888));
#29805=CARTESIAN_POINT('Ctrl Pts',(-61.4660640362003,-98.2744271357387,
177.646659841956));
#29806=CARTESIAN_POINT('Ctrl Pts',(-60.2881165490778,-98.3057229790511,
178.821287620784));
#29807=CARTESIAN_POINT('Ctrl Pts',(-59.1101690619552,-98.3370188223636,
179.995915399612));
#29808=CARTESIAN_POINT('Ctrl Pts',(-57.4484162994641,-98.4198915402821,
179.995915330104));
#29809=CARTESIAN_POINT('Ctrl Pts',(-55.786663536973,-98.5027642582008,179.995915260595));
#29810=CARTESIAN_POINT('Ctrl Pts',(-54.6087161475965,-98.5340600910929,
178.821287383467));
#29811=CARTESIAN_POINT('Ctrl Pts',(-56.2237961054143,-113.614380048479,
178.813912075476));
#29812=CARTESIAN_POINT('Ctrl Pts',(-55.0488864554725,-113.645352038053,
177.6423391512));
#29813=CARTESIAN_POINT('Ctrl Pts',(-55.0389484614927,-113.552130266048,
175.985484901707));
#29814=CARTESIAN_POINT('Ctrl Pts',(-55.0290104675128,-113.458908494044,
174.328630652215));
#29815=CARTESIAN_POINT('Ctrl Pts',(-56.1840440891124,-113.241492964766,
173.157057825983));
#29816=CARTESIAN_POINT('Ctrl Pts',(-57.3390777107121,-113.024077435489,
171.985484999752));
#29817=CARTESIAN_POINT('Ctrl Pts',(-58.9766583348819,-112.755219171892,
171.985485069079));
#29818=CARTESIAN_POINT('Ctrl Pts',(-60.6142389590518,-112.486360908295,
171.985485138407));
#29819=CARTESIAN_POINT('Ctrl Pts',(-61.7692724831595,-112.268945389411,
173.157058062683));
#29820=CARTESIAN_POINT('Ctrl Pts',(-62.9243060072673,-112.051529870527,
174.328630986959));
#29821=CARTESIAN_POINT('Ctrl Pts',(-62.9143678754131,-111.95830811322,175.985485236451));
#29822=CARTESIAN_POINT('Ctrl Pts',(-62.9044297435589,-111.865086355914,
177.642339485944));
#29823=CARTESIAN_POINT('Ctrl Pts',(-61.7295199961253,-111.896058355881,
178.813912312176));
#29824=CARTESIAN_POINT('Ctrl Pts',(-60.5546102486917,-111.927030355848,
179.985485138407));
#29825=CARTESIAN_POINT('Ctrl Pts',(-58.8971534986878,-112.009445090134,
179.985485069079));
#29826=CARTESIAN_POINT('Ctrl Pts',(-57.2396967486839,-112.09185982442,179.985484999752));
#29827=CARTESIAN_POINT('Ctrl Pts',(-56.0647870987421,-112.122831813994,
178.813912075476));
#29828=CARTESIAN_POINT('Ctrl Pts',(-54.8898774488003,-112.153803803567,
177.6423391512));
#29829=CARTESIAN_POINT('Ctrl Pts',(-54.8799394548205,-112.060582031563,
175.985484901707));
#29830=CARTESIAN_POINT('Ctrl Pts',(-54.8700014608406,-111.967360259558,
174.328630652215));
#29831=CARTESIAN_POINT('Ctrl Pts',(-56.0250350824402,-111.749944730281,
173.157057825983));
#29832=CARTESIAN_POINT('Ctrl Pts',(-57.1800687040398,-111.532529201003,
171.985484999752));
#29833=CARTESIAN_POINT('Ctrl Pts',(-58.8176493282097,-111.263670937406,
171.985485069079));
#29834=CARTESIAN_POINT('Ctrl Pts',(-60.4552299523796,-110.994812673809,
171.985485138407));
#29835=CARTESIAN_POINT('Ctrl Pts',(-61.6102634764873,-110.777397154925,
173.157058062683));
#29836=CARTESIAN_POINT('Ctrl Pts',(-62.7652970005951,-110.559981636041,
174.328630986959));
#29837=CARTESIAN_POINT('Ctrl Pts',(-62.7553588687409,-110.466759878735,
175.985485236451));
#29838=CARTESIAN_POINT('Ctrl Pts',(-62.7454207368867,-110.373538121429,
177.642339485944));
#29839=CARTESIAN_POINT('Ctrl Pts',(-61.5705109894531,-110.404510121395,
178.813912312176));
#29840=CARTESIAN_POINT('Ctrl Pts',(-60.3956012420194,-110.435482121362,
179.985485138407));
#29841=CARTESIAN_POINT('Ctrl Pts',(-58.7381444920155,-110.517896855648,
179.985485069079));
#29842=CARTESIAN_POINT('Ctrl Pts',(-57.0806877420116,-110.600311589935,
179.985484999752));
#29843=CARTESIAN_POINT('Ctrl Pts',(-55.9057780920699,-110.631283579508,
178.813912075476));
#29844=CARTESIAN_POINT('Ctrl Pts',(-54.7308684421281,-110.662255569082,
177.6423391512));
#29845=CARTESIAN_POINT('Ctrl Pts',(-54.7209304481482,-110.569033797077,
175.985484901707));
#29846=CARTESIAN_POINT('Ctrl Pts',(-54.7109924541684,-110.475812025073,
174.328630652215));
#29847=CARTESIAN_POINT('Ctrl Pts',(-55.866026075768,-110.258396495795,173.157057825983));
#29848=CARTESIAN_POINT('Ctrl Pts',(-57.0210596973676,-110.040980966518,
171.985484999752));
#29849=CARTESIAN_POINT('Ctrl Pts',(-58.6586403215375,-109.772122702921,
171.985485069079));
#29850=CARTESIAN_POINT('Ctrl Pts',(-60.2962209457073,-109.503264439324,
171.985485138407));
#29851=CARTESIAN_POINT('Ctrl Pts',(-61.4512544698151,-109.28584892044,173.157058062683));
#29852=CARTESIAN_POINT('Ctrl Pts',(-62.6062879939228,-109.068433401555,
174.328630986959));
#29853=CARTESIAN_POINT('Ctrl Pts',(-62.5963498620687,-108.975211644249,
175.985485236451));
#29854=CARTESIAN_POINT('Ctrl Pts',(-62.5864117302145,-108.881989886943,
177.642339485944));
#29855=CARTESIAN_POINT('Ctrl Pts',(-61.4115019827808,-108.91296188691,178.813912312176));
#29856=CARTESIAN_POINT('Ctrl Pts',(-60.2365922353472,-108.943933886877,
179.985485138407));
#29857=CARTESIAN_POINT('Ctrl Pts',(-58.5791354853433,-109.026348621163,
179.985485069079));
#29858=CARTESIAN_POINT('Ctrl Pts',(-56.9216787353394,-109.108763355449,
179.985484999752));
#29859=CARTESIAN_POINT('Ctrl Pts',(-55.7467690853976,-109.139735345023,
178.813912075476));
#29860=CARTESIAN_POINT('Ctrl Pts',(-54.5718594354559,-109.170707334596,
177.6423391512));
#29861=CARTESIAN_POINT('Ctrl Pts',(-54.561921441476,-109.077485562592,175.985484901707));
#29862=CARTESIAN_POINT('Ctrl Pts',(-54.5519834474962,-108.984263790587,
174.328630652215));
#29863=CARTESIAN_POINT('Ctrl Pts',(-55.7070170690958,-108.76684826131,173.157057825983));
#29864=CARTESIAN_POINT('Ctrl Pts',(-56.8620506906954,-108.549432732032,
171.985484999752));
#29865=CARTESIAN_POINT('Ctrl Pts',(-58.4996313148652,-108.280574468435,
171.985485069079));
#29866=CARTESIAN_POINT('Ctrl Pts',(-60.1372119390351,-108.011716204838,
171.985485138407));
#29867=CARTESIAN_POINT('Ctrl Pts',(-61.2922454631428,-107.794300685954,
173.157058062683));
#29868=CARTESIAN_POINT('Ctrl Pts',(-62.4472789872506,-107.57688516707,174.328630986959));
#29869=CARTESIAN_POINT('Ctrl Pts',(-62.4373408553964,-107.483663409764,
175.985485236451));
#29870=CARTESIAN_POINT('Ctrl Pts',(-62.4274027235423,-107.390441652457,
177.642339485944));
#29871=CARTESIAN_POINT('Ctrl Pts',(-61.2524929761086,-107.421413652424,
178.813912312176));
#29872=CARTESIAN_POINT('Ctrl Pts',(-60.077583228675,-107.452385652391,179.985485138407));
#29873=CARTESIAN_POINT('Ctrl Pts',(-58.4201264786711,-107.534800386677,
179.985485069079));
#29874=CARTESIAN_POINT('Ctrl Pts',(-56.7626697286672,-107.617215120964,
179.985484999752));
#29875=CARTESIAN_POINT('Ctrl Pts',(-55.5877600787254,-107.648187110537,
178.813912075476));
#29876=CARTESIAN_POINT('Ctrl Pts',(-54.4128504287836,-107.67915910011,177.6423391512));
#29877=CARTESIAN_POINT('Ctrl Pts',(-54.4029124348038,-107.585937328106,
175.985484901707));
#29878=CARTESIAN_POINT('Ctrl Pts',(-54.3929744408239,-107.492715556102,
174.328630652215));
#29879=CARTESIAN_POINT('Ctrl Pts',(-55.5480080624235,-107.275300026824,
173.157057825983));
#29880=CARTESIAN_POINT('Ctrl Pts',(-56.7030416840231,-107.057884497547,
171.985484999752));
#29881=CARTESIAN_POINT('Ctrl Pts',(-58.340622308193,-106.78902623395,171.985485069079));
#29882=CARTESIAN_POINT('Ctrl Pts',(-59.9782029323629,-106.520167970353,
171.985485138407));
#29883=CARTESIAN_POINT('Ctrl Pts',(-61.1332364564706,-106.302752451468,
173.157058062683));
#29884=CARTESIAN_POINT('Ctrl Pts',(-62.2882699805784,-106.085336932584,
174.328630986959));
#29885=CARTESIAN_POINT('Ctrl Pts',(-62.2783318487242,-105.992115175278,
175.985485236451));
#29886=CARTESIAN_POINT('Ctrl Pts',(-62.26839371687,-105.898893417972,177.642339485944));
#29887=CARTESIAN_POINT('Ctrl Pts',(-61.0934839694364,-105.929865417939,
178.813912312176));
#29888=CARTESIAN_POINT('Ctrl Pts',(-59.9185742220028,-105.960837417905,
179.985485138407));
#29889=CARTESIAN_POINT('Ctrl Pts',(-58.2611174719989,-106.043252152192,
179.985485069079));
#29890=CARTESIAN_POINT('Ctrl Pts',(-56.603660721995,-106.125666886478,179.985484999752));
#29891=CARTESIAN_POINT('Ctrl Pts',(-55.4287510720532,-106.156638876051,
178.813912075476));
#29892=CARTESIAN_POINT('Ctrl Pts',(-54.2538414221114,-106.187610865625,
177.6423391512));
#29893=CARTESIAN_POINT('Ctrl Pts',(-54.2439034281315,-106.09438909362,175.985484901707));
#29894=CARTESIAN_POINT('Ctrl Pts',(-54.2339654341517,-106.001167321616,
174.328630652215));
#29895=CARTESIAN_POINT('Ctrl Pts',(-55.3889990557513,-105.783751792338,
173.157057825983));
#29896=CARTESIAN_POINT('Ctrl Pts',(-56.5440326773509,-105.566336263061,
171.985484999752));
#29897=CARTESIAN_POINT('Ctrl Pts',(-58.1816133015208,-105.297477999464,
171.985485069079));
#29898=CARTESIAN_POINT('Ctrl Pts',(-59.8191939256906,-105.028619735867,
171.985485138407));
#29899=CARTESIAN_POINT('Ctrl Pts',(-60.9742274497984,-104.811204216983,
173.157058062683));
#29900=CARTESIAN_POINT('Ctrl Pts',(-62.1292609739061,-104.593788698099,
174.328630986959));
#29901=CARTESIAN_POINT('Ctrl Pts',(-62.119322842052,-104.500566940792,175.985485236451));
#29902=CARTESIAN_POINT('Ctrl Pts',(-62.1093847101978,-104.407345183486,
177.642339485944));
#29903=CARTESIAN_POINT('Ctrl Pts',(-60.9344749627642,-104.438317183453,
178.813912312176));
#29904=CARTESIAN_POINT('Ctrl Pts',(-59.7595652153305,-104.46928918342,179.985485138407));
#29905=CARTESIAN_POINT('Ctrl Pts',(-58.1021084653266,-104.551703917706,
179.985485069079));
#29906=CARTESIAN_POINT('Ctrl Pts',(-56.4446517153227,-104.634118651992,
179.985484999752));
#29907=CARTESIAN_POINT('Ctrl Pts',(-55.269742065381,-104.665090641566,178.813912075476));
#29908=CARTESIAN_POINT('Ctrl Pts',(-54.0948324154392,-104.696062631139,
177.6423391512));
#29909=CARTESIAN_POINT('Ctrl Pts',(-54.0848944214593,-104.602840859135,
175.985484901707));
#29910=CARTESIAN_POINT('Ctrl Pts',(-54.0749564274795,-104.50961908713,174.328630652215));
#29911=CARTESIAN_POINT('Ctrl Pts',(-55.2299900490791,-104.292203557853,
173.157057825983));
#29912=CARTESIAN_POINT('Ctrl Pts',(-56.3850236706787,-104.074788028575,
171.985484999752));
#29913=CARTESIAN_POINT('Ctrl Pts',(-58.0226042948486,-103.805929764978,
171.985485069079));
#29914=CARTESIAN_POINT('Ctrl Pts',(-59.6601849190184,-103.537071501381,
171.985485138407));
#29915=CARTESIAN_POINT('Ctrl Pts',(-60.8152184431262,-103.319655982497,
173.157058062683));
#29916=CARTESIAN_POINT('Ctrl Pts',(-61.9702519672339,-103.102240463613,
174.328630986959));
#29917=CARTESIAN_POINT('Ctrl Pts',(-61.9603138353797,-103.009018706307,
175.985485236451));
#29918=CARTESIAN_POINT('Ctrl Pts',(-61.9503757035256,-102.915796949001,
177.642339485944));
#29919=CARTESIAN_POINT('Ctrl Pts',(-60.7754659560919,-102.946768948967,
178.813912312176));
#29920=CARTESIAN_POINT('Ctrl Pts',(-59.6005562086583,-102.977740948934,
179.985485138407));
#29921=CARTESIAN_POINT('Ctrl Pts',(-57.9430994586544,-103.06015568322,179.985485069079));
#29922=CARTESIAN_POINT('Ctrl Pts',(-56.2856427086505,-103.142570417507,
179.985484999752));
#29923=CARTESIAN_POINT('Ctrl Pts',(-55.1107330587087,-103.17354240708,178.813912075476));
#29924=CARTESIAN_POINT('Ctrl Pts',(-53.935823408767,-103.204514396654,177.6423391512));
#29925=CARTESIAN_POINT('Ctrl Pts',(-53.9258854147871,-103.111292624649,
175.985484901707));
#29926=CARTESIAN_POINT('Ctrl Pts',(-53.9159474208072,-103.018070852645,
174.328630652215));
#29927=CARTESIAN_POINT('Ctrl Pts',(-55.0709810424069,-102.800655323367,
173.157057825983));
#29928=CARTESIAN_POINT('Ctrl Pts',(-56.2260146640065,-102.58323979409,171.985484999752));
#29929=CARTESIAN_POINT('Ctrl Pts',(-57.8635952881763,-102.314381530493,
171.985485069079));
#29930=CARTESIAN_POINT('Ctrl Pts',(-59.5011759123462,-102.045523266896,
171.985485138407));
#29931=CARTESIAN_POINT('Ctrl Pts',(-60.6562094364539,-101.828107748012,
173.157058062683));
#29932=CARTESIAN_POINT('Ctrl Pts',(-61.8112429605617,-101.610692229127,
174.328630986959));
#29933=CARTESIAN_POINT('Ctrl Pts',(-61.8013048287075,-101.517470471821,
175.985485236451));
#29934=CARTESIAN_POINT('Ctrl Pts',(-61.7913666968533,-101.424248714515,
177.642339485944));
#29935=CARTESIAN_POINT('Ctrl Pts',(-60.6164569494197,-101.455220714482,
178.813912312176));
#29936=CARTESIAN_POINT('Ctrl Pts',(-59.4415472019861,-101.486192714449,
179.985485138407));
#29937=CARTESIAN_POINT('Ctrl Pts',(-57.7840904519822,-101.568607448735,
179.985485069079));
#29938=CARTESIAN_POINT('Ctrl Pts',(-56.1266337019783,-101.651022183021,
179.985484999752));
#29939=CARTESIAN_POINT('Ctrl Pts',(-54.9517240520365,-101.681994172595,
178.813912075476));
#29940=CARTESIAN_POINT('Ctrl Pts',(-53.7768144020947,-101.712966162168,
177.6423391512));
#29941=CARTESIAN_POINT('Ctrl Pts',(-53.7668764081149,-101.619744390164,
175.985484901707));
#29942=CARTESIAN_POINT('Ctrl Pts',(-53.756938414135,-101.526522618159,174.328630652215));
#29943=CARTESIAN_POINT('Ctrl Pts',(-54.9119720357346,-101.309107088882,
173.157057825983));
#29944=CARTESIAN_POINT('Ctrl Pts',(-56.0670056573342,-101.091691559604,
171.985484999752));
#29945=CARTESIAN_POINT('Ctrl Pts',(-57.7045862815041,-100.822833296007,
171.985485069079));
#29946=CARTESIAN_POINT('Ctrl Pts',(-59.342166905674,-100.55397503241,171.985485138407));
#29947=CARTESIAN_POINT('Ctrl Pts',(-60.4972004297817,-100.336559513526,
173.157058062683));
#29948=CARTESIAN_POINT('Ctrl Pts',(-61.6522339538895,-100.119143994642,
174.328630986959));
#29949=CARTESIAN_POINT('Ctrl Pts',(-61.6422958220353,-100.025922237336,
175.985485236451));
#29950=CARTESIAN_POINT('Ctrl Pts',(-61.6323576901811,-99.9327004800294,
177.642339485944));
#29951=CARTESIAN_POINT('Ctrl Pts',(-60.4574479427475,-99.9636724799962,
178.813912312176));
#29952=CARTESIAN_POINT('Ctrl Pts',(-59.2825381953138,-99.994644479963,179.985485138407));
#29953=CARTESIAN_POINT('Ctrl Pts',(-57.6250814453099,-100.077059214249,
179.985485069079));
#29954=CARTESIAN_POINT('Ctrl Pts',(-55.9676246953061,-100.159473948536,
179.985484999752));
#29955=CARTESIAN_POINT('Ctrl Pts',(-54.7927150453643,-100.190445938109,
178.813912075476));
#29956=CARTESIAN_POINT('Ctrl Pts',(-53.6178053954225,-100.221417927683,
177.6423391512));
#29957=CARTESIAN_POINT('Ctrl Pts',(-53.6078674014426,-100.128196155678,
175.985484901707));
#29958=CARTESIAN_POINT('Ctrl Pts',(-53.5979294074628,-100.034974383673,
174.328630652215));
#29959=CARTESIAN_POINT('Ctrl Pts',(-54.7529630290624,-99.817558854396,173.157057825983));
#29960=CARTESIAN_POINT('Ctrl Pts',(-55.907996650662,-99.6001433251185,171.985484999752));
#29961=CARTESIAN_POINT('Ctrl Pts',(-57.5455772748319,-99.3312850615215,
171.985485069079));
#29962=CARTESIAN_POINT('Ctrl Pts',(-59.1831578990017,-99.0624267979246,
171.985485138407));
#29963=CARTESIAN_POINT('Ctrl Pts',(-60.3381914231095,-98.8450112790404,
173.157058062683));
#29964=CARTESIAN_POINT('Ctrl Pts',(-61.4932249472172,-98.6275957601562,
174.328630986959));
#29965=CARTESIAN_POINT('Ctrl Pts',(-61.4832868153631,-98.53437400285,175.985485236451));
#29966=CARTESIAN_POINT('Ctrl Pts',(-61.4733486835089,-98.4411522455438,
177.642339485944));
#29967=CARTESIAN_POINT('Ctrl Pts',(-60.2984389360752,-98.4721242455106,
178.813912312176));
#29968=CARTESIAN_POINT('Ctrl Pts',(-59.1235291886416,-98.5030962454774,
179.985485138407));
#29969=CARTESIAN_POINT('Ctrl Pts',(-57.4660724386377,-98.5855109797636,
179.985485069079));
#29970=CARTESIAN_POINT('Ctrl Pts',(-55.8086156886338,-98.6679257140499,
179.985484999752));
#29971=CARTESIAN_POINT('Ctrl Pts',(-54.633706038692,-98.6988977036234,178.813912075476));
#29972=CARTESIAN_POINT('Ctrl Pts',(-56.2237961054143,-113.614380048479,
178.813912075476));
#29973=CARTESIAN_POINT('Ctrl Pts',(-55.0488864554725,-113.645352038053,
177.6423391512));
#29974=CARTESIAN_POINT('Ctrl Pts',(-55.0389484614927,-113.552130266048,
175.985484901707));
#29975=CARTESIAN_POINT('Ctrl Pts',(-55.0290104675128,-113.458908494044,
174.328630652215));
#29976=CARTESIAN_POINT('Ctrl Pts',(-56.1840440891124,-113.241492964766,
173.157057825983));
#29977=CARTESIAN_POINT('Ctrl Pts',(-57.3390777107121,-113.024077435489,
171.985484999752));
#29978=CARTESIAN_POINT('Ctrl Pts',(-58.9766583348819,-112.755219171892,
171.985485069079));
#29979=CARTESIAN_POINT('Ctrl Pts',(-60.6142389590518,-112.486360908295,
171.985485138407));
#29980=CARTESIAN_POINT('Ctrl Pts',(-61.7692724831595,-112.268945389411,
173.157058062683));
#29981=CARTESIAN_POINT('Ctrl Pts',(-62.9243060072673,-112.051529870527,
174.328630986959));
#29982=CARTESIAN_POINT('Ctrl Pts',(-62.9143678754131,-111.95830811322,175.985485236451));
#29983=CARTESIAN_POINT('Ctrl Pts',(-62.9044297435589,-111.865086355914,
177.642339485944));
#29984=CARTESIAN_POINT('Ctrl Pts',(-61.7295199961253,-111.896058355881,
178.813912312176));
#29985=CARTESIAN_POINT('Ctrl Pts',(-60.5546102486917,-111.927030355848,
179.985485138407));
#29986=CARTESIAN_POINT('Ctrl Pts',(-58.8971534986878,-112.009445090134,
179.985485069079));
#29987=CARTESIAN_POINT('Ctrl Pts',(-57.2396967486839,-112.09185982442,179.985484999752));
#29988=CARTESIAN_POINT('Ctrl Pts',(-56.0647870987421,-112.122831813994,
178.813912075476));
#29989=CARTESIAN_POINT('Ctrl Pts',(-54.8898774488003,-112.153803803567,
177.6423391512));
#29990=CARTESIAN_POINT('Ctrl Pts',(-54.8799394548205,-112.060582031563,
175.985484901707));
#29991=CARTESIAN_POINT('Ctrl Pts',(-54.8700014608406,-111.967360259558,
174.328630652215));
#29992=CARTESIAN_POINT('Ctrl Pts',(-56.0250350824402,-111.749944730281,
173.157057825983));
#29993=CARTESIAN_POINT('Ctrl Pts',(-57.1800687040398,-111.532529201003,
171.985484999752));
#29994=CARTESIAN_POINT('Ctrl Pts',(-58.8176493282097,-111.263670937406,
171.985485069079));
#29995=CARTESIAN_POINT('Ctrl Pts',(-60.4552299523796,-110.994812673809,
171.985485138407));
#29996=CARTESIAN_POINT('Ctrl Pts',(-61.6102634764873,-110.777397154925,
173.157058062683));
#29997=CARTESIAN_POINT('Ctrl Pts',(-62.7652970005951,-110.559981636041,
174.328630986959));
#29998=CARTESIAN_POINT('Ctrl Pts',(-62.7553588687409,-110.466759878735,
175.985485236451));
#29999=CARTESIAN_POINT('Ctrl Pts',(-62.7454207368867,-110.373538121429,
177.642339485944));
#30000=CARTESIAN_POINT('Ctrl Pts',(-61.5705109894531,-110.404510121395,
178.813912312176));
#30001=CARTESIAN_POINT('Ctrl Pts',(-60.3956012420194,-110.435482121362,
179.985485138407));
#30002=CARTESIAN_POINT('Ctrl Pts',(-58.7381444920155,-110.517896855648,
179.985485069079));
#30003=CARTESIAN_POINT('Ctrl Pts',(-57.0806877420116,-110.600311589935,
179.985484999752));
#30004=CARTESIAN_POINT('Ctrl Pts',(-55.9057780920699,-110.631283579508,
178.813912075476));
#30005=CARTESIAN_POINT('Ctrl Pts',(-54.7308684421281,-110.662255569082,
177.6423391512));
#30006=CARTESIAN_POINT('Ctrl Pts',(-54.7209304481482,-110.569033797077,
175.985484901707));
#30007=CARTESIAN_POINT('Ctrl Pts',(-54.7109924541684,-110.475812025073,
174.328630652215));
#30008=CARTESIAN_POINT('Ctrl Pts',(-55.866026075768,-110.258396495795,173.157057825983));
#30009=CARTESIAN_POINT('Ctrl Pts',(-57.0210596973676,-110.040980966518,
171.985484999752));
#30010=CARTESIAN_POINT('Ctrl Pts',(-58.6586403215375,-109.772122702921,
171.985485069079));
#30011=CARTESIAN_POINT('Ctrl Pts',(-60.2962209457073,-109.503264439324,
171.985485138407));
#30012=CARTESIAN_POINT('Ctrl Pts',(-61.4512544698151,-109.28584892044,173.157058062683));
#30013=CARTESIAN_POINT('Ctrl Pts',(-62.6062879939228,-109.068433401555,
174.328630986959));
#30014=CARTESIAN_POINT('Ctrl Pts',(-62.5963498620687,-108.975211644249,
175.985485236451));
#30015=CARTESIAN_POINT('Ctrl Pts',(-62.5864117302145,-108.881989886943,
177.642339485944));
#30016=CARTESIAN_POINT('Ctrl Pts',(-61.4115019827808,-108.91296188691,178.813912312176));
#30017=CARTESIAN_POINT('Ctrl Pts',(-60.2365922353472,-108.943933886877,
179.985485138407));
#30018=CARTESIAN_POINT('Ctrl Pts',(-58.5791354853433,-109.026348621163,
179.985485069079));
#30019=CARTESIAN_POINT('Ctrl Pts',(-56.9216787353394,-109.108763355449,
179.985484999752));
#30020=CARTESIAN_POINT('Ctrl Pts',(-55.7467690853976,-109.139735345023,
178.813912075476));
#30021=CARTESIAN_POINT('Ctrl Pts',(-54.5718594354559,-109.170707334596,
177.6423391512));
#30022=CARTESIAN_POINT('Ctrl Pts',(-54.561921441476,-109.077485562592,175.985484901707));
#30023=CARTESIAN_POINT('Ctrl Pts',(-54.5519834474962,-108.984263790587,
174.328630652215));
#30024=CARTESIAN_POINT('Ctrl Pts',(-55.7070170690958,-108.76684826131,173.157057825983));
#30025=CARTESIAN_POINT('Ctrl Pts',(-56.8620506906954,-108.549432732032,
171.985484999752));
#30026=CARTESIAN_POINT('Ctrl Pts',(-58.4996313148652,-108.280574468435,
171.985485069079));
#30027=CARTESIAN_POINT('Ctrl Pts',(-60.1372119390351,-108.011716204838,
171.985485138407));
#30028=CARTESIAN_POINT('Ctrl Pts',(-61.2922454631428,-107.794300685954,
173.157058062683));
#30029=CARTESIAN_POINT('Ctrl Pts',(-62.4472789872506,-107.57688516707,174.328630986959));
#30030=CARTESIAN_POINT('Ctrl Pts',(-62.4373408553964,-107.483663409764,
175.985485236451));
#30031=CARTESIAN_POINT('Ctrl Pts',(-62.4274027235423,-107.390441652457,
177.642339485944));
#30032=CARTESIAN_POINT('Ctrl Pts',(-61.2524929761086,-107.421413652424,
178.813912312176));
#30033=CARTESIAN_POINT('Ctrl Pts',(-60.077583228675,-107.452385652391,179.985485138407));
#30034=CARTESIAN_POINT('Ctrl Pts',(-58.4201264786711,-107.534800386677,
179.985485069079));
#30035=CARTESIAN_POINT('Ctrl Pts',(-56.7626697286672,-107.617215120964,
179.985484999752));
#30036=CARTESIAN_POINT('Ctrl Pts',(-55.5877600787254,-107.648187110537,
178.813912075476));
#30037=CARTESIAN_POINT('Ctrl Pts',(-54.4128504287836,-107.67915910011,177.6423391512));
#30038=CARTESIAN_POINT('Ctrl Pts',(-54.4029124348038,-107.585937328106,
175.985484901707));
#30039=CARTESIAN_POINT('Ctrl Pts',(-54.3929744408239,-107.492715556102,
174.328630652215));
#30040=CARTESIAN_POINT('Ctrl Pts',(-55.5480080624235,-107.275300026824,
173.157057825983));
#30041=CARTESIAN_POINT('Ctrl Pts',(-56.7030416840231,-107.057884497547,
171.985484999752));
#30042=CARTESIAN_POINT('Ctrl Pts',(-58.340622308193,-106.78902623395,171.985485069079));
#30043=CARTESIAN_POINT('Ctrl Pts',(-59.9782029323629,-106.520167970353,
171.985485138407));
#30044=CARTESIAN_POINT('Ctrl Pts',(-61.1332364564706,-106.302752451468,
173.157058062683));
#30045=CARTESIAN_POINT('Ctrl Pts',(-62.2882699805784,-106.085336932584,
174.328630986959));
#30046=CARTESIAN_POINT('Ctrl Pts',(-62.2783318487242,-105.992115175278,
175.985485236451));
#30047=CARTESIAN_POINT('Ctrl Pts',(-62.26839371687,-105.898893417972,177.642339485944));
#30048=CARTESIAN_POINT('Ctrl Pts',(-61.0934839694364,-105.929865417939,
178.813912312176));
#30049=CARTESIAN_POINT('Ctrl Pts',(-59.9185742220028,-105.960837417905,
179.985485138407));
#30050=CARTESIAN_POINT('Ctrl Pts',(-58.2611174719989,-106.043252152192,
179.985485069079));
#30051=CARTESIAN_POINT('Ctrl Pts',(-56.603660721995,-106.125666886478,179.985484999752));
#30052=CARTESIAN_POINT('Ctrl Pts',(-55.4287510720532,-106.156638876051,
178.813912075476));
#30053=CARTESIAN_POINT('Ctrl Pts',(-54.2538414221114,-106.187610865625,
177.6423391512));
#30054=CARTESIAN_POINT('Ctrl Pts',(-54.2439034281315,-106.09438909362,175.985484901707));
#30055=CARTESIAN_POINT('Ctrl Pts',(-54.2339654341517,-106.001167321616,
174.328630652215));
#30056=CARTESIAN_POINT('Ctrl Pts',(-55.3889990557513,-105.783751792338,
173.157057825983));
#30057=CARTESIAN_POINT('Ctrl Pts',(-56.5440326773509,-105.566336263061,
171.985484999752));
#30058=CARTESIAN_POINT('Ctrl Pts',(-58.1816133015208,-105.297477999464,
171.985485069079));
#30059=CARTESIAN_POINT('Ctrl Pts',(-59.8191939256906,-105.028619735867,
171.985485138407));
#30060=CARTESIAN_POINT('Ctrl Pts',(-60.9742274497984,-104.811204216983,
173.157058062683));
#30061=CARTESIAN_POINT('Ctrl Pts',(-62.1292609739061,-104.593788698099,
174.328630986959));
#30062=CARTESIAN_POINT('Ctrl Pts',(-62.119322842052,-104.500566940792,175.985485236451));
#30063=CARTESIAN_POINT('Ctrl Pts',(-62.1093847101978,-104.407345183486,
177.642339485944));
#30064=CARTESIAN_POINT('Ctrl Pts',(-60.9344749627642,-104.438317183453,
178.813912312176));
#30065=CARTESIAN_POINT('Ctrl Pts',(-59.7595652153305,-104.46928918342,179.985485138407));
#30066=CARTESIAN_POINT('Ctrl Pts',(-58.1021084653266,-104.551703917706,
179.985485069079));
#30067=CARTESIAN_POINT('Ctrl Pts',(-56.4446517153227,-104.634118651992,
179.985484999752));
#30068=CARTESIAN_POINT('Ctrl Pts',(-55.269742065381,-104.665090641566,178.813912075476));
#30069=CARTESIAN_POINT('Ctrl Pts',(-54.0948324154392,-104.696062631139,
177.6423391512));
#30070=CARTESIAN_POINT('Ctrl Pts',(-54.0848944214593,-104.602840859135,
175.985484901707));
#30071=CARTESIAN_POINT('Ctrl Pts',(-54.0749564274795,-104.50961908713,174.328630652215));
#30072=CARTESIAN_POINT('Ctrl Pts',(-55.2299900490791,-104.292203557853,
173.157057825983));
#30073=CARTESIAN_POINT('Ctrl Pts',(-56.3850236706787,-104.074788028575,
171.985484999752));
#30074=CARTESIAN_POINT('Ctrl Pts',(-58.0226042948486,-103.805929764978,
171.985485069079));
#30075=CARTESIAN_POINT('Ctrl Pts',(-59.6601849190184,-103.537071501381,
171.985485138407));
#30076=CARTESIAN_POINT('Ctrl Pts',(-60.8152184431262,-103.319655982497,
173.157058062683));
#30077=CARTESIAN_POINT('Ctrl Pts',(-61.9702519672339,-103.102240463613,
174.328630986959));
#30078=CARTESIAN_POINT('Ctrl Pts',(-61.9603138353797,-103.009018706307,
175.985485236451));
#30079=CARTESIAN_POINT('Ctrl Pts',(-61.9503757035256,-102.915796949001,
177.642339485944));
#30080=CARTESIAN_POINT('Ctrl Pts',(-60.7754659560919,-102.946768948967,
178.813912312176));
#30081=CARTESIAN_POINT('Ctrl Pts',(-59.6005562086583,-102.977740948934,
179.985485138407));
#30082=CARTESIAN_POINT('Ctrl Pts',(-57.9430994586544,-103.06015568322,179.985485069079));
#30083=CARTESIAN_POINT('Ctrl Pts',(-56.2856427086505,-103.142570417507,
179.985484999752));
#30084=CARTESIAN_POINT('Ctrl Pts',(-55.1107330587087,-103.17354240708,178.813912075476));
#30085=CARTESIAN_POINT('Ctrl Pts',(-53.935823408767,-103.204514396654,177.6423391512));
#30086=CARTESIAN_POINT('Ctrl Pts',(-53.9258854147871,-103.111292624649,
175.985484901707));
#30087=CARTESIAN_POINT('Ctrl Pts',(-53.9159474208072,-103.018070852645,
174.328630652215));
#30088=CARTESIAN_POINT('Ctrl Pts',(-55.0709810424069,-102.800655323367,
173.157057825983));
#30089=CARTESIAN_POINT('Ctrl Pts',(-56.2260146640065,-102.58323979409,171.985484999752));
#30090=CARTESIAN_POINT('Ctrl Pts',(-57.8635952881763,-102.314381530493,
171.985485069079));
#30091=CARTESIAN_POINT('Ctrl Pts',(-59.5011759123462,-102.045523266896,
171.985485138407));
#30092=CARTESIAN_POINT('Ctrl Pts',(-60.6562094364539,-101.828107748012,
173.157058062683));
#30093=CARTESIAN_POINT('Ctrl Pts',(-61.8112429605617,-101.610692229127,
174.328630986959));
#30094=CARTESIAN_POINT('Ctrl Pts',(-61.8013048287075,-101.517470471821,
175.985485236451));
#30095=CARTESIAN_POINT('Ctrl Pts',(-61.7913666968533,-101.424248714515,
177.642339485944));
#30096=CARTESIAN_POINT('Ctrl Pts',(-60.6164569494197,-101.455220714482,
178.813912312176));
#30097=CARTESIAN_POINT('Ctrl Pts',(-59.4415472019861,-101.486192714449,
179.985485138407));
#30098=CARTESIAN_POINT('Ctrl Pts',(-57.7840904519822,-101.568607448735,
179.985485069079));
#30099=CARTESIAN_POINT('Ctrl Pts',(-56.1266337019783,-101.651022183021,
179.985484999752));
#30100=CARTESIAN_POINT('Ctrl Pts',(-54.9517240520365,-101.681994172595,
178.813912075476));
#30101=CARTESIAN_POINT('Ctrl Pts',(-53.7768144020947,-101.712966162168,
177.6423391512));
#30102=CARTESIAN_POINT('Ctrl Pts',(-53.7668764081149,-101.619744390164,
175.985484901707));
#30103=CARTESIAN_POINT('Ctrl Pts',(-53.756938414135,-101.526522618159,174.328630652215));
#30104=CARTESIAN_POINT('Ctrl Pts',(-54.9119720357346,-101.309107088882,
173.157057825983));
#30105=CARTESIAN_POINT('Ctrl Pts',(-56.0670056573342,-101.091691559604,
171.985484999752));
#30106=CARTESIAN_POINT('Ctrl Pts',(-57.7045862815041,-100.822833296007,
171.985485069079));
#30107=CARTESIAN_POINT('Ctrl Pts',(-59.342166905674,-100.55397503241,171.985485138407));
#30108=CARTESIAN_POINT('Ctrl Pts',(-60.4972004297817,-100.336559513526,
173.157058062683));
#30109=CARTESIAN_POINT('Ctrl Pts',(-61.6522339538895,-100.119143994642,
174.328630986959));
#30110=CARTESIAN_POINT('Ctrl Pts',(-61.6422958220353,-100.025922237336,
175.985485236451));
#30111=CARTESIAN_POINT('Ctrl Pts',(-61.6323576901811,-99.9327004800294,
177.642339485944));
#30112=CARTESIAN_POINT('Ctrl Pts',(-60.4574479427475,-99.9636724799962,
178.813912312176));
#30113=CARTESIAN_POINT('Ctrl Pts',(-59.2825381953138,-99.994644479963,179.985485138407));
#30114=CARTESIAN_POINT('Ctrl Pts',(-57.6250814453099,-100.077059214249,
179.985485069079));
#30115=CARTESIAN_POINT('Ctrl Pts',(-55.9676246953061,-100.159473948536,
179.985484999752));
#30116=CARTESIAN_POINT('Ctrl Pts',(-54.7927150453643,-100.190445938109,
178.813912075476));
#30117=CARTESIAN_POINT('Ctrl Pts',(-53.6178053954225,-100.221417927683,
177.6423391512));
#30118=CARTESIAN_POINT('Ctrl Pts',(-53.6078674014426,-100.128196155678,
175.985484901707));
#30119=CARTESIAN_POINT('Ctrl Pts',(-53.5979294074628,-100.034974383673,
174.328630652215));
#30120=CARTESIAN_POINT('Ctrl Pts',(-54.7529630290624,-99.817558854396,173.157057825983));
#30121=CARTESIAN_POINT('Ctrl Pts',(-55.907996650662,-99.6001433251185,171.985484999752));
#30122=CARTESIAN_POINT('Ctrl Pts',(-57.5455772748319,-99.3312850615215,
171.985485069079));
#30123=CARTESIAN_POINT('Ctrl Pts',(-59.1831578990017,-99.0624267979246,
171.985485138407));
#30124=CARTESIAN_POINT('Ctrl Pts',(-60.3381914231095,-98.8450112790404,
173.157058062683));
#30125=CARTESIAN_POINT('Ctrl Pts',(-61.4932249472172,-98.6275957601562,
174.328630986959));
#30126=CARTESIAN_POINT('Ctrl Pts',(-61.4832868153631,-98.53437400285,175.985485236451));
#30127=CARTESIAN_POINT('Ctrl Pts',(-61.4733486835089,-98.4411522455438,
177.642339485944));
#30128=CARTESIAN_POINT('Ctrl Pts',(-60.2984389360752,-98.4721242455106,
178.813912312176));
#30129=CARTESIAN_POINT('Ctrl Pts',(-59.1235291886416,-98.5030962454774,
179.985485138407));
#30130=CARTESIAN_POINT('Ctrl Pts',(-57.4660724386377,-98.5855109797636,
179.985485069079));
#30131=CARTESIAN_POINT('Ctrl Pts',(-55.8086156886338,-98.6679257140499,
179.985484999752));
#30132=CARTESIAN_POINT('Ctrl Pts',(-54.633706038692,-98.6988977036234,178.813912075476));
#30133=CARTESIAN_POINT('Ctrl Pts',(-56.9964983346804,-113.864655531781,
178.072094410988));
#30134=CARTESIAN_POINT('Ctrl Pts',(-56.1271283009022,-113.863054956993,
177.207792449865));
#30135=CARTESIAN_POINT('Ctrl Pts',(-56.117190288842,-113.769833186916,175.985484945604));
#30136=CARTESIAN_POINT('Ctrl Pts',(-56.1072522767819,-113.676611416839,
174.763177441344));
#30137=CARTESIAN_POINT('Ctrl Pts',(-56.9567462566485,-113.491768454648,
173.89887555255));
#30138=CARTESIAN_POINT('Ctrl Pts',(-57.8062402365152,-113.306925492458,
173.034573663757));
#30139=CARTESIAN_POINT('Ctrl Pts',(-59.011722573584,-113.084131793069,173.034573714903));
#30140=CARTESIAN_POINT('Ctrl Pts',(-60.2172049106529,-112.86133809368,173.034573766048));
#30141=CARTESIAN_POINT('Ctrl Pts',(-61.0666988185971,-112.676495139156,
173.898875727171));
#30142=CARTESIAN_POINT('Ctrl Pts',(-61.9161927265413,-112.491652184633,
174.763177688294));
#30143=CARTESIAN_POINT('Ctrl Pts',(-61.9062546127674,-112.398430425399,
175.985485192554));
#30144=CARTESIAN_POINT('Ctrl Pts',(-61.8963164989935,-112.305208666166,
177.207792696815));
#30145=CARTESIAN_POINT('Ctrl Pts',(-61.0269463932928,-112.303608099046,
178.072094585608));
#30146=CARTESIAN_POINT('Ctrl Pts',(-60.1575762875921,-112.302007531926,
178.936396474401));
#30147=CARTESIAN_POINT('Ctrl Pts',(-58.9322178246893,-112.338357702004,
178.936396423256));
#30148=CARTESIAN_POINT('Ctrl Pts',(-57.7068593617864,-112.374707872082,
178.936396372111));
#30149=CARTESIAN_POINT('Ctrl Pts',(-56.8374893280082,-112.373107297295,
178.072094410988));
#30150=CARTESIAN_POINT('Ctrl Pts',(-55.9681192942299,-112.371506722508,
177.207792449865));
#30151=CARTESIAN_POINT('Ctrl Pts',(-55.9581812821698,-112.278284952431,
175.985484945604));
#30152=CARTESIAN_POINT('Ctrl Pts',(-55.9482432701096,-112.185063182354,
174.763177441344));
#30153=CARTESIAN_POINT('Ctrl Pts',(-56.7977372499763,-112.000220220163,
173.89887555255));
#30154=CARTESIAN_POINT('Ctrl Pts',(-57.647231229843,-111.815377257972,173.034573663757));
#30155=CARTESIAN_POINT('Ctrl Pts',(-58.8527135669118,-111.592583558583,
173.034573714903));
#30156=CARTESIAN_POINT('Ctrl Pts',(-60.0581959039807,-111.369789859194,
173.034573766048));
#30157=CARTESIAN_POINT('Ctrl Pts',(-60.9076898119249,-111.184946904671,
173.898875727171));
#30158=CARTESIAN_POINT('Ctrl Pts',(-61.7571837198691,-111.000103950148,
174.763177688294));
#30159=CARTESIAN_POINT('Ctrl Pts',(-61.7472456060952,-110.906882190914,
175.985485192554));
#30160=CARTESIAN_POINT('Ctrl Pts',(-61.7373074923213,-110.81366043168,177.207792696815));
#30161=CARTESIAN_POINT('Ctrl Pts',(-60.8679373866206,-110.81205986456,178.072094585608));
#30162=CARTESIAN_POINT('Ctrl Pts',(-59.9985672809199,-110.81045929744,178.936396474401));
#30163=CARTESIAN_POINT('Ctrl Pts',(-58.7732088180171,-110.846809467519,
178.936396423256));
#30164=CARTESIAN_POINT('Ctrl Pts',(-57.5478503551142,-110.883159637597,
178.936396372111));
#30165=CARTESIAN_POINT('Ctrl Pts',(-56.6784803213359,-110.881559062809,
178.072094410988));
#30166=CARTESIAN_POINT('Ctrl Pts',(-55.8091102875577,-110.879958488022,
177.207792449865));
#30167=CARTESIAN_POINT('Ctrl Pts',(-55.7991722754976,-110.786736717945,
175.985484945604));
#30168=CARTESIAN_POINT('Ctrl Pts',(-55.7892342634374,-110.693514947868,
174.763177441344));
#30169=CARTESIAN_POINT('Ctrl Pts',(-56.6387282433041,-110.508671985677,
173.89887555255));
#30170=CARTESIAN_POINT('Ctrl Pts',(-57.4882222231708,-110.323829023487,
173.034573663757));
#30171=CARTESIAN_POINT('Ctrl Pts',(-58.6937045602396,-110.101035324098,
173.034573714903));
#30172=CARTESIAN_POINT('Ctrl Pts',(-59.8991868973084,-109.878241624709,
173.034573766048));
#30173=CARTESIAN_POINT('Ctrl Pts',(-60.7486808052526,-109.693398670185,
173.898875727171));
#30174=CARTESIAN_POINT('Ctrl Pts',(-61.5981747131968,-109.508555715662,
174.763177688294));
#30175=CARTESIAN_POINT('Ctrl Pts',(-61.588236599423,-109.415333956428,175.985485192554));
#30176=CARTESIAN_POINT('Ctrl Pts',(-61.5782984856491,-109.322112197195,
177.207792696815));
#30177=CARTESIAN_POINT('Ctrl Pts',(-60.7089283799484,-109.320511630075,
178.072094585608));
#30178=CARTESIAN_POINT('Ctrl Pts',(-59.8395582742477,-109.318911062955,
178.936396474401));
#30179=CARTESIAN_POINT('Ctrl Pts',(-58.6141998113448,-109.355261233033,
178.936396423256));
#30180=CARTESIAN_POINT('Ctrl Pts',(-57.388841348442,-109.391611403111,178.936396372111));
#30181=CARTESIAN_POINT('Ctrl Pts',(-56.5194713146637,-109.390010828324,
178.072094410988));
#30182=CARTESIAN_POINT('Ctrl Pts',(-55.6501012808855,-109.388410253536,
177.207792449865));
#30183=CARTESIAN_POINT('Ctrl Pts',(-55.6401632688253,-109.295188483459,
175.985484945604));
#30184=CARTESIAN_POINT('Ctrl Pts',(-55.6302252567652,-109.201966713382,
174.763177441344));
#30185=CARTESIAN_POINT('Ctrl Pts',(-56.4797192366319,-109.017123751192,
173.89887555255));
#30186=CARTESIAN_POINT('Ctrl Pts',(-57.3292132164985,-108.832280789001,
173.034573663757));
#30187=CARTESIAN_POINT('Ctrl Pts',(-58.5346955535674,-108.609487089612,
173.034573714903));
#30188=CARTESIAN_POINT('Ctrl Pts',(-59.7401778906362,-108.386693390223,
173.034573766048));
#30189=CARTESIAN_POINT('Ctrl Pts',(-60.5896717985804,-108.2018504357,173.898875727171));
#30190=CARTESIAN_POINT('Ctrl Pts',(-61.4391657065246,-108.017007481176,
174.763177688294));
#30191=CARTESIAN_POINT('Ctrl Pts',(-61.4292275927507,-107.923785721943,
175.985485192554));
#30192=CARTESIAN_POINT('Ctrl Pts',(-61.4192894789769,-107.830563962709,
177.207792696815));
#30193=CARTESIAN_POINT('Ctrl Pts',(-60.5499193732762,-107.828963395589,
178.072094585608));
#30194=CARTESIAN_POINT('Ctrl Pts',(-59.6805492675755,-107.827362828469,
178.936396474401));
#30195=CARTESIAN_POINT('Ctrl Pts',(-58.4551908046726,-107.863712998547,
178.936396423256));
#30196=CARTESIAN_POINT('Ctrl Pts',(-57.2298323417698,-107.900063168626,
178.936396372111));
#30197=CARTESIAN_POINT('Ctrl Pts',(-56.3604623079915,-107.898462593838,
178.072094410988));
#30198=CARTESIAN_POINT('Ctrl Pts',(-55.4910922742133,-107.896862019051,
177.207792449865));
#30199=CARTESIAN_POINT('Ctrl Pts',(-55.4811542621531,-107.803640248974,
175.985484945604));
#30200=CARTESIAN_POINT('Ctrl Pts',(-55.471216250093,-107.710418478897,174.763177441344));
#30201=CARTESIAN_POINT('Ctrl Pts',(-56.3207102299596,-107.525575516706,
173.89887555255));
#30202=CARTESIAN_POINT('Ctrl Pts',(-57.1702042098263,-107.340732554515,
173.034573663757));
#30203=CARTESIAN_POINT('Ctrl Pts',(-58.3756865468951,-107.117938855126,
173.034573714903));
#30204=CARTESIAN_POINT('Ctrl Pts',(-59.581168883964,-106.895145155737,173.034573766048));
#30205=CARTESIAN_POINT('Ctrl Pts',(-60.4306627919082,-106.710302201214,
173.898875727171));
#30206=CARTESIAN_POINT('Ctrl Pts',(-61.2801566998524,-106.525459246691,
174.763177688294));
#30207=CARTESIAN_POINT('Ctrl Pts',(-61.2702185860785,-106.432237487457,
175.985485192554));
#30208=CARTESIAN_POINT('Ctrl Pts',(-61.2602804723046,-106.339015728223,
177.207792696815));
#30209=CARTESIAN_POINT('Ctrl Pts',(-60.3909103666039,-106.337415161103,
178.072094585608));
#30210=CARTESIAN_POINT('Ctrl Pts',(-59.5215402609032,-106.335814593983,
178.936396474401));
#30211=CARTESIAN_POINT('Ctrl Pts',(-58.2961817980004,-106.372164764062,
178.936396423256));
#30212=CARTESIAN_POINT('Ctrl Pts',(-57.0708233350975,-106.40851493414,178.936396372111));
#30213=CARTESIAN_POINT('Ctrl Pts',(-56.2014533013193,-106.406914359353,
178.072094410988));
#30214=CARTESIAN_POINT('Ctrl Pts',(-55.332083267541,-106.405313784565,177.207792449865));
#30215=CARTESIAN_POINT('Ctrl Pts',(-55.3221452554809,-106.312092014488,
175.985484945604));
#30216=CARTESIAN_POINT('Ctrl Pts',(-55.3122072434207,-106.218870244411,
174.763177441344));
#30217=CARTESIAN_POINT('Ctrl Pts',(-56.1617012232874,-106.034027282221,
173.89887555255));
#30218=CARTESIAN_POINT('Ctrl Pts',(-57.0111952031541,-105.84918432003,173.034573663757));
#30219=CARTESIAN_POINT('Ctrl Pts',(-58.2166775402229,-105.626390620641,
173.034573714903));
#30220=CARTESIAN_POINT('Ctrl Pts',(-59.4221598772917,-105.403596921252,
173.034573766048));
#30221=CARTESIAN_POINT('Ctrl Pts',(-60.2716537852359,-105.218753966728,
173.898875727171));
#30222=CARTESIAN_POINT('Ctrl Pts',(-61.1211476931802,-105.033911012205,
174.763177688294));
#30223=CARTESIAN_POINT('Ctrl Pts',(-61.1112095794063,-104.940689252971,
175.985485192554));
#30224=CARTESIAN_POINT('Ctrl Pts',(-61.1012714656324,-104.847467493738,
177.207792696815));
#30225=CARTESIAN_POINT('Ctrl Pts',(-60.2319013599317,-104.845866926618,
178.072094585608));
#30226=CARTESIAN_POINT('Ctrl Pts',(-59.362531254231,-104.844266359498,178.936396474401));
#30227=CARTESIAN_POINT('Ctrl Pts',(-58.1371727913281,-104.880616529576,
178.936396423256));
#30228=CARTESIAN_POINT('Ctrl Pts',(-56.9118143284253,-104.916966699654,
178.936396372111));
#30229=CARTESIAN_POINT('Ctrl Pts',(-56.042444294647,-104.915366124867,178.072094410988));
#30230=CARTESIAN_POINT('Ctrl Pts',(-55.1730742608688,-104.91376555008,177.207792449865));
#30231=CARTESIAN_POINT('Ctrl Pts',(-55.1631362488087,-104.820543780003,
175.985484945604));
#30232=CARTESIAN_POINT('Ctrl Pts',(-55.1531982367485,-104.727322009926,
174.763177441344));
#30233=CARTESIAN_POINT('Ctrl Pts',(-56.0026922166152,-104.542479047735,
173.89887555255));
#30234=CARTESIAN_POINT('Ctrl Pts',(-56.8521861964818,-104.357636085544,
173.034573663757));
#30235=CARTESIAN_POINT('Ctrl Pts',(-58.0576685335507,-104.134842386155,
173.034573714903));
#30236=CARTESIAN_POINT('Ctrl Pts',(-59.2631508706195,-103.912048686766,
173.034573766048));
#30237=CARTESIAN_POINT('Ctrl Pts',(-60.1126447785637,-103.727205732243,
173.898875727171));
#30238=CARTESIAN_POINT('Ctrl Pts',(-60.9621386865079,-103.54236277772,174.763177688294));
#30239=CARTESIAN_POINT('Ctrl Pts',(-60.952200572734,-103.449141018486,175.985485192554));
#30240=CARTESIAN_POINT('Ctrl Pts',(-60.9422624589602,-103.355919259252,
177.207792696815));
#30241=CARTESIAN_POINT('Ctrl Pts',(-60.0728923532595,-103.354318692132,
178.072094585608));
#30242=CARTESIAN_POINT('Ctrl Pts',(-59.2035222475588,-103.352718125012,
178.936396474401));
#30243=CARTESIAN_POINT('Ctrl Pts',(-57.9781637846559,-103.389068295091,
178.936396423256));
#30244=CARTESIAN_POINT('Ctrl Pts',(-56.7528053217531,-103.425418465169,
178.936396372111));
#30245=CARTESIAN_POINT('Ctrl Pts',(-55.8834352879748,-103.423817890381,
178.072094410988));
#30246=CARTESIAN_POINT('Ctrl Pts',(-55.0140652541966,-103.422217315594,
177.207792449865));
#30247=CARTESIAN_POINT('Ctrl Pts',(-55.0041272421364,-103.328995545517,
175.985484945604));
#30248=CARTESIAN_POINT('Ctrl Pts',(-54.9941892300763,-103.23577377544,174.763177441344));
#30249=CARTESIAN_POINT('Ctrl Pts',(-55.8436832099429,-103.050930813249,
173.89887555255));
#30250=CARTESIAN_POINT('Ctrl Pts',(-56.6931771898096,-102.866087851059,
173.034573663757));
#30251=CARTESIAN_POINT('Ctrl Pts',(-57.8986595268784,-102.64329415167,173.034573714903));
#30252=CARTESIAN_POINT('Ctrl Pts',(-59.1041418639473,-102.420500452281,
173.034573766048));
#30253=CARTESIAN_POINT('Ctrl Pts',(-59.9536357718915,-102.235657497757,
173.898875727171));
#30254=CARTESIAN_POINT('Ctrl Pts',(-60.8031296798357,-102.050814543234,
174.763177688294));
#30255=CARTESIAN_POINT('Ctrl Pts',(-60.7931915660618,-101.957592784,175.985485192554));
#30256=CARTESIAN_POINT('Ctrl Pts',(-60.783253452288,-101.864371024767,177.207792696815));
#30257=CARTESIAN_POINT('Ctrl Pts',(-59.9138833465873,-101.862770457647,
178.072094585608));
#30258=CARTESIAN_POINT('Ctrl Pts',(-59.0445132408866,-101.861169890527,
178.936396474401));
#30259=CARTESIAN_POINT('Ctrl Pts',(-57.8191547779837,-101.897520060605,
178.936396423256));
#30260=CARTESIAN_POINT('Ctrl Pts',(-56.5937963150808,-101.933870230683,
178.936396372111));
#30261=CARTESIAN_POINT('Ctrl Pts',(-55.7244262813026,-101.932269655896,
178.072094410988));
#30262=CARTESIAN_POINT('Ctrl Pts',(-54.8550562475244,-101.930669081108,
177.207792449865));
#30263=CARTESIAN_POINT('Ctrl Pts',(-54.8451182354642,-101.837447311031,
175.985484945604));
#30264=CARTESIAN_POINT('Ctrl Pts',(-54.8351802234041,-101.744225540954,
174.763177441344));
#30265=CARTESIAN_POINT('Ctrl Pts',(-55.6846742032707,-101.559382578764,
173.89887555255));
#30266=CARTESIAN_POINT('Ctrl Pts',(-56.5341681831374,-101.374539616573,
173.034573663757));
#30267=CARTESIAN_POINT('Ctrl Pts',(-57.7396505202062,-101.151745917184,
173.034573714903));
#30268=CARTESIAN_POINT('Ctrl Pts',(-58.9451328572751,-100.928952217795,
173.034573766048));
#30269=CARTESIAN_POINT('Ctrl Pts',(-59.7946267652193,-100.744109263272,
173.898875727171));
#30270=CARTESIAN_POINT('Ctrl Pts',(-60.6441206731635,-100.559266308748,
174.763177688294));
#30271=CARTESIAN_POINT('Ctrl Pts',(-60.6341825593896,-100.466044549515,
175.985485192554));
#30272=CARTESIAN_POINT('Ctrl Pts',(-60.6242444456157,-100.372822790281,
177.207792696815));
#30273=CARTESIAN_POINT('Ctrl Pts',(-59.754874339915,-100.371222223161,178.072094585608));
#30274=CARTESIAN_POINT('Ctrl Pts',(-58.8855042342143,-100.369621656041,
178.936396474401));
#30275=CARTESIAN_POINT('Ctrl Pts',(-57.6601457713115,-100.405971826119,
178.936396423256));
#30276=CARTESIAN_POINT('Ctrl Pts',(-56.4347873084086,-100.442321996198,
178.936396372111));
#30277=CARTESIAN_POINT('Ctrl Pts',(-55.5654172746304,-100.44072142141,178.072094410988));
#30278=CARTESIAN_POINT('Ctrl Pts',(-54.6960472408521,-100.439120846623,
177.207792449865));
#30279=CARTESIAN_POINT('Ctrl Pts',(-54.686109228792,-100.345899076546,175.985484945604));
#30280=CARTESIAN_POINT('Ctrl Pts',(-54.6761712167318,-100.252677306469,
174.763177441344));
#30281=CARTESIAN_POINT('Ctrl Pts',(-55.5256651965985,-100.067834344278,
173.89887555255));
#30282=CARTESIAN_POINT('Ctrl Pts',(-56.3751591764652,-99.8829913820874,
173.034573663757));
#30283=CARTESIAN_POINT('Ctrl Pts',(-57.580641513534,-99.6601976826983,173.034573714903));
#30284=CARTESIAN_POINT('Ctrl Pts',(-58.7861238506028,-99.4374039833093,
173.034573766048));
#30285=CARTESIAN_POINT('Ctrl Pts',(-59.635617758547,-99.252561028786,173.898875727171));
#30286=CARTESIAN_POINT('Ctrl Pts',(-60.4851116664912,-99.0677180742627,
174.763177688294));
#30287=CARTESIAN_POINT('Ctrl Pts',(-60.4751735527174,-98.9744963150291,
175.985485192554));
#30288=CARTESIAN_POINT('Ctrl Pts',(-60.4652354389435,-98.8812745557954,
177.207792696815));
#30289=CARTESIAN_POINT('Ctrl Pts',(-59.5958653332428,-98.8796739886754,
178.072094585608));
#30290=CARTESIAN_POINT('Ctrl Pts',(-58.7264952275421,-98.8780734215554,
178.936396474401));
#30291=CARTESIAN_POINT('Ctrl Pts',(-57.5011367646392,-98.9144235916337,
178.936396423256));
#30292=CARTESIAN_POINT('Ctrl Pts',(-56.2757783017364,-98.9507737617121,
178.936396372111));
#30293=CARTESIAN_POINT('Ctrl Pts',(-55.4064082679581,-98.9491731869247,
178.072094410988));
#30294=CARTESIAN_POINT('Ctrl Pts',(-61.229590586797,-104.432475997293,178.485485069079));
#30295=CARTESIAN_POINT('Ctrl Pts',(-61.0910183824403,-104.434190515171,
178.657813499464));
#30296=CARTESIAN_POINT('Ctrl Pts',(-60.9344749627642,-104.438317183453,
178.813912312176));
#30297=CARTESIAN_POINT('Ctrl Pts',(-59.7595652153305,-104.46928918342,179.985485138407));
#30298=CARTESIAN_POINT('Ctrl Pts',(-58.1021084653266,-104.551703917706,
179.985485069079));
#30299=CARTESIAN_POINT('Ctrl Pts',(-56.4446517153227,-104.634118651992,
179.985484999752));
#30300=CARTESIAN_POINT('Ctrl Pts',(-55.269742065381,-104.665090641566,178.813912075476));
#30301=CARTESIAN_POINT('Ctrl Pts',(-54.0948324154392,-104.696062631139,
177.6423391512));
#30302=CARTESIAN_POINT('Ctrl Pts',(-54.0848944214593,-104.602840859135,
175.985484901707));
#30303=CARTESIAN_POINT('Ctrl Pts',(-54.0749564274795,-104.50961908713,174.328630652215));
#30304=CARTESIAN_POINT('Ctrl Pts',(-55.2299900490791,-104.292203557853,
173.157057825983));
#30305=CARTESIAN_POINT('Ctrl Pts',(-56.3850236706787,-104.074788028575,
171.985484999752));
#30306=CARTESIAN_POINT('Ctrl Pts',(-58.0226042948486,-103.805929764978,
171.985485069079));
#30307=CARTESIAN_POINT('Ctrl Pts',(-59.6601849190184,-103.537071501381,
171.985485138407));
#30308=CARTESIAN_POINT('Ctrl Pts',(-60.8152184431262,-103.319655982497,
173.157058062683));
#30309=CARTESIAN_POINT('Ctrl Pts',(-60.9691134640793,-103.290687848555,
173.313156769748));
#30310=CARTESIAN_POINT('Ctrl Pts',(-61.1049326680501,-103.263150419372,
173.485485069079));
#30311=CARTESIAN_POINT('Ctrl Pts',(-56.8733667677527,-112.709647553905,
178.072094410988));
#30312=CARTESIAN_POINT('Ctrl Pts',(-56.0039967339745,-112.708046979118,
177.207792449865));
#30313=CARTESIAN_POINT('Ctrl Pts',(-55.9940587219143,-112.614825209041,
175.985484945604));
#30314=CARTESIAN_POINT('Ctrl Pts',(-55.9841207098542,-112.521603438964,
174.763177441344));
#30315=CARTESIAN_POINT('Ctrl Pts',(-56.8336146897208,-112.336760476773,
173.89887555255));
#30316=CARTESIAN_POINT('Ctrl Pts',(-57.6831086695875,-112.151917514582,
173.034573663757));
#30317=CARTESIAN_POINT('Ctrl Pts',(-58.8885910066563,-111.929123815193,
173.034573714903));
#30318=CARTESIAN_POINT('Ctrl Pts',(-60.0940733437252,-111.706330115804,
173.034573766048));
#30319=CARTESIAN_POINT('Ctrl Pts',(-60.9435672516694,-111.521487161281,
173.898875727171));
#30320=CARTESIAN_POINT('Ctrl Pts',(-61.7930611596136,-111.336644206758,
174.763177688294));
#30321=CARTESIAN_POINT('Ctrl Pts',(-61.7831230458397,-111.243422447524,
175.985485192554));
#30322=CARTESIAN_POINT('Ctrl Pts',(-61.7731849320658,-111.15020068829,177.207792696815));
#30323=CARTESIAN_POINT('Ctrl Pts',(-60.9038148263651,-111.14860012117,178.072094585608));
#30324=CARTESIAN_POINT('Ctrl Pts',(-60.0344447206644,-111.14699955405,178.936396474401));
#30325=CARTESIAN_POINT('Ctrl Pts',(-58.8090862577616,-111.183349724129,
178.936396423256));
#30326=CARTESIAN_POINT('Ctrl Pts',(-57.5837277948587,-111.219699894207,
178.936396372111));
#30327=CARTESIAN_POINT('Ctrl Pts',(-56.7143577610805,-111.21809931942,178.072094410988));
#30328=CARTESIAN_POINT('Ctrl Pts',(-55.8449877273022,-111.216498744632,
177.207792449865));
#30329=CARTESIAN_POINT('Ctrl Pts',(-55.8350497152421,-111.123276974555,
175.985484945604));
#30330=CARTESIAN_POINT('Ctrl Pts',(-55.8251117031819,-111.030055204478,
174.763177441344));
#30331=CARTESIAN_POINT('Ctrl Pts',(-56.6746056830486,-110.845212242287,
173.89887555255));
#30332=CARTESIAN_POINT('Ctrl Pts',(-57.5240996629153,-110.660369280097,
173.034573663757));
#30333=CARTESIAN_POINT('Ctrl Pts',(-58.7295819999841,-110.437575580708,
173.034573714903));
#30334=CARTESIAN_POINT('Ctrl Pts',(-59.9350643370529,-110.214781881319,
173.034573766048));
#30335=CARTESIAN_POINT('Ctrl Pts',(-60.7845582449971,-110.029938926795,
173.898875727171));
#30336=CARTESIAN_POINT('Ctrl Pts',(-61.6340521529414,-109.845095972272,
174.763177688294));
#30337=CARTESIAN_POINT('Ctrl Pts',(-61.6241140391675,-109.751874213038,
175.985485192554));
#30338=CARTESIAN_POINT('Ctrl Pts',(-61.6141759253936,-109.658652453805,
177.207792696815));
#30339=CARTESIAN_POINT('Ctrl Pts',(-60.7448058196929,-109.657051886685,
178.072094585608));
#30340=CARTESIAN_POINT('Ctrl Pts',(-59.8754357139922,-109.655451319565,
178.936396474401));
#30341=CARTESIAN_POINT('Ctrl Pts',(-58.6500772510893,-109.691801489643,
178.936396423256));
#30342=CARTESIAN_POINT('Ctrl Pts',(-57.4247187881865,-109.728151659721,
178.936396372111));
#30343=CARTESIAN_POINT('Ctrl Pts',(-56.5553487544082,-109.726551084934,
178.072094410988));
#30344=CARTESIAN_POINT('Ctrl Pts',(-55.68597872063,-109.724950510147,177.207792449865));
#30345=CARTESIAN_POINT('Ctrl Pts',(-55.6760407085698,-109.63172874007,175.985484945604));
#30346=CARTESIAN_POINT('Ctrl Pts',(-55.6661026965097,-109.538506969993,
174.763177441344));
#30347=CARTESIAN_POINT('Ctrl Pts',(-56.5155966763764,-109.353664007802,
173.89887555255));
#30348=CARTESIAN_POINT('Ctrl Pts',(-57.365090656243,-109.168821045611,173.034573663757));
#30349=CARTESIAN_POINT('Ctrl Pts',(-58.5705729933119,-108.946027346222,
173.034573714903));
#30350=CARTESIAN_POINT('Ctrl Pts',(-59.7760553303807,-108.723233646833,
173.034573766048));
#30351=CARTESIAN_POINT('Ctrl Pts',(-60.6255492383249,-108.53839069231,173.898875727171));
#30352=CARTESIAN_POINT('Ctrl Pts',(-61.4750431462691,-108.353547737786,
174.763177688294));
#30353=CARTESIAN_POINT('Ctrl Pts',(-61.4651050324952,-108.260325978553,
175.985485192554));
#30354=CARTESIAN_POINT('Ctrl Pts',(-61.4551669187214,-108.167104219319,
177.207792696815));
#30355=CARTESIAN_POINT('Ctrl Pts',(-60.5857968130207,-108.165503652199,
178.072094585608));
#30356=CARTESIAN_POINT('Ctrl Pts',(-59.71642670732,-108.163903085079,178.936396474401));
#30357=CARTESIAN_POINT('Ctrl Pts',(-58.4910682444171,-108.200253255158,
178.936396423256));
#30358=CARTESIAN_POINT('Ctrl Pts',(-57.2657097815143,-108.236603425236,
178.936396372111));
#30359=CARTESIAN_POINT('Ctrl Pts',(-56.396339747736,-108.235002850448,178.072094410988));
#30360=CARTESIAN_POINT('Ctrl Pts',(-55.5269697139578,-108.233402275661,
177.207792449865));
#30361=CARTESIAN_POINT('Ctrl Pts',(-55.5170317018976,-108.140180505584,
175.985484945604));
#30362=CARTESIAN_POINT('Ctrl Pts',(-55.5070936898375,-108.046958735507,
174.763177441344));
#30363=CARTESIAN_POINT('Ctrl Pts',(-56.3565876697041,-107.862115773316,
173.89887555255));
#30364=CARTESIAN_POINT('Ctrl Pts',(-57.2060816495708,-107.677272811126,
173.034573663757));
#30365=CARTESIAN_POINT('Ctrl Pts',(-58.4115639866396,-107.454479111736,
173.034573714903));
#30366=CARTESIAN_POINT('Ctrl Pts',(-59.6170463237085,-107.231685412347,
173.034573766048));
#30367=CARTESIAN_POINT('Ctrl Pts',(-60.4665402316527,-107.046842457824,
173.898875727171));
#30368=CARTESIAN_POINT('Ctrl Pts',(-61.3160341395969,-106.861999503301,
174.763177688294));
#30369=CARTESIAN_POINT('Ctrl Pts',(-61.306096025823,-106.768777744067,175.985485192554));
#30370=CARTESIAN_POINT('Ctrl Pts',(-61.2961579120492,-106.675555984834,
177.207792696815));
#30371=CARTESIAN_POINT('Ctrl Pts',(-60.4267878063484,-106.673955417714,
178.072094585608));
#30372=CARTESIAN_POINT('Ctrl Pts',(-59.5574177006478,-106.672354850594,
178.936396474401));
#30373=CARTESIAN_POINT('Ctrl Pts',(-58.3320592377449,-106.708705020672,
178.936396423256));
#30374=CARTESIAN_POINT('Ctrl Pts',(-57.106700774842,-106.74505519075,178.936396372111));
#30375=CARTESIAN_POINT('Ctrl Pts',(-56.2373307410638,-106.743454615963,
178.072094410988));
#30376=CARTESIAN_POINT('Ctrl Pts',(-55.3679607072856,-106.741854041175,
177.207792449865));
#30377=CARTESIAN_POINT('Ctrl Pts',(-55.3580226952254,-106.648632271098,
175.985484945604));
#30378=CARTESIAN_POINT('Ctrl Pts',(-55.3480846831652,-106.555410501021,
174.763177441344));
#30379=CARTESIAN_POINT('Ctrl Pts',(-56.1975786630319,-106.370567538831,
173.89887555255));
#30380=CARTESIAN_POINT('Ctrl Pts',(-57.0470726428986,-106.18572457664,173.034573663757));
#30381=CARTESIAN_POINT('Ctrl Pts',(-58.2525549799674,-105.962930877251,
173.034573714903));
#30382=CARTESIAN_POINT('Ctrl Pts',(-59.4580373170363,-105.740137177862,
173.034573766048));
#30383=CARTESIAN_POINT('Ctrl Pts',(-60.3075312249805,-105.555294223339,
173.898875727171));
#30384=CARTESIAN_POINT('Ctrl Pts',(-61.1570251329247,-105.370451268815,
174.763177688294));
#30385=CARTESIAN_POINT('Ctrl Pts',(-61.1470870191508,-105.277229509582,
175.985485192554));
#30386=CARTESIAN_POINT('Ctrl Pts',(-61.1371489053769,-105.184007750348,
177.207792696815));
#30387=CARTESIAN_POINT('Ctrl Pts',(-60.2677787996762,-105.182407183228,
178.072094585608));
#30388=CARTESIAN_POINT('Ctrl Pts',(-59.3984086939755,-105.180806616108,
178.936396474401));
#30389=CARTESIAN_POINT('Ctrl Pts',(-58.1730502310727,-105.217156786186,
178.936396423256));
#30390=CARTESIAN_POINT('Ctrl Pts',(-56.9476917681698,-105.253506956265,
178.936396372111));
#30391=CARTESIAN_POINT('Ctrl Pts',(-56.0783217343916,-105.251906381477,
178.072094410988));
#30392=CARTESIAN_POINT('Ctrl Pts',(-55.2089517006133,-105.25030580669,177.207792449865));
#30393=CARTESIAN_POINT('Ctrl Pts',(-55.1990136885532,-105.157084036613,
175.985484945604));
#30394=CARTESIAN_POINT('Ctrl Pts',(-55.189075676493,-105.063862266536,174.763177441344));
#30395=CARTESIAN_POINT('Ctrl Pts',(-56.0385696563597,-104.879019304345,
173.89887555255));
#30396=CARTESIAN_POINT('Ctrl Pts',(-56.8880636362264,-104.694176342154,
173.034573663757));
#30397=CARTESIAN_POINT('Ctrl Pts',(-58.0935459732952,-104.471382642765,
173.034573714903));
#30398=CARTESIAN_POINT('Ctrl Pts',(-59.299028310364,-104.248588943376,173.034573766048));
#30399=CARTESIAN_POINT('Ctrl Pts',(-60.1485222183082,-104.063745988853,
173.898875727171));
#30400=CARTESIAN_POINT('Ctrl Pts',(-60.9980161262524,-103.87890303433,174.763177688294));
#30401=CARTESIAN_POINT('Ctrl Pts',(-60.9880780124786,-103.785681275096,
175.985485192554));
#30402=CARTESIAN_POINT('Ctrl Pts',(-60.9781398987047,-103.692459515862,
177.207792696815));
#30403=CARTESIAN_POINT('Ctrl Pts',(-60.108769793004,-103.690858948742,178.072094585608));
#30404=CARTESIAN_POINT('Ctrl Pts',(-59.2393996873033,-103.689258381622,
178.936396474401));
#30405=CARTESIAN_POINT('Ctrl Pts',(-58.0140412244004,-103.725608551701,
178.936396423256));
#30406=CARTESIAN_POINT('Ctrl Pts',(-56.7886827614976,-103.761958721779,
178.936396372111));
#30407=CARTESIAN_POINT('Ctrl Pts',(-55.9193127277193,-103.760358146992,
178.072094410988));
#30408=CARTESIAN_POINT('Ctrl Pts',(-55.0499426939411,-103.758757572204,
177.207792449865));
#30409=CARTESIAN_POINT('Ctrl Pts',(-55.0400046818809,-103.665535802127,
175.985484945604));
#30410=CARTESIAN_POINT('Ctrl Pts',(-55.0300666698208,-103.57231403205,174.763177441344));
#30411=CARTESIAN_POINT('Ctrl Pts',(-55.8795606496874,-103.387471069859,
173.89887555255));
#30412=CARTESIAN_POINT('Ctrl Pts',(-56.7290546295541,-103.202628107669,
173.034573663757));
#30413=CARTESIAN_POINT('Ctrl Pts',(-57.934536966623,-102.97983440828,173.034573714903));
#30414=CARTESIAN_POINT('Ctrl Pts',(-59.1400193036918,-102.757040708891,
173.034573766048));
#30415=CARTESIAN_POINT('Ctrl Pts',(-59.989513211636,-102.572197754367,173.898875727171));
#30416=CARTESIAN_POINT('Ctrl Pts',(-60.8390071195802,-102.387354799844,
174.763177688294));
#30417=CARTESIAN_POINT('Ctrl Pts',(-60.8290690058063,-102.29413304061,175.985485192554));
#30418=CARTESIAN_POINT('Ctrl Pts',(-60.8191308920325,-102.200911281377,
177.207792696815));
#30419=CARTESIAN_POINT('Ctrl Pts',(-59.9497607863318,-102.199310714257,
178.072094585608));
#30420=CARTESIAN_POINT('Ctrl Pts',(-59.0803906806311,-102.197710147137,
178.936396474401));
#30421=CARTESIAN_POINT('Ctrl Pts',(-57.8550322177282,-102.234060317215,
178.936396423256));
#30422=CARTESIAN_POINT('Ctrl Pts',(-56.6296737548253,-102.270410487293,
178.936396372111));
#30423=CARTESIAN_POINT('Ctrl Pts',(-55.7603037210471,-102.268809912506,
178.072094410988));
#30424=CARTESIAN_POINT('Ctrl Pts',(-54.8909336872689,-102.267209337719,
177.207792449865));
#30425=CARTESIAN_POINT('Ctrl Pts',(-54.8809956752087,-102.173987567642,
175.985484945604));
#30426=CARTESIAN_POINT('Ctrl Pts',(-54.8710576631486,-102.080765797565,
174.763177441344));
#30427=CARTESIAN_POINT('Ctrl Pts',(-55.7205516430152,-101.895922835374,
173.89887555255));
#30428=CARTESIAN_POINT('Ctrl Pts',(-56.5700456228819,-101.711079873183,
173.034573663757));
#30429=CARTESIAN_POINT('Ctrl Pts',(-57.7755279599507,-101.488286173794,
173.034573714903));
#30430=CARTESIAN_POINT('Ctrl Pts',(-58.9810102970196,-101.265492474405,
173.034573766048));
#30431=CARTESIAN_POINT('Ctrl Pts',(-59.8305042049638,-101.080649519882,
173.898875727171));
#30432=CARTESIAN_POINT('Ctrl Pts',(-60.679998112908,-100.895806565358,174.763177688294));
#30433=CARTESIAN_POINT('Ctrl Pts',(-60.6700599991341,-100.802584806125,
175.985485192554));
#30434=CARTESIAN_POINT('Ctrl Pts',(-60.6601218853602,-100.709363046891,
177.207792696815));
#30435=CARTESIAN_POINT('Ctrl Pts',(-59.7907517796595,-100.707762479771,
178.072094585608));
#30436=CARTESIAN_POINT('Ctrl Pts',(-58.9213816739588,-100.706161912651,
178.936396474401));
#30437=CARTESIAN_POINT('Ctrl Pts',(-57.696023211056,-100.742512082729,178.936396423256));
#30438=CARTESIAN_POINT('Ctrl Pts',(-56.4706647481531,-100.778862252808,
178.936396372111));
#30439=CARTESIAN_POINT('Ctrl Pts',(-55.6012947143749,-100.77726167802,178.072094410988));
#30440=CARTESIAN_POINT('Ctrl Pts',(-54.7319246805966,-100.775661103233,
177.207792449865));
#30441=CARTESIAN_POINT('Ctrl Pts',(-54.7219866685365,-100.682439333156,
175.985484945604));
#30442=CARTESIAN_POINT('Ctrl Pts',(-54.7120486564763,-100.589217563079,
174.763177441344));
#30443=CARTESIAN_POINT('Ctrl Pts',(-55.561542636343,-100.404374600888,173.89887555255));
#30444=CARTESIAN_POINT('Ctrl Pts',(-56.4110366162097,-100.219531638698,
173.034573663757));
#30445=CARTESIAN_POINT('Ctrl Pts',(-57.6165189532785,-99.9967379393085,
173.034573714903));
#30446=CARTESIAN_POINT('Ctrl Pts',(-58.8220012903473,-99.7739442399195,
173.034573766048));
#30447=CARTESIAN_POINT('Ctrl Pts',(-59.6714951982915,-99.5891012853962,
173.898875727171));
#30448=CARTESIAN_POINT('Ctrl Pts',(-60.5209891062358,-99.4042583308729,
174.763177688294));
#30449=CARTESIAN_POINT('Ctrl Pts',(-60.5110509924619,-99.3110365716392,
175.985485192554));
#30450=CARTESIAN_POINT('Ctrl Pts',(-60.501112878688,-99.2178148124055,177.207792696815));
#30451=CARTESIAN_POINT('Ctrl Pts',(-59.6317427729873,-99.2162142452855,
178.072094585608));
#30452=CARTESIAN_POINT('Ctrl Pts',(-58.7623726672866,-99.2146136781656,
178.936396474401));
#30453=CARTESIAN_POINT('Ctrl Pts',(-57.5370142043838,-99.2509638482439,
178.936396423256));
#30454=CARTESIAN_POINT('Ctrl Pts',(-56.3116557414809,-99.2873140183222,
178.936396372111));
#30455=CARTESIAN_POINT('Ctrl Pts',(-55.4422857077027,-99.2857134435348,
178.072094410988));
#30456=CARTESIAN_POINT('Ctrl Pts',(-54.5729156739244,-99.2841128687474,
177.207792449865));
#30457=CARTESIAN_POINT('Ctrl Pts',(-54.5629776618643,-99.1908910986704,
175.985484945604));
#30458=CARTESIAN_POINT('Ctrl Pts',(-54.5530396498041,-99.0976693285933,
174.763177441344));
#30459=CARTESIAN_POINT('Ctrl Pts',(-55.4025336296708,-98.9128263664026,
173.89887555255));
#30460=CARTESIAN_POINT('Ctrl Pts',(-56.2520276095374,-98.727983404212,173.034573663757));
#30461=CARTESIAN_POINT('Ctrl Pts',(-57.4575099466063,-98.5051897048229,
173.034573714903));
#30462=CARTESIAN_POINT('Ctrl Pts',(-58.6629922836751,-98.2823960054338,
173.034573766048));
#30463=CARTESIAN_POINT('Ctrl Pts',(-59.5124861916193,-98.0975530509106,
173.898875727171));
#30464=CARTESIAN_POINT('Ctrl Pts',(-60.3619800995635,-97.9127100963873,
174.763177688294));
#30465=CARTESIAN_POINT('Ctrl Pts',(-60.3520419857897,-97.8194883371536,
175.985485192554));
#30466=CARTESIAN_POINT('Ctrl Pts',(-60.3421038720158,-97.7262665779199,
177.207792696815));
#30467=CARTESIAN_POINT('Ctrl Pts',(-59.4727337663151,-97.7246660108,178.072094585608));
#30468=CARTESIAN_POINT('Ctrl Pts',(-58.6033636606144,-97.72306544368,178.936396474401));
#30469=CARTESIAN_POINT('Ctrl Pts',(-57.3780051977115,-97.7594156137583,
178.936396423256));
#30470=CARTESIAN_POINT('Ctrl Pts',(-56.1526467348087,-97.7957657838366,
178.936396372111));
#30471=CARTESIAN_POINT('Ctrl Pts',(-55.2832767010304,-97.7941652090492,
178.072094410988));
#30472=CARTESIAN_POINT('Ctrl Pts',(-56.1707931031902,-113.117197303651,
178.813912075476));
#30473=CARTESIAN_POINT('Ctrl Pts',(-54.9958834532485,-113.148169293224,
177.6423391512));
#30474=CARTESIAN_POINT('Ctrl Pts',(-54.9859454592686,-113.05494752122,175.985484901707));
#30475=CARTESIAN_POINT('Ctrl Pts',(-54.9760074652888,-112.961725749215,
174.328630652215));
#30476=CARTESIAN_POINT('Ctrl Pts',(-56.1310410868884,-112.744310219938,
173.157057825983));
#30477=CARTESIAN_POINT('Ctrl Pts',(-57.286074708488,-112.52689469066,171.985484999752));
#30478=CARTESIAN_POINT('Ctrl Pts',(-58.9236553326579,-112.258036427063,
171.985485069079));
#30479=CARTESIAN_POINT('Ctrl Pts',(-60.5612359568277,-111.989178163466,
171.985485138407));
#30480=CARTESIAN_POINT('Ctrl Pts',(-61.7162694809355,-111.771762644582,
173.157058062683));
#30481=CARTESIAN_POINT('Ctrl Pts',(-62.8713030050432,-111.554347125698,
174.328630986959));
#30482=CARTESIAN_POINT('Ctrl Pts',(-62.861364873189,-111.461125368392,175.985485236451));
#30483=CARTESIAN_POINT('Ctrl Pts',(-62.8514267413349,-111.367903611086,
177.642339485944));
#30484=CARTESIAN_POINT('Ctrl Pts',(-61.6765169939012,-111.398875611052,
178.813912312176));
#30485=CARTESIAN_POINT('Ctrl Pts',(-60.5016072464676,-111.429847611019,
179.985485138407));
#30486=CARTESIAN_POINT('Ctrl Pts',(-58.8441504964637,-111.512262345305,
179.985485069079));
#30487=CARTESIAN_POINT('Ctrl Pts',(-57.1866937464598,-111.594677079592,
179.985484999752));
#30488=CARTESIAN_POINT('Ctrl Pts',(-56.011784096518,-111.625649069165,178.813912075476));
#30489=CARTESIAN_POINT('Ctrl Pts',(-54.8368744465762,-111.656621058739,
177.6423391512));
#30490=CARTESIAN_POINT('Ctrl Pts',(-54.8269364525964,-111.563399286734,
175.985484901707));
#30491=CARTESIAN_POINT('Ctrl Pts',(-54.8169984586165,-111.47017751473,174.328630652215));
#30492=CARTESIAN_POINT('Ctrl Pts',(-55.9720320802161,-111.252761985452,
173.157057825983));
#30493=CARTESIAN_POINT('Ctrl Pts',(-57.1270657018158,-111.035346456175,
171.985484999752));
#30494=CARTESIAN_POINT('Ctrl Pts',(-58.7646463259856,-110.766488192578,
171.985485069079));
#30495=CARTESIAN_POINT('Ctrl Pts',(-60.4022269501555,-110.497629928981,
171.985485138407));
#30496=CARTESIAN_POINT('Ctrl Pts',(-61.5572604742632,-110.280214410097,
173.157058062683));
#30497=CARTESIAN_POINT('Ctrl Pts',(-62.712293998371,-110.062798891212,174.328630986959));
#30498=CARTESIAN_POINT('Ctrl Pts',(-62.7023558665168,-109.969577133906,
175.985485236451));
#30499=CARTESIAN_POINT('Ctrl Pts',(-62.6924177346626,-109.8763553766,177.642339485944));
#30500=CARTESIAN_POINT('Ctrl Pts',(-61.517507987229,-109.907327376567,178.813912312176));
#30501=CARTESIAN_POINT('Ctrl Pts',(-60.3425982397954,-109.938299376534,
179.985485138407));
#30502=CARTESIAN_POINT('Ctrl Pts',(-58.6851414897915,-110.02071411082,179.985485069079));
#30503=CARTESIAN_POINT('Ctrl Pts',(-57.0276847397876,-110.103128845106,
179.985484999752));
#30504=CARTESIAN_POINT('Ctrl Pts',(-55.8527750898458,-110.13410083468,178.813912075476));
#30505=CARTESIAN_POINT('Ctrl Pts',(-54.677865439904,-110.165072824253,177.6423391512));
#30506=CARTESIAN_POINT('Ctrl Pts',(-54.6679274459242,-110.071851052249,
175.985484901707));
#30507=CARTESIAN_POINT('Ctrl Pts',(-54.6579894519443,-109.978629280244,
174.328630652215));
#30508=CARTESIAN_POINT('Ctrl Pts',(-55.8130230735439,-109.761213750967,
173.157057825983));
#30509=CARTESIAN_POINT('Ctrl Pts',(-56.9680566951435,-109.543798221689,
171.985484999752));
#30510=CARTESIAN_POINT('Ctrl Pts',(-58.6056373193134,-109.274939958092,
171.985485069079));
#30511=CARTESIAN_POINT('Ctrl Pts',(-60.2432179434833,-109.006081694495,
171.985485138407));
#30512=CARTESIAN_POINT('Ctrl Pts',(-61.398251467591,-108.788666175611,173.157058062683));
#30513=CARTESIAN_POINT('Ctrl Pts',(-62.5532849916988,-108.571250656727,
174.328630986959));
#30514=CARTESIAN_POINT('Ctrl Pts',(-62.5433468598446,-108.478028899421,
175.985485236451));
#30515=CARTESIAN_POINT('Ctrl Pts',(-62.5334087279904,-108.384807142114,
177.642339485944));
#30516=CARTESIAN_POINT('Ctrl Pts',(-61.3584989805568,-108.415779142081,
178.813912312176));
#30517=CARTESIAN_POINT('Ctrl Pts',(-60.1835892331231,-108.446751142048,
179.985485138407));
#30518=CARTESIAN_POINT('Ctrl Pts',(-58.5261324831192,-108.529165876334,
179.985485069079));
#30519=CARTESIAN_POINT('Ctrl Pts',(-56.8686757331153,-108.611580610621,
179.985484999752));
#30520=CARTESIAN_POINT('Ctrl Pts',(-55.6937660831736,-108.642552600194,
178.813912075476));
#30521=CARTESIAN_POINT('Ctrl Pts',(-54.5188564332318,-108.673524589768,
177.6423391512));
#30522=CARTESIAN_POINT('Ctrl Pts',(-54.5089184392519,-108.580302817763,
175.985484901707));
#30523=CARTESIAN_POINT('Ctrl Pts',(-54.4989804452721,-108.487081045759,
174.328630652215));
#30524=CARTESIAN_POINT('Ctrl Pts',(-55.6540140668717,-108.269665516481,
173.157057825983));
#30525=CARTESIAN_POINT('Ctrl Pts',(-56.8090476884713,-108.052249987204,
171.985484999752));
#30526=CARTESIAN_POINT('Ctrl Pts',(-58.4466283126412,-107.783391723607,
171.985485069079));
#30527=CARTESIAN_POINT('Ctrl Pts',(-60.084208936811,-107.51453346001,171.985485138407));
#30528=CARTESIAN_POINT('Ctrl Pts',(-61.2392424609188,-107.297117941125,
173.157058062683));
#30529=CARTESIAN_POINT('Ctrl Pts',(-62.3942759850265,-107.079702422241,
174.328630986959));
#30530=CARTESIAN_POINT('Ctrl Pts',(-62.3843378531723,-106.986480664935,
175.985485236451));
#30531=CARTESIAN_POINT('Ctrl Pts',(-62.3743997213182,-106.893258907629,
177.642339485944));
#30532=CARTESIAN_POINT('Ctrl Pts',(-61.1994899738845,-106.924230907596,
178.813912312176));
#30533=CARTESIAN_POINT('Ctrl Pts',(-60.0245802264509,-106.955202907562,
179.985485138407));
#30534=CARTESIAN_POINT('Ctrl Pts',(-58.367123476447,-107.037617641849,179.985485069079));
#30535=CARTESIAN_POINT('Ctrl Pts',(-56.7096667264431,-107.120032376135,
179.985484999752));
#30536=CARTESIAN_POINT('Ctrl Pts',(-55.5347570765013,-107.151004365708,
178.813912075476));
#30537=CARTESIAN_POINT('Ctrl Pts',(-54.3598474265596,-107.181976355282,
177.6423391512));
#30538=CARTESIAN_POINT('Ctrl Pts',(-54.3499094325797,-107.088754583277,
175.985484901707));
#30539=CARTESIAN_POINT('Ctrl Pts',(-54.3399714385998,-106.995532811273,
174.328630652215));
#30540=CARTESIAN_POINT('Ctrl Pts',(-55.4950050601995,-106.778117281995,
173.157057825983));
#30541=CARTESIAN_POINT('Ctrl Pts',(-56.6500386817991,-106.560701752718,
171.985484999752));
#30542=CARTESIAN_POINT('Ctrl Pts',(-58.2876193059689,-106.291843489121,
171.985485069079));
#30543=CARTESIAN_POINT('Ctrl Pts',(-59.9251999301388,-106.022985225524,
171.985485138407));
#30544=CARTESIAN_POINT('Ctrl Pts',(-61.0802334542465,-105.80556970664,173.157058062683));
#30545=CARTESIAN_POINT('Ctrl Pts',(-62.2352669783543,-105.588154187756,
174.328630986959));
#30546=CARTESIAN_POINT('Ctrl Pts',(-62.2253288465001,-105.494932430449,
175.985485236451));
#30547=CARTESIAN_POINT('Ctrl Pts',(-62.2153907146459,-105.401710673143,
177.642339485944));
#30548=CARTESIAN_POINT('Ctrl Pts',(-61.0404809672123,-105.43268267311,178.813912312176));
#30549=CARTESIAN_POINT('Ctrl Pts',(-59.8655712197787,-105.463654673077,
179.985485138407));
#30550=CARTESIAN_POINT('Ctrl Pts',(-58.2081144697748,-105.546069407363,
179.985485069079));
#30551=CARTESIAN_POINT('Ctrl Pts',(-56.5506577197709,-105.628484141649,
179.985484999752));
#30552=CARTESIAN_POINT('Ctrl Pts',(-55.3757480698291,-105.659456131223,
178.813912075476));
#30553=CARTESIAN_POINT('Ctrl Pts',(-54.2008384198873,-105.690428120796,
177.6423391512));
#30554=CARTESIAN_POINT('Ctrl Pts',(-54.1909004259075,-105.597206348792,
175.985484901707));
#30555=CARTESIAN_POINT('Ctrl Pts',(-54.1809624319276,-105.503984576787,
174.328630652215));
#30556=CARTESIAN_POINT('Ctrl Pts',(-55.3359960535272,-105.28656904751,173.157057825983));
#30557=CARTESIAN_POINT('Ctrl Pts',(-56.4910296751268,-105.069153518232,
171.985484999752));
#30558=CARTESIAN_POINT('Ctrl Pts',(-58.1286102992967,-104.800295254635,
171.985485069079));
#30559=CARTESIAN_POINT('Ctrl Pts',(-59.7661909234666,-104.531436991038,
171.985485138407));
#30560=CARTESIAN_POINT('Ctrl Pts',(-60.9212244475743,-104.314021472154,
173.157058062683));
#30561=CARTESIAN_POINT('Ctrl Pts',(-62.0762579716821,-104.09660595327,174.328630986959));
#30562=CARTESIAN_POINT('Ctrl Pts',(-62.0663198398279,-104.003384195964,
175.985485236451));
#30563=CARTESIAN_POINT('Ctrl Pts',(-62.0563817079737,-103.910162438658,
177.642339485944));
#30564=CARTESIAN_POINT('Ctrl Pts',(-60.8814719605401,-103.941134438624,
178.813912312176));
#30565=CARTESIAN_POINT('Ctrl Pts',(-59.7065622131064,-103.972106438591,
179.985485138407));
#30566=CARTESIAN_POINT('Ctrl Pts',(-58.0491054631025,-104.054521172878,
179.985485069079));
#30567=CARTESIAN_POINT('Ctrl Pts',(-56.3916487130987,-104.136935907164,
179.985484999752));
#30568=CARTESIAN_POINT('Ctrl Pts',(-55.2167390631569,-104.167907896737,
178.813912075476));
#30569=CARTESIAN_POINT('Ctrl Pts',(-54.0418294132151,-104.198879886311,
177.6423391512));
#30570=CARTESIAN_POINT('Ctrl Pts',(-54.0318914192353,-104.105658114306,
175.985484901707));
#30571=CARTESIAN_POINT('Ctrl Pts',(-54.0219534252554,-104.012436342302,
174.328630652215));
#30572=CARTESIAN_POINT('Ctrl Pts',(-55.176987046855,-103.795020813024,173.157057825983));
#30573=CARTESIAN_POINT('Ctrl Pts',(-56.3320206684546,-103.577605283747,
171.985484999752));
#30574=CARTESIAN_POINT('Ctrl Pts',(-57.9696012926245,-103.30874702015,171.985485069079));
#30575=CARTESIAN_POINT('Ctrl Pts',(-59.6071819167943,-103.039888756553,
171.985485138407));
#30576=CARTESIAN_POINT('Ctrl Pts',(-60.7622154409021,-102.822473237669,
173.157058062683));
#30577=CARTESIAN_POINT('Ctrl Pts',(-61.9172489650099,-102.605057718784,
174.328630986959));
#30578=CARTESIAN_POINT('Ctrl Pts',(-61.9073108331557,-102.511835961478,
175.985485236451));
#30579=CARTESIAN_POINT('Ctrl Pts',(-61.8973727013015,-102.418614204172,
177.642339485944));
#30580=CARTESIAN_POINT('Ctrl Pts',(-60.7224629538678,-102.449586204139,
178.813912312176));
#30581=CARTESIAN_POINT('Ctrl Pts',(-59.5475532064342,-102.480558204106,
179.985485138407));
#30582=CARTESIAN_POINT('Ctrl Pts',(-57.8900964564303,-102.562972938392,
179.985485069079));
#30583=CARTESIAN_POINT('Ctrl Pts',(-56.2326397064264,-102.645387672678,
179.985484999752));
#30584=CARTESIAN_POINT('Ctrl Pts',(-55.0577300564847,-102.676359662252,
178.813912075476));
#30585=CARTESIAN_POINT('Ctrl Pts',(-53.8828204065429,-102.707331651825,
177.6423391512));
#30586=CARTESIAN_POINT('Ctrl Pts',(-53.872882412563,-102.614109879821,175.985484901707));
#30587=CARTESIAN_POINT('Ctrl Pts',(-53.8629444185832,-102.520888107816,
174.328630652215));
#30588=CARTESIAN_POINT('Ctrl Pts',(-55.0179780401828,-102.303472578539,
173.157057825983));
#30589=CARTESIAN_POINT('Ctrl Pts',(-56.1730116617824,-102.086057049261,
171.985484999752));
#30590=CARTESIAN_POINT('Ctrl Pts',(-57.8105922859523,-101.817198785664,
171.985485069079));
#30591=CARTESIAN_POINT('Ctrl Pts',(-59.4481729101221,-101.548340522067,
171.985485138407));
#30592=CARTESIAN_POINT('Ctrl Pts',(-60.6032064342299,-101.330925003183,
173.157058062683));
#30593=CARTESIAN_POINT('Ctrl Pts',(-61.7582399583376,-101.113509484299,
174.328630986959));
#30594=CARTESIAN_POINT('Ctrl Pts',(-61.7483018264834,-101.020287726993,
175.985485236451));
#30595=CARTESIAN_POINT('Ctrl Pts',(-61.7383636946293,-100.927065969686,
177.642339485944));
#30596=CARTESIAN_POINT('Ctrl Pts',(-60.5634539471956,-100.958037969653,
178.813912312176));
#30597=CARTESIAN_POINT('Ctrl Pts',(-59.388544199762,-100.98900996962,179.985485138407));
#30598=CARTESIAN_POINT('Ctrl Pts',(-57.7310874497581,-101.071424703906,
179.985485069079));
#30599=CARTESIAN_POINT('Ctrl Pts',(-56.0736306997542,-101.153839438193,
179.985484999752));
#30600=CARTESIAN_POINT('Ctrl Pts',(-54.8987210498124,-101.184811427766,
178.813912075476));
#30601=CARTESIAN_POINT('Ctrl Pts',(-53.7238113998707,-101.21578341734,177.6423391512));
#30602=CARTESIAN_POINT('Ctrl Pts',(-53.7138734058908,-101.122561645335,
175.985484901707));
#30603=CARTESIAN_POINT('Ctrl Pts',(-53.7039354119109,-101.029339873331,
174.328630652215));
#30604=CARTESIAN_POINT('Ctrl Pts',(-54.8589690335105,-100.811924344053,
173.157057825983));
#30605=CARTESIAN_POINT('Ctrl Pts',(-56.0140026551102,-100.594508814776,
171.985484999752));
#30606=CARTESIAN_POINT('Ctrl Pts',(-57.65158327928,-100.325650551179,171.985485069079));
#30607=CARTESIAN_POINT('Ctrl Pts',(-59.2891639034499,-100.056792287582,
171.985485138407));
#30608=CARTESIAN_POINT('Ctrl Pts',(-60.4441974275576,-99.8393767686974,
173.157058062683));
#30609=CARTESIAN_POINT('Ctrl Pts',(-61.5992309516654,-99.6219612498133,
174.328630986959));
#30610=CARTESIAN_POINT('Ctrl Pts',(-61.5892928198112,-99.528739492507,175.985485236451));
#30611=CARTESIAN_POINT('Ctrl Pts',(-61.579354687957,-99.4355177352008,177.642339485944));
#30612=CARTESIAN_POINT('Ctrl Pts',(-60.4044449405234,-99.4664897351676,
178.813912312176));
#30613=CARTESIAN_POINT('Ctrl Pts',(-59.2295351930898,-99.4974617351344,
179.985485138407));
#30614=CARTESIAN_POINT('Ctrl Pts',(-57.5720784430859,-99.5798764694207,
179.985485069079));
#30615=CARTESIAN_POINT('Ctrl Pts',(-55.914621693082,-99.662291203707,179.985484999752));
#30616=CARTESIAN_POINT('Ctrl Pts',(-54.7397120431402,-99.6932631932805,
178.813912075476));
#30617=CARTESIAN_POINT('Ctrl Pts',(-53.5648023931984,-99.724235182854,177.6423391512));
#30618=CARTESIAN_POINT('Ctrl Pts',(-53.5548643992186,-99.6310134108495,
175.985484901707));
#30619=CARTESIAN_POINT('Ctrl Pts',(-53.5449264052387,-99.5377916388449,
174.328630652215));
#30620=CARTESIAN_POINT('Ctrl Pts',(-54.6999600268383,-99.3203761095675,
173.157057825983));
#30621=CARTESIAN_POINT('Ctrl Pts',(-55.8549936484379,-99.10296058029,171.985484999752));
#30622=CARTESIAN_POINT('Ctrl Pts',(-57.4925742726078,-98.834102316693,171.985485069079));
#30623=CARTESIAN_POINT('Ctrl Pts',(-59.1301548967777,-98.565244053096,171.985485138407));
#30624=CARTESIAN_POINT('Ctrl Pts',(-60.2851884208854,-98.3478285342118,
173.157058062683));
#30625=CARTESIAN_POINT('Ctrl Pts',(-61.4402219449932,-98.1304130153276,
174.328630986959));
#30626=CARTESIAN_POINT('Ctrl Pts',(-61.430283813139,-98.0371912580215,175.985485236451));
#30627=CARTESIAN_POINT('Ctrl Pts',(-61.4203456812848,-97.9439695007152,
177.642339485944));
#30628=CARTESIAN_POINT('Ctrl Pts',(-60.2454359338512,-97.974941500682,178.813912312176));
#30629=CARTESIAN_POINT('Ctrl Pts',(-59.0705261864175,-98.0059135006488,
179.985485138407));
#30630=CARTESIAN_POINT('Ctrl Pts',(-57.4130694364136,-98.0883282349351,
179.985485069079));
#30631=CARTESIAN_POINT('Ctrl Pts',(-55.7556126864097,-98.1707429692214,
179.985484999752));
#30632=CARTESIAN_POINT('Ctrl Pts',(-54.580703036468,-98.2017149587949,178.813912075476));
#30633=CARTESIAN_POINT('Ctrl Pts',(-61.176587584573,-103.935293252465,178.485485069079));
#30634=CARTESIAN_POINT('Ctrl Pts',(-61.0380153802162,-103.937007770342,
178.657813499464));
#30635=CARTESIAN_POINT('Ctrl Pts',(-60.8814719605401,-103.941134438624,
178.813912312176));
#30636=CARTESIAN_POINT('Ctrl Pts',(-59.7065622131064,-103.972106438591,
179.985485138407));
#30637=CARTESIAN_POINT('Ctrl Pts',(-58.0491054631025,-104.054521172878,
179.985485069079));
#30638=CARTESIAN_POINT('Ctrl Pts',(-56.3916487130987,-104.136935907164,
179.985484999752));
#30639=CARTESIAN_POINT('Ctrl Pts',(-55.2167390631569,-104.167907896737,
178.813912075476));
#30640=CARTESIAN_POINT('Ctrl Pts',(-54.0418294132151,-104.198879886311,
177.6423391512));
#30641=CARTESIAN_POINT('Ctrl Pts',(-54.0318914192353,-104.105658114306,
175.985484901707));
#30642=CARTESIAN_POINT('Ctrl Pts',(-54.0219534252554,-104.012436342302,
174.328630652215));
#30643=CARTESIAN_POINT('Ctrl Pts',(-55.176987046855,-103.795020813024,173.157057825983));
#30644=CARTESIAN_POINT('Ctrl Pts',(-56.3320206684546,-103.577605283747,
171.985484999752));
#30645=CARTESIAN_POINT('Ctrl Pts',(-57.9696012926245,-103.30874702015,171.985485069079));
#30646=CARTESIAN_POINT('Ctrl Pts',(-59.6071819167943,-103.039888756553,
171.985485138407));
#30647=CARTESIAN_POINT('Ctrl Pts',(-60.7622154409021,-102.822473237669,
173.157058062683));
#30648=CARTESIAN_POINT('Ctrl Pts',(-60.9161104618553,-102.793505103726,
173.313156769748));
#30649=CARTESIAN_POINT('Ctrl Pts',(-61.0519296658261,-102.765967674544,
173.485485069079));
#30650=CARTESIAN_POINT('Ctrl Pts',(-56.1707931031902,-113.117197303651,
178.813912075476));
#30651=CARTESIAN_POINT('Ctrl Pts',(-54.9958834532485,-113.148169293224,
177.6423391512));
#30652=CARTESIAN_POINT('Ctrl Pts',(-54.9859454592686,-113.05494752122,175.985484901707));
#30653=CARTESIAN_POINT('Ctrl Pts',(-54.9760074652888,-112.961725749215,
174.328630652215));
#30654=CARTESIAN_POINT('Ctrl Pts',(-56.1310410868884,-112.744310219938,
173.157057825983));
#30655=CARTESIAN_POINT('Ctrl Pts',(-57.286074708488,-112.52689469066,171.985484999752));
#30656=CARTESIAN_POINT('Ctrl Pts',(-58.9236553326578,-112.258036427063,
171.985485069079));
#30657=CARTESIAN_POINT('Ctrl Pts',(-60.5612359568277,-111.989178163466,
171.985485138407));
#30658=CARTESIAN_POINT('Ctrl Pts',(-61.7162694809355,-111.771762644582,
173.157058062683));
#30659=CARTESIAN_POINT('Ctrl Pts',(-62.8713030050432,-111.554347125698,
174.328630986959));
#30660=CARTESIAN_POINT('Ctrl Pts',(-62.861364873189,-111.461125368392,175.985485236451));
#30661=CARTESIAN_POINT('Ctrl Pts',(-62.8514267413349,-111.367903611086,
177.642339485944));
#30662=CARTESIAN_POINT('Ctrl Pts',(-61.6765169939012,-111.398875611052,
178.813912312176));
#30663=CARTESIAN_POINT('Ctrl Pts',(-60.5016072464676,-111.429847611019,
179.985485138407));
#30664=CARTESIAN_POINT('Ctrl Pts',(-58.8441504964637,-111.512262345305,
179.985485069079));
#30665=CARTESIAN_POINT('Ctrl Pts',(-57.1866937464598,-111.594677079592,
179.985484999752));
#30666=CARTESIAN_POINT('Ctrl Pts',(-56.011784096518,-111.625649069165,178.813912075476));
#30667=CARTESIAN_POINT('Ctrl Pts',(-54.8368744465763,-111.656621058739,
177.6423391512));
#30668=CARTESIAN_POINT('Ctrl Pts',(-54.8269364525964,-111.563399286734,
175.985484901707));
#30669=CARTESIAN_POINT('Ctrl Pts',(-54.8169984586165,-111.47017751473,174.328630652215));
#30670=CARTESIAN_POINT('Ctrl Pts',(-55.9720320802161,-111.252761985452,
173.157057825983));
#30671=CARTESIAN_POINT('Ctrl Pts',(-57.1270657018158,-111.035346456175,
171.985484999752));
#30672=CARTESIAN_POINT('Ctrl Pts',(-58.7646463259856,-110.766488192578,
171.985485069079));
#30673=CARTESIAN_POINT('Ctrl Pts',(-60.4022269501555,-110.497629928981,
171.985485138407));
#30674=CARTESIAN_POINT('Ctrl Pts',(-61.5572604742632,-110.280214410097,
173.157058062683));
#30675=CARTESIAN_POINT('Ctrl Pts',(-62.712293998371,-110.062798891212,174.328630986959));
#30676=CARTESIAN_POINT('Ctrl Pts',(-62.7023558665168,-109.969577133906,
175.985485236451));
#30677=CARTESIAN_POINT('Ctrl Pts',(-62.6924177346626,-109.8763553766,177.642339485944));
#30678=CARTESIAN_POINT('Ctrl Pts',(-61.517507987229,-109.907327376567,178.813912312176));
#30679=CARTESIAN_POINT('Ctrl Pts',(-60.3425982397954,-109.938299376534,
179.985485138407));
#30680=CARTESIAN_POINT('Ctrl Pts',(-58.6851414897915,-110.02071411082,179.985485069079));
#30681=CARTESIAN_POINT('Ctrl Pts',(-57.0276847397876,-110.103128845106,
179.985484999752));
#30682=CARTESIAN_POINT('Ctrl Pts',(-55.8527750898458,-110.13410083468,178.813912075476));
#30683=CARTESIAN_POINT('Ctrl Pts',(-54.677865439904,-110.165072824253,177.6423391512));
#30684=CARTESIAN_POINT('Ctrl Pts',(-54.6679274459242,-110.071851052249,
175.985484901707));
#30685=CARTESIAN_POINT('Ctrl Pts',(-54.6579894519443,-109.978629280244,
174.328630652215));
#30686=CARTESIAN_POINT('Ctrl Pts',(-55.8130230735439,-109.761213750967,
173.157057825983));
#30687=CARTESIAN_POINT('Ctrl Pts',(-56.9680566951435,-109.543798221689,
171.985484999752));
#30688=CARTESIAN_POINT('Ctrl Pts',(-58.6056373193134,-109.274939958092,
171.985485069079));
#30689=CARTESIAN_POINT('Ctrl Pts',(-60.2432179434833,-109.006081694495,
171.985485138407));
#30690=CARTESIAN_POINT('Ctrl Pts',(-61.398251467591,-108.788666175611,173.157058062683));
#30691=CARTESIAN_POINT('Ctrl Pts',(-62.5532849916988,-108.571250656727,
174.328630986959));
#30692=CARTESIAN_POINT('Ctrl Pts',(-62.5433468598446,-108.478028899421,
175.985485236451));
#30693=CARTESIAN_POINT('Ctrl Pts',(-62.5334087279904,-108.384807142114,
177.642339485944));
#30694=CARTESIAN_POINT('Ctrl Pts',(-61.3584989805568,-108.415779142081,
178.813912312176));
#30695=CARTESIAN_POINT('Ctrl Pts',(-60.1835892331231,-108.446751142048,
179.985485138407));
#30696=CARTESIAN_POINT('Ctrl Pts',(-58.5261324831192,-108.529165876334,
179.985485069079));
#30697=CARTESIAN_POINT('Ctrl Pts',(-56.8686757331153,-108.611580610621,
179.985484999752));
#30698=CARTESIAN_POINT('Ctrl Pts',(-55.6937660831736,-108.642552600194,
178.813912075476));
#30699=CARTESIAN_POINT('Ctrl Pts',(-54.5188564332318,-108.673524589768,
177.6423391512));
#30700=CARTESIAN_POINT('Ctrl Pts',(-54.5089184392519,-108.580302817763,
175.985484901707));
#30701=CARTESIAN_POINT('Ctrl Pts',(-54.4989804452721,-108.487081045759,
174.328630652215));
#30702=CARTESIAN_POINT('Ctrl Pts',(-55.6540140668717,-108.269665516481,
173.157057825983));
#30703=CARTESIAN_POINT('Ctrl Pts',(-56.8090476884713,-108.052249987204,
171.985484999752));
#30704=CARTESIAN_POINT('Ctrl Pts',(-58.4466283126412,-107.783391723607,
171.985485069079));
#30705=CARTESIAN_POINT('Ctrl Pts',(-60.084208936811,-107.51453346001,171.985485138407));
#30706=CARTESIAN_POINT('Ctrl Pts',(-61.2392424609188,-107.297117941125,
173.157058062683));
#30707=CARTESIAN_POINT('Ctrl Pts',(-62.3942759850265,-107.079702422241,
174.328630986959));
#30708=CARTESIAN_POINT('Ctrl Pts',(-62.3843378531723,-106.986480664935,
175.985485236451));
#30709=CARTESIAN_POINT('Ctrl Pts',(-62.3743997213182,-106.893258907629,
177.642339485944));
#30710=CARTESIAN_POINT('Ctrl Pts',(-61.1994899738845,-106.924230907596,
178.813912312176));
#30711=CARTESIAN_POINT('Ctrl Pts',(-60.0245802264509,-106.955202907562,
179.985485138407));
#30712=CARTESIAN_POINT('Ctrl Pts',(-58.367123476447,-107.037617641849,179.985485069079));
#30713=CARTESIAN_POINT('Ctrl Pts',(-56.7096667264431,-107.120032376135,
179.985484999752));
#30714=CARTESIAN_POINT('Ctrl Pts',(-55.5347570765013,-107.151004365708,
178.813912075476));
#30715=CARTESIAN_POINT('Ctrl Pts',(-54.3598474265596,-107.181976355282,
177.6423391512));
#30716=CARTESIAN_POINT('Ctrl Pts',(-54.3499094325797,-107.088754583277,
175.985484901707));
#30717=CARTESIAN_POINT('Ctrl Pts',(-54.3399714385998,-106.995532811273,
174.328630652215));
#30718=CARTESIAN_POINT('Ctrl Pts',(-55.4950050601995,-106.778117281995,
173.157057825983));
#30719=CARTESIAN_POINT('Ctrl Pts',(-56.6500386817991,-106.560701752718,
171.985484999752));
#30720=CARTESIAN_POINT('Ctrl Pts',(-58.2876193059689,-106.291843489121,
171.985485069079));
#30721=CARTESIAN_POINT('Ctrl Pts',(-59.9251999301388,-106.022985225524,
171.985485138407));
#30722=CARTESIAN_POINT('Ctrl Pts',(-61.0802334542465,-105.80556970664,173.157058062683));
#30723=CARTESIAN_POINT('Ctrl Pts',(-62.2352669783543,-105.588154187756,
174.328630986959));
#30724=CARTESIAN_POINT('Ctrl Pts',(-62.2253288465001,-105.494932430449,
175.985485236451));
#30725=CARTESIAN_POINT('Ctrl Pts',(-62.2153907146459,-105.401710673143,
177.642339485944));
#30726=CARTESIAN_POINT('Ctrl Pts',(-61.0404809672123,-105.43268267311,178.813912312176));
#30727=CARTESIAN_POINT('Ctrl Pts',(-59.8655712197787,-105.463654673077,
179.985485138407));
#30728=CARTESIAN_POINT('Ctrl Pts',(-58.2081144697748,-105.546069407363,
179.985485069079));
#30729=CARTESIAN_POINT('Ctrl Pts',(-56.5506577197709,-105.628484141649,
179.985484999752));
#30730=CARTESIAN_POINT('Ctrl Pts',(-55.3757480698291,-105.659456131223,
178.813912075476));
#30731=CARTESIAN_POINT('Ctrl Pts',(-54.2008384198873,-105.690428120796,
177.6423391512));
#30732=CARTESIAN_POINT('Ctrl Pts',(-54.1909004259075,-105.597206348792,
175.985484901707));
#30733=CARTESIAN_POINT('Ctrl Pts',(-54.1809624319276,-105.503984576787,
174.328630652215));
#30734=CARTESIAN_POINT('Ctrl Pts',(-55.3359960535272,-105.28656904751,173.157057825983));
#30735=CARTESIAN_POINT('Ctrl Pts',(-56.4910296751268,-105.069153518232,
171.985484999752));
#30736=CARTESIAN_POINT('Ctrl Pts',(-58.1286102992967,-104.800295254635,
171.985485069079));
#30737=CARTESIAN_POINT('Ctrl Pts',(-59.7661909234666,-104.531436991038,
171.985485138407));
#30738=CARTESIAN_POINT('Ctrl Pts',(-60.9212244475743,-104.314021472154,
173.157058062683));
#30739=CARTESIAN_POINT('Ctrl Pts',(-62.0762579716821,-104.09660595327,174.328630986959));
#30740=CARTESIAN_POINT('Ctrl Pts',(-62.0663198398279,-104.003384195964,
175.985485236451));
#30741=CARTESIAN_POINT('Ctrl Pts',(-62.0563817079737,-103.910162438658,
177.642339485944));
#30742=CARTESIAN_POINT('Ctrl Pts',(-60.8814719605401,-103.941134438624,
178.813912312176));
#30743=CARTESIAN_POINT('Ctrl Pts',(-59.7065622131064,-103.972106438591,
179.985485138407));
#30744=CARTESIAN_POINT('Ctrl Pts',(-58.0491054631025,-104.054521172878,
179.985485069079));
#30745=CARTESIAN_POINT('Ctrl Pts',(-56.3916487130987,-104.136935907164,
179.985484999752));
#30746=CARTESIAN_POINT('Ctrl Pts',(-55.2167390631569,-104.167907896737,
178.813912075476));
#30747=CARTESIAN_POINT('Ctrl Pts',(-54.0418294132151,-104.198879886311,
177.6423391512));
#30748=CARTESIAN_POINT('Ctrl Pts',(-54.0318914192353,-104.105658114306,
175.985484901707));
#30749=CARTESIAN_POINT('Ctrl Pts',(-54.0219534252554,-104.012436342302,
174.328630652215));
#30750=CARTESIAN_POINT('Ctrl Pts',(-55.176987046855,-103.795020813024,173.157057825983));
#30751=CARTESIAN_POINT('Ctrl Pts',(-56.3320206684546,-103.577605283747,
171.985484999752));
#30752=CARTESIAN_POINT('Ctrl Pts',(-57.9696012926245,-103.30874702015,171.985485069079));
#30753=CARTESIAN_POINT('Ctrl Pts',(-59.6071819167943,-103.039888756553,
171.985485138407));
#30754=CARTESIAN_POINT('Ctrl Pts',(-60.7622154409021,-102.822473237669,
173.157058062683));
#30755=CARTESIAN_POINT('Ctrl Pts',(-61.9172489650099,-102.605057718784,
174.328630986959));
#30756=CARTESIAN_POINT('Ctrl Pts',(-61.9073108331557,-102.511835961478,
175.985485236451));
#30757=CARTESIAN_POINT('Ctrl Pts',(-61.8973727013015,-102.418614204172,
177.642339485944));
#30758=CARTESIAN_POINT('Ctrl Pts',(-60.7224629538678,-102.449586204139,
178.813912312176));
#30759=CARTESIAN_POINT('Ctrl Pts',(-59.5475532064342,-102.480558204106,
179.985485138407));
#30760=CARTESIAN_POINT('Ctrl Pts',(-57.8900964564303,-102.562972938392,
179.985485069079));
#30761=CARTESIAN_POINT('Ctrl Pts',(-56.2326397064264,-102.645387672678,
179.985484999752));
#30762=CARTESIAN_POINT('Ctrl Pts',(-55.0577300564847,-102.676359662252,
178.813912075476));
#30763=CARTESIAN_POINT('Ctrl Pts',(-53.8828204065429,-102.707331651825,
177.6423391512));
#30764=CARTESIAN_POINT('Ctrl Pts',(-53.872882412563,-102.614109879821,175.985484901707));
#30765=CARTESIAN_POINT('Ctrl Pts',(-53.8629444185832,-102.520888107816,
174.328630652215));
#30766=CARTESIAN_POINT('Ctrl Pts',(-55.0179780401828,-102.303472578539,
173.157057825983));
#30767=CARTESIAN_POINT('Ctrl Pts',(-56.1730116617824,-102.086057049261,
171.985484999752));
#30768=CARTESIAN_POINT('Ctrl Pts',(-57.8105922859523,-101.817198785664,
171.985485069079));
#30769=CARTESIAN_POINT('Ctrl Pts',(-59.4481729101221,-101.548340522067,
171.985485138407));
#30770=CARTESIAN_POINT('Ctrl Pts',(-60.6032064342299,-101.330925003183,
173.157058062683));
#30771=CARTESIAN_POINT('Ctrl Pts',(-61.7582399583376,-101.113509484299,
174.328630986959));
#30772=CARTESIAN_POINT('Ctrl Pts',(-61.7483018264834,-101.020287726993,
175.985485236451));
#30773=CARTESIAN_POINT('Ctrl Pts',(-61.7383636946293,-100.927065969686,
177.642339485944));
#30774=CARTESIAN_POINT('Ctrl Pts',(-60.5634539471956,-100.958037969653,
178.813912312176));
#30775=CARTESIAN_POINT('Ctrl Pts',(-59.388544199762,-100.98900996962,179.985485138407));
#30776=CARTESIAN_POINT('Ctrl Pts',(-57.7310874497581,-101.071424703906,
179.985485069079));
#30777=CARTESIAN_POINT('Ctrl Pts',(-56.0736306997542,-101.153839438193,
179.985484999752));
#30778=CARTESIAN_POINT('Ctrl Pts',(-54.8987210498124,-101.184811427766,
178.813912075476));
#30779=CARTESIAN_POINT('Ctrl Pts',(-53.7238113998707,-101.21578341734,177.6423391512));
#30780=CARTESIAN_POINT('Ctrl Pts',(-53.7138734058908,-101.122561645335,
175.985484901707));
#30781=CARTESIAN_POINT('Ctrl Pts',(-53.7039354119109,-101.029339873331,
174.328630652215));
#30782=CARTESIAN_POINT('Ctrl Pts',(-54.8589690335105,-100.811924344053,
173.157057825983));
#30783=CARTESIAN_POINT('Ctrl Pts',(-56.0140026551102,-100.594508814776,
171.985484999752));
#30784=CARTESIAN_POINT('Ctrl Pts',(-57.65158327928,-100.325650551179,171.985485069079));
#30785=CARTESIAN_POINT('Ctrl Pts',(-59.2891639034499,-100.056792287582,
171.985485138407));
#30786=CARTESIAN_POINT('Ctrl Pts',(-60.4441974275576,-99.8393767686974,
173.157058062683));
#30787=CARTESIAN_POINT('Ctrl Pts',(-61.5992309516654,-99.6219612498133,
174.328630986959));
#30788=CARTESIAN_POINT('Ctrl Pts',(-61.5892928198112,-99.528739492507,175.985485236451));
#30789=CARTESIAN_POINT('Ctrl Pts',(-61.579354687957,-99.4355177352008,177.642339485944));
#30790=CARTESIAN_POINT('Ctrl Pts',(-60.4044449405234,-99.4664897351676,
178.813912312176));
#30791=CARTESIAN_POINT('Ctrl Pts',(-59.2295351930898,-99.4974617351344,
179.985485138407));
#30792=CARTESIAN_POINT('Ctrl Pts',(-57.5720784430859,-99.5798764694207,
179.985485069079));
#30793=CARTESIAN_POINT('Ctrl Pts',(-55.914621693082,-99.662291203707,179.985484999752));
#30794=CARTESIAN_POINT('Ctrl Pts',(-54.7397120431402,-99.6932631932805,
178.813912075476));
#30795=CARTESIAN_POINT('Ctrl Pts',(-53.5648023931984,-99.724235182854,177.6423391512));
#30796=CARTESIAN_POINT('Ctrl Pts',(-53.5548643992186,-99.6310134108495,
175.985484901707));
#30797=CARTESIAN_POINT('Ctrl Pts',(-53.5449264052387,-99.5377916388449,
174.328630652215));
#30798=CARTESIAN_POINT('Ctrl Pts',(-54.6999600268383,-99.3203761095675,
173.157057825983));
#30799=CARTESIAN_POINT('Ctrl Pts',(-55.8549936484379,-99.10296058029,171.985484999752));
#30800=CARTESIAN_POINT('Ctrl Pts',(-57.4925742726078,-98.834102316693,171.985485069079));
#30801=CARTESIAN_POINT('Ctrl Pts',(-59.1301548967777,-98.5652440530961,
171.985485138407));
#30802=CARTESIAN_POINT('Ctrl Pts',(-60.2851884208854,-98.3478285342118,
173.157058062683));
#30803=CARTESIAN_POINT('Ctrl Pts',(-61.4402219449932,-98.1304130153276,
174.328630986959));
#30804=CARTESIAN_POINT('Ctrl Pts',(-61.430283813139,-98.0371912580215,175.985485236451));
#30805=CARTESIAN_POINT('Ctrl Pts',(-61.4203456812848,-97.9439695007152,
177.642339485944));
#30806=CARTESIAN_POINT('Ctrl Pts',(-60.2454359338512,-97.974941500682,178.813912312176));
#30807=CARTESIAN_POINT('Ctrl Pts',(-59.0705261864175,-98.0059135006488,
179.985485138407));
#30808=CARTESIAN_POINT('Ctrl Pts',(-57.4130694364136,-98.0883282349351,
179.985485069079));
#30809=CARTESIAN_POINT('Ctrl Pts',(-55.7556126864097,-98.1707429692214,
179.985484999752));
#30810=CARTESIAN_POINT('Ctrl Pts',(-54.580703036468,-98.2017149587949,178.813912075476));
#30811=CARTESIAN_POINT('Ctrl Pts',(-56.181115489574,-113.283598570176,178.821287383467));
#30812=CARTESIAN_POINT('Ctrl Pts',(-55.0031681001975,-113.314894403068,
177.646659506339));
#30813=CARTESIAN_POINT('Ctrl Pts',(-54.9932301063974,-113.221672631044,
175.985484901271));
#30814=CARTESIAN_POINT('Ctrl Pts',(-54.9832921125973,-113.12845085902,174.324310296203));
#30815=CARTESIAN_POINT('Ctrl Pts',(-56.1413634738858,-112.910711486397,
173.149682517375));
#30816=CARTESIAN_POINT('Ctrl Pts',(-57.2994348351743,-112.692972113774,
171.975054738546));
#30817=CARTESIAN_POINT('Ctrl Pts',(-58.9413114718314,-112.423655866545,
171.975054808055));
#30818=CARTESIAN_POINT('Ctrl Pts',(-60.5831881084886,-112.154339619316,
171.975054877564));
#30819=CARTESIAN_POINT('Ctrl Pts',(-61.741259372031,-111.936600257113,173.149682754692));
#30820=CARTESIAN_POINT('Ctrl Pts',(-62.8993306355734,-111.71886089491,174.32431063182));
#30821=CARTESIAN_POINT('Ctrl Pts',(-62.8893925035395,-111.625639137623,
175.985485236888));
#30822=CARTESIAN_POINT('Ctrl Pts',(-62.8794543715055,-111.532417380336,
177.646659841956));
#30823=CARTESIAN_POINT('Ctrl Pts',(-61.701506884383,-111.563713223648,178.821287620784));
#30824=CARTESIAN_POINT('Ctrl Pts',(-60.5235593972605,-111.595009066961,
179.995915399612));
#30825=CARTESIAN_POINT('Ctrl Pts',(-58.8618066347693,-111.677881784879,
179.995915330104));
#30826=CARTESIAN_POINT('Ctrl Pts',(-57.2000538722782,-111.760754502798,
179.995915260595));
#30827=CARTESIAN_POINT('Ctrl Pts',(-56.0221064829017,-111.79205033569,178.821287383467));
#30828=CARTESIAN_POINT('Ctrl Pts',(-54.8441590935253,-111.823346168582,
177.646659506339));
#30829=CARTESIAN_POINT('Ctrl Pts',(-54.8342210997252,-111.730124396559,
175.985484901271));
#30830=CARTESIAN_POINT('Ctrl Pts',(-54.8242831059251,-111.636902624535,
174.324310296203));
#30831=CARTESIAN_POINT('Ctrl Pts',(-55.9823544672136,-111.419163251912,
173.149682517375));
#30832=CARTESIAN_POINT('Ctrl Pts',(-57.1404258285021,-111.201423879289,
171.975054738546));
#30833=CARTESIAN_POINT('Ctrl Pts',(-58.7823024651592,-110.932107632059,
171.975054808055));
#30834=CARTESIAN_POINT('Ctrl Pts',(-60.4241791018163,-110.66279138483,171.975054877564));
#30835=CARTESIAN_POINT('Ctrl Pts',(-61.5822503653587,-110.445052022627,
173.149682754692));
#30836=CARTESIAN_POINT('Ctrl Pts',(-62.7403216289012,-110.227312660424,
174.32431063182));
#30837=CARTESIAN_POINT('Ctrl Pts',(-62.7303834968672,-110.134090903137,
175.985485236888));
#30838=CARTESIAN_POINT('Ctrl Pts',(-62.7204453648333,-110.04086914585,177.646659841956));
#30839=CARTESIAN_POINT('Ctrl Pts',(-61.5424978777108,-110.072164989163,
178.821287620784));
#30840=CARTESIAN_POINT('Ctrl Pts',(-60.3645503905882,-110.103460832475,
179.995915399612));
#30841=CARTESIAN_POINT('Ctrl Pts',(-58.7027976280971,-110.186333550394,
179.995915330104));
#30842=CARTESIAN_POINT('Ctrl Pts',(-57.041044865606,-110.269206268313,179.995915260595));
#30843=CARTESIAN_POINT('Ctrl Pts',(-55.8630974762295,-110.300502101205,
178.821287383467));
#30844=CARTESIAN_POINT('Ctrl Pts',(-54.6851500868531,-110.331797934097,
177.646659506339));
#30845=CARTESIAN_POINT('Ctrl Pts',(-54.675212093053,-110.238576162073,175.985484901271));
#30846=CARTESIAN_POINT('Ctrl Pts',(-54.6652740992529,-110.145354390049,
174.324310296203));
#30847=CARTESIAN_POINT('Ctrl Pts',(-55.8233454605414,-109.927615017426,
173.149682517375));
#30848=CARTESIAN_POINT('Ctrl Pts',(-56.9814168218299,-109.709875644803,
171.975054738546));
#30849=CARTESIAN_POINT('Ctrl Pts',(-58.623293458487,-109.440559397574,171.975054808055));
#30850=CARTESIAN_POINT('Ctrl Pts',(-60.2651700951441,-109.171243150344,
171.975054877564));
#30851=CARTESIAN_POINT('Ctrl Pts',(-61.4232413586865,-108.953503788142,
173.149682754692));
#30852=CARTESIAN_POINT('Ctrl Pts',(-62.581312622229,-108.735764425939,174.32431063182));
#30853=CARTESIAN_POINT('Ctrl Pts',(-62.571374490195,-108.642542668652,175.985485236888));
#30854=CARTESIAN_POINT('Ctrl Pts',(-62.5614363581611,-108.549320911365,
177.646659841956));
#30855=CARTESIAN_POINT('Ctrl Pts',(-61.3834888710385,-108.580616754677,
178.821287620784));
#30856=CARTESIAN_POINT('Ctrl Pts',(-60.205541383916,-108.61191259799,179.995915399612));
#30857=CARTESIAN_POINT('Ctrl Pts',(-58.5437886214249,-108.694785315908,
179.995915330104));
#30858=CARTESIAN_POINT('Ctrl Pts',(-56.8820358589338,-108.777658033827,
179.995915260595));
#30859=CARTESIAN_POINT('Ctrl Pts',(-55.7040884695573,-108.808953866719,
178.821287383467));
#30860=CARTESIAN_POINT('Ctrl Pts',(-54.5261410801808,-108.840249699611,
177.646659506339));
#30861=CARTESIAN_POINT('Ctrl Pts',(-54.5162030863807,-108.747027927587,
175.985484901271));
#30862=CARTESIAN_POINT('Ctrl Pts',(-54.5062650925806,-108.653806155564,
174.324310296203));
#30863=CARTESIAN_POINT('Ctrl Pts',(-55.6643364538691,-108.436066782941,
173.149682517375));
#30864=CARTESIAN_POINT('Ctrl Pts',(-56.8224078151577,-108.218327410317,
171.975054738546));
#30865=CARTESIAN_POINT('Ctrl Pts',(-58.4642844518147,-107.949011163088,
171.975054808055));
#30866=CARTESIAN_POINT('Ctrl Pts',(-60.1061610884719,-107.679694915859,
171.975054877564));
#30867=CARTESIAN_POINT('Ctrl Pts',(-61.2642323520143,-107.461955553656,
173.149682754692));
#30868=CARTESIAN_POINT('Ctrl Pts',(-62.4223036155567,-107.244216191453,
174.32431063182));
#30869=CARTESIAN_POINT('Ctrl Pts',(-62.4123654835228,-107.150994434166,
175.985485236888));
#30870=CARTESIAN_POINT('Ctrl Pts',(-62.4024273514889,-107.057772676879,
177.646659841956));
#30871=CARTESIAN_POINT('Ctrl Pts',(-61.2244798643663,-107.089068520192,
178.821287620784));
#30872=CARTESIAN_POINT('Ctrl Pts',(-60.0465323772438,-107.120364363504,
179.995915399612));
#30873=CARTESIAN_POINT('Ctrl Pts',(-58.3847796147526,-107.203237081423,
179.995915330104));
#30874=CARTESIAN_POINT('Ctrl Pts',(-56.7230268522615,-107.286109799341,
179.995915260595));
#30875=CARTESIAN_POINT('Ctrl Pts',(-55.5450794628851,-107.317405632233,
178.821287383467));
#30876=CARTESIAN_POINT('Ctrl Pts',(-54.3671320735086,-107.348701465125,
177.646659506339));
#30877=CARTESIAN_POINT('Ctrl Pts',(-54.3571940797085,-107.255479693102,
175.985484901271));
#30878=CARTESIAN_POINT('Ctrl Pts',(-54.3472560859084,-107.162257921078,
174.324310296203));
#30879=CARTESIAN_POINT('Ctrl Pts',(-55.5053274471969,-106.944518548455,
173.149682517375));
#30880=CARTESIAN_POINT('Ctrl Pts',(-56.6633988084854,-106.726779175832,
171.975054738546));
#30881=CARTESIAN_POINT('Ctrl Pts',(-58.3052754451425,-106.457462928602,
171.975054808055));
#30882=CARTESIAN_POINT('Ctrl Pts',(-59.9471520817997,-106.188146681373,
171.975054877564));
#30883=CARTESIAN_POINT('Ctrl Pts',(-61.1052233453421,-105.97040731917,173.149682754692));
#30884=CARTESIAN_POINT('Ctrl Pts',(-62.2632946088845,-105.752667956968,
174.32431063182));
#30885=CARTESIAN_POINT('Ctrl Pts',(-62.2533564768505,-105.659446199681,
175.985485236888));
#30886=CARTESIAN_POINT('Ctrl Pts',(-62.2434183448166,-105.566224442394,
177.646659841956));
#30887=CARTESIAN_POINT('Ctrl Pts',(-61.0654708576941,-105.597520285706,
178.821287620784));
#30888=CARTESIAN_POINT('Ctrl Pts',(-59.8875233705716,-105.628816129018,
179.995915399612));
#30889=CARTESIAN_POINT('Ctrl Pts',(-58.2257706080804,-105.711688846937,
179.995915330104));
#30890=CARTESIAN_POINT('Ctrl Pts',(-56.5640178455893,-105.794561564856,
179.995915260595));
#30891=CARTESIAN_POINT('Ctrl Pts',(-55.3860704562128,-105.825857397748,
178.821287383467));
#30892=CARTESIAN_POINT('Ctrl Pts',(-54.2081230668364,-105.85715323064,177.646659506339));
#30893=CARTESIAN_POINT('Ctrl Pts',(-54.1981850730363,-105.763931458616,
175.985484901271));
#30894=CARTESIAN_POINT('Ctrl Pts',(-54.1882470792362,-105.670709686593,
174.324310296203));
#30895=CARTESIAN_POINT('Ctrl Pts',(-55.3463184405247,-105.452970313969,
173.149682517375));
#30896=CARTESIAN_POINT('Ctrl Pts',(-56.5043898018132,-105.235230941346,
171.975054738546));
#30897=CARTESIAN_POINT('Ctrl Pts',(-58.1462664384703,-104.965914694117,
171.975054808055));
#30898=CARTESIAN_POINT('Ctrl Pts',(-59.7881430751274,-104.696598446888,
171.975054877564));
#30899=CARTESIAN_POINT('Ctrl Pts',(-60.9462143386698,-104.478859084685,
173.149682754692));
#30900=CARTESIAN_POINT('Ctrl Pts',(-62.1042856022123,-104.261119722482,
174.32431063182));
#30901=CARTESIAN_POINT('Ctrl Pts',(-62.0943474701783,-104.167897965195,
175.985485236888));
#30902=CARTESIAN_POINT('Ctrl Pts',(-62.0844093381444,-104.074676207908,
177.646659841956));
#30903=CARTESIAN_POINT('Ctrl Pts',(-60.9064618510219,-104.10597205122,178.821287620784));
#30904=CARTESIAN_POINT('Ctrl Pts',(-59.7285143638993,-104.137267894533,
179.995915399612));
#30905=CARTESIAN_POINT('Ctrl Pts',(-58.0667616014082,-104.220140612451,
179.995915330104));
#30906=CARTESIAN_POINT('Ctrl Pts',(-56.4050088389171,-104.30301333037,179.995915260595));
#30907=CARTESIAN_POINT('Ctrl Pts',(-55.2270614495406,-104.334309163262,
178.821287383467));
#30908=CARTESIAN_POINT('Ctrl Pts',(-54.0491140601642,-104.365604996154,
177.646659506339));
#30909=CARTESIAN_POINT('Ctrl Pts',(-54.039176066364,-104.272383224131,175.985484901271));
#30910=CARTESIAN_POINT('Ctrl Pts',(-54.029238072564,-104.179161452107,174.324310296203));
#30911=CARTESIAN_POINT('Ctrl Pts',(-55.1873094338524,-103.961422079484,
173.149682517375));
#30912=CARTESIAN_POINT('Ctrl Pts',(-56.345380795141,-103.743682706861,171.975054738546));
#30913=CARTESIAN_POINT('Ctrl Pts',(-57.9872574317981,-103.474366459631,
171.975054808055));
#30914=CARTESIAN_POINT('Ctrl Pts',(-59.6291340684552,-103.205050212402,
171.975054877564));
#30915=CARTESIAN_POINT('Ctrl Pts',(-60.7872053319976,-102.987310850199,
173.149682754692));
#30916=CARTESIAN_POINT('Ctrl Pts',(-61.94527659554,-102.769571487996,174.32431063182));
#30917=CARTESIAN_POINT('Ctrl Pts',(-61.9353384635061,-102.676349730709,
175.985485236888));
#30918=CARTESIAN_POINT('Ctrl Pts',(-61.9254003314722,-102.583127973422,
177.646659841956));
#30919=CARTESIAN_POINT('Ctrl Pts',(-60.7474528443496,-102.614423816735,
178.821287620784));
#30920=CARTESIAN_POINT('Ctrl Pts',(-59.5695053572271,-102.645719660047,
179.995915399612));
#30921=CARTESIAN_POINT('Ctrl Pts',(-57.907752594736,-102.728592377966,179.995915330104));
#30922=CARTESIAN_POINT('Ctrl Pts',(-56.2459998322448,-102.811465095885,
179.995915260595));
#30923=CARTESIAN_POINT('Ctrl Pts',(-55.0680524428684,-102.842760928777,
178.821287383467));
#30924=CARTESIAN_POINT('Ctrl Pts',(-53.8901050534919,-102.874056761669,
177.646659506339));
#30925=CARTESIAN_POINT('Ctrl Pts',(-53.8801670596918,-102.780834989645,
175.985484901271));
#30926=CARTESIAN_POINT('Ctrl Pts',(-53.8702290658917,-102.687613217621,
174.324310296203));
#30927=CARTESIAN_POINT('Ctrl Pts',(-55.0283004271802,-102.469873844998,
173.149682517375));
#30928=CARTESIAN_POINT('Ctrl Pts',(-56.1863717884687,-102.252134472375,
171.975054738546));
#30929=CARTESIAN_POINT('Ctrl Pts',(-57.8282484251258,-101.982818225146,
171.975054808055));
#30930=CARTESIAN_POINT('Ctrl Pts',(-59.470125061783,-101.713501977916,171.975054877564));
#30931=CARTESIAN_POINT('Ctrl Pts',(-60.6281963253254,-101.495762615714,
173.149682754692));
#30932=CARTESIAN_POINT('Ctrl Pts',(-61.7862675888678,-101.278023253511,
174.32431063182));
#30933=CARTESIAN_POINT('Ctrl Pts',(-61.7763294568339,-101.184801496224,
175.985485236888));
#30934=CARTESIAN_POINT('Ctrl Pts',(-61.7663913247999,-101.091579738937,
177.646659841956));
#30935=CARTESIAN_POINT('Ctrl Pts',(-60.5884438376774,-101.122875582249,
178.821287620784));
#30936=CARTESIAN_POINT('Ctrl Pts',(-59.4104963505549,-101.154171425562,
179.995915399612));
#30937=CARTESIAN_POINT('Ctrl Pts',(-57.7487435880637,-101.23704414348,179.995915330104));
#30938=CARTESIAN_POINT('Ctrl Pts',(-56.0869908255726,-101.319916861399,
179.995915260595));
#30939=CARTESIAN_POINT('Ctrl Pts',(-54.9090434361961,-101.351212694291,
178.821287383467));
#30940=CARTESIAN_POINT('Ctrl Pts',(-53.7310960468197,-101.382508527183,
177.646659506339));
#30941=CARTESIAN_POINT('Ctrl Pts',(-53.7211580530196,-101.289286755159,
175.985484901271));
#30942=CARTESIAN_POINT('Ctrl Pts',(-53.7112200592195,-101.196064983136,
174.324310296203));
#30943=CARTESIAN_POINT('Ctrl Pts',(-54.869291420508,-100.978325610513,173.149682517375));
#30944=CARTESIAN_POINT('Ctrl Pts',(-56.0273627817965,-100.760586237889,
171.975054738546));
#30945=CARTESIAN_POINT('Ctrl Pts',(-57.6692394184536,-100.49126999066,171.975054808055));
#30946=CARTESIAN_POINT('Ctrl Pts',(-59.3111160551107,-100.221953743431,
171.975054877564));
#30947=CARTESIAN_POINT('Ctrl Pts',(-60.4691873186531,-100.004214381228,
173.149682754692));
#30948=CARTESIAN_POINT('Ctrl Pts',(-61.6272585821956,-99.7864750190253,
174.32431063182));
#30949=CARTESIAN_POINT('Ctrl Pts',(-61.6173204501616,-99.6932532617382,
175.985485236888));
#30950=CARTESIAN_POINT('Ctrl Pts',(-61.6073823181277,-99.6000315044512,
177.646659841956));
#30951=CARTESIAN_POINT('Ctrl Pts',(-60.4294348310052,-99.6313273477637,
178.821287620784));
#30952=CARTESIAN_POINT('Ctrl Pts',(-59.2514873438827,-99.6626231910761,
179.995915399612));
#30953=CARTESIAN_POINT('Ctrl Pts',(-57.5897345813915,-99.7454959089947,
179.995915330104));
#30954=CARTESIAN_POINT('Ctrl Pts',(-55.9279818189004,-99.8283686269133,
179.995915260595));
#30955=CARTESIAN_POINT('Ctrl Pts',(-54.7500344295239,-99.8596644598054,
178.821287383467));
#30956=CARTESIAN_POINT('Ctrl Pts',(-53.5720870401475,-99.8909602926975,
177.646659506339));
#30957=CARTESIAN_POINT('Ctrl Pts',(-53.5621490463474,-99.7977385206737,
175.985484901271));
#30958=CARTESIAN_POINT('Ctrl Pts',(-53.5522110525473,-99.7045167486501,
174.324310296203));
#30959=CARTESIAN_POINT('Ctrl Pts',(-54.7102824138358,-99.4867773760269,
173.149682517375));
#30960=CARTESIAN_POINT('Ctrl Pts',(-55.8683537751243,-99.2690380034038,
171.975054738546));
#30961=CARTESIAN_POINT('Ctrl Pts',(-57.5102304117814,-98.9997217561745,
171.975054808055));
#30962=CARTESIAN_POINT('Ctrl Pts',(-59.1521070484385,-98.7304055089452,
171.975054877564));
#30963=CARTESIAN_POINT('Ctrl Pts',(-60.3101783119809,-98.5126661467424,
173.149682754692));
#30964=CARTESIAN_POINT('Ctrl Pts',(-61.4682495755234,-98.2949267845397,
174.32431063182));
#30965=CARTESIAN_POINT('Ctrl Pts',(-61.4583114434894,-98.2017050272526,
175.985485236888));
#30966=CARTESIAN_POINT('Ctrl Pts',(-61.4483733114555,-98.1084832699656,
177.646659841956));
#30967=CARTESIAN_POINT('Ctrl Pts',(-60.2704258243329,-98.139779113278,178.821287620784));
#30968=CARTESIAN_POINT('Ctrl Pts',(-59.0924783372104,-98.1710749565905,
179.995915399612));
#30969=CARTESIAN_POINT('Ctrl Pts',(-57.4307255747193,-98.2539476745091,
179.995915330104));
#30970=CARTESIAN_POINT('Ctrl Pts',(-55.7689728122282,-98.3368203924277,
179.995915260595));
#30971=CARTESIAN_POINT('Ctrl Pts',(-54.5910254228517,-98.3681162253198,
178.821287383467));
#30972=CARTESIAN_POINT('Ctrl Pts',(-56.1988062143188,-113.449542435949,
178.821287383467));
#30973=CARTESIAN_POINT('Ctrl Pts',(-55.0208588249424,-113.480838268841,
177.646659506339));
#30974=CARTESIAN_POINT('Ctrl Pts',(-55.0109208311422,-113.387616496817,
175.985484901271));
#30975=CARTESIAN_POINT('Ctrl Pts',(-55.0009828373422,-113.294394724794,
174.324310296203));
#30976=CARTESIAN_POINT('Ctrl Pts',(-56.1590541986307,-113.07665535217,173.149682517375));
#30977=CARTESIAN_POINT('Ctrl Pts',(-57.3171255599192,-112.858915979547,
171.975054738546));
#30978=CARTESIAN_POINT('Ctrl Pts',(-58.9590021965763,-112.589599732318,
171.975054808055));
#30979=CARTESIAN_POINT('Ctrl Pts',(-60.6008788332334,-112.320283485089,
171.975054877564));
#30980=CARTESIAN_POINT('Ctrl Pts',(-61.7589500967758,-112.102544122886,
173.149682754692));
#30981=CARTESIAN_POINT('Ctrl Pts',(-62.9170213603182,-111.884804760683,
174.32431063182));
#30982=CARTESIAN_POINT('Ctrl Pts',(-62.9070832282843,-111.791583003396,
175.985485236888));
#30983=CARTESIAN_POINT('Ctrl Pts',(-62.8971450962504,-111.698361246109,
177.646659841956));
#30984=CARTESIAN_POINT('Ctrl Pts',(-61.7191976091278,-111.729657089422,
178.821287620784));
#30985=CARTESIAN_POINT('Ctrl Pts',(-60.5412501220053,-111.760952932734,
179.995915399612));
#30986=CARTESIAN_POINT('Ctrl Pts',(-58.8794973595142,-111.843825650653,
179.995915330104));
#30987=CARTESIAN_POINT('Ctrl Pts',(-57.217744597023,-111.926698368571,179.995915260595));
#30988=CARTESIAN_POINT('Ctrl Pts',(-56.0397972076466,-111.957994201463,
178.821287383467));
#30989=CARTESIAN_POINT('Ctrl Pts',(-54.8618498182701,-111.989290034355,
177.646659506339));
#30990=CARTESIAN_POINT('Ctrl Pts',(-54.85191182447,-111.896068262332,175.985484901271));
#30991=CARTESIAN_POINT('Ctrl Pts',(-54.8419738306699,-111.802846490308,
174.324310296203));
#30992=CARTESIAN_POINT('Ctrl Pts',(-56.0000451919584,-111.585107117685,
173.149682517375));
#30993=CARTESIAN_POINT('Ctrl Pts',(-57.158116553247,-111.367367745062,171.975054738546));
#30994=CARTESIAN_POINT('Ctrl Pts',(-58.799993189904,-111.098051497832,171.975054808055));
#30995=CARTESIAN_POINT('Ctrl Pts',(-60.4418698265612,-110.828735250603,
171.975054877564));
#30996=CARTESIAN_POINT('Ctrl Pts',(-61.5999410901036,-110.6109958884,173.149682754692));
#30997=CARTESIAN_POINT('Ctrl Pts',(-62.758012353646,-110.393256526198,174.32431063182));
#30998=CARTESIAN_POINT('Ctrl Pts',(-62.7480742216121,-110.30003476891,175.985485236888));
#30999=CARTESIAN_POINT('Ctrl Pts',(-62.7381360895782,-110.206813011623,
177.646659841956));
#31000=CARTESIAN_POINT('Ctrl Pts',(-61.5601886024556,-110.238108854936,
178.821287620784));
#31001=CARTESIAN_POINT('Ctrl Pts',(-60.3822411153331,-110.269404698248,
179.995915399612));
#31002=CARTESIAN_POINT('Ctrl Pts',(-58.7204883528419,-110.352277416167,
179.995915330104));
#31003=CARTESIAN_POINT('Ctrl Pts',(-57.0587355903508,-110.435150134086,
179.995915260595));
#31004=CARTESIAN_POINT('Ctrl Pts',(-55.8807882009743,-110.466445966978,
178.821287383467));
#31005=CARTESIAN_POINT('Ctrl Pts',(-54.7028408115979,-110.49774179987,177.646659506339));
#31006=CARTESIAN_POINT('Ctrl Pts',(-54.6929028177978,-110.404520027846,
175.985484901271));
#31007=CARTESIAN_POINT('Ctrl Pts',(-54.6829648239977,-110.311298255822,
174.324310296203));
#31008=CARTESIAN_POINT('Ctrl Pts',(-55.8410361852862,-110.093558883199,
173.149682517375));
#31009=CARTESIAN_POINT('Ctrl Pts',(-56.9991075465747,-109.875819510576,
171.975054738546));
#31010=CARTESIAN_POINT('Ctrl Pts',(-58.6409841832318,-109.606503263347,
171.975054808055));
#31011=CARTESIAN_POINT('Ctrl Pts',(-60.2828608198889,-109.337187016117,
171.975054877564));
#31012=CARTESIAN_POINT('Ctrl Pts',(-61.4409320834313,-109.119447653915,
173.149682754692));
#31013=CARTESIAN_POINT('Ctrl Pts',(-62.5990033469738,-108.901708291712,
174.32431063182));
#31014=CARTESIAN_POINT('Ctrl Pts',(-62.5890652149398,-108.808486534425,
175.985485236888));
#31015=CARTESIAN_POINT('Ctrl Pts',(-62.5791270829059,-108.715264777138,
177.646659841956));
#31016=CARTESIAN_POINT('Ctrl Pts',(-61.4011795957834,-108.74656062045,178.821287620784));
#31017=CARTESIAN_POINT('Ctrl Pts',(-60.2232321086609,-108.777856463763,
179.995915399612));
#31018=CARTESIAN_POINT('Ctrl Pts',(-58.5614793461697,-108.860729181681,
179.995915330104));
#31019=CARTESIAN_POINT('Ctrl Pts',(-56.8997265836786,-108.9436018996,179.995915260595));
#31020=CARTESIAN_POINT('Ctrl Pts',(-55.7217791943021,-108.974897732492,
178.821287383467));
#31021=CARTESIAN_POINT('Ctrl Pts',(-54.5438318049257,-109.006193565384,
177.646659506339));
#31022=CARTESIAN_POINT('Ctrl Pts',(-54.5338938111256,-108.91297179336,175.985484901271));
#31023=CARTESIAN_POINT('Ctrl Pts',(-54.5239558173255,-108.819750021337,
174.324310296203));
#31024=CARTESIAN_POINT('Ctrl Pts',(-55.682027178614,-108.602010648714,173.149682517375));
#31025=CARTESIAN_POINT('Ctrl Pts',(-56.8400985399025,-108.384271276091,
171.975054738546));
#31026=CARTESIAN_POINT('Ctrl Pts',(-58.4819751765596,-108.114955028861,
171.975054808055));
#31027=CARTESIAN_POINT('Ctrl Pts',(-60.1238518132167,-107.845638781632,
171.975054877564));
#31028=CARTESIAN_POINT('Ctrl Pts',(-61.2819230767591,-107.627899419429,
173.149682754692));
#31029=CARTESIAN_POINT('Ctrl Pts',(-62.4399943403016,-107.410160057226,
174.32431063182));
#31030=CARTESIAN_POINT('Ctrl Pts',(-62.4300562082676,-107.316938299939,
175.985485236888));
#31031=CARTESIAN_POINT('Ctrl Pts',(-62.4201180762337,-107.223716542652,
177.646659841956));
#31032=CARTESIAN_POINT('Ctrl Pts',(-61.2421705891111,-107.255012385965,
178.821287620784));
#31033=CARTESIAN_POINT('Ctrl Pts',(-60.0642231019886,-107.286308229277,
179.995915399612));
#31034=CARTESIAN_POINT('Ctrl Pts',(-58.4024703394975,-107.369180947196,
179.995915330104));
#31035=CARTESIAN_POINT('Ctrl Pts',(-56.7407175770064,-107.452053665114,
179.995915260595));
#31036=CARTESIAN_POINT('Ctrl Pts',(-55.5627701876299,-107.483349498006,
178.821287383467));
#31037=CARTESIAN_POINT('Ctrl Pts',(-54.3848227982534,-107.514645330899,
177.646659506339));
#31038=CARTESIAN_POINT('Ctrl Pts',(-54.3748848044533,-107.421423558875,
175.985484901271));
#31039=CARTESIAN_POINT('Ctrl Pts',(-54.3649468106533,-107.328201786851,
174.324310296203));
#31040=CARTESIAN_POINT('Ctrl Pts',(-55.5230181719417,-107.110462414228,
173.149682517375));
#31041=CARTESIAN_POINT('Ctrl Pts',(-56.6810895332303,-106.892723041605,
171.975054738546));
#31042=CARTESIAN_POINT('Ctrl Pts',(-58.3229661698874,-106.623406794376,
171.975054808055));
#31043=CARTESIAN_POINT('Ctrl Pts',(-59.9648428065445,-106.354090547146,
171.975054877564));
#31044=CARTESIAN_POINT('Ctrl Pts',(-61.1229140700869,-106.136351184943,
173.149682754692));
#31045=CARTESIAN_POINT('Ctrl Pts',(-62.2809853336293,-105.918611822741,
174.32431063182));
#31046=CARTESIAN_POINT('Ctrl Pts',(-62.2710472015954,-105.825390065454,
175.985485236888));
#31047=CARTESIAN_POINT('Ctrl Pts',(-62.2611090695615,-105.732168308167,
177.646659841956));
#31048=CARTESIAN_POINT('Ctrl Pts',(-61.0831615824389,-105.763464151479,
178.821287620784));
#31049=CARTESIAN_POINT('Ctrl Pts',(-59.9052140953164,-105.794759994792,
179.995915399612));
#31050=CARTESIAN_POINT('Ctrl Pts',(-58.2434613328252,-105.87763271271,179.995915330104));
#31051=CARTESIAN_POINT('Ctrl Pts',(-56.5817085703341,-105.960505430629,
179.995915260595));
#31052=CARTESIAN_POINT('Ctrl Pts',(-55.4037611809577,-105.991801263521,
178.821287383467));
#31053=CARTESIAN_POINT('Ctrl Pts',(-54.2258137915812,-106.023097096413,
177.646659506339));
#31054=CARTESIAN_POINT('Ctrl Pts',(-54.2158757977811,-105.929875324389,
175.985484901271));
#31055=CARTESIAN_POINT('Ctrl Pts',(-54.205937803981,-105.836653552366,174.324310296203));
#31056=CARTESIAN_POINT('Ctrl Pts',(-55.3640091652695,-105.618914179742,
173.149682517375));
#31057=CARTESIAN_POINT('Ctrl Pts',(-56.522080526558,-105.401174807119,171.975054738546));
#31058=CARTESIAN_POINT('Ctrl Pts',(-58.1639571632151,-105.13185855989,171.975054808055));
#31059=CARTESIAN_POINT('Ctrl Pts',(-59.8058337998722,-104.862542312661,
171.975054877564));
#31060=CARTESIAN_POINT('Ctrl Pts',(-60.9639050634147,-104.644802950458,
173.149682754692));
#31061=CARTESIAN_POINT('Ctrl Pts',(-62.1219763269571,-104.427063588255,
174.32431063182));
#31062=CARTESIAN_POINT('Ctrl Pts',(-62.1120381949232,-104.333841830968,
175.985485236888));
#31063=CARTESIAN_POINT('Ctrl Pts',(-62.1021000628892,-104.240620073681,
177.646659841956));
#31064=CARTESIAN_POINT('Ctrl Pts',(-60.9241525757667,-104.271915916993,
178.821287620784));
#31065=CARTESIAN_POINT('Ctrl Pts',(-59.7462050886442,-104.303211760306,
179.995915399612));
#31066=CARTESIAN_POINT('Ctrl Pts',(-58.084452326153,-104.386084478225,179.995915330104));
#31067=CARTESIAN_POINT('Ctrl Pts',(-56.4226995636619,-104.468957196143,
179.995915260595));
#31068=CARTESIAN_POINT('Ctrl Pts',(-55.2447521742854,-104.500253029035,
178.821287383467));
#31069=CARTESIAN_POINT('Ctrl Pts',(-54.066804784909,-104.531548861927,177.646659506339));
#31070=CARTESIAN_POINT('Ctrl Pts',(-54.0568667911089,-104.438327089904,
175.985484901271));
#31071=CARTESIAN_POINT('Ctrl Pts',(-54.0469287973088,-104.34510531788,174.324310296203));
#31072=CARTESIAN_POINT('Ctrl Pts',(-55.2050001585973,-104.127365945257,
173.149682517375));
#31073=CARTESIAN_POINT('Ctrl Pts',(-56.3630715198858,-103.909626572634,
171.975054738546));
#31074=CARTESIAN_POINT('Ctrl Pts',(-58.0049481565429,-103.640310325404,
171.975054808055));
#31075=CARTESIAN_POINT('Ctrl Pts',(-59.6468247932,-103.370994078175,171.975054877564));
#31076=CARTESIAN_POINT('Ctrl Pts',(-60.8048960567424,-103.153254715972,
173.149682754692));
#31077=CARTESIAN_POINT('Ctrl Pts',(-61.9629673202849,-102.93551535377,174.32431063182));
#31078=CARTESIAN_POINT('Ctrl Pts',(-61.9530291882509,-102.842293596483,
175.985485236888));
#31079=CARTESIAN_POINT('Ctrl Pts',(-61.943091056217,-102.749071839196,177.646659841956));
#31080=CARTESIAN_POINT('Ctrl Pts',(-60.7651435690945,-102.780367682508,
178.821287620784));
#31081=CARTESIAN_POINT('Ctrl Pts',(-59.587196081972,-102.81166352582,179.995915399612));
#31082=CARTESIAN_POINT('Ctrl Pts',(-57.9254433194808,-102.894536243739,
179.995915330104));
#31083=CARTESIAN_POINT('Ctrl Pts',(-56.2636905569897,-102.977408961658,
179.995915260595));
#31084=CARTESIAN_POINT('Ctrl Pts',(-55.0857431676132,-103.00870479455,178.821287383467));
#31085=CARTESIAN_POINT('Ctrl Pts',(-53.9077957782368,-103.040000627442,
177.646659506339));
#31086=CARTESIAN_POINT('Ctrl Pts',(-53.8978577844367,-102.946778855418,
175.985484901271));
#31087=CARTESIAN_POINT('Ctrl Pts',(-53.8879197906366,-102.853557083394,
174.324310296203));
#31088=CARTESIAN_POINT('Ctrl Pts',(-55.0459911519251,-102.635817710771,
173.149682517375));
#31089=CARTESIAN_POINT('Ctrl Pts',(-56.2040625132136,-102.418078338148,
171.975054738546));
#31090=CARTESIAN_POINT('Ctrl Pts',(-57.8459391498707,-102.148762090919,
171.975054808055));
#31091=CARTESIAN_POINT('Ctrl Pts',(-59.4878157865278,-101.879445843689,
171.975054877564));
#31092=CARTESIAN_POINT('Ctrl Pts',(-60.6458870500702,-101.661706481487,
173.149682754692));
#31093=CARTESIAN_POINT('Ctrl Pts',(-61.8039583136126,-101.443967119284,
174.32431063182));
#31094=CARTESIAN_POINT('Ctrl Pts',(-61.7940201815787,-101.350745361997,
175.985485236888));
#31095=CARTESIAN_POINT('Ctrl Pts',(-61.7840820495448,-101.25752360471,177.646659841956));
#31096=CARTESIAN_POINT('Ctrl Pts',(-60.6061345624222,-101.288819448022,
178.821287620784));
#31097=CARTESIAN_POINT('Ctrl Pts',(-59.4281870752997,-101.320115291335,
179.995915399612));
#31098=CARTESIAN_POINT('Ctrl Pts',(-57.7664343128086,-101.402988009253,
179.995915330104));
#31099=CARTESIAN_POINT('Ctrl Pts',(-56.1046815503175,-101.485860727172,
179.995915260595));
#31100=CARTESIAN_POINT('Ctrl Pts',(-54.926734160941,-101.517156560064,178.821287383467));
#31101=CARTESIAN_POINT('Ctrl Pts',(-53.7487867715645,-101.548452392956,
177.646659506339));
#31102=CARTESIAN_POINT('Ctrl Pts',(-53.7388487777644,-101.455230620932,
175.985484901271));
#31103=CARTESIAN_POINT('Ctrl Pts',(-53.7289107839643,-101.362008848909,
174.324310296203));
#31104=CARTESIAN_POINT('Ctrl Pts',(-54.8869821452528,-101.144269476286,
173.149682517375));
#31105=CARTESIAN_POINT('Ctrl Pts',(-56.0450535065414,-100.926530103662,
171.975054738546));
#31106=CARTESIAN_POINT('Ctrl Pts',(-57.6869301431984,-100.657213856433,
171.975054808055));
#31107=CARTESIAN_POINT('Ctrl Pts',(-59.3288067798556,-100.387897609204,
171.975054877564));
#31108=CARTESIAN_POINT('Ctrl Pts',(-60.486878043398,-100.170158247001,173.149682754692));
#31109=CARTESIAN_POINT('Ctrl Pts',(-61.6449493069404,-99.9524188847983,
174.32431063182));
#31110=CARTESIAN_POINT('Ctrl Pts',(-61.6350111749065,-99.8591971275113,
175.985485236888));
#31111=CARTESIAN_POINT('Ctrl Pts',(-61.6250730428726,-99.7659753702243,
177.646659841956));
#31112=CARTESIAN_POINT('Ctrl Pts',(-60.44712555575,-99.7972712135367,178.821287620784));
#31113=CARTESIAN_POINT('Ctrl Pts',(-59.2691780686275,-99.8285670568492,
179.995915399612));
#31114=CARTESIAN_POINT('Ctrl Pts',(-57.6074253061363,-99.9114397747677,
179.995915330104));
#31115=CARTESIAN_POINT('Ctrl Pts',(-55.9456725436452,-99.9943124926864,
179.995915260595));
#31116=CARTESIAN_POINT('Ctrl Pts',(-54.7677251542687,-100.025608325578,
178.821287383467));
#31117=CARTESIAN_POINT('Ctrl Pts',(-53.5897777648923,-100.05690415847,177.646659506339));
#31118=CARTESIAN_POINT('Ctrl Pts',(-53.5798397710922,-99.9636823864468,
175.985484901271));
#31119=CARTESIAN_POINT('Ctrl Pts',(-53.5699017772921,-99.8704606144232,
174.324310296203));
#31120=CARTESIAN_POINT('Ctrl Pts',(-54.7279731385806,-99.6527212418,173.149682517375));
#31121=CARTESIAN_POINT('Ctrl Pts',(-55.8860444998691,-99.4349818691769,
171.975054738546));
#31122=CARTESIAN_POINT('Ctrl Pts',(-57.5279211365262,-99.1656656219475,
171.975054808055));
#31123=CARTESIAN_POINT('Ctrl Pts',(-59.1697977731833,-98.8963493747183,
171.975054877564));
#31124=CARTESIAN_POINT('Ctrl Pts',(-60.3278690367257,-98.6786100125155,
173.149682754692));
#31125=CARTESIAN_POINT('Ctrl Pts',(-61.4859403002682,-98.4608706503128,
174.32431063182));
#31126=CARTESIAN_POINT('Ctrl Pts',(-61.4760021682342,-98.3676488930257,
175.985485236888));
#31127=CARTESIAN_POINT('Ctrl Pts',(-61.4660640362003,-98.2744271357387,
177.646659841956));
#31128=CARTESIAN_POINT('Ctrl Pts',(-60.2881165490778,-98.3057229790511,
178.821287620784));
#31129=CARTESIAN_POINT('Ctrl Pts',(-59.1101690619552,-98.3370188223636,
179.995915399612));
#31130=CARTESIAN_POINT('Ctrl Pts',(-57.4484162994641,-98.4198915402821,
179.995915330104));
#31131=CARTESIAN_POINT('Ctrl Pts',(-55.786663536973,-98.5027642582008,179.995915260595));
#31132=CARTESIAN_POINT('Ctrl Pts',(-54.6087161475965,-98.5340600910929,
178.821287383467));
#31133=CARTESIAN_POINT('Ctrl Pts',(-56.2237961054143,-113.614380048479,
178.813912075476));
#31134=CARTESIAN_POINT('Ctrl Pts',(-55.0488864554725,-113.645352038053,
177.6423391512));
#31135=CARTESIAN_POINT('Ctrl Pts',(-55.0389484614927,-113.552130266048,
175.985484901707));
#31136=CARTESIAN_POINT('Ctrl Pts',(-55.0290104675128,-113.458908494044,
174.328630652215));
#31137=CARTESIAN_POINT('Ctrl Pts',(-56.1840440891124,-113.241492964766,
173.157057825983));
#31138=CARTESIAN_POINT('Ctrl Pts',(-57.3390777107121,-113.024077435489,
171.985484999752));
#31139=CARTESIAN_POINT('Ctrl Pts',(-58.9766583348819,-112.755219171892,
171.985485069079));
#31140=CARTESIAN_POINT('Ctrl Pts',(-60.6142389590518,-112.486360908295,
171.985485138407));
#31141=CARTESIAN_POINT('Ctrl Pts',(-61.7692724831595,-112.268945389411,
173.157058062683));
#31142=CARTESIAN_POINT('Ctrl Pts',(-62.9243060072673,-112.051529870527,
174.328630986959));
#31143=CARTESIAN_POINT('Ctrl Pts',(-62.9143678754131,-111.95830811322,175.985485236451));
#31144=CARTESIAN_POINT('Ctrl Pts',(-62.9044297435589,-111.865086355914,
177.642339485944));
#31145=CARTESIAN_POINT('Ctrl Pts',(-61.7295199961253,-111.896058355881,
178.813912312176));
#31146=CARTESIAN_POINT('Ctrl Pts',(-60.5546102486917,-111.927030355848,
179.985485138407));
#31147=CARTESIAN_POINT('Ctrl Pts',(-58.8971534986878,-112.009445090134,
179.985485069079));
#31148=CARTESIAN_POINT('Ctrl Pts',(-57.2396967486839,-112.09185982442,179.985484999752));
#31149=CARTESIAN_POINT('Ctrl Pts',(-56.0647870987421,-112.122831813994,
178.813912075476));
#31150=CARTESIAN_POINT('Ctrl Pts',(-54.8898774488003,-112.153803803567,
177.6423391512));
#31151=CARTESIAN_POINT('Ctrl Pts',(-54.8799394548205,-112.060582031563,
175.985484901707));
#31152=CARTESIAN_POINT('Ctrl Pts',(-54.8700014608406,-111.967360259558,
174.328630652215));
#31153=CARTESIAN_POINT('Ctrl Pts',(-56.0250350824402,-111.749944730281,
173.157057825983));
#31154=CARTESIAN_POINT('Ctrl Pts',(-57.1800687040398,-111.532529201003,
171.985484999752));
#31155=CARTESIAN_POINT('Ctrl Pts',(-58.8176493282097,-111.263670937406,
171.985485069079));
#31156=CARTESIAN_POINT('Ctrl Pts',(-60.4552299523796,-110.994812673809,
171.985485138407));
#31157=CARTESIAN_POINT('Ctrl Pts',(-61.6102634764873,-110.777397154925,
173.157058062683));
#31158=CARTESIAN_POINT('Ctrl Pts',(-62.7652970005951,-110.559981636041,
174.328630986959));
#31159=CARTESIAN_POINT('Ctrl Pts',(-62.7553588687409,-110.466759878735,
175.985485236451));
#31160=CARTESIAN_POINT('Ctrl Pts',(-62.7454207368867,-110.373538121429,
177.642339485944));
#31161=CARTESIAN_POINT('Ctrl Pts',(-61.5705109894531,-110.404510121395,
178.813912312176));
#31162=CARTESIAN_POINT('Ctrl Pts',(-60.3956012420194,-110.435482121362,
179.985485138407));
#31163=CARTESIAN_POINT('Ctrl Pts',(-58.7381444920155,-110.517896855648,
179.985485069079));
#31164=CARTESIAN_POINT('Ctrl Pts',(-57.0806877420116,-110.600311589935,
179.985484999752));
#31165=CARTESIAN_POINT('Ctrl Pts',(-55.9057780920699,-110.631283579508,
178.813912075476));
#31166=CARTESIAN_POINT('Ctrl Pts',(-54.7308684421281,-110.662255569082,
177.6423391512));
#31167=CARTESIAN_POINT('Ctrl Pts',(-54.7209304481482,-110.569033797077,
175.985484901707));
#31168=CARTESIAN_POINT('Ctrl Pts',(-54.7109924541684,-110.475812025073,
174.328630652215));
#31169=CARTESIAN_POINT('Ctrl Pts',(-55.866026075768,-110.258396495795,173.157057825983));
#31170=CARTESIAN_POINT('Ctrl Pts',(-57.0210596973676,-110.040980966518,
171.985484999752));
#31171=CARTESIAN_POINT('Ctrl Pts',(-58.6586403215375,-109.772122702921,
171.985485069079));
#31172=CARTESIAN_POINT('Ctrl Pts',(-60.2962209457073,-109.503264439324,
171.985485138407));
#31173=CARTESIAN_POINT('Ctrl Pts',(-61.4512544698151,-109.28584892044,173.157058062683));
#31174=CARTESIAN_POINT('Ctrl Pts',(-62.6062879939228,-109.068433401555,
174.328630986959));
#31175=CARTESIAN_POINT('Ctrl Pts',(-62.5963498620687,-108.975211644249,
175.985485236451));
#31176=CARTESIAN_POINT('Ctrl Pts',(-62.5864117302145,-108.881989886943,
177.642339485944));
#31177=CARTESIAN_POINT('Ctrl Pts',(-61.4115019827808,-108.91296188691,178.813912312176));
#31178=CARTESIAN_POINT('Ctrl Pts',(-60.2365922353472,-108.943933886877,
179.985485138407));
#31179=CARTESIAN_POINT('Ctrl Pts',(-58.5791354853433,-109.026348621163,
179.985485069079));
#31180=CARTESIAN_POINT('Ctrl Pts',(-56.9216787353394,-109.108763355449,
179.985484999752));
#31181=CARTESIAN_POINT('Ctrl Pts',(-55.7467690853976,-109.139735345023,
178.813912075476));
#31182=CARTESIAN_POINT('Ctrl Pts',(-54.5718594354559,-109.170707334596,
177.6423391512));
#31183=CARTESIAN_POINT('Ctrl Pts',(-54.561921441476,-109.077485562592,175.985484901707));
#31184=CARTESIAN_POINT('Ctrl Pts',(-54.5519834474962,-108.984263790587,
174.328630652215));
#31185=CARTESIAN_POINT('Ctrl Pts',(-55.7070170690958,-108.76684826131,173.157057825983));
#31186=CARTESIAN_POINT('Ctrl Pts',(-56.8620506906954,-108.549432732032,
171.985484999752));
#31187=CARTESIAN_POINT('Ctrl Pts',(-58.4996313148652,-108.280574468435,
171.985485069079));
#31188=CARTESIAN_POINT('Ctrl Pts',(-60.1372119390351,-108.011716204838,
171.985485138407));
#31189=CARTESIAN_POINT('Ctrl Pts',(-61.2922454631428,-107.794300685954,
173.157058062683));
#31190=CARTESIAN_POINT('Ctrl Pts',(-62.4472789872506,-107.57688516707,174.328630986959));
#31191=CARTESIAN_POINT('Ctrl Pts',(-62.4373408553964,-107.483663409764,
175.985485236451));
#31192=CARTESIAN_POINT('Ctrl Pts',(-62.4274027235423,-107.390441652457,
177.642339485944));
#31193=CARTESIAN_POINT('Ctrl Pts',(-61.2524929761086,-107.421413652424,
178.813912312176));
#31194=CARTESIAN_POINT('Ctrl Pts',(-60.077583228675,-107.452385652391,179.985485138407));
#31195=CARTESIAN_POINT('Ctrl Pts',(-58.4201264786711,-107.534800386677,
179.985485069079));
#31196=CARTESIAN_POINT('Ctrl Pts',(-56.7626697286672,-107.617215120964,
179.985484999752));
#31197=CARTESIAN_POINT('Ctrl Pts',(-55.5877600787254,-107.648187110537,
178.813912075476));
#31198=CARTESIAN_POINT('Ctrl Pts',(-54.4128504287836,-107.67915910011,177.6423391512));
#31199=CARTESIAN_POINT('Ctrl Pts',(-54.4029124348038,-107.585937328106,
175.985484901707));
#31200=CARTESIAN_POINT('Ctrl Pts',(-54.3929744408239,-107.492715556102,
174.328630652215));
#31201=CARTESIAN_POINT('Ctrl Pts',(-55.5480080624235,-107.275300026824,
173.157057825983));
#31202=CARTESIAN_POINT('Ctrl Pts',(-56.7030416840231,-107.057884497547,
171.985484999752));
#31203=CARTESIAN_POINT('Ctrl Pts',(-58.340622308193,-106.78902623395,171.985485069079));
#31204=CARTESIAN_POINT('Ctrl Pts',(-59.9782029323629,-106.520167970353,
171.985485138407));
#31205=CARTESIAN_POINT('Ctrl Pts',(-61.1332364564706,-106.302752451468,
173.157058062683));
#31206=CARTESIAN_POINT('Ctrl Pts',(-62.2882699805784,-106.085336932584,
174.328630986959));
#31207=CARTESIAN_POINT('Ctrl Pts',(-62.2783318487242,-105.992115175278,
175.985485236451));
#31208=CARTESIAN_POINT('Ctrl Pts',(-62.26839371687,-105.898893417972,177.642339485944));
#31209=CARTESIAN_POINT('Ctrl Pts',(-61.0934839694364,-105.929865417939,
178.813912312176));
#31210=CARTESIAN_POINT('Ctrl Pts',(-59.9185742220028,-105.960837417905,
179.985485138407));
#31211=CARTESIAN_POINT('Ctrl Pts',(-58.2611174719989,-106.043252152192,
179.985485069079));
#31212=CARTESIAN_POINT('Ctrl Pts',(-56.603660721995,-106.125666886478,179.985484999752));
#31213=CARTESIAN_POINT('Ctrl Pts',(-55.4287510720532,-106.156638876051,
178.813912075476));
#31214=CARTESIAN_POINT('Ctrl Pts',(-54.2538414221114,-106.187610865625,
177.6423391512));
#31215=CARTESIAN_POINT('Ctrl Pts',(-54.2439034281315,-106.09438909362,175.985484901707));
#31216=CARTESIAN_POINT('Ctrl Pts',(-54.2339654341517,-106.001167321616,
174.328630652215));
#31217=CARTESIAN_POINT('Ctrl Pts',(-55.3889990557513,-105.783751792338,
173.157057825983));
#31218=CARTESIAN_POINT('Ctrl Pts',(-56.5440326773509,-105.566336263061,
171.985484999752));
#31219=CARTESIAN_POINT('Ctrl Pts',(-58.1816133015208,-105.297477999464,
171.985485069079));
#31220=CARTESIAN_POINT('Ctrl Pts',(-59.8191939256906,-105.028619735867,
171.985485138407));
#31221=CARTESIAN_POINT('Ctrl Pts',(-60.9742274497984,-104.811204216983,
173.157058062683));
#31222=CARTESIAN_POINT('Ctrl Pts',(-62.1292609739061,-104.593788698099,
174.328630986959));
#31223=CARTESIAN_POINT('Ctrl Pts',(-62.119322842052,-104.500566940792,175.985485236451));
#31224=CARTESIAN_POINT('Ctrl Pts',(-62.1093847101978,-104.407345183486,
177.642339485944));
#31225=CARTESIAN_POINT('Ctrl Pts',(-60.9344749627642,-104.438317183453,
178.813912312176));
#31226=CARTESIAN_POINT('Ctrl Pts',(-59.7595652153305,-104.46928918342,179.985485138407));
#31227=CARTESIAN_POINT('Ctrl Pts',(-58.1021084653266,-104.551703917706,
179.985485069079));
#31228=CARTESIAN_POINT('Ctrl Pts',(-56.4446517153227,-104.634118651992,
179.985484999752));
#31229=CARTESIAN_POINT('Ctrl Pts',(-55.269742065381,-104.665090641566,178.813912075476));
#31230=CARTESIAN_POINT('Ctrl Pts',(-54.0948324154392,-104.696062631139,
177.6423391512));
#31231=CARTESIAN_POINT('Ctrl Pts',(-54.0848944214593,-104.602840859135,
175.985484901707));
#31232=CARTESIAN_POINT('Ctrl Pts',(-54.0749564274795,-104.50961908713,174.328630652215));
#31233=CARTESIAN_POINT('Ctrl Pts',(-55.2299900490791,-104.292203557853,
173.157057825983));
#31234=CARTESIAN_POINT('Ctrl Pts',(-56.3850236706787,-104.074788028575,
171.985484999752));
#31235=CARTESIAN_POINT('Ctrl Pts',(-58.0226042948486,-103.805929764978,
171.985485069079));
#31236=CARTESIAN_POINT('Ctrl Pts',(-59.6601849190184,-103.537071501381,
171.985485138407));
#31237=CARTESIAN_POINT('Ctrl Pts',(-60.8152184431262,-103.319655982497,
173.157058062683));
#31238=CARTESIAN_POINT('Ctrl Pts',(-61.9702519672339,-103.102240463613,
174.328630986959));
#31239=CARTESIAN_POINT('Ctrl Pts',(-61.9603138353797,-103.009018706307,
175.985485236451));
#31240=CARTESIAN_POINT('Ctrl Pts',(-61.9503757035256,-102.915796949001,
177.642339485944));
#31241=CARTESIAN_POINT('Ctrl Pts',(-60.7754659560919,-102.946768948967,
178.813912312176));
#31242=CARTESIAN_POINT('Ctrl Pts',(-59.6005562086583,-102.977740948934,
179.985485138407));
#31243=CARTESIAN_POINT('Ctrl Pts',(-57.9430994586544,-103.06015568322,179.985485069079));
#31244=CARTESIAN_POINT('Ctrl Pts',(-56.2856427086505,-103.142570417507,
179.985484999752));
#31245=CARTESIAN_POINT('Ctrl Pts',(-55.1107330587087,-103.17354240708,178.813912075476));
#31246=CARTESIAN_POINT('Ctrl Pts',(-53.935823408767,-103.204514396654,177.6423391512));
#31247=CARTESIAN_POINT('Ctrl Pts',(-53.9258854147871,-103.111292624649,
175.985484901707));
#31248=CARTESIAN_POINT('Ctrl Pts',(-53.9159474208072,-103.018070852645,
174.328630652215));
#31249=CARTESIAN_POINT('Ctrl Pts',(-55.0709810424069,-102.800655323367,
173.157057825983));
#31250=CARTESIAN_POINT('Ctrl Pts',(-56.2260146640065,-102.58323979409,171.985484999752));
#31251=CARTESIAN_POINT('Ctrl Pts',(-57.8635952881763,-102.314381530493,
171.985485069079));
#31252=CARTESIAN_POINT('Ctrl Pts',(-59.5011759123462,-102.045523266896,
171.985485138407));
#31253=CARTESIAN_POINT('Ctrl Pts',(-60.6562094364539,-101.828107748012,
173.157058062683));
#31254=CARTESIAN_POINT('Ctrl Pts',(-61.8112429605617,-101.610692229127,
174.328630986959));
#31255=CARTESIAN_POINT('Ctrl Pts',(-61.8013048287075,-101.517470471821,
175.985485236451));
#31256=CARTESIAN_POINT('Ctrl Pts',(-61.7913666968533,-101.424248714515,
177.642339485944));
#31257=CARTESIAN_POINT('Ctrl Pts',(-60.6164569494197,-101.455220714482,
178.813912312176));
#31258=CARTESIAN_POINT('Ctrl Pts',(-59.4415472019861,-101.486192714449,
179.985485138407));
#31259=CARTESIAN_POINT('Ctrl Pts',(-57.7840904519822,-101.568607448735,
179.985485069079));
#31260=CARTESIAN_POINT('Ctrl Pts',(-56.1266337019783,-101.651022183021,
179.985484999752));
#31261=CARTESIAN_POINT('Ctrl Pts',(-54.9517240520365,-101.681994172595,
178.813912075476));
#31262=CARTESIAN_POINT('Ctrl Pts',(-53.7768144020947,-101.712966162168,
177.6423391512));
#31263=CARTESIAN_POINT('Ctrl Pts',(-53.7668764081149,-101.619744390164,
175.985484901707));
#31264=CARTESIAN_POINT('Ctrl Pts',(-53.756938414135,-101.526522618159,174.328630652215));
#31265=CARTESIAN_POINT('Ctrl Pts',(-54.9119720357346,-101.309107088882,
173.157057825983));
#31266=CARTESIAN_POINT('Ctrl Pts',(-56.0670056573342,-101.091691559604,
171.985484999752));
#31267=CARTESIAN_POINT('Ctrl Pts',(-57.7045862815041,-100.822833296007,
171.985485069079));
#31268=CARTESIAN_POINT('Ctrl Pts',(-59.342166905674,-100.55397503241,171.985485138407));
#31269=CARTESIAN_POINT('Ctrl Pts',(-60.4972004297817,-100.336559513526,
173.157058062683));
#31270=CARTESIAN_POINT('Ctrl Pts',(-61.6522339538895,-100.119143994642,
174.328630986959));
#31271=CARTESIAN_POINT('Ctrl Pts',(-61.6422958220353,-100.025922237336,
175.985485236451));
#31272=CARTESIAN_POINT('Ctrl Pts',(-61.6323576901811,-99.9327004800294,
177.642339485944));
#31273=CARTESIAN_POINT('Ctrl Pts',(-60.4574479427475,-99.9636724799962,
178.813912312176));
#31274=CARTESIAN_POINT('Ctrl Pts',(-59.2825381953138,-99.994644479963,179.985485138407));
#31275=CARTESIAN_POINT('Ctrl Pts',(-57.6250814453099,-100.077059214249,
179.985485069079));
#31276=CARTESIAN_POINT('Ctrl Pts',(-55.9676246953061,-100.159473948536,
179.985484999752));
#31277=CARTESIAN_POINT('Ctrl Pts',(-54.7927150453643,-100.190445938109,
178.813912075476));
#31278=CARTESIAN_POINT('Ctrl Pts',(-53.6178053954225,-100.221417927683,
177.6423391512));
#31279=CARTESIAN_POINT('Ctrl Pts',(-53.6078674014426,-100.128196155678,
175.985484901707));
#31280=CARTESIAN_POINT('Ctrl Pts',(-53.5979294074628,-100.034974383673,
174.328630652215));
#31281=CARTESIAN_POINT('Ctrl Pts',(-54.7529630290624,-99.817558854396,173.157057825983));
#31282=CARTESIAN_POINT('Ctrl Pts',(-55.907996650662,-99.6001433251185,171.985484999752));
#31283=CARTESIAN_POINT('Ctrl Pts',(-57.5455772748319,-99.3312850615215,
171.985485069079));
#31284=CARTESIAN_POINT('Ctrl Pts',(-59.1831578990017,-99.0624267979246,
171.985485138407));
#31285=CARTESIAN_POINT('Ctrl Pts',(-60.3381914231095,-98.8450112790404,
173.157058062683));
#31286=CARTESIAN_POINT('Ctrl Pts',(-61.4932249472172,-98.6275957601562,
174.328630986959));
#31287=CARTESIAN_POINT('Ctrl Pts',(-61.4832868153631,-98.53437400285,175.985485236451));
#31288=CARTESIAN_POINT('Ctrl Pts',(-61.4733486835089,-98.4411522455438,
177.642339485944));
#31289=CARTESIAN_POINT('Ctrl Pts',(-60.2984389360752,-98.4721242455106,
178.813912312176));
#31290=CARTESIAN_POINT('Ctrl Pts',(-59.1235291886416,-98.5030962454774,
179.985485138407));
#31291=CARTESIAN_POINT('Ctrl Pts',(-57.4660724386377,-98.5855109797636,
179.985485069079));
#31292=CARTESIAN_POINT('Ctrl Pts',(-55.8086156886338,-98.6679257140499,
179.985484999752));
#31293=CARTESIAN_POINT('Ctrl Pts',(-54.633706038692,-98.6988977036234,178.813912075476));
#31294=CARTESIAN_POINT('Ctrl Pts',(-56.8733667677527,-112.709647553905,
178.072094410988));
#31295=CARTESIAN_POINT('Ctrl Pts',(-56.0039967339745,-112.708046979118,
177.207792449865));
#31296=CARTESIAN_POINT('Ctrl Pts',(-55.9940587219143,-112.614825209041,
175.985484945604));
#31297=CARTESIAN_POINT('Ctrl Pts',(-55.9841207098542,-112.521603438964,
174.763177441344));
#31298=CARTESIAN_POINT('Ctrl Pts',(-56.8336146897208,-112.336760476773,
173.89887555255));
#31299=CARTESIAN_POINT('Ctrl Pts',(-57.6831086695875,-112.151917514582,
173.034573663757));
#31300=CARTESIAN_POINT('Ctrl Pts',(-58.8885910066563,-111.929123815193,
173.034573714903));
#31301=CARTESIAN_POINT('Ctrl Pts',(-60.0940733437252,-111.706330115804,
173.034573766048));
#31302=CARTESIAN_POINT('Ctrl Pts',(-60.9435672516694,-111.521487161281,
173.898875727171));
#31303=CARTESIAN_POINT('Ctrl Pts',(-61.7930611596136,-111.336644206758,
174.763177688294));
#31304=CARTESIAN_POINT('Ctrl Pts',(-61.7831230458397,-111.243422447524,
175.985485192554));
#31305=CARTESIAN_POINT('Ctrl Pts',(-61.7731849320658,-111.15020068829,177.207792696815));
#31306=CARTESIAN_POINT('Ctrl Pts',(-60.9038148263651,-111.14860012117,178.072094585608));
#31307=CARTESIAN_POINT('Ctrl Pts',(-60.0344447206644,-111.14699955405,178.936396474401));
#31308=CARTESIAN_POINT('Ctrl Pts',(-58.8090862577616,-111.183349724129,
178.936396423256));
#31309=CARTESIAN_POINT('Ctrl Pts',(-57.5837277948587,-111.219699894207,
178.936396372111));
#31310=CARTESIAN_POINT('Ctrl Pts',(-56.7143577610805,-111.21809931942,178.072094410988));
#31311=CARTESIAN_POINT('Ctrl Pts',(-55.8449877273022,-111.216498744632,
177.207792449865));
#31312=CARTESIAN_POINT('Ctrl Pts',(-55.8350497152421,-111.123276974555,
175.985484945604));
#31313=CARTESIAN_POINT('Ctrl Pts',(-55.8251117031819,-111.030055204478,
174.763177441344));
#31314=CARTESIAN_POINT('Ctrl Pts',(-56.6746056830486,-110.845212242287,
173.89887555255));
#31315=CARTESIAN_POINT('Ctrl Pts',(-57.5240996629153,-110.660369280097,
173.034573663757));
#31316=CARTESIAN_POINT('Ctrl Pts',(-58.7295819999841,-110.437575580708,
173.034573714903));
#31317=CARTESIAN_POINT('Ctrl Pts',(-59.9350643370529,-110.214781881319,
173.034573766048));
#31318=CARTESIAN_POINT('Ctrl Pts',(-60.7845582449971,-110.029938926795,
173.898875727171));
#31319=CARTESIAN_POINT('Ctrl Pts',(-61.6340521529414,-109.845095972272,
174.763177688294));
#31320=CARTESIAN_POINT('Ctrl Pts',(-61.6241140391675,-109.751874213038,
175.985485192554));
#31321=CARTESIAN_POINT('Ctrl Pts',(-61.6141759253936,-109.658652453805,
177.207792696815));
#31322=CARTESIAN_POINT('Ctrl Pts',(-60.7448058196929,-109.657051886685,
178.072094585608));
#31323=CARTESIAN_POINT('Ctrl Pts',(-59.8754357139922,-109.655451319565,
178.936396474401));
#31324=CARTESIAN_POINT('Ctrl Pts',(-58.6500772510893,-109.691801489643,
178.936396423256));
#31325=CARTESIAN_POINT('Ctrl Pts',(-57.4247187881865,-109.728151659721,
178.936396372111));
#31326=CARTESIAN_POINT('Ctrl Pts',(-56.5553487544082,-109.726551084934,
178.072094410988));
#31327=CARTESIAN_POINT('Ctrl Pts',(-55.68597872063,-109.724950510147,177.207792449865));
#31328=CARTESIAN_POINT('Ctrl Pts',(-55.6760407085698,-109.63172874007,175.985484945604));
#31329=CARTESIAN_POINT('Ctrl Pts',(-55.6661026965097,-109.538506969993,
174.763177441344));
#31330=CARTESIAN_POINT('Ctrl Pts',(-56.5155966763764,-109.353664007802,
173.89887555255));
#31331=CARTESIAN_POINT('Ctrl Pts',(-57.365090656243,-109.168821045611,173.034573663757));
#31332=CARTESIAN_POINT('Ctrl Pts',(-58.5705729933119,-108.946027346222,
173.034573714903));
#31333=CARTESIAN_POINT('Ctrl Pts',(-59.7760553303807,-108.723233646833,
173.034573766048));
#31334=CARTESIAN_POINT('Ctrl Pts',(-60.6255492383249,-108.53839069231,173.898875727171));
#31335=CARTESIAN_POINT('Ctrl Pts',(-61.4750431462691,-108.353547737786,
174.763177688294));
#31336=CARTESIAN_POINT('Ctrl Pts',(-61.4651050324952,-108.260325978553,
175.985485192554));
#31337=CARTESIAN_POINT('Ctrl Pts',(-61.4551669187214,-108.167104219319,
177.207792696815));
#31338=CARTESIAN_POINT('Ctrl Pts',(-60.5857968130207,-108.165503652199,
178.072094585608));
#31339=CARTESIAN_POINT('Ctrl Pts',(-59.71642670732,-108.163903085079,178.936396474401));
#31340=CARTESIAN_POINT('Ctrl Pts',(-58.4910682444171,-108.200253255158,
178.936396423256));
#31341=CARTESIAN_POINT('Ctrl Pts',(-57.2657097815143,-108.236603425236,
178.936396372111));
#31342=CARTESIAN_POINT('Ctrl Pts',(-56.396339747736,-108.235002850448,178.072094410988));
#31343=CARTESIAN_POINT('Ctrl Pts',(-55.5269697139578,-108.233402275661,
177.207792449865));
#31344=CARTESIAN_POINT('Ctrl Pts',(-55.5170317018976,-108.140180505584,
175.985484945604));
#31345=CARTESIAN_POINT('Ctrl Pts',(-55.5070936898375,-108.046958735507,
174.763177441344));
#31346=CARTESIAN_POINT('Ctrl Pts',(-56.3565876697041,-107.862115773316,
173.89887555255));
#31347=CARTESIAN_POINT('Ctrl Pts',(-57.2060816495708,-107.677272811126,
173.034573663757));
#31348=CARTESIAN_POINT('Ctrl Pts',(-58.4115639866396,-107.454479111736,
173.034573714903));
#31349=CARTESIAN_POINT('Ctrl Pts',(-59.6170463237085,-107.231685412347,
173.034573766048));
#31350=CARTESIAN_POINT('Ctrl Pts',(-60.4665402316527,-107.046842457824,
173.898875727171));
#31351=CARTESIAN_POINT('Ctrl Pts',(-61.3160341395969,-106.861999503301,
174.763177688294));
#31352=CARTESIAN_POINT('Ctrl Pts',(-61.306096025823,-106.768777744067,175.985485192554));
#31353=CARTESIAN_POINT('Ctrl Pts',(-61.2961579120492,-106.675555984834,
177.207792696815));
#31354=CARTESIAN_POINT('Ctrl Pts',(-60.4267878063484,-106.673955417714,
178.072094585608));
#31355=CARTESIAN_POINT('Ctrl Pts',(-59.5574177006478,-106.672354850594,
178.936396474401));
#31356=CARTESIAN_POINT('Ctrl Pts',(-58.3320592377449,-106.708705020672,
178.936396423256));
#31357=CARTESIAN_POINT('Ctrl Pts',(-57.106700774842,-106.74505519075,178.936396372111));
#31358=CARTESIAN_POINT('Ctrl Pts',(-56.2373307410638,-106.743454615963,
178.072094410988));
#31359=CARTESIAN_POINT('Ctrl Pts',(-55.3679607072856,-106.741854041175,
177.207792449865));
#31360=CARTESIAN_POINT('Ctrl Pts',(-55.3580226952254,-106.648632271098,
175.985484945604));
#31361=CARTESIAN_POINT('Ctrl Pts',(-55.3480846831652,-106.555410501021,
174.763177441344));
#31362=CARTESIAN_POINT('Ctrl Pts',(-56.1975786630319,-106.370567538831,
173.89887555255));
#31363=CARTESIAN_POINT('Ctrl Pts',(-57.0470726428986,-106.18572457664,173.034573663757));
#31364=CARTESIAN_POINT('Ctrl Pts',(-58.2525549799674,-105.962930877251,
173.034573714903));
#31365=CARTESIAN_POINT('Ctrl Pts',(-59.4580373170363,-105.740137177862,
173.034573766048));
#31366=CARTESIAN_POINT('Ctrl Pts',(-60.3075312249805,-105.555294223339,
173.898875727171));
#31367=CARTESIAN_POINT('Ctrl Pts',(-61.1570251329247,-105.370451268815,
174.763177688294));
#31368=CARTESIAN_POINT('Ctrl Pts',(-61.1470870191508,-105.277229509582,
175.985485192554));
#31369=CARTESIAN_POINT('Ctrl Pts',(-61.1371489053769,-105.184007750348,
177.207792696815));
#31370=CARTESIAN_POINT('Ctrl Pts',(-60.2677787996762,-105.182407183228,
178.072094585608));
#31371=CARTESIAN_POINT('Ctrl Pts',(-59.3984086939755,-105.180806616108,
178.936396474401));
#31372=CARTESIAN_POINT('Ctrl Pts',(-58.1730502310727,-105.217156786186,
178.936396423256));
#31373=CARTESIAN_POINT('Ctrl Pts',(-56.9476917681698,-105.253506956265,
178.936396372111));
#31374=CARTESIAN_POINT('Ctrl Pts',(-56.0783217343916,-105.251906381477,
178.072094410988));
#31375=CARTESIAN_POINT('Ctrl Pts',(-55.2089517006133,-105.25030580669,177.207792449865));
#31376=CARTESIAN_POINT('Ctrl Pts',(-55.1990136885532,-105.157084036613,
175.985484945604));
#31377=CARTESIAN_POINT('Ctrl Pts',(-55.189075676493,-105.063862266536,174.763177441344));
#31378=CARTESIAN_POINT('Ctrl Pts',(-56.0385696563597,-104.879019304345,
173.89887555255));
#31379=CARTESIAN_POINT('Ctrl Pts',(-56.8880636362264,-104.694176342154,
173.034573663757));
#31380=CARTESIAN_POINT('Ctrl Pts',(-58.0935459732952,-104.471382642765,
173.034573714903));
#31381=CARTESIAN_POINT('Ctrl Pts',(-59.299028310364,-104.248588943376,173.034573766048));
#31382=CARTESIAN_POINT('Ctrl Pts',(-60.1485222183082,-104.063745988853,
173.898875727171));
#31383=CARTESIAN_POINT('Ctrl Pts',(-60.9980161262524,-103.87890303433,174.763177688294));
#31384=CARTESIAN_POINT('Ctrl Pts',(-60.9880780124786,-103.785681275096,
175.985485192554));
#31385=CARTESIAN_POINT('Ctrl Pts',(-60.9781398987047,-103.692459515862,
177.207792696815));
#31386=CARTESIAN_POINT('Ctrl Pts',(-60.108769793004,-103.690858948742,178.072094585608));
#31387=CARTESIAN_POINT('Ctrl Pts',(-59.2393996873033,-103.689258381622,
178.936396474401));
#31388=CARTESIAN_POINT('Ctrl Pts',(-58.0140412244004,-103.725608551701,
178.936396423256));
#31389=CARTESIAN_POINT('Ctrl Pts',(-56.7886827614976,-103.761958721779,
178.936396372111));
#31390=CARTESIAN_POINT('Ctrl Pts',(-55.9193127277193,-103.760358146992,
178.072094410988));
#31391=CARTESIAN_POINT('Ctrl Pts',(-55.0499426939411,-103.758757572204,
177.207792449865));
#31392=CARTESIAN_POINT('Ctrl Pts',(-55.0400046818809,-103.665535802127,
175.985484945604));
#31393=CARTESIAN_POINT('Ctrl Pts',(-55.0300666698208,-103.57231403205,174.763177441344));
#31394=CARTESIAN_POINT('Ctrl Pts',(-55.8795606496874,-103.387471069859,
173.89887555255));
#31395=CARTESIAN_POINT('Ctrl Pts',(-56.7290546295541,-103.202628107669,
173.034573663757));
#31396=CARTESIAN_POINT('Ctrl Pts',(-57.934536966623,-102.97983440828,173.034573714903));
#31397=CARTESIAN_POINT('Ctrl Pts',(-59.1400193036918,-102.757040708891,
173.034573766048));
#31398=CARTESIAN_POINT('Ctrl Pts',(-59.989513211636,-102.572197754367,173.898875727171));
#31399=CARTESIAN_POINT('Ctrl Pts',(-60.8390071195802,-102.387354799844,
174.763177688294));
#31400=CARTESIAN_POINT('Ctrl Pts',(-60.8290690058063,-102.29413304061,175.985485192554));
#31401=CARTESIAN_POINT('Ctrl Pts',(-60.8191308920325,-102.200911281377,
177.207792696815));
#31402=CARTESIAN_POINT('Ctrl Pts',(-59.9497607863318,-102.199310714257,
178.072094585608));
#31403=CARTESIAN_POINT('Ctrl Pts',(-59.0803906806311,-102.197710147137,
178.936396474401));
#31404=CARTESIAN_POINT('Ctrl Pts',(-57.8550322177282,-102.234060317215,
178.936396423256));
#31405=CARTESIAN_POINT('Ctrl Pts',(-56.6296737548253,-102.270410487293,
178.936396372111));
#31406=CARTESIAN_POINT('Ctrl Pts',(-55.7603037210471,-102.268809912506,
178.072094410988));
#31407=CARTESIAN_POINT('Ctrl Pts',(-54.8909336872689,-102.267209337719,
177.207792449865));
#31408=CARTESIAN_POINT('Ctrl Pts',(-54.8809956752087,-102.173987567642,
175.985484945604));
#31409=CARTESIAN_POINT('Ctrl Pts',(-54.8710576631486,-102.080765797565,
174.763177441344));
#31410=CARTESIAN_POINT('Ctrl Pts',(-55.7205516430152,-101.895922835374,
173.89887555255));
#31411=CARTESIAN_POINT('Ctrl Pts',(-56.5700456228819,-101.711079873183,
173.034573663757));
#31412=CARTESIAN_POINT('Ctrl Pts',(-57.7755279599507,-101.488286173794,
173.034573714903));
#31413=CARTESIAN_POINT('Ctrl Pts',(-58.9810102970196,-101.265492474405,
173.034573766048));
#31414=CARTESIAN_POINT('Ctrl Pts',(-59.8305042049638,-101.080649519882,
173.898875727171));
#31415=CARTESIAN_POINT('Ctrl Pts',(-60.679998112908,-100.895806565358,174.763177688294));
#31416=CARTESIAN_POINT('Ctrl Pts',(-60.6700599991341,-100.802584806125,
175.985485192554));
#31417=CARTESIAN_POINT('Ctrl Pts',(-60.6601218853602,-100.709363046891,
177.207792696815));
#31418=CARTESIAN_POINT('Ctrl Pts',(-59.7907517796595,-100.707762479771,
178.072094585608));
#31419=CARTESIAN_POINT('Ctrl Pts',(-58.9213816739588,-100.706161912651,
178.936396474401));
#31420=CARTESIAN_POINT('Ctrl Pts',(-57.696023211056,-100.742512082729,178.936396423256));
#31421=CARTESIAN_POINT('Ctrl Pts',(-56.4706647481531,-100.778862252808,
178.936396372111));
#31422=CARTESIAN_POINT('Ctrl Pts',(-55.6012947143749,-100.77726167802,178.072094410988));
#31423=CARTESIAN_POINT('Ctrl Pts',(-54.7319246805966,-100.775661103233,
177.207792449865));
#31424=CARTESIAN_POINT('Ctrl Pts',(-54.7219866685365,-100.682439333156,
175.985484945604));
#31425=CARTESIAN_POINT('Ctrl Pts',(-54.7120486564763,-100.589217563079,
174.763177441344));
#31426=CARTESIAN_POINT('Ctrl Pts',(-55.561542636343,-100.404374600888,173.89887555255));
#31427=CARTESIAN_POINT('Ctrl Pts',(-56.4110366162097,-100.219531638698,
173.034573663757));
#31428=CARTESIAN_POINT('Ctrl Pts',(-57.6165189532785,-99.9967379393085,
173.034573714903));
#31429=CARTESIAN_POINT('Ctrl Pts',(-58.8220012903473,-99.7739442399195,
173.034573766048));
#31430=CARTESIAN_POINT('Ctrl Pts',(-59.6714951982915,-99.5891012853962,
173.898875727171));
#31431=CARTESIAN_POINT('Ctrl Pts',(-60.5209891062358,-99.4042583308729,
174.763177688294));
#31432=CARTESIAN_POINT('Ctrl Pts',(-60.5110509924619,-99.3110365716392,
175.985485192554));
#31433=CARTESIAN_POINT('Ctrl Pts',(-60.501112878688,-99.2178148124055,177.207792696815));
#31434=CARTESIAN_POINT('Ctrl Pts',(-59.6317427729873,-99.2162142452855,
178.072094585608));
#31435=CARTESIAN_POINT('Ctrl Pts',(-58.7623726672866,-99.2146136781656,
178.936396474401));
#31436=CARTESIAN_POINT('Ctrl Pts',(-57.5370142043838,-99.2509638482439,
178.936396423256));
#31437=CARTESIAN_POINT('Ctrl Pts',(-56.3116557414809,-99.2873140183222,
178.936396372111));
#31438=CARTESIAN_POINT('Ctrl Pts',(-55.4422857077027,-99.2857134435348,
178.072094410988));
#31439=CARTESIAN_POINT('Ctrl Pts',(-54.5729156739244,-99.2841128687474,
177.207792449865));
#31440=CARTESIAN_POINT('Ctrl Pts',(-54.5629776618643,-99.1908910986704,
175.985484945604));
#31441=CARTESIAN_POINT('Ctrl Pts',(-54.5530396498041,-99.0976693285933,
174.763177441344));
#31442=CARTESIAN_POINT('Ctrl Pts',(-55.4025336296708,-98.9128263664026,
173.89887555255));
#31443=CARTESIAN_POINT('Ctrl Pts',(-56.2520276095374,-98.727983404212,173.034573663757));
#31444=CARTESIAN_POINT('Ctrl Pts',(-57.4575099466063,-98.5051897048229,
173.034573714903));
#31445=CARTESIAN_POINT('Ctrl Pts',(-58.6629922836751,-98.2823960054338,
173.034573766048));
#31446=CARTESIAN_POINT('Ctrl Pts',(-59.5124861916193,-98.0975530509106,
173.898875727171));
#31447=CARTESIAN_POINT('Ctrl Pts',(-60.3619800995635,-97.9127100963873,
174.763177688294));
#31448=CARTESIAN_POINT('Ctrl Pts',(-60.3520419857897,-97.8194883371536,
175.985485192554));
#31449=CARTESIAN_POINT('Ctrl Pts',(-60.3421038720158,-97.7262665779199,
177.207792696815));
#31450=CARTESIAN_POINT('Ctrl Pts',(-59.4727337663151,-97.7246660108,178.072094585608));
#31451=CARTESIAN_POINT('Ctrl Pts',(-58.6033636606144,-97.72306544368,178.936396474401));
#31452=CARTESIAN_POINT('Ctrl Pts',(-57.3780051977115,-97.7594156137583,
178.936396423256));
#31453=CARTESIAN_POINT('Ctrl Pts',(-56.1526467348087,-97.7957657838366,
178.936396372111));
#31454=CARTESIAN_POINT('Ctrl Pts',(-55.2832767010304,-97.7941652090492,
178.072094410988));
#31455=CARTESIAN_POINT('Ctrl Pts',(-56.1707879621501,-113.117200285871,
178.813917503681));
#31456=CARTESIAN_POINT('Ctrl Pts',(-54.9958760764408,-113.148172513793,
177.642342330969));
#31457=CARTESIAN_POINT('Ctrl Pts',(-54.9859380824611,-113.054950741788,
175.985484901707));
#31458=CARTESIAN_POINT('Ctrl Pts',(-54.9760000884813,-112.961728969784,
174.328627472445));
#31459=CARTESIAN_POINT('Ctrl Pts',(-56.1310359458487,-112.744313202158,
173.157052397777));
#31460=CARTESIAN_POINT('Ctrl Pts',(-57.2860718032161,-112.526897434533,
171.985477323109));
#31461=CARTESIAN_POINT('Ctrl Pts',(-58.9236555892389,-112.258038833861,
171.985477392437));
#31462=CARTESIAN_POINT('Ctrl Pts',(-60.5612393752617,-111.98918023319,171.985477461765));
#31463=CARTESIAN_POINT('Ctrl Pts',(-61.7162751351371,-111.771764475958,
173.157052634477));
#31464=CARTESIAN_POINT('Ctrl Pts',(-62.8713108950124,-111.554348718726,
174.32862780719));
#31465=CARTESIAN_POINT('Ctrl Pts',(-62.8613727631581,-111.46112696142,175.985485236452));
#31466=CARTESIAN_POINT('Ctrl Pts',(-62.8514346313038,-111.367905204114,
177.642342665714));
#31467=CARTESIAN_POINT('Ctrl Pts',(-61.6765226481024,-111.398877442428,
178.813917740382));
#31468=CARTESIAN_POINT('Ctrl Pts',(-60.501610664901,-111.429849680743,179.98549281505));
#31469=CARTESIAN_POINT('Ctrl Pts',(-58.8441507530441,-111.512264752104,
179.985492745722));
#31470=CARTESIAN_POINT('Ctrl Pts',(-57.1866908411873,-111.594679823465,
179.985492676394));
#31471=CARTESIAN_POINT('Ctrl Pts',(-56.0117789554779,-111.625652051386,
178.813917503681));
#31472=CARTESIAN_POINT('Ctrl Pts',(-54.8368670697686,-111.656624279307,
177.642342330969));
#31473=CARTESIAN_POINT('Ctrl Pts',(-54.8269290757888,-111.563402507303,
175.985484901707));
#31474=CARTESIAN_POINT('Ctrl Pts',(-54.8169910818091,-111.470180735298,
174.328627472445));
#31475=CARTESIAN_POINT('Ctrl Pts',(-55.9720269391765,-111.252764967673,
173.157052397777));
#31476=CARTESIAN_POINT('Ctrl Pts',(-57.1270627965439,-111.035349200047,
171.985477323109));
#31477=CARTESIAN_POINT('Ctrl Pts',(-58.7646465825667,-110.766490599376,
171.985477392437));
#31478=CARTESIAN_POINT('Ctrl Pts',(-60.4022303685895,-110.497631998704,
171.985477461765));
#31479=CARTESIAN_POINT('Ctrl Pts',(-61.5572661284649,-110.280216241472,
173.157052634477));
#31480=CARTESIAN_POINT('Ctrl Pts',(-62.7123018883402,-110.06280048424,174.32862780719));
#31481=CARTESIAN_POINT('Ctrl Pts',(-62.7023637564859,-109.969578726934,
175.985485236452));
#31482=CARTESIAN_POINT('Ctrl Pts',(-62.6924256246316,-109.876356969628,
177.642342665714));
#31483=CARTESIAN_POINT('Ctrl Pts',(-61.5175136414302,-109.907329207943,
178.813917740382));
#31484=CARTESIAN_POINT('Ctrl Pts',(-60.3426016582288,-109.938301446257,
179.98549281505));
#31485=CARTESIAN_POINT('Ctrl Pts',(-58.6851417463719,-110.020716517618,
179.985492745722));
#31486=CARTESIAN_POINT('Ctrl Pts',(-57.0276818345151,-110.103131588979,
179.985492676394));
#31487=CARTESIAN_POINT('Ctrl Pts',(-55.8527699488057,-110.1341038169,178.813917503681));
#31488=CARTESIAN_POINT('Ctrl Pts',(-54.6778580630964,-110.165076044821,
177.642342330969));
#31489=CARTESIAN_POINT('Ctrl Pts',(-54.6679200691166,-110.071854272817,
175.985484901707));
#31490=CARTESIAN_POINT('Ctrl Pts',(-54.6579820751369,-109.978632500812,
174.328627472445));
#31491=CARTESIAN_POINT('Ctrl Pts',(-55.8130179325043,-109.761216733187,
173.157052397777));
#31492=CARTESIAN_POINT('Ctrl Pts',(-56.9680537898716,-109.543800965562,
171.985477323109));
#31493=CARTESIAN_POINT('Ctrl Pts',(-58.6056375758945,-109.27494236489,171.985477392437));
#31494=CARTESIAN_POINT('Ctrl Pts',(-60.2432213619173,-109.006083764219,
171.985477461765));
#31495=CARTESIAN_POINT('Ctrl Pts',(-61.3982571217926,-108.788668006987,
173.157052634477));
#31496=CARTESIAN_POINT('Ctrl Pts',(-62.553292881668,-108.571252249755,174.32862780719));
#31497=CARTESIAN_POINT('Ctrl Pts',(-62.5433547498136,-108.478030492449,
175.985485236452));
#31498=CARTESIAN_POINT('Ctrl Pts',(-62.5334166179593,-108.384808735142,
177.642342665714));
#31499=CARTESIAN_POINT('Ctrl Pts',(-61.3585046347579,-108.415780973457,
178.813917740382));
#31500=CARTESIAN_POINT('Ctrl Pts',(-60.1835926515565,-108.446753211771,
179.98549281505));
#31501=CARTESIAN_POINT('Ctrl Pts',(-58.5261327396997,-108.529168283132,
179.985492745722));
#31502=CARTESIAN_POINT('Ctrl Pts',(-56.8686728278428,-108.611583354493,
179.985492676394));
#31503=CARTESIAN_POINT('Ctrl Pts',(-55.6937609421335,-108.642555582415,
178.813917503681));
#31504=CARTESIAN_POINT('Ctrl Pts',(-54.5188490564241,-108.673527810336,
177.642342330969));
#31505=CARTESIAN_POINT('Ctrl Pts',(-54.5089110624444,-108.580306038331,
175.985484901707));
#31506=CARTESIAN_POINT('Ctrl Pts',(-54.4989730684647,-108.487084266327,
174.328627472445));
#31507=CARTESIAN_POINT('Ctrl Pts',(-55.654008925832,-108.269668498702,173.157052397777));
#31508=CARTESIAN_POINT('Ctrl Pts',(-56.8090447831994,-108.052252731076,
171.985477323109));
#31509=CARTESIAN_POINT('Ctrl Pts',(-58.4466285692222,-107.783394130405,
171.985477392437));
#31510=CARTESIAN_POINT('Ctrl Pts',(-60.0842123552451,-107.514535529733,
171.985477461765));
#31511=CARTESIAN_POINT('Ctrl Pts',(-61.2392481151204,-107.297119772501,
173.157052634477));
#31512=CARTESIAN_POINT('Ctrl Pts',(-62.3942838749957,-107.079704015269,
174.32862780719));
#31513=CARTESIAN_POINT('Ctrl Pts',(-62.3843457431414,-106.986482257963,
175.985485236452));
#31514=CARTESIAN_POINT('Ctrl Pts',(-62.3744076112871,-106.893260500657,
177.642342665714));
#31515=CARTESIAN_POINT('Ctrl Pts',(-61.1994956280857,-106.924232738971,
178.813917740382));
#31516=CARTESIAN_POINT('Ctrl Pts',(-60.0245836448843,-106.955204977286,
179.98549281505));
#31517=CARTESIAN_POINT('Ctrl Pts',(-58.3671237330274,-107.037620048647,
179.985492745722));
#31518=CARTESIAN_POINT('Ctrl Pts',(-56.7096638211706,-107.120035120008,
179.985492676394));
#31519=CARTESIAN_POINT('Ctrl Pts',(-55.5347519354612,-107.151007347929,
178.813917503681));
#31520=CARTESIAN_POINT('Ctrl Pts',(-54.3598400497519,-107.18197957585,177.642342330969));
#31521=CARTESIAN_POINT('Ctrl Pts',(-54.3499020557721,-107.088757803846,
175.985484901707));
#31522=CARTESIAN_POINT('Ctrl Pts',(-54.3399640617924,-106.995536031841,
174.328627472445));
#31523=CARTESIAN_POINT('Ctrl Pts',(-55.4949999191598,-106.778120264216,
173.157052397777));
#31524=CARTESIAN_POINT('Ctrl Pts',(-56.6500357765272,-106.560704496591,
171.985477323109));
#31525=CARTESIAN_POINT('Ctrl Pts',(-58.28761956255,-106.291845895919,171.985477392437));
#31526=CARTESIAN_POINT('Ctrl Pts',(-59.9252033485729,-106.022987295247,
171.985477461765));
#31527=CARTESIAN_POINT('Ctrl Pts',(-61.0802391084482,-105.805571538015,
173.157052634477));
#31528=CARTESIAN_POINT('Ctrl Pts',(-62.2352748683235,-105.588155780784,
174.32862780719));
#31529=CARTESIAN_POINT('Ctrl Pts',(-62.2253367364692,-105.494934023477,
175.985485236452));
#31530=CARTESIAN_POINT('Ctrl Pts',(-62.2153986046149,-105.401712266171,
177.642342665714));
#31531=CARTESIAN_POINT('Ctrl Pts',(-61.0404866214135,-105.432684504486,
178.813917740382));
#31532=CARTESIAN_POINT('Ctrl Pts',(-59.8655746382121,-105.4636567428,179.98549281505));
#31533=CARTESIAN_POINT('Ctrl Pts',(-58.2081147263552,-105.546071814161,
179.985492745722));
#31534=CARTESIAN_POINT('Ctrl Pts',(-56.5506548144984,-105.628486885522,
179.985492676394));
#31535=CARTESIAN_POINT('Ctrl Pts',(-55.375742928789,-105.659459113443,178.813917503681));
#31536=CARTESIAN_POINT('Ctrl Pts',(-54.2008310430796,-105.690431341365,
177.642342330969));
#31537=CARTESIAN_POINT('Ctrl Pts',(-54.1908930490999,-105.59720956936,175.985484901707));
#31538=CARTESIAN_POINT('Ctrl Pts',(-54.1809550551202,-105.503987797356,
174.328627472445));
#31539=CARTESIAN_POINT('Ctrl Pts',(-55.3359909124876,-105.28657202973,173.157052397777));
#31540=CARTESIAN_POINT('Ctrl Pts',(-56.491026769855,-105.069156262105,171.985477323109));
#31541=CARTESIAN_POINT('Ctrl Pts',(-58.1286105558778,-104.800297661433,
171.985477392437));
#31542=CARTESIAN_POINT('Ctrl Pts',(-59.7661943419006,-104.531439060762,
171.985477461765));
#31543=CARTESIAN_POINT('Ctrl Pts',(-60.9212301017759,-104.31402330353,173.157052634477));
#31544=CARTESIAN_POINT('Ctrl Pts',(-62.0762658616513,-104.096607546298,
174.32862780719));
#31545=CARTESIAN_POINT('Ctrl Pts',(-62.066327729797,-104.003385788992,175.985485236452));
#31546=CARTESIAN_POINT('Ctrl Pts',(-62.0563895979427,-103.910164031686,
177.642342665714));
#31547=CARTESIAN_POINT('Ctrl Pts',(-60.8814776147413,-103.94113627,178.813917740382));
#31548=CARTESIAN_POINT('Ctrl Pts',(-59.7065656315398,-103.972108508315,
179.98549281505));
#31549=CARTESIAN_POINT('Ctrl Pts',(-58.049105719683,-104.054523579676,179.985492745722));
#31550=CARTESIAN_POINT('Ctrl Pts',(-56.3916458078261,-104.136938651037,
179.985492676394));
#31551=CARTESIAN_POINT('Ctrl Pts',(-55.2167339221168,-104.167910878958,
178.813917503681));
#31552=CARTESIAN_POINT('Ctrl Pts',(-54.0418220364074,-104.198883106879,
177.642342330969));
#31553=CARTESIAN_POINT('Ctrl Pts',(-54.0318840424277,-104.105661334875,
175.985484901707));
#31554=CARTESIAN_POINT('Ctrl Pts',(-54.021946048448,-104.01243956287,174.328627472445));
#31555=CARTESIAN_POINT('Ctrl Pts',(-55.1769819058153,-103.795023795245,
173.157052397777));
#31556=CARTESIAN_POINT('Ctrl Pts',(-56.3320177631827,-103.577608027619,
171.985477323109));
#31557=CARTESIAN_POINT('Ctrl Pts',(-57.9696015492056,-103.308749426948,
171.985477392437));
#31558=CARTESIAN_POINT('Ctrl Pts',(-59.6071853352284,-103.039890826276,
171.985477461765));
#31559=CARTESIAN_POINT('Ctrl Pts',(-60.7622210951037,-102.822475069044,
173.157052634477));
#31560=CARTESIAN_POINT('Ctrl Pts',(-61.9172568549791,-102.605059311812,
174.32862780719));
#31561=CARTESIAN_POINT('Ctrl Pts',(-61.9073187231247,-102.511837554506,
175.985485236452));
#31562=CARTESIAN_POINT('Ctrl Pts',(-61.8973805912704,-102.4186157972,177.642342665714));
#31563=CARTESIAN_POINT('Ctrl Pts',(-60.722468608069,-102.449588035515,178.813917740382));
#31564=CARTESIAN_POINT('Ctrl Pts',(-59.5475566248676,-102.480560273829,
179.98549281505));
#31565=CARTESIAN_POINT('Ctrl Pts',(-57.8900967130108,-102.56297534519,179.985492745722));
#31566=CARTESIAN_POINT('Ctrl Pts',(-56.2326368011539,-102.645390416551,
179.985492676394));
#31567=CARTESIAN_POINT('Ctrl Pts',(-55.0577249154445,-102.676362644472,
178.813917503681));
#31568=CARTESIAN_POINT('Ctrl Pts',(-53.8828130297352,-102.707334872393,
177.642342330969));
#31569=CARTESIAN_POINT('Ctrl Pts',(-53.8728750357555,-102.614113100389,
175.985484901707));
#31570=CARTESIAN_POINT('Ctrl Pts',(-53.8629370417758,-102.520891328384,
174.328627472445));
#31571=CARTESIAN_POINT('Ctrl Pts',(-55.0179728991431,-102.303475560759,
173.157052397777));
#31572=CARTESIAN_POINT('Ctrl Pts',(-56.1730087565105,-102.086059793134,
171.985477323109));
#31573=CARTESIAN_POINT('Ctrl Pts',(-57.8105925425333,-101.817201192462,
171.985477392437));
#31574=CARTESIAN_POINT('Ctrl Pts',(-59.4481763285562,-101.548342591791,
171.985477461765));
#31575=CARTESIAN_POINT('Ctrl Pts',(-60.6032120884315,-101.330926834559,
173.157052634477));
#31576=CARTESIAN_POINT('Ctrl Pts',(-61.7582478483068,-101.113511077327,
174.32862780719));
#31577=CARTESIAN_POINT('Ctrl Pts',(-61.7483097164525,-101.020289320021,
175.985485236452));
#31578=CARTESIAN_POINT('Ctrl Pts',(-61.7383715845982,-100.927067562714,
177.642342665714));
#31579=CARTESIAN_POINT('Ctrl Pts',(-60.5634596013968,-100.958039801029,
178.813917740382));
#31580=CARTESIAN_POINT('Ctrl Pts',(-59.3885476181954,-100.989012039343,
179.98549281505));
#31581=CARTESIAN_POINT('Ctrl Pts',(-57.7310877063385,-101.071427110704,
179.985492745722));
#31582=CARTESIAN_POINT('Ctrl Pts',(-56.0736277944817,-101.153842182065,
179.985492676394));
#31583=CARTESIAN_POINT('Ctrl Pts',(-54.8987159087723,-101.184814409987,
178.813917503681));
#31584=CARTESIAN_POINT('Ctrl Pts',(-53.723804023063,-101.215786637908,177.642342330969));
#31585=CARTESIAN_POINT('Ctrl Pts',(-53.7138660290832,-101.122564865903,
175.985484901707));
#31586=CARTESIAN_POINT('Ctrl Pts',(-53.7039280351035,-101.029343093899,
174.328627472445));
#31587=CARTESIAN_POINT('Ctrl Pts',(-54.8589638924709,-100.811927326274,
173.157052397777));
#31588=CARTESIAN_POINT('Ctrl Pts',(-56.0139997498383,-100.594511558648,
171.985477323109));
#31589=CARTESIAN_POINT('Ctrl Pts',(-57.6515835358611,-100.325652957977,
171.985477392437));
#31590=CARTESIAN_POINT('Ctrl Pts',(-59.2891673218839,-100.056794357305,
171.985477461765));
#31591=CARTESIAN_POINT('Ctrl Pts',(-60.4442030817593,-99.8393786000731,
173.157052634477));
#31592=CARTESIAN_POINT('Ctrl Pts',(-61.5992388416346,-99.6219628428411,
174.32862780719));
#31593=CARTESIAN_POINT('Ctrl Pts',(-61.5893007097803,-99.5287410855349,
175.985485236452));
#31594=CARTESIAN_POINT('Ctrl Pts',(-61.579362577926,-99.4355193282287,177.642342665714));
#31595=CARTESIAN_POINT('Ctrl Pts',(-60.4044505947246,-99.4664915665433,
178.813917740382));
#31596=CARTESIAN_POINT('Ctrl Pts',(-59.2295386115232,-99.4974638048579,
179.98549281505));
#31597=CARTESIAN_POINT('Ctrl Pts',(-57.5720786996663,-99.5798788762188,
179.985492745722));
#31598=CARTESIAN_POINT('Ctrl Pts',(-55.9146187878095,-99.6622939475797,
179.985492676394));
#31599=CARTESIAN_POINT('Ctrl Pts',(-54.7397069021001,-99.693266175501,178.813917503681));
#31600=CARTESIAN_POINT('Ctrl Pts',(-53.5647950163907,-99.7242384034223,
177.642342330969));
#31601=CARTESIAN_POINT('Ctrl Pts',(-53.554857022411,-99.6310166314178,175.985484901707));
#31602=CARTESIAN_POINT('Ctrl Pts',(-53.5449190284313,-99.5377948594132,
174.328627472445));
#31603=CARTESIAN_POINT('Ctrl Pts',(-54.6999548857987,-99.3203790917879,
173.157052397777));
#31604=CARTESIAN_POINT('Ctrl Pts',(-55.854990743166,-99.1029633241627,171.985477323109));
#31605=CARTESIAN_POINT('Ctrl Pts',(-57.4925745291889,-98.8341047234911,
171.985477392437));
#31606=CARTESIAN_POINT('Ctrl Pts',(-59.1301583152117,-98.5652461228194,
171.985477461765));
#31607=CARTESIAN_POINT('Ctrl Pts',(-60.285194075087,-98.3478303655875,173.157052634477));
#31608=CARTESIAN_POINT('Ctrl Pts',(-61.4402298349624,-98.1304146083555,
174.32862780719));
#31609=CARTESIAN_POINT('Ctrl Pts',(-61.430291703108,-98.0371928510493,175.985485236452));
#31610=CARTESIAN_POINT('Ctrl Pts',(-61.4203535712537,-97.9439710937432,
177.642342665714));
#31611=CARTESIAN_POINT('Ctrl Pts',(-60.2454415880523,-97.9749433320577,
178.813917740382));
#31612=CARTESIAN_POINT('Ctrl Pts',(-59.0705296048509,-98.0059155703723,
179.98549281505));
#31613=CARTESIAN_POINT('Ctrl Pts',(-57.4130696929941,-98.0883306417332,
179.985492745722));
#31614=CARTESIAN_POINT('Ctrl Pts',(-55.7556097811372,-98.1707457130942,
179.985492676394));
#31615=CARTESIAN_POINT('Ctrl Pts',(-54.5806978954278,-98.2017179410154,
178.813917503681));
#31616=CARTESIAN_POINT('Ctrl Pts',(-60.8888270505345,-111.922827698136,
172.515418850865));
#31617=CARTESIAN_POINT('Ctrl Pts',(-61.3449147819398,-111.841663883713,
172.780385782991));
#31618=CARTESIAN_POINT('Ctrl Pts',(-61.7162694809355,-111.771762644582,
173.157058062683));
#31619=CARTESIAN_POINT('Ctrl Pts',(-61.8701645018886,-111.74279451064,173.313156769748));
#31620=CARTESIAN_POINT('Ctrl Pts',(-62.0059837058594,-111.715257081458,
173.485485069079));
#31621=CARTESIAN_POINT('Ctrl Pts',(-56.1707931031902,-113.117197303651,
178.813912075476));
#31622=CARTESIAN_POINT('Ctrl Pts',(-54.9958834532485,-113.148169293224,
177.6423391512));
#31623=CARTESIAN_POINT('Ctrl Pts',(-54.9859454592686,-113.05494752122,175.985484901707));
#31624=CARTESIAN_POINT('Ctrl Pts',(-54.9760074652888,-112.961725749215,
174.328630652215));
#31625=CARTESIAN_POINT('Ctrl Pts',(-56.1310410868884,-112.744310219938,
173.157057825983));
#31626=CARTESIAN_POINT('Ctrl Pts',(-57.286074708488,-112.52689469066,171.985484999752));
#31627=CARTESIAN_POINT('Ctrl Pts',(-58.9236553326578,-112.258036427063,
171.985485069079));
#31628=CARTESIAN_POINT('Ctrl Pts',(-60.5612359568277,-111.989178163466,
171.985485138407));
#31629=CARTESIAN_POINT('Ctrl Pts',(-61.7162694809355,-111.771762644582,
173.157058062683));
#31630=CARTESIAN_POINT('Ctrl Pts',(-62.8713030050432,-111.554347125698,
174.328630986959));
#31631=CARTESIAN_POINT('Ctrl Pts',(-62.861364873189,-111.461125368392,175.985485236451));
#31632=CARTESIAN_POINT('Ctrl Pts',(-62.8514267413349,-111.367903611086,
177.642339485944));
#31633=CARTESIAN_POINT('Ctrl Pts',(-61.6765169939012,-111.398875611052,
178.813912312176));
#31634=CARTESIAN_POINT('Ctrl Pts',(-60.5016072464676,-111.429847611019,
179.985485138407));
#31635=CARTESIAN_POINT('Ctrl Pts',(-58.8441504964637,-111.512262345305,
179.985485069079));
#31636=CARTESIAN_POINT('Ctrl Pts',(-57.1866937464598,-111.594677079592,
179.985484999752));
#31637=CARTESIAN_POINT('Ctrl Pts',(-56.011784096518,-111.625649069165,178.813912075476));
#31638=CARTESIAN_POINT('Ctrl Pts',(-54.8368744465763,-111.656621058739,
177.6423391512));
#31639=CARTESIAN_POINT('Ctrl Pts',(-54.8269364525964,-111.563399286734,
175.985484901707));
#31640=CARTESIAN_POINT('Ctrl Pts',(-54.8169984586165,-111.47017751473,174.328630652215));
#31641=CARTESIAN_POINT('Ctrl Pts',(-55.9720320802161,-111.252761985452,
173.157057825983));
#31642=CARTESIAN_POINT('Ctrl Pts',(-57.1270657018158,-111.035346456175,
171.985484999752));
#31643=CARTESIAN_POINT('Ctrl Pts',(-58.7646463259856,-110.766488192578,
171.985485069079));
#31644=CARTESIAN_POINT('Ctrl Pts',(-60.4022269501555,-110.497629928981,
171.985485138407));
#31645=CARTESIAN_POINT('Ctrl Pts',(-61.5572604742632,-110.280214410097,
173.157058062683));
#31646=CARTESIAN_POINT('Ctrl Pts',(-62.712293998371,-110.062798891212,174.328630986959));
#31647=CARTESIAN_POINT('Ctrl Pts',(-62.7023558665168,-109.969577133906,
175.985485236451));
#31648=CARTESIAN_POINT('Ctrl Pts',(-62.6924177346626,-109.8763553766,177.642339485944));
#31649=CARTESIAN_POINT('Ctrl Pts',(-61.517507987229,-109.907327376567,178.813912312176));
#31650=CARTESIAN_POINT('Ctrl Pts',(-60.3425982397954,-109.938299376534,
179.985485138407));
#31651=CARTESIAN_POINT('Ctrl Pts',(-58.6851414897915,-110.02071411082,179.985485069079));
#31652=CARTESIAN_POINT('Ctrl Pts',(-57.0276847397876,-110.103128845106,
179.985484999752));
#31653=CARTESIAN_POINT('Ctrl Pts',(-55.8527750898458,-110.13410083468,178.813912075476));
#31654=CARTESIAN_POINT('Ctrl Pts',(-54.677865439904,-110.165072824253,177.6423391512));
#31655=CARTESIAN_POINT('Ctrl Pts',(-54.6679274459242,-110.071851052249,
175.985484901707));
#31656=CARTESIAN_POINT('Ctrl Pts',(-54.6579894519443,-109.978629280244,
174.328630652215));
#31657=CARTESIAN_POINT('Ctrl Pts',(-55.8130230735439,-109.761213750967,
173.157057825983));
#31658=CARTESIAN_POINT('Ctrl Pts',(-56.9680566951435,-109.543798221689,
171.985484999752));
#31659=CARTESIAN_POINT('Ctrl Pts',(-58.6056373193134,-109.274939958092,
171.985485069079));
#31660=CARTESIAN_POINT('Ctrl Pts',(-60.2432179434833,-109.006081694495,
171.985485138407));
#31661=CARTESIAN_POINT('Ctrl Pts',(-61.398251467591,-108.788666175611,173.157058062683));
#31662=CARTESIAN_POINT('Ctrl Pts',(-62.5532849916988,-108.571250656727,
174.328630986959));
#31663=CARTESIAN_POINT('Ctrl Pts',(-62.5433468598446,-108.478028899421,
175.985485236451));
#31664=CARTESIAN_POINT('Ctrl Pts',(-62.5334087279904,-108.384807142114,
177.642339485944));
#31665=CARTESIAN_POINT('Ctrl Pts',(-61.3584989805568,-108.415779142081,
178.813912312176));
#31666=CARTESIAN_POINT('Ctrl Pts',(-60.1835892331231,-108.446751142048,
179.985485138407));
#31667=CARTESIAN_POINT('Ctrl Pts',(-58.5261324831192,-108.529165876334,
179.985485069079));
#31668=CARTESIAN_POINT('Ctrl Pts',(-56.8686757331153,-108.611580610621,
179.985484999752));
#31669=CARTESIAN_POINT('Ctrl Pts',(-55.6937660831736,-108.642552600194,
178.813912075476));
#31670=CARTESIAN_POINT('Ctrl Pts',(-54.5188564332318,-108.673524589768,
177.6423391512));
#31671=CARTESIAN_POINT('Ctrl Pts',(-54.5089184392519,-108.580302817763,
175.985484901707));
#31672=CARTESIAN_POINT('Ctrl Pts',(-54.4989804452721,-108.487081045759,
174.328630652215));
#31673=CARTESIAN_POINT('Ctrl Pts',(-55.6540140668717,-108.269665516481,
173.157057825983));
#31674=CARTESIAN_POINT('Ctrl Pts',(-56.8090476884713,-108.052249987204,
171.985484999752));
#31675=CARTESIAN_POINT('Ctrl Pts',(-58.4466283126412,-107.783391723607,
171.985485069079));
#31676=CARTESIAN_POINT('Ctrl Pts',(-60.084208936811,-107.51453346001,171.985485138407));
#31677=CARTESIAN_POINT('Ctrl Pts',(-61.2392424609188,-107.297117941125,
173.157058062683));
#31678=CARTESIAN_POINT('Ctrl Pts',(-62.3942759850265,-107.079702422241,
174.328630986959));
#31679=CARTESIAN_POINT('Ctrl Pts',(-62.3843378531723,-106.986480664935,
175.985485236451));
#31680=CARTESIAN_POINT('Ctrl Pts',(-62.3743997213182,-106.893258907629,
177.642339485944));
#31681=CARTESIAN_POINT('Ctrl Pts',(-61.1994899738845,-106.924230907596,
178.813912312176));
#31682=CARTESIAN_POINT('Ctrl Pts',(-60.0245802264509,-106.955202907562,
179.985485138407));
#31683=CARTESIAN_POINT('Ctrl Pts',(-58.367123476447,-107.037617641849,179.985485069079));
#31684=CARTESIAN_POINT('Ctrl Pts',(-56.7096667264431,-107.120032376135,
179.985484999752));
#31685=CARTESIAN_POINT('Ctrl Pts',(-55.5347570765013,-107.151004365708,
178.813912075476));
#31686=CARTESIAN_POINT('Ctrl Pts',(-54.3598474265596,-107.181976355282,
177.6423391512));
#31687=CARTESIAN_POINT('Ctrl Pts',(-54.3499094325797,-107.088754583277,
175.985484901707));
#31688=CARTESIAN_POINT('Ctrl Pts',(-54.3399714385998,-106.995532811273,
174.328630652215));
#31689=CARTESIAN_POINT('Ctrl Pts',(-55.4950050601995,-106.778117281995,
173.157057825983));
#31690=CARTESIAN_POINT('Ctrl Pts',(-56.6500386817991,-106.560701752718,
171.985484999752));
#31691=CARTESIAN_POINT('Ctrl Pts',(-58.2876193059689,-106.291843489121,
171.985485069079));
#31692=CARTESIAN_POINT('Ctrl Pts',(-59.9251999301388,-106.022985225524,
171.985485138407));
#31693=CARTESIAN_POINT('Ctrl Pts',(-61.0802334542465,-105.80556970664,173.157058062683));
#31694=CARTESIAN_POINT('Ctrl Pts',(-62.2352669783543,-105.588154187756,
174.328630986959));
#31695=CARTESIAN_POINT('Ctrl Pts',(-62.2253288465001,-105.494932430449,
175.985485236451));
#31696=CARTESIAN_POINT('Ctrl Pts',(-62.2153907146459,-105.401710673143,
177.642339485944));
#31697=CARTESIAN_POINT('Ctrl Pts',(-61.0404809672123,-105.43268267311,178.813912312176));
#31698=CARTESIAN_POINT('Ctrl Pts',(-59.8655712197787,-105.463654673077,
179.985485138407));
#31699=CARTESIAN_POINT('Ctrl Pts',(-58.2081144697748,-105.546069407363,
179.985485069079));
#31700=CARTESIAN_POINT('Ctrl Pts',(-56.5506577197709,-105.628484141649,
179.985484999752));
#31701=CARTESIAN_POINT('Ctrl Pts',(-55.3757480698291,-105.659456131223,
178.813912075476));
#31702=CARTESIAN_POINT('Ctrl Pts',(-54.2008384198873,-105.690428120796,
177.6423391512));
#31703=CARTESIAN_POINT('Ctrl Pts',(-54.1909004259075,-105.597206348792,
175.985484901707));
#31704=CARTESIAN_POINT('Ctrl Pts',(-54.1809624319276,-105.503984576787,
174.328630652215));
#31705=CARTESIAN_POINT('Ctrl Pts',(-55.3359960535272,-105.28656904751,173.157057825983));
#31706=CARTESIAN_POINT('Ctrl Pts',(-56.4910296751268,-105.069153518232,
171.985484999752));
#31707=CARTESIAN_POINT('Ctrl Pts',(-58.1286102992967,-104.800295254635,
171.985485069079));
#31708=CARTESIAN_POINT('Ctrl Pts',(-59.7661909234666,-104.531436991038,
171.985485138407));
#31709=CARTESIAN_POINT('Ctrl Pts',(-60.9212244475743,-104.314021472154,
173.157058062683));
#31710=CARTESIAN_POINT('Ctrl Pts',(-62.0762579716821,-104.09660595327,174.328630986959));
#31711=CARTESIAN_POINT('Ctrl Pts',(-62.0663198398279,-104.003384195964,
175.985485236451));
#31712=CARTESIAN_POINT('Ctrl Pts',(-62.0563817079737,-103.910162438658,
177.642339485944));
#31713=CARTESIAN_POINT('Ctrl Pts',(-60.8814719605401,-103.941134438624,
178.813912312176));
#31714=CARTESIAN_POINT('Ctrl Pts',(-59.7065622131064,-103.972106438591,
179.985485138407));
#31715=CARTESIAN_POINT('Ctrl Pts',(-58.0491054631025,-104.054521172878,
179.985485069079));
#31716=CARTESIAN_POINT('Ctrl Pts',(-56.3916487130987,-104.136935907164,
179.985484999752));
#31717=CARTESIAN_POINT('Ctrl Pts',(-55.2167390631569,-104.167907896737,
178.813912075476));
#31718=CARTESIAN_POINT('Ctrl Pts',(-54.0418294132151,-104.198879886311,
177.6423391512));
#31719=CARTESIAN_POINT('Ctrl Pts',(-54.0318914192353,-104.105658114306,
175.985484901707));
#31720=CARTESIAN_POINT('Ctrl Pts',(-54.0219534252554,-104.012436342302,
174.328630652215));
#31721=CARTESIAN_POINT('Ctrl Pts',(-55.176987046855,-103.795020813024,173.157057825983));
#31722=CARTESIAN_POINT('Ctrl Pts',(-56.3320206684546,-103.577605283747,
171.985484999752));
#31723=CARTESIAN_POINT('Ctrl Pts',(-57.9696012926245,-103.30874702015,171.985485069079));
#31724=CARTESIAN_POINT('Ctrl Pts',(-59.6071819167943,-103.039888756553,
171.985485138407));
#31725=CARTESIAN_POINT('Ctrl Pts',(-60.7622154409021,-102.822473237669,
173.157058062683));
#31726=CARTESIAN_POINT('Ctrl Pts',(-61.9172489650099,-102.605057718784,
174.328630986959));
#31727=CARTESIAN_POINT('Ctrl Pts',(-61.9073108331557,-102.511835961478,
175.985485236451));
#31728=CARTESIAN_POINT('Ctrl Pts',(-61.8973727013015,-102.418614204172,
177.642339485944));
#31729=CARTESIAN_POINT('Ctrl Pts',(-60.7224629538678,-102.449586204139,
178.813912312176));
#31730=CARTESIAN_POINT('Ctrl Pts',(-59.5475532064342,-102.480558204106,
179.985485138407));
#31731=CARTESIAN_POINT('Ctrl Pts',(-57.8900964564303,-102.562972938392,
179.985485069079));
#31732=CARTESIAN_POINT('Ctrl Pts',(-56.2326397064264,-102.645387672678,
179.985484999752));
#31733=CARTESIAN_POINT('Ctrl Pts',(-55.0577300564847,-102.676359662252,
178.813912075476));
#31734=CARTESIAN_POINT('Ctrl Pts',(-53.8828204065429,-102.707331651825,
177.6423391512));
#31735=CARTESIAN_POINT('Ctrl Pts',(-53.872882412563,-102.614109879821,175.985484901707));
#31736=CARTESIAN_POINT('Ctrl Pts',(-53.8629444185832,-102.520888107816,
174.328630652215));
#31737=CARTESIAN_POINT('Ctrl Pts',(-55.0179780401828,-102.303472578539,
173.157057825983));
#31738=CARTESIAN_POINT('Ctrl Pts',(-56.1730116617824,-102.086057049261,
171.985484999752));
#31739=CARTESIAN_POINT('Ctrl Pts',(-57.8105922859523,-101.817198785664,
171.985485069079));
#31740=CARTESIAN_POINT('Ctrl Pts',(-59.4481729101221,-101.548340522067,
171.985485138407));
#31741=CARTESIAN_POINT('Ctrl Pts',(-60.6032064342299,-101.330925003183,
173.157058062683));
#31742=CARTESIAN_POINT('Ctrl Pts',(-61.7582399583376,-101.113509484299,
174.328630986959));
#31743=CARTESIAN_POINT('Ctrl Pts',(-61.7483018264834,-101.020287726993,
175.985485236451));
#31744=CARTESIAN_POINT('Ctrl Pts',(-61.7383636946293,-100.927065969686,
177.642339485944));
#31745=CARTESIAN_POINT('Ctrl Pts',(-60.5634539471956,-100.958037969653,
178.813912312176));
#31746=CARTESIAN_POINT('Ctrl Pts',(-59.388544199762,-100.98900996962,179.985485138407));
#31747=CARTESIAN_POINT('Ctrl Pts',(-57.7310874497581,-101.071424703906,
179.985485069079));
#31748=CARTESIAN_POINT('Ctrl Pts',(-56.0736306997542,-101.153839438193,
179.985484999752));
#31749=CARTESIAN_POINT('Ctrl Pts',(-54.8987210498124,-101.184811427766,
178.813912075476));
#31750=CARTESIAN_POINT('Ctrl Pts',(-53.7238113998707,-101.21578341734,177.6423391512));
#31751=CARTESIAN_POINT('Ctrl Pts',(-53.7138734058908,-101.122561645335,
175.985484901707));
#31752=CARTESIAN_POINT('Ctrl Pts',(-53.7039354119109,-101.029339873331,
174.328630652215));
#31753=CARTESIAN_POINT('Ctrl Pts',(-54.8589690335105,-100.811924344053,
173.157057825983));
#31754=CARTESIAN_POINT('Ctrl Pts',(-56.0140026551102,-100.594508814776,
171.985484999752));
#31755=CARTESIAN_POINT('Ctrl Pts',(-57.65158327928,-100.325650551179,171.985485069079));
#31756=CARTESIAN_POINT('Ctrl Pts',(-59.2891639034499,-100.056792287582,
171.985485138407));
#31757=CARTESIAN_POINT('Ctrl Pts',(-60.4441974275576,-99.8393767686974,
173.157058062683));
#31758=CARTESIAN_POINT('Ctrl Pts',(-61.5992309516654,-99.6219612498133,
174.328630986959));
#31759=CARTESIAN_POINT('Ctrl Pts',(-61.5892928198112,-99.528739492507,175.985485236451));
#31760=CARTESIAN_POINT('Ctrl Pts',(-61.579354687957,-99.4355177352008,177.642339485944));
#31761=CARTESIAN_POINT('Ctrl Pts',(-60.4044449405234,-99.4664897351676,
178.813912312176));
#31762=CARTESIAN_POINT('Ctrl Pts',(-59.2295351930898,-99.4974617351344,
179.985485138407));
#31763=CARTESIAN_POINT('Ctrl Pts',(-57.5720784430859,-99.5798764694207,
179.985485069079));
#31764=CARTESIAN_POINT('Ctrl Pts',(-55.914621693082,-99.662291203707,179.985484999752));
#31765=CARTESIAN_POINT('Ctrl Pts',(-54.7397120431402,-99.6932631932805,
178.813912075476));
#31766=CARTESIAN_POINT('Ctrl Pts',(-53.5648023931984,-99.724235182854,177.6423391512));
#31767=CARTESIAN_POINT('Ctrl Pts',(-53.5548643992186,-99.6310134108495,
175.985484901707));
#31768=CARTESIAN_POINT('Ctrl Pts',(-53.5449264052387,-99.5377916388449,
174.328630652215));
#31769=CARTESIAN_POINT('Ctrl Pts',(-54.6999600268383,-99.3203761095675,
173.157057825983));
#31770=CARTESIAN_POINT('Ctrl Pts',(-55.8549936484379,-99.10296058029,171.985484999752));
#31771=CARTESIAN_POINT('Ctrl Pts',(-57.4925742726078,-98.834102316693,171.985485069079));
#31772=CARTESIAN_POINT('Ctrl Pts',(-59.1301548967777,-98.5652440530961,
171.985485138407));
#31773=CARTESIAN_POINT('Ctrl Pts',(-60.2851884208854,-98.3478285342118,
173.157058062683));
#31774=CARTESIAN_POINT('Ctrl Pts',(-61.4402219449932,-98.1304130153276,
174.328630986959));
#31775=CARTESIAN_POINT('Ctrl Pts',(-61.430283813139,-98.0371912580215,175.985485236451));
#31776=CARTESIAN_POINT('Ctrl Pts',(-61.4203456812848,-97.9439695007152,
177.642339485944));
#31777=CARTESIAN_POINT('Ctrl Pts',(-60.2454359338512,-97.974941500682,178.813912312176));
#31778=CARTESIAN_POINT('Ctrl Pts',(-59.0705261864175,-98.0059135006488,
179.985485138407));
#31779=CARTESIAN_POINT('Ctrl Pts',(-57.4130694364136,-98.0883282349351,
179.985485069079));
#31780=CARTESIAN_POINT('Ctrl Pts',(-55.7556126864097,-98.1707429692214,
179.985484999752));
#31781=CARTESIAN_POINT('Ctrl Pts',(-54.580703036468,-98.2017149587949,178.813912075476));
#31782=CARTESIAN_POINT('Ctrl Pts',(-56.181115489574,-113.283598570176,178.821287383467));
#31783=CARTESIAN_POINT('Ctrl Pts',(-55.0031681001975,-113.314894403068,
177.646659506339));
#31784=CARTESIAN_POINT('Ctrl Pts',(-54.9932301063974,-113.221672631044,
175.985484901271));
#31785=CARTESIAN_POINT('Ctrl Pts',(-54.9832921125973,-113.12845085902,174.324310296203));
#31786=CARTESIAN_POINT('Ctrl Pts',(-56.1413634738858,-112.910711486397,
173.149682517375));
#31787=CARTESIAN_POINT('Ctrl Pts',(-57.2994348351743,-112.692972113774,
171.975054738546));
#31788=CARTESIAN_POINT('Ctrl Pts',(-58.9413114718314,-112.423655866545,
171.975054808055));
#31789=CARTESIAN_POINT('Ctrl Pts',(-60.5831881084886,-112.154339619316,
171.975054877564));
#31790=CARTESIAN_POINT('Ctrl Pts',(-61.741259372031,-111.936600257113,173.149682754692));
#31791=CARTESIAN_POINT('Ctrl Pts',(-62.8993306355734,-111.71886089491,174.32431063182));
#31792=CARTESIAN_POINT('Ctrl Pts',(-62.8893925035395,-111.625639137623,
175.985485236888));
#31793=CARTESIAN_POINT('Ctrl Pts',(-62.8794543715055,-111.532417380336,
177.646659841956));
#31794=CARTESIAN_POINT('Ctrl Pts',(-61.701506884383,-111.563713223648,178.821287620784));
#31795=CARTESIAN_POINT('Ctrl Pts',(-60.5235593972605,-111.595009066961,
179.995915399612));
#31796=CARTESIAN_POINT('Ctrl Pts',(-58.8618066347693,-111.677881784879,
179.995915330104));
#31797=CARTESIAN_POINT('Ctrl Pts',(-57.2000538722782,-111.760754502798,
179.995915260595));
#31798=CARTESIAN_POINT('Ctrl Pts',(-56.0221064829017,-111.79205033569,178.821287383467));
#31799=CARTESIAN_POINT('Ctrl Pts',(-54.8441590935253,-111.823346168582,
177.646659506339));
#31800=CARTESIAN_POINT('Ctrl Pts',(-54.8342210997252,-111.730124396559,
175.985484901271));
#31801=CARTESIAN_POINT('Ctrl Pts',(-54.8242831059251,-111.636902624535,
174.324310296203));
#31802=CARTESIAN_POINT('Ctrl Pts',(-55.9823544672136,-111.419163251912,
173.149682517375));
#31803=CARTESIAN_POINT('Ctrl Pts',(-57.1404258285021,-111.201423879289,
171.975054738546));
#31804=CARTESIAN_POINT('Ctrl Pts',(-58.7823024651592,-110.932107632059,
171.975054808055));
#31805=CARTESIAN_POINT('Ctrl Pts',(-60.4241791018163,-110.66279138483,171.975054877564));
#31806=CARTESIAN_POINT('Ctrl Pts',(-61.5822503653587,-110.445052022627,
173.149682754692));
#31807=CARTESIAN_POINT('Ctrl Pts',(-62.7403216289012,-110.227312660424,
174.32431063182));
#31808=CARTESIAN_POINT('Ctrl Pts',(-62.7303834968672,-110.134090903137,
175.985485236888));
#31809=CARTESIAN_POINT('Ctrl Pts',(-62.7204453648333,-110.04086914585,177.646659841956));
#31810=CARTESIAN_POINT('Ctrl Pts',(-61.5424978777108,-110.072164989163,
178.821287620784));
#31811=CARTESIAN_POINT('Ctrl Pts',(-60.3645503905882,-110.103460832475,
179.995915399612));
#31812=CARTESIAN_POINT('Ctrl Pts',(-58.7027976280971,-110.186333550394,
179.995915330104));
#31813=CARTESIAN_POINT('Ctrl Pts',(-57.041044865606,-110.269206268313,179.995915260595));
#31814=CARTESIAN_POINT('Ctrl Pts',(-55.8630974762295,-110.300502101205,
178.821287383467));
#31815=CARTESIAN_POINT('Ctrl Pts',(-54.6851500868531,-110.331797934097,
177.646659506339));
#31816=CARTESIAN_POINT('Ctrl Pts',(-54.675212093053,-110.238576162073,175.985484901271));
#31817=CARTESIAN_POINT('Ctrl Pts',(-54.6652740992529,-110.145354390049,
174.324310296203));
#31818=CARTESIAN_POINT('Ctrl Pts',(-55.8233454605414,-109.927615017426,
173.149682517375));
#31819=CARTESIAN_POINT('Ctrl Pts',(-56.9814168218299,-109.709875644803,
171.975054738546));
#31820=CARTESIAN_POINT('Ctrl Pts',(-58.623293458487,-109.440559397574,171.975054808055));
#31821=CARTESIAN_POINT('Ctrl Pts',(-60.2651700951441,-109.171243150344,
171.975054877564));
#31822=CARTESIAN_POINT('Ctrl Pts',(-61.4232413586865,-108.953503788142,
173.149682754692));
#31823=CARTESIAN_POINT('Ctrl Pts',(-62.581312622229,-108.735764425939,174.32431063182));
#31824=CARTESIAN_POINT('Ctrl Pts',(-62.571374490195,-108.642542668652,175.985485236888));
#31825=CARTESIAN_POINT('Ctrl Pts',(-62.5614363581611,-108.549320911365,
177.646659841956));
#31826=CARTESIAN_POINT('Ctrl Pts',(-61.3834888710385,-108.580616754677,
178.821287620784));
#31827=CARTESIAN_POINT('Ctrl Pts',(-60.205541383916,-108.61191259799,179.995915399612));
#31828=CARTESIAN_POINT('Ctrl Pts',(-58.5437886214249,-108.694785315908,
179.995915330104));
#31829=CARTESIAN_POINT('Ctrl Pts',(-56.8820358589338,-108.777658033827,
179.995915260595));
#31830=CARTESIAN_POINT('Ctrl Pts',(-55.7040884695573,-108.808953866719,
178.821287383467));
#31831=CARTESIAN_POINT('Ctrl Pts',(-54.5261410801808,-108.840249699611,
177.646659506339));
#31832=CARTESIAN_POINT('Ctrl Pts',(-54.5162030863807,-108.747027927587,
175.985484901271));
#31833=CARTESIAN_POINT('Ctrl Pts',(-54.5062650925806,-108.653806155564,
174.324310296203));
#31834=CARTESIAN_POINT('Ctrl Pts',(-55.6643364538691,-108.436066782941,
173.149682517375));
#31835=CARTESIAN_POINT('Ctrl Pts',(-56.8224078151577,-108.218327410317,
171.975054738546));
#31836=CARTESIAN_POINT('Ctrl Pts',(-58.4642844518147,-107.949011163088,
171.975054808055));
#31837=CARTESIAN_POINT('Ctrl Pts',(-60.1061610884719,-107.679694915859,
171.975054877564));
#31838=CARTESIAN_POINT('Ctrl Pts',(-61.2642323520143,-107.461955553656,
173.149682754692));
#31839=CARTESIAN_POINT('Ctrl Pts',(-62.4223036155567,-107.244216191453,
174.32431063182));
#31840=CARTESIAN_POINT('Ctrl Pts',(-62.4123654835228,-107.150994434166,
175.985485236888));
#31841=CARTESIAN_POINT('Ctrl Pts',(-62.4024273514889,-107.057772676879,
177.646659841956));
#31842=CARTESIAN_POINT('Ctrl Pts',(-61.2244798643663,-107.089068520192,
178.821287620784));
#31843=CARTESIAN_POINT('Ctrl Pts',(-60.0465323772438,-107.120364363504,
179.995915399612));
#31844=CARTESIAN_POINT('Ctrl Pts',(-58.3847796147526,-107.203237081423,
179.995915330104));
#31845=CARTESIAN_POINT('Ctrl Pts',(-56.7230268522615,-107.286109799341,
179.995915260595));
#31846=CARTESIAN_POINT('Ctrl Pts',(-55.5450794628851,-107.317405632233,
178.821287383467));
#31847=CARTESIAN_POINT('Ctrl Pts',(-54.3671320735086,-107.348701465125,
177.646659506339));
#31848=CARTESIAN_POINT('Ctrl Pts',(-54.3571940797085,-107.255479693102,
175.985484901271));
#31849=CARTESIAN_POINT('Ctrl Pts',(-54.3472560859084,-107.162257921078,
174.324310296203));
#31850=CARTESIAN_POINT('Ctrl Pts',(-55.5053274471969,-106.944518548455,
173.149682517375));
#31851=CARTESIAN_POINT('Ctrl Pts',(-56.6633988084854,-106.726779175832,
171.975054738546));
#31852=CARTESIAN_POINT('Ctrl Pts',(-58.3052754451425,-106.457462928602,
171.975054808055));
#31853=CARTESIAN_POINT('Ctrl Pts',(-59.9471520817997,-106.188146681373,
171.975054877564));
#31854=CARTESIAN_POINT('Ctrl Pts',(-61.1052233453421,-105.97040731917,173.149682754692));
#31855=CARTESIAN_POINT('Ctrl Pts',(-62.2632946088845,-105.752667956968,
174.32431063182));
#31856=CARTESIAN_POINT('Ctrl Pts',(-62.2533564768505,-105.659446199681,
175.985485236888));
#31857=CARTESIAN_POINT('Ctrl Pts',(-62.2434183448166,-105.566224442394,
177.646659841956));
#31858=CARTESIAN_POINT('Ctrl Pts',(-61.0654708576941,-105.597520285706,
178.821287620784));
#31859=CARTESIAN_POINT('Ctrl Pts',(-59.8875233705716,-105.628816129018,
179.995915399612));
#31860=CARTESIAN_POINT('Ctrl Pts',(-58.2257706080804,-105.711688846937,
179.995915330104));
#31861=CARTESIAN_POINT('Ctrl Pts',(-56.5640178455893,-105.794561564856,
179.995915260595));
#31862=CARTESIAN_POINT('Ctrl Pts',(-55.3860704562128,-105.825857397748,
178.821287383467));
#31863=CARTESIAN_POINT('Ctrl Pts',(-54.2081230668364,-105.85715323064,177.646659506339));
#31864=CARTESIAN_POINT('Ctrl Pts',(-54.1981850730363,-105.763931458616,
175.985484901271));
#31865=CARTESIAN_POINT('Ctrl Pts',(-54.1882470792362,-105.670709686593,
174.324310296203));
#31866=CARTESIAN_POINT('Ctrl Pts',(-55.3463184405247,-105.452970313969,
173.149682517375));
#31867=CARTESIAN_POINT('Ctrl Pts',(-56.5043898018132,-105.235230941346,
171.975054738546));
#31868=CARTESIAN_POINT('Ctrl Pts',(-58.1462664384703,-104.965914694117,
171.975054808055));
#31869=CARTESIAN_POINT('Ctrl Pts',(-59.7881430751274,-104.696598446888,
171.975054877564));
#31870=CARTESIAN_POINT('Ctrl Pts',(-60.9462143386698,-104.478859084685,
173.149682754692));
#31871=CARTESIAN_POINT('Ctrl Pts',(-62.1042856022123,-104.261119722482,
174.32431063182));
#31872=CARTESIAN_POINT('Ctrl Pts',(-62.0943474701783,-104.167897965195,
175.985485236888));
#31873=CARTESIAN_POINT('Ctrl Pts',(-62.0844093381444,-104.074676207908,
177.646659841956));
#31874=CARTESIAN_POINT('Ctrl Pts',(-60.9064618510219,-104.10597205122,178.821287620784));
#31875=CARTESIAN_POINT('Ctrl Pts',(-59.7285143638993,-104.137267894533,
179.995915399612));
#31876=CARTESIAN_POINT('Ctrl Pts',(-58.0667616014082,-104.220140612451,
179.995915330104));
#31877=CARTESIAN_POINT('Ctrl Pts',(-56.4050088389171,-104.30301333037,179.995915260595));
#31878=CARTESIAN_POINT('Ctrl Pts',(-55.2270614495406,-104.334309163262,
178.821287383467));
#31879=CARTESIAN_POINT('Ctrl Pts',(-54.0491140601642,-104.365604996154,
177.646659506339));
#31880=CARTESIAN_POINT('Ctrl Pts',(-54.039176066364,-104.272383224131,175.985484901271));
#31881=CARTESIAN_POINT('Ctrl Pts',(-54.029238072564,-104.179161452107,174.324310296203));
#31882=CARTESIAN_POINT('Ctrl Pts',(-55.1873094338524,-103.961422079484,
173.149682517375));
#31883=CARTESIAN_POINT('Ctrl Pts',(-56.345380795141,-103.743682706861,171.975054738546));
#31884=CARTESIAN_POINT('Ctrl Pts',(-57.9872574317981,-103.474366459631,
171.975054808055));
#31885=CARTESIAN_POINT('Ctrl Pts',(-59.6291340684552,-103.205050212402,
171.975054877564));
#31886=CARTESIAN_POINT('Ctrl Pts',(-60.7872053319976,-102.987310850199,
173.149682754692));
#31887=CARTESIAN_POINT('Ctrl Pts',(-61.94527659554,-102.769571487996,174.32431063182));
#31888=CARTESIAN_POINT('Ctrl Pts',(-61.9353384635061,-102.676349730709,
175.985485236888));
#31889=CARTESIAN_POINT('Ctrl Pts',(-61.9254003314722,-102.583127973422,
177.646659841956));
#31890=CARTESIAN_POINT('Ctrl Pts',(-60.7474528443496,-102.614423816735,
178.821287620784));
#31891=CARTESIAN_POINT('Ctrl Pts',(-59.5695053572271,-102.645719660047,
179.995915399612));
#31892=CARTESIAN_POINT('Ctrl Pts',(-57.907752594736,-102.728592377966,179.995915330104));
#31893=CARTESIAN_POINT('Ctrl Pts',(-56.2459998322448,-102.811465095885,
179.995915260595));
#31894=CARTESIAN_POINT('Ctrl Pts',(-55.0680524428684,-102.842760928777,
178.821287383467));
#31895=CARTESIAN_POINT('Ctrl Pts',(-53.8901050534919,-102.874056761669,
177.646659506339));
#31896=CARTESIAN_POINT('Ctrl Pts',(-53.8801670596918,-102.780834989645,
175.985484901271));
#31897=CARTESIAN_POINT('Ctrl Pts',(-53.8702290658917,-102.687613217621,
174.324310296203));
#31898=CARTESIAN_POINT('Ctrl Pts',(-55.0283004271802,-102.469873844998,
173.149682517375));
#31899=CARTESIAN_POINT('Ctrl Pts',(-56.1863717884687,-102.252134472375,
171.975054738546));
#31900=CARTESIAN_POINT('Ctrl Pts',(-57.8282484251258,-101.982818225146,
171.975054808055));
#31901=CARTESIAN_POINT('Ctrl Pts',(-59.470125061783,-101.713501977916,171.975054877564));
#31902=CARTESIAN_POINT('Ctrl Pts',(-60.6281963253254,-101.495762615714,
173.149682754692));
#31903=CARTESIAN_POINT('Ctrl Pts',(-61.7862675888678,-101.278023253511,
174.32431063182));
#31904=CARTESIAN_POINT('Ctrl Pts',(-61.7763294568339,-101.184801496224,
175.985485236888));
#31905=CARTESIAN_POINT('Ctrl Pts',(-61.7663913247999,-101.091579738937,
177.646659841956));
#31906=CARTESIAN_POINT('Ctrl Pts',(-60.5884438376774,-101.122875582249,
178.821287620784));
#31907=CARTESIAN_POINT('Ctrl Pts',(-59.4104963505549,-101.154171425562,
179.995915399612));
#31908=CARTESIAN_POINT('Ctrl Pts',(-57.7487435880637,-101.23704414348,179.995915330104));
#31909=CARTESIAN_POINT('Ctrl Pts',(-56.0869908255726,-101.319916861399,
179.995915260595));
#31910=CARTESIAN_POINT('Ctrl Pts',(-54.9090434361961,-101.351212694291,
178.821287383467));
#31911=CARTESIAN_POINT('Ctrl Pts',(-53.7310960468197,-101.382508527183,
177.646659506339));
#31912=CARTESIAN_POINT('Ctrl Pts',(-53.7211580530196,-101.289286755159,
175.985484901271));
#31913=CARTESIAN_POINT('Ctrl Pts',(-53.7112200592195,-101.196064983136,
174.324310296203));
#31914=CARTESIAN_POINT('Ctrl Pts',(-54.869291420508,-100.978325610513,173.149682517375));
#31915=CARTESIAN_POINT('Ctrl Pts',(-56.0273627817965,-100.760586237889,
171.975054738546));
#31916=CARTESIAN_POINT('Ctrl Pts',(-57.6692394184536,-100.49126999066,171.975054808055));
#31917=CARTESIAN_POINT('Ctrl Pts',(-59.3111160551107,-100.221953743431,
171.975054877564));
#31918=CARTESIAN_POINT('Ctrl Pts',(-60.4691873186531,-100.004214381228,
173.149682754692));
#31919=CARTESIAN_POINT('Ctrl Pts',(-61.6272585821956,-99.7864750190253,
174.32431063182));
#31920=CARTESIAN_POINT('Ctrl Pts',(-61.6173204501616,-99.6932532617382,
175.985485236888));
#31921=CARTESIAN_POINT('Ctrl Pts',(-61.6073823181277,-99.6000315044512,
177.646659841956));
#31922=CARTESIAN_POINT('Ctrl Pts',(-60.4294348310052,-99.6313273477637,
178.821287620784));
#31923=CARTESIAN_POINT('Ctrl Pts',(-59.2514873438827,-99.6626231910761,
179.995915399612));
#31924=CARTESIAN_POINT('Ctrl Pts',(-57.5897345813915,-99.7454959089947,
179.995915330104));
#31925=CARTESIAN_POINT('Ctrl Pts',(-55.9279818189004,-99.8283686269133,
179.995915260595));
#31926=CARTESIAN_POINT('Ctrl Pts',(-54.7500344295239,-99.8596644598054,
178.821287383467));
#31927=CARTESIAN_POINT('Ctrl Pts',(-53.5720870401475,-99.8909602926975,
177.646659506339));
#31928=CARTESIAN_POINT('Ctrl Pts',(-53.5621490463474,-99.7977385206737,
175.985484901271));
#31929=CARTESIAN_POINT('Ctrl Pts',(-53.5522110525473,-99.7045167486501,
174.324310296203));
#31930=CARTESIAN_POINT('Ctrl Pts',(-54.7102824138358,-99.4867773760269,
173.149682517375));
#31931=CARTESIAN_POINT('Ctrl Pts',(-55.8683537751243,-99.2690380034038,
171.975054738546));
#31932=CARTESIAN_POINT('Ctrl Pts',(-57.5102304117814,-98.9997217561745,
171.975054808055));
#31933=CARTESIAN_POINT('Ctrl Pts',(-59.1521070484385,-98.7304055089452,
171.975054877564));
#31934=CARTESIAN_POINT('Ctrl Pts',(-60.3101783119809,-98.5126661467424,
173.149682754692));
#31935=CARTESIAN_POINT('Ctrl Pts',(-61.4682495755234,-98.2949267845397,
174.32431063182));
#31936=CARTESIAN_POINT('Ctrl Pts',(-61.4583114434894,-98.2017050272526,
175.985485236888));
#31937=CARTESIAN_POINT('Ctrl Pts',(-61.4483733114555,-98.1084832699656,
177.646659841956));
#31938=CARTESIAN_POINT('Ctrl Pts',(-60.2704258243329,-98.139779113278,178.821287620784));
#31939=CARTESIAN_POINT('Ctrl Pts',(-59.0924783372104,-98.1710749565905,
179.995915399612));
#31940=CARTESIAN_POINT('Ctrl Pts',(-57.4307255747193,-98.2539476745091,
179.995915330104));
#31941=CARTESIAN_POINT('Ctrl Pts',(-55.7689728122282,-98.3368203924277,
179.995915260595));
#31942=CARTESIAN_POINT('Ctrl Pts',(-54.5910254228517,-98.3681162253198,
178.821287383467));
#31943=CARTESIAN_POINT('Ctrl Pts',(-56.1988062143188,-113.449542435949,
178.821287383467));
#31944=CARTESIAN_POINT('Ctrl Pts',(-55.0208588249424,-113.480838268841,
177.646659506339));
#31945=CARTESIAN_POINT('Ctrl Pts',(-55.0109208311422,-113.387616496817,
175.985484901271));
#31946=CARTESIAN_POINT('Ctrl Pts',(-55.0009828373422,-113.294394724794,
174.324310296203));
#31947=CARTESIAN_POINT('Ctrl Pts',(-56.1590541986307,-113.07665535217,173.149682517375));
#31948=CARTESIAN_POINT('Ctrl Pts',(-57.3171255599192,-112.858915979547,
171.975054738546));
#31949=CARTESIAN_POINT('Ctrl Pts',(-58.9590021965763,-112.589599732318,
171.975054808055));
#31950=CARTESIAN_POINT('Ctrl Pts',(-60.6008788332334,-112.320283485089,
171.975054877564));
#31951=CARTESIAN_POINT('Ctrl Pts',(-61.7589500967758,-112.102544122886,
173.149682754692));
#31952=CARTESIAN_POINT('Ctrl Pts',(-62.9170213603182,-111.884804760683,
174.32431063182));
#31953=CARTESIAN_POINT('Ctrl Pts',(-62.9070832282843,-111.791583003396,
175.985485236888));
#31954=CARTESIAN_POINT('Ctrl Pts',(-62.8971450962504,-111.698361246109,
177.646659841956));
#31955=CARTESIAN_POINT('Ctrl Pts',(-61.7191976091278,-111.729657089422,
178.821287620784));
#31956=CARTESIAN_POINT('Ctrl Pts',(-60.5412501220053,-111.760952932734,
179.995915399612));
#31957=CARTESIAN_POINT('Ctrl Pts',(-58.8794973595142,-111.843825650653,
179.995915330104));
#31958=CARTESIAN_POINT('Ctrl Pts',(-57.217744597023,-111.926698368571,179.995915260595));
#31959=CARTESIAN_POINT('Ctrl Pts',(-56.0397972076466,-111.957994201463,
178.821287383467));
#31960=CARTESIAN_POINT('Ctrl Pts',(-54.8618498182701,-111.989290034355,
177.646659506339));
#31961=CARTESIAN_POINT('Ctrl Pts',(-54.85191182447,-111.896068262332,175.985484901271));
#31962=CARTESIAN_POINT('Ctrl Pts',(-54.8419738306699,-111.802846490308,
174.324310296203));
#31963=CARTESIAN_POINT('Ctrl Pts',(-56.0000451919584,-111.585107117685,
173.149682517375));
#31964=CARTESIAN_POINT('Ctrl Pts',(-57.158116553247,-111.367367745062,171.975054738546));
#31965=CARTESIAN_POINT('Ctrl Pts',(-58.799993189904,-111.098051497832,171.975054808055));
#31966=CARTESIAN_POINT('Ctrl Pts',(-60.4418698265612,-110.828735250603,
171.975054877564));
#31967=CARTESIAN_POINT('Ctrl Pts',(-61.5999410901036,-110.6109958884,173.149682754692));
#31968=CARTESIAN_POINT('Ctrl Pts',(-62.758012353646,-110.393256526198,174.32431063182));
#31969=CARTESIAN_POINT('Ctrl Pts',(-62.7480742216121,-110.30003476891,175.985485236888));
#31970=CARTESIAN_POINT('Ctrl Pts',(-62.7381360895782,-110.206813011623,
177.646659841956));
#31971=CARTESIAN_POINT('Ctrl Pts',(-61.5601886024556,-110.238108854936,
178.821287620784));
#31972=CARTESIAN_POINT('Ctrl Pts',(-60.3822411153331,-110.269404698248,
179.995915399612));
#31973=CARTESIAN_POINT('Ctrl Pts',(-58.7204883528419,-110.352277416167,
179.995915330104));
#31974=CARTESIAN_POINT('Ctrl Pts',(-57.0587355903508,-110.435150134086,
179.995915260595));
#31975=CARTESIAN_POINT('Ctrl Pts',(-55.8807882009743,-110.466445966978,
178.821287383467));
#31976=CARTESIAN_POINT('Ctrl Pts',(-54.7028408115979,-110.49774179987,177.646659506339));
#31977=CARTESIAN_POINT('Ctrl Pts',(-54.6929028177978,-110.404520027846,
175.985484901271));
#31978=CARTESIAN_POINT('Ctrl Pts',(-54.6829648239977,-110.311298255822,
174.324310296203));
#31979=CARTESIAN_POINT('Ctrl Pts',(-55.8410361852862,-110.093558883199,
173.149682517375));
#31980=CARTESIAN_POINT('Ctrl Pts',(-56.9991075465747,-109.875819510576,
171.975054738546));
#31981=CARTESIAN_POINT('Ctrl Pts',(-58.6409841832318,-109.606503263347,
171.975054808055));
#31982=CARTESIAN_POINT('Ctrl Pts',(-60.2828608198889,-109.337187016117,
171.975054877564));
#31983=CARTESIAN_POINT('Ctrl Pts',(-61.4409320834313,-109.119447653915,
173.149682754692));
#31984=CARTESIAN_POINT('Ctrl Pts',(-62.5990033469738,-108.901708291712,
174.32431063182));
#31985=CARTESIAN_POINT('Ctrl Pts',(-62.5890652149398,-108.808486534425,
175.985485236888));
#31986=CARTESIAN_POINT('Ctrl Pts',(-62.5791270829059,-108.715264777138,
177.646659841956));
#31987=CARTESIAN_POINT('Ctrl Pts',(-61.4011795957834,-108.74656062045,178.821287620784));
#31988=CARTESIAN_POINT('Ctrl Pts',(-60.2232321086609,-108.777856463763,
179.995915399612));
#31989=CARTESIAN_POINT('Ctrl Pts',(-58.5614793461697,-108.860729181681,
179.995915330104));
#31990=CARTESIAN_POINT('Ctrl Pts',(-56.8997265836786,-108.9436018996,179.995915260595));
#31991=CARTESIAN_POINT('Ctrl Pts',(-55.7217791943021,-108.974897732492,
178.821287383467));
#31992=CARTESIAN_POINT('Ctrl Pts',(-54.5438318049257,-109.006193565384,
177.646659506339));
#31993=CARTESIAN_POINT('Ctrl Pts',(-54.5338938111256,-108.91297179336,175.985484901271));
#31994=CARTESIAN_POINT('Ctrl Pts',(-54.5239558173255,-108.819750021337,
174.324310296203));
#31995=CARTESIAN_POINT('Ctrl Pts',(-55.682027178614,-108.602010648714,173.149682517375));
#31996=CARTESIAN_POINT('Ctrl Pts',(-56.8400985399025,-108.384271276091,
171.975054738546));
#31997=CARTESIAN_POINT('Ctrl Pts',(-58.4819751765596,-108.114955028861,
171.975054808055));
#31998=CARTESIAN_POINT('Ctrl Pts',(-60.1238518132167,-107.845638781632,
171.975054877564));
#31999=CARTESIAN_POINT('Ctrl Pts',(-61.2819230767591,-107.627899419429,
173.149682754692));
#32000=CARTESIAN_POINT('Ctrl Pts',(-62.4399943403016,-107.410160057226,
174.32431063182));
#32001=CARTESIAN_POINT('Ctrl Pts',(-62.4300562082676,-107.316938299939,
175.985485236888));
#32002=CARTESIAN_POINT('Ctrl Pts',(-62.4201180762337,-107.223716542652,
177.646659841956));
#32003=CARTESIAN_POINT('Ctrl Pts',(-61.2421705891111,-107.255012385965,
178.821287620784));
#32004=CARTESIAN_POINT('Ctrl Pts',(-60.0642231019886,-107.286308229277,
179.995915399612));
#32005=CARTESIAN_POINT('Ctrl Pts',(-58.4024703394975,-107.369180947196,
179.995915330104));
#32006=CARTESIAN_POINT('Ctrl Pts',(-56.7407175770064,-107.452053665114,
179.995915260595));
#32007=CARTESIAN_POINT('Ctrl Pts',(-55.5627701876299,-107.483349498006,
178.821287383467));
#32008=CARTESIAN_POINT('Ctrl Pts',(-54.3848227982534,-107.514645330899,
177.646659506339));
#32009=CARTESIAN_POINT('Ctrl Pts',(-54.3748848044533,-107.421423558875,
175.985484901271));
#32010=CARTESIAN_POINT('Ctrl Pts',(-54.3649468106533,-107.328201786851,
174.324310296203));
#32011=CARTESIAN_POINT('Ctrl Pts',(-55.5230181719417,-107.110462414228,
173.149682517375));
#32012=CARTESIAN_POINT('Ctrl Pts',(-56.6810895332303,-106.892723041605,
171.975054738546));
#32013=CARTESIAN_POINT('Ctrl Pts',(-58.3229661698874,-106.623406794376,
171.975054808055));
#32014=CARTESIAN_POINT('Ctrl Pts',(-59.9648428065445,-106.354090547146,
171.975054877564));
#32015=CARTESIAN_POINT('Ctrl Pts',(-61.1229140700869,-106.136351184943,
173.149682754692));
#32016=CARTESIAN_POINT('Ctrl Pts',(-62.2809853336293,-105.918611822741,
174.32431063182));
#32017=CARTESIAN_POINT('Ctrl Pts',(-62.2710472015954,-105.825390065454,
175.985485236888));
#32018=CARTESIAN_POINT('Ctrl Pts',(-62.2611090695615,-105.732168308167,
177.646659841956));
#32019=CARTESIAN_POINT('Ctrl Pts',(-61.0831615824389,-105.763464151479,
178.821287620784));
#32020=CARTESIAN_POINT('Ctrl Pts',(-59.9052140953164,-105.794759994792,
179.995915399612));
#32021=CARTESIAN_POINT('Ctrl Pts',(-58.2434613328252,-105.87763271271,179.995915330104));
#32022=CARTESIAN_POINT('Ctrl Pts',(-56.5817085703341,-105.960505430629,
179.995915260595));
#32023=CARTESIAN_POINT('Ctrl Pts',(-55.4037611809577,-105.991801263521,
178.821287383467));
#32024=CARTESIAN_POINT('Ctrl Pts',(-54.2258137915812,-106.023097096413,
177.646659506339));
#32025=CARTESIAN_POINT('Ctrl Pts',(-54.2158757977811,-105.929875324389,
175.985484901271));
#32026=CARTESIAN_POINT('Ctrl Pts',(-54.205937803981,-105.836653552366,174.324310296203));
#32027=CARTESIAN_POINT('Ctrl Pts',(-55.3640091652695,-105.618914179742,
173.149682517375));
#32028=CARTESIAN_POINT('Ctrl Pts',(-56.522080526558,-105.401174807119,171.975054738546));
#32029=CARTESIAN_POINT('Ctrl Pts',(-58.1639571632151,-105.13185855989,171.975054808055));
#32030=CARTESIAN_POINT('Ctrl Pts',(-59.8058337998722,-104.862542312661,
171.975054877564));
#32031=CARTESIAN_POINT('Ctrl Pts',(-60.9639050634147,-104.644802950458,
173.149682754692));
#32032=CARTESIAN_POINT('Ctrl Pts',(-62.1219763269571,-104.427063588255,
174.32431063182));
#32033=CARTESIAN_POINT('Ctrl Pts',(-62.1120381949232,-104.333841830968,
175.985485236888));
#32034=CARTESIAN_POINT('Ctrl Pts',(-62.1021000628892,-104.240620073681,
177.646659841956));
#32035=CARTESIAN_POINT('Ctrl Pts',(-60.9241525757667,-104.271915916993,
178.821287620784));
#32036=CARTESIAN_POINT('Ctrl Pts',(-59.7462050886442,-104.303211760306,
179.995915399612));
#32037=CARTESIAN_POINT('Ctrl Pts',(-58.084452326153,-104.386084478225,179.995915330104));
#32038=CARTESIAN_POINT('Ctrl Pts',(-56.4226995636619,-104.468957196143,
179.995915260595));
#32039=CARTESIAN_POINT('Ctrl Pts',(-55.2447521742854,-104.500253029035,
178.821287383467));
#32040=CARTESIAN_POINT('Ctrl Pts',(-54.066804784909,-104.531548861927,177.646659506339));
#32041=CARTESIAN_POINT('Ctrl Pts',(-54.0568667911089,-104.438327089904,
175.985484901271));
#32042=CARTESIAN_POINT('Ctrl Pts',(-54.0469287973088,-104.34510531788,174.324310296203));
#32043=CARTESIAN_POINT('Ctrl Pts',(-55.2050001585973,-104.127365945257,
173.149682517375));
#32044=CARTESIAN_POINT('Ctrl Pts',(-56.3630715198858,-103.909626572634,
171.975054738546));
#32045=CARTESIAN_POINT('Ctrl Pts',(-58.0049481565429,-103.640310325404,
171.975054808055));
#32046=CARTESIAN_POINT('Ctrl Pts',(-59.6468247932,-103.370994078175,171.975054877564));
#32047=CARTESIAN_POINT('Ctrl Pts',(-60.8048960567424,-103.153254715972,
173.149682754692));
#32048=CARTESIAN_POINT('Ctrl Pts',(-61.9629673202849,-102.93551535377,174.32431063182));
#32049=CARTESIAN_POINT('Ctrl Pts',(-61.9530291882509,-102.842293596483,
175.985485236888));
#32050=CARTESIAN_POINT('Ctrl Pts',(-61.943091056217,-102.749071839196,177.646659841956));
#32051=CARTESIAN_POINT('Ctrl Pts',(-60.7651435690945,-102.780367682508,
178.821287620784));
#32052=CARTESIAN_POINT('Ctrl Pts',(-59.587196081972,-102.81166352582,179.995915399612));
#32053=CARTESIAN_POINT('Ctrl Pts',(-57.9254433194808,-102.894536243739,
179.995915330104));
#32054=CARTESIAN_POINT('Ctrl Pts',(-56.2636905569897,-102.977408961658,
179.995915260595));
#32055=CARTESIAN_POINT('Ctrl Pts',(-55.0857431676132,-103.00870479455,178.821287383467));
#32056=CARTESIAN_POINT('Ctrl Pts',(-53.9077957782368,-103.040000627442,
177.646659506339));
#32057=CARTESIAN_POINT('Ctrl Pts',(-53.8978577844367,-102.946778855418,
175.985484901271));
#32058=CARTESIAN_POINT('Ctrl Pts',(-53.8879197906366,-102.853557083394,
174.324310296203));
#32059=CARTESIAN_POINT('Ctrl Pts',(-55.0459911519251,-102.635817710771,
173.149682517375));
#32060=CARTESIAN_POINT('Ctrl Pts',(-56.2040625132136,-102.418078338148,
171.975054738546));
#32061=CARTESIAN_POINT('Ctrl Pts',(-57.8459391498707,-102.148762090919,
171.975054808055));
#32062=CARTESIAN_POINT('Ctrl Pts',(-59.4878157865278,-101.879445843689,
171.975054877564));
#32063=CARTESIAN_POINT('Ctrl Pts',(-60.6458870500702,-101.661706481487,
173.149682754692));
#32064=CARTESIAN_POINT('Ctrl Pts',(-61.8039583136126,-101.443967119284,
174.32431063182));
#32065=CARTESIAN_POINT('Ctrl Pts',(-61.7940201815787,-101.350745361997,
175.985485236888));
#32066=CARTESIAN_POINT('Ctrl Pts',(-61.7840820495448,-101.25752360471,177.646659841956));
#32067=CARTESIAN_POINT('Ctrl Pts',(-60.6061345624222,-101.288819448022,
178.821287620784));
#32068=CARTESIAN_POINT('Ctrl Pts',(-59.4281870752997,-101.320115291335,
179.995915399612));
#32069=CARTESIAN_POINT('Ctrl Pts',(-57.7664343128086,-101.402988009253,
179.995915330104));
#32070=CARTESIAN_POINT('Ctrl Pts',(-56.1046815503175,-101.485860727172,
179.995915260595));
#32071=CARTESIAN_POINT('Ctrl Pts',(-54.926734160941,-101.517156560064,178.821287383467));
#32072=CARTESIAN_POINT('Ctrl Pts',(-53.7487867715645,-101.548452392956,
177.646659506339));
#32073=CARTESIAN_POINT('Ctrl Pts',(-53.7388487777644,-101.455230620932,
175.985484901271));
#32074=CARTESIAN_POINT('Ctrl Pts',(-53.7289107839643,-101.362008848909,
174.324310296203));
#32075=CARTESIAN_POINT('Ctrl Pts',(-54.8869821452528,-101.144269476286,
173.149682517375));
#32076=CARTESIAN_POINT('Ctrl Pts',(-56.0450535065414,-100.926530103662,
171.975054738546));
#32077=CARTESIAN_POINT('Ctrl Pts',(-57.6869301431984,-100.657213856433,
171.975054808055));
#32078=CARTESIAN_POINT('Ctrl Pts',(-59.3288067798556,-100.387897609204,
171.975054877564));
#32079=CARTESIAN_POINT('Ctrl Pts',(-60.486878043398,-100.170158247001,173.149682754692));
#32080=CARTESIAN_POINT('Ctrl Pts',(-61.6449493069404,-99.9524188847983,
174.32431063182));
#32081=CARTESIAN_POINT('Ctrl Pts',(-61.6350111749065,-99.8591971275113,
175.985485236888));
#32082=CARTESIAN_POINT('Ctrl Pts',(-61.6250730428726,-99.7659753702243,
177.646659841956));
#32083=CARTESIAN_POINT('Ctrl Pts',(-60.44712555575,-99.7972712135367,178.821287620784));
#32084=CARTESIAN_POINT('Ctrl Pts',(-59.2691780686275,-99.8285670568492,
179.995915399612));
#32085=CARTESIAN_POINT('Ctrl Pts',(-57.6074253061363,-99.9114397747677,
179.995915330104));
#32086=CARTESIAN_POINT('Ctrl Pts',(-55.9456725436452,-99.9943124926864,
179.995915260595));
#32087=CARTESIAN_POINT('Ctrl Pts',(-54.7677251542687,-100.025608325578,
178.821287383467));
#32088=CARTESIAN_POINT('Ctrl Pts',(-53.5897777648923,-100.05690415847,177.646659506339));
#32089=CARTESIAN_POINT('Ctrl Pts',(-53.5798397710922,-99.9636823864468,
175.985484901271));
#32090=CARTESIAN_POINT('Ctrl Pts',(-53.5699017772921,-99.8704606144232,
174.324310296203));
#32091=CARTESIAN_POINT('Ctrl Pts',(-54.7279731385806,-99.6527212418,173.149682517375));
#32092=CARTESIAN_POINT('Ctrl Pts',(-55.8860444998691,-99.4349818691769,
171.975054738546));
#32093=CARTESIAN_POINT('Ctrl Pts',(-57.5279211365262,-99.1656656219475,
171.975054808055));
#32094=CARTESIAN_POINT('Ctrl Pts',(-59.1697977731833,-98.8963493747183,
171.975054877564));
#32095=CARTESIAN_POINT('Ctrl Pts',(-60.3278690367257,-98.6786100125155,
173.149682754692));
#32096=CARTESIAN_POINT('Ctrl Pts',(-61.4859403002682,-98.4608706503128,
174.32431063182));
#32097=CARTESIAN_POINT('Ctrl Pts',(-61.4760021682342,-98.3676488930257,
175.985485236888));
#32098=CARTESIAN_POINT('Ctrl Pts',(-61.4660640362003,-98.2744271357387,
177.646659841956));
#32099=CARTESIAN_POINT('Ctrl Pts',(-60.2881165490778,-98.3057229790511,
178.821287620784));
#32100=CARTESIAN_POINT('Ctrl Pts',(-59.1101690619552,-98.3370188223636,
179.995915399612));
#32101=CARTESIAN_POINT('Ctrl Pts',(-57.4484162994641,-98.4198915402821,
179.995915330104));
#32102=CARTESIAN_POINT('Ctrl Pts',(-55.786663536973,-98.5027642582008,179.995915260595));
#32103=CARTESIAN_POINT('Ctrl Pts',(-54.6087161475965,-98.5340600910929,
178.821287383467));
#32104=CARTESIAN_POINT('Ctrl Pts',(-56.2237961054143,-113.614380048479,
178.813912075476));
#32105=CARTESIAN_POINT('Ctrl Pts',(-55.0488864554725,-113.645352038053,
177.6423391512));
#32106=CARTESIAN_POINT('Ctrl Pts',(-55.0389484614927,-113.552130266048,
175.985484901707));
#32107=CARTESIAN_POINT('Ctrl Pts',(-55.0290104675128,-113.458908494044,
174.328630652215));
#32108=CARTESIAN_POINT('Ctrl Pts',(-56.1840440891124,-113.241492964766,
173.157057825983));
#32109=CARTESIAN_POINT('Ctrl Pts',(-57.3390777107121,-113.024077435489,
171.985484999752));
#32110=CARTESIAN_POINT('Ctrl Pts',(-58.9766583348819,-112.755219171892,
171.985485069079));
#32111=CARTESIAN_POINT('Ctrl Pts',(-60.6142389590518,-112.486360908295,
171.985485138407));
#32112=CARTESIAN_POINT('Ctrl Pts',(-61.7692724831595,-112.268945389411,
173.157058062683));
#32113=CARTESIAN_POINT('Ctrl Pts',(-62.9243060072673,-112.051529870527,
174.328630986959));
#32114=CARTESIAN_POINT('Ctrl Pts',(-62.9143678754131,-111.95830811322,175.985485236451));
#32115=CARTESIAN_POINT('Ctrl Pts',(-62.9044297435589,-111.865086355914,
177.642339485944));
#32116=CARTESIAN_POINT('Ctrl Pts',(-61.7295199961253,-111.896058355881,
178.813912312176));
#32117=CARTESIAN_POINT('Ctrl Pts',(-60.5546102486917,-111.927030355848,
179.985485138407));
#32118=CARTESIAN_POINT('Ctrl Pts',(-58.8971534986878,-112.009445090134,
179.985485069079));
#32119=CARTESIAN_POINT('Ctrl Pts',(-57.2396967486839,-112.09185982442,179.985484999752));
#32120=CARTESIAN_POINT('Ctrl Pts',(-56.0647870987421,-112.122831813994,
178.813912075476));
#32121=CARTESIAN_POINT('Ctrl Pts',(-54.8898774488003,-112.153803803567,
177.6423391512));
#32122=CARTESIAN_POINT('Ctrl Pts',(-54.8799394548205,-112.060582031563,
175.985484901707));
#32123=CARTESIAN_POINT('Ctrl Pts',(-54.8700014608406,-111.967360259558,
174.328630652215));
#32124=CARTESIAN_POINT('Ctrl Pts',(-56.0250350824402,-111.749944730281,
173.157057825983));
#32125=CARTESIAN_POINT('Ctrl Pts',(-57.1800687040398,-111.532529201003,
171.985484999752));
#32126=CARTESIAN_POINT('Ctrl Pts',(-58.8176493282097,-111.263670937406,
171.985485069079));
#32127=CARTESIAN_POINT('Ctrl Pts',(-60.4552299523796,-110.994812673809,
171.985485138407));
#32128=CARTESIAN_POINT('Ctrl Pts',(-61.6102634764873,-110.777397154925,
173.157058062683));
#32129=CARTESIAN_POINT('Ctrl Pts',(-62.7652970005951,-110.559981636041,
174.328630986959));
#32130=CARTESIAN_POINT('Ctrl Pts',(-62.7553588687409,-110.466759878735,
175.985485236451));
#32131=CARTESIAN_POINT('Ctrl Pts',(-62.7454207368867,-110.373538121429,
177.642339485944));
#32132=CARTESIAN_POINT('Ctrl Pts',(-61.5705109894531,-110.404510121395,
178.813912312176));
#32133=CARTESIAN_POINT('Ctrl Pts',(-60.3956012420194,-110.435482121362,
179.985485138407));
#32134=CARTESIAN_POINT('Ctrl Pts',(-58.7381444920155,-110.517896855648,
179.985485069079));
#32135=CARTESIAN_POINT('Ctrl Pts',(-57.0806877420116,-110.600311589935,
179.985484999752));
#32136=CARTESIAN_POINT('Ctrl Pts',(-55.9057780920699,-110.631283579508,
178.813912075476));
#32137=CARTESIAN_POINT('Ctrl Pts',(-54.7308684421281,-110.662255569082,
177.6423391512));
#32138=CARTESIAN_POINT('Ctrl Pts',(-54.7209304481482,-110.569033797077,
175.985484901707));
#32139=CARTESIAN_POINT('Ctrl Pts',(-54.7109924541684,-110.475812025073,
174.328630652215));
#32140=CARTESIAN_POINT('Ctrl Pts',(-55.866026075768,-110.258396495795,173.157057825983));
#32141=CARTESIAN_POINT('Ctrl Pts',(-57.0210596973676,-110.040980966518,
171.985484999752));
#32142=CARTESIAN_POINT('Ctrl Pts',(-58.6586403215375,-109.772122702921,
171.985485069079));
#32143=CARTESIAN_POINT('Ctrl Pts',(-60.2962209457073,-109.503264439324,
171.985485138407));
#32144=CARTESIAN_POINT('Ctrl Pts',(-61.4512544698151,-109.28584892044,173.157058062683));
#32145=CARTESIAN_POINT('Ctrl Pts',(-62.6062879939228,-109.068433401555,
174.328630986959));
#32146=CARTESIAN_POINT('Ctrl Pts',(-62.5963498620687,-108.975211644249,
175.985485236451));
#32147=CARTESIAN_POINT('Ctrl Pts',(-62.5864117302145,-108.881989886943,
177.642339485944));
#32148=CARTESIAN_POINT('Ctrl Pts',(-61.4115019827808,-108.91296188691,178.813912312176));
#32149=CARTESIAN_POINT('Ctrl Pts',(-60.2365922353472,-108.943933886877,
179.985485138407));
#32150=CARTESIAN_POINT('Ctrl Pts',(-58.5791354853433,-109.026348621163,
179.985485069079));
#32151=CARTESIAN_POINT('Ctrl Pts',(-56.9216787353394,-109.108763355449,
179.985484999752));
#32152=CARTESIAN_POINT('Ctrl Pts',(-55.7467690853976,-109.139735345023,
178.813912075476));
#32153=CARTESIAN_POINT('Ctrl Pts',(-54.5718594354559,-109.170707334596,
177.6423391512));
#32154=CARTESIAN_POINT('Ctrl Pts',(-54.561921441476,-109.077485562592,175.985484901707));
#32155=CARTESIAN_POINT('Ctrl Pts',(-54.5519834474962,-108.984263790587,
174.328630652215));
#32156=CARTESIAN_POINT('Ctrl Pts',(-55.7070170690958,-108.76684826131,173.157057825983));
#32157=CARTESIAN_POINT('Ctrl Pts',(-56.8620506906954,-108.549432732032,
171.985484999752));
#32158=CARTESIAN_POINT('Ctrl Pts',(-58.4996313148652,-108.280574468435,
171.985485069079));
#32159=CARTESIAN_POINT('Ctrl Pts',(-60.1372119390351,-108.011716204838,
171.985485138407));
#32160=CARTESIAN_POINT('Ctrl Pts',(-61.2922454631428,-107.794300685954,
173.157058062683));
#32161=CARTESIAN_POINT('Ctrl Pts',(-62.4472789872506,-107.57688516707,174.328630986959));
#32162=CARTESIAN_POINT('Ctrl Pts',(-62.4373408553964,-107.483663409764,
175.985485236451));
#32163=CARTESIAN_POINT('Ctrl Pts',(-62.4274027235423,-107.390441652457,
177.642339485944));
#32164=CARTESIAN_POINT('Ctrl Pts',(-61.2524929761086,-107.421413652424,
178.813912312176));
#32165=CARTESIAN_POINT('Ctrl Pts',(-60.077583228675,-107.452385652391,179.985485138407));
#32166=CARTESIAN_POINT('Ctrl Pts',(-58.4201264786711,-107.534800386677,
179.985485069079));
#32167=CARTESIAN_POINT('Ctrl Pts',(-56.7626697286672,-107.617215120964,
179.985484999752));
#32168=CARTESIAN_POINT('Ctrl Pts',(-55.5877600787254,-107.648187110537,
178.813912075476));
#32169=CARTESIAN_POINT('Ctrl Pts',(-54.4128504287836,-107.67915910011,177.6423391512));
#32170=CARTESIAN_POINT('Ctrl Pts',(-54.4029124348038,-107.585937328106,
175.985484901707));
#32171=CARTESIAN_POINT('Ctrl Pts',(-54.3929744408239,-107.492715556102,
174.328630652215));
#32172=CARTESIAN_POINT('Ctrl Pts',(-55.5480080624235,-107.275300026824,
173.157057825983));
#32173=CARTESIAN_POINT('Ctrl Pts',(-56.7030416840231,-107.057884497547,
171.985484999752));
#32174=CARTESIAN_POINT('Ctrl Pts',(-58.340622308193,-106.78902623395,171.985485069079));
#32175=CARTESIAN_POINT('Ctrl Pts',(-59.9782029323629,-106.520167970353,
171.985485138407));
#32176=CARTESIAN_POINT('Ctrl Pts',(-61.1332364564706,-106.302752451468,
173.157058062683));
#32177=CARTESIAN_POINT('Ctrl Pts',(-62.2882699805784,-106.085336932584,
174.328630986959));
#32178=CARTESIAN_POINT('Ctrl Pts',(-62.2783318487242,-105.992115175278,
175.985485236451));
#32179=CARTESIAN_POINT('Ctrl Pts',(-62.26839371687,-105.898893417972,177.642339485944));
#32180=CARTESIAN_POINT('Ctrl Pts',(-61.0934839694364,-105.929865417939,
178.813912312176));
#32181=CARTESIAN_POINT('Ctrl Pts',(-59.9185742220028,-105.960837417905,
179.985485138407));
#32182=CARTESIAN_POINT('Ctrl Pts',(-58.2611174719989,-106.043252152192,
179.985485069079));
#32183=CARTESIAN_POINT('Ctrl Pts',(-56.603660721995,-106.125666886478,179.985484999752));
#32184=CARTESIAN_POINT('Ctrl Pts',(-55.4287510720532,-106.156638876051,
178.813912075476));
#32185=CARTESIAN_POINT('Ctrl Pts',(-54.2538414221114,-106.187610865625,
177.6423391512));
#32186=CARTESIAN_POINT('Ctrl Pts',(-54.2439034281315,-106.09438909362,175.985484901707));
#32187=CARTESIAN_POINT('Ctrl Pts',(-54.2339654341517,-106.001167321616,
174.328630652215));
#32188=CARTESIAN_POINT('Ctrl Pts',(-55.3889990557513,-105.783751792338,
173.157057825983));
#32189=CARTESIAN_POINT('Ctrl Pts',(-56.5440326773509,-105.566336263061,
171.985484999752));
#32190=CARTESIAN_POINT('Ctrl Pts',(-58.1816133015208,-105.297477999464,
171.985485069079));
#32191=CARTESIAN_POINT('Ctrl Pts',(-59.8191939256906,-105.028619735867,
171.985485138407));
#32192=CARTESIAN_POINT('Ctrl Pts',(-60.9742274497984,-104.811204216983,
173.157058062683));
#32193=CARTESIAN_POINT('Ctrl Pts',(-62.1292609739061,-104.593788698099,
174.328630986959));
#32194=CARTESIAN_POINT('Ctrl Pts',(-62.119322842052,-104.500566940792,175.985485236451));
#32195=CARTESIAN_POINT('Ctrl Pts',(-62.1093847101978,-104.407345183486,
177.642339485944));
#32196=CARTESIAN_POINT('Ctrl Pts',(-60.9344749627642,-104.438317183453,
178.813912312176));
#32197=CARTESIAN_POINT('Ctrl Pts',(-59.7595652153305,-104.46928918342,179.985485138407));
#32198=CARTESIAN_POINT('Ctrl Pts',(-58.1021084653266,-104.551703917706,
179.985485069079));
#32199=CARTESIAN_POINT('Ctrl Pts',(-56.4446517153227,-104.634118651992,
179.985484999752));
#32200=CARTESIAN_POINT('Ctrl Pts',(-55.269742065381,-104.665090641566,178.813912075476));
#32201=CARTESIAN_POINT('Ctrl Pts',(-54.0948324154392,-104.696062631139,
177.6423391512));
#32202=CARTESIAN_POINT('Ctrl Pts',(-54.0848944214593,-104.602840859135,
175.985484901707));
#32203=CARTESIAN_POINT('Ctrl Pts',(-54.0749564274795,-104.50961908713,174.328630652215));
#32204=CARTESIAN_POINT('Ctrl Pts',(-55.2299900490791,-104.292203557853,
173.157057825983));
#32205=CARTESIAN_POINT('Ctrl Pts',(-56.3850236706787,-104.074788028575,
171.985484999752));
#32206=CARTESIAN_POINT('Ctrl Pts',(-58.0226042948486,-103.805929764978,
171.985485069079));
#32207=CARTESIAN_POINT('Ctrl Pts',(-59.6601849190184,-103.537071501381,
171.985485138407));
#32208=CARTESIAN_POINT('Ctrl Pts',(-60.8152184431262,-103.319655982497,
173.157058062683));
#32209=CARTESIAN_POINT('Ctrl Pts',(-61.9702519672339,-103.102240463613,
174.328630986959));
#32210=CARTESIAN_POINT('Ctrl Pts',(-61.9603138353797,-103.009018706307,
175.985485236451));
#32211=CARTESIAN_POINT('Ctrl Pts',(-61.9503757035256,-102.915796949001,
177.642339485944));
#32212=CARTESIAN_POINT('Ctrl Pts',(-60.7754659560919,-102.946768948967,
178.813912312176));
#32213=CARTESIAN_POINT('Ctrl Pts',(-59.6005562086583,-102.977740948934,
179.985485138407));
#32214=CARTESIAN_POINT('Ctrl Pts',(-57.9430994586544,-103.06015568322,179.985485069079));
#32215=CARTESIAN_POINT('Ctrl Pts',(-56.2856427086505,-103.142570417507,
179.985484999752));
#32216=CARTESIAN_POINT('Ctrl Pts',(-55.1107330587087,-103.17354240708,178.813912075476));
#32217=CARTESIAN_POINT('Ctrl Pts',(-53.935823408767,-103.204514396654,177.6423391512));
#32218=CARTESIAN_POINT('Ctrl Pts',(-53.9258854147871,-103.111292624649,
175.985484901707));
#32219=CARTESIAN_POINT('Ctrl Pts',(-53.9159474208072,-103.018070852645,
174.328630652215));
#32220=CARTESIAN_POINT('Ctrl Pts',(-55.0709810424069,-102.800655323367,
173.157057825983));
#32221=CARTESIAN_POINT('Ctrl Pts',(-56.2260146640065,-102.58323979409,171.985484999752));
#32222=CARTESIAN_POINT('Ctrl Pts',(-57.8635952881763,-102.314381530493,
171.985485069079));
#32223=CARTESIAN_POINT('Ctrl Pts',(-59.5011759123462,-102.045523266896,
171.985485138407));
#32224=CARTESIAN_POINT('Ctrl Pts',(-60.6562094364539,-101.828107748012,
173.157058062683));
#32225=CARTESIAN_POINT('Ctrl Pts',(-61.8112429605617,-101.610692229127,
174.328630986959));
#32226=CARTESIAN_POINT('Ctrl Pts',(-61.8013048287075,-101.517470471821,
175.985485236451));
#32227=CARTESIAN_POINT('Ctrl Pts',(-61.7913666968533,-101.424248714515,
177.642339485944));
#32228=CARTESIAN_POINT('Ctrl Pts',(-60.6164569494197,-101.455220714482,
178.813912312176));
#32229=CARTESIAN_POINT('Ctrl Pts',(-59.4415472019861,-101.486192714449,
179.985485138407));
#32230=CARTESIAN_POINT('Ctrl Pts',(-57.7840904519822,-101.568607448735,
179.985485069079));
#32231=CARTESIAN_POINT('Ctrl Pts',(-56.1266337019783,-101.651022183021,
179.985484999752));
#32232=CARTESIAN_POINT('Ctrl Pts',(-54.9517240520365,-101.681994172595,
178.813912075476));
#32233=CARTESIAN_POINT('Ctrl Pts',(-53.7768144020947,-101.712966162168,
177.6423391512));
#32234=CARTESIAN_POINT('Ctrl Pts',(-53.7668764081149,-101.619744390164,
175.985484901707));
#32235=CARTESIAN_POINT('Ctrl Pts',(-53.756938414135,-101.526522618159,174.328630652215));
#32236=CARTESIAN_POINT('Ctrl Pts',(-54.9119720357346,-101.309107088882,
173.157057825983));
#32237=CARTESIAN_POINT('Ctrl Pts',(-56.0670056573342,-101.091691559604,
171.985484999752));
#32238=CARTESIAN_POINT('Ctrl Pts',(-57.7045862815041,-100.822833296007,
171.985485069079));
#32239=CARTESIAN_POINT('Ctrl Pts',(-59.342166905674,-100.55397503241,171.985485138407));
#32240=CARTESIAN_POINT('Ctrl Pts',(-60.4972004297817,-100.336559513526,
173.157058062683));
#32241=CARTESIAN_POINT('Ctrl Pts',(-61.6522339538895,-100.119143994642,
174.328630986959));
#32242=CARTESIAN_POINT('Ctrl Pts',(-61.6422958220353,-100.025922237336,
175.985485236451));
#32243=CARTESIAN_POINT('Ctrl Pts',(-61.6323576901811,-99.9327004800294,
177.642339485944));
#32244=CARTESIAN_POINT('Ctrl Pts',(-60.4574479427475,-99.9636724799962,
178.813912312176));
#32245=CARTESIAN_POINT('Ctrl Pts',(-59.2825381953138,-99.994644479963,179.985485138407));
#32246=CARTESIAN_POINT('Ctrl Pts',(-57.6250814453099,-100.077059214249,
179.985485069079));
#32247=CARTESIAN_POINT('Ctrl Pts',(-55.9676246953061,-100.159473948536,
179.985484999752));
#32248=CARTESIAN_POINT('Ctrl Pts',(-54.7927150453643,-100.190445938109,
178.813912075476));
#32249=CARTESIAN_POINT('Ctrl Pts',(-53.6178053954225,-100.221417927683,
177.6423391512));
#32250=CARTESIAN_POINT('Ctrl Pts',(-53.6078674014426,-100.128196155678,
175.985484901707));
#32251=CARTESIAN_POINT('Ctrl Pts',(-53.5979294074628,-100.034974383673,
174.328630652215));
#32252=CARTESIAN_POINT('Ctrl Pts',(-54.7529630290624,-99.817558854396,173.157057825983));
#32253=CARTESIAN_POINT('Ctrl Pts',(-55.907996650662,-99.6001433251185,171.985484999752));
#32254=CARTESIAN_POINT('Ctrl Pts',(-57.5455772748319,-99.3312850615215,
171.985485069079));
#32255=CARTESIAN_POINT('Ctrl Pts',(-59.1831578990017,-99.0624267979246,
171.985485138407));
#32256=CARTESIAN_POINT('Ctrl Pts',(-60.3381914231095,-98.8450112790404,
173.157058062683));
#32257=CARTESIAN_POINT('Ctrl Pts',(-61.4932249472172,-98.6275957601562,
174.328630986959));
#32258=CARTESIAN_POINT('Ctrl Pts',(-61.4832868153631,-98.53437400285,175.985485236451));
#32259=CARTESIAN_POINT('Ctrl Pts',(-61.4733486835089,-98.4411522455438,
177.642339485944));
#32260=CARTESIAN_POINT('Ctrl Pts',(-60.2984389360752,-98.4721242455106,
178.813912312176));
#32261=CARTESIAN_POINT('Ctrl Pts',(-59.1235291886416,-98.5030962454774,
179.985485138407));
#32262=CARTESIAN_POINT('Ctrl Pts',(-57.4660724386377,-98.5855109797636,
179.985485069079));
#32263=CARTESIAN_POINT('Ctrl Pts',(-55.8086156886338,-98.6679257140499,
179.985484999752));
#32264=CARTESIAN_POINT('Ctrl Pts',(-54.633706038692,-98.6988977036234,178.813912075476));
#32265=CARTESIAN_POINT('Origin',(-31.7758655563387,23.6116972707429,178.485485069079));
#32266=CARTESIAN_POINT('Origin',(-31.7758655563387,23.6116972707429,173.985485069079));
#32267=CARTESIAN_POINT('Origin',(-31.7758655563387,23.6116972707429,177.985485069079));
#32268=CARTESIAN_POINT('Ctrl Pts',(-33.7101944105682,36.1001541204655,173.485485069079));
#32269=CARTESIAN_POINT('Ctrl Pts',(-33.9682581825426,35.6003903982821,173.143998023837));
#32270=CARTESIAN_POINT('Ctrl Pts',(-33.3358320373305,35.4434146616551,173.235485069079));
#32271=CARTESIAN_POINT('Ctrl Pts',(-33.5757636385812,36.3604914102378,172.982269696584));
#32272=CARTESIAN_POINT('Ctrl Pts',(-33.8204276914646,35.8561010262747,172.645545369172));
#32273=CARTESIAN_POINT('Ctrl Pts',(-33.1880191877447,35.7136289261714,172.732268406515));
#32274=CARTESIAN_POINT('Ctrl Pts',(-33.4516565150982,36.6248074047901,172.479340629102));
#32275=CARTESIAN_POINT('Ctrl Pts',(-33.6822917663529,36.1173819195843,172.144313013639));
#32276=CARTESIAN_POINT('Ctrl Pts',(-33.0506074115036,35.9881357503632,172.229339795881));
#32277=CARTESIAN_POINT('Ctrl Pts',(-33.3378144598069,36.8927267103254,171.976487691182));
#32278=CARTESIAN_POINT('Ctrl Pts',(-33.5545758603726,36.3825939324359,171.641904135334));
#32279=CARTESIAN_POINT('Ctrl Pts',(-32.9232632882234,36.2665888893428,171.726487691182));
#32280=CARTESIAN_POINT('Origin',(-33.26592800316,35.8707475833996,173.485485069079));
#32281=CARTESIAN_POINT('Ctrl Pts',(-34.1412494001895,35.3369392868692,173.985485069079));
#32282=CARTESIAN_POINT('Ctrl Pts',(-34.1412494001895,35.3369392868692,173.485485069079));
#32283=CARTESIAN_POINT('Ctrl Pts',(-33.7154041461839,35.0749167312735,173.485485069079));
#32284=CARTESIAN_POINT('Ctrl Pts',(-34.0503675686949,35.4846425887064,173.985485046591));
#32285=CARTESIAN_POINT('Ctrl Pts',(-34.0908546515829,35.4188420329393,173.456207535552));
#32286=CARTESIAN_POINT('Ctrl Pts',(-33.6387071223109,35.1455646668778,173.485485069079));
#32287=CARTESIAN_POINT('Ctrl Pts',(-33.9619493301675,35.6363826725923,173.940377868901));
#32288=CARTESIAN_POINT('Ctrl Pts',(-34.050965142566,35.4840104825677,173.400217226376));
#32289=CARTESIAN_POINT('Ctrl Pts',(-33.5621652331424,35.2185830930478,173.462931467345));
#32290=CARTESIAN_POINT('Ctrl Pts',(-33.8135226820125,35.9025198720883,173.769060220931));
#32291=CARTESIAN_POINT('Ctrl Pts',(-33.9938812681979,35.5714820882983,173.274080148675));
#32292=CARTESIAN_POINT('Ctrl Pts',(-33.4306927660806,35.3472393598486,173.37727264665));
#32293=CARTESIAN_POINT('Ctrl Pts',(-33.7516274460001,36.0199153180548,173.640581477849));
#32294=CARTESIAN_POINT('Ctrl Pts',(-33.977283069749,35.5920962921692,173.203436824419));
#32295=CARTESIAN_POINT('Ctrl Pts',(-33.3741378393645,35.4043412967755,173.312985330162));
#32296=CARTESIAN_POINT('Ctrl Pts',(-33.7101944105682,36.1001541204655,173.485485069079));
#32297=CARTESIAN_POINT('Ctrl Pts',(-33.9682581825426,35.6003903982821,173.143998023837));
#32298=CARTESIAN_POINT('Ctrl Pts',(-33.3358320373305,35.4434146616551,173.235485069079));
#32299=CARTESIAN_POINT('Origin',(-33.7154041461839,35.0749167312736,173.985485069079));
#32300=CARTESIAN_POINT('Origin',(-44.1060283439209,41.4682670878081,173.985485069079));
#32301=CARTESIAN_POINT('Origin',(-37.1738630900728,31.4290895869696,173.985485069079));
#32302=CARTESIAN_POINT('Origin',(-31.7758655563387,23.6116972707429,173.985485069079));
#32303=CARTESIAN_POINT('Origin',(-41.1020539958444,25.42062214227,173.985485069079));
#32304=CARTESIAN_POINT('Origin',(-36.6843857876575,24.5637629925993,173.985485069079));
#32305=CARTESIAN_POINT('Origin',(-36.6843857876575,24.5637629925993,177.985485069079));
#32306=CARTESIAN_POINT('Origin',(-41.1020539958444,25.42062214227,177.985485069079));
#32307=CARTESIAN_POINT('Origin',(-31.7758655563387,23.6116972707429,177.985485069079));
#32308=CARTESIAN_POINT('Origin',(-37.1738630900728,31.4290895869696,177.985485069079));
#32309=CARTESIAN_POINT('Origin',(-44.1060283439209,41.4682670878081,177.985485069079));
#32310=CARTESIAN_POINT('Origin',(-33.7154041461839,35.0749167312736,177.985485069079));
#32311=CARTESIAN_POINT('Ctrl Pts',(-33.7101944105682,36.1001541204655,178.485485069079));
#32312=CARTESIAN_POINT('Ctrl Pts',(-33.9682581825426,35.6003903982821,178.826972114322));
#32313=CARTESIAN_POINT('Ctrl Pts',(-33.3358320373305,35.4434146616551,178.735485069079));
#32314=CARTESIAN_POINT('Ctrl Pts',(-33.7516006038855,36.0199673002257,178.330489138169));
#32315=CARTESIAN_POINT('Ctrl Pts',(-33.977279425657,35.5920996411968,178.767557313941));
#32316=CARTESIAN_POINT('Ctrl Pts',(-33.3741156308558,35.4043639502364,178.658029740133));
#32317=CARTESIAN_POINT('Ctrl Pts',(-33.8133066023579,35.9029147229749,178.202225990637));
#32318=CARTESIAN_POINT('Ctrl Pts',(-33.9938040222832,35.5715957197603,178.697100878701));
#32319=CARTESIAN_POINT('Ctrl Pts',(-33.4304994268961,35.3474306123349,178.593855528671));
#32320=CARTESIAN_POINT('Ctrl Pts',(-33.9618960455694,35.6364708201442,178.030587223347));
#32321=CARTESIAN_POINT('Ctrl Pts',(-34.0509357072909,35.484060062052,178.570779964287));
#32322=CARTESIAN_POINT('Ctrl Pts',(-33.5621199729607,35.2186253327459,178.508036147401));
#32323=CARTESIAN_POINT('Ctrl Pts',(-34.0500285364698,35.4851935918964,177.985485070059));
#32324=CARTESIAN_POINT('Ctrl Pts',(-34.0906717048824,35.4191393620078,178.514868872724));
#32325=CARTESIAN_POINT('Ctrl Pts',(-33.6384206503181,35.1458285437047,178.485485069079));
#32326=CARTESIAN_POINT('Ctrl Pts',(-34.1412494001895,35.3369392868692,177.985485069079));
#32327=CARTESIAN_POINT('Ctrl Pts',(-34.1412494001895,35.3369392868692,178.485485069079));
#32328=CARTESIAN_POINT('Ctrl Pts',(-33.7154041461839,35.0749167312735,178.485485069079));
#32329=CARTESIAN_POINT('Origin',(-33.26592800316,35.8707475833996,178.485485069079));
#32330=CARTESIAN_POINT('Ctrl Pts',(-33.3358320373305,35.4434146616551,178.735485069079));
#32331=CARTESIAN_POINT('Ctrl Pts',(-33.9682581825426,35.6003903982821,178.826972114322));
#32332=CARTESIAN_POINT('Ctrl Pts',(-33.7101944105682,36.1001541204655,178.485485069079));
#32333=CARTESIAN_POINT('Ctrl Pts',(-33.1880191877447,35.7136289261714,179.238701731644));
#32334=CARTESIAN_POINT('Ctrl Pts',(-33.8204276914644,35.8561010262749,179.325424768988));
#32335=CARTESIAN_POINT('Ctrl Pts',(-33.5757636385812,36.3604914102378,178.988700441575));
#32336=CARTESIAN_POINT('Ctrl Pts',(-33.0506074115094,35.9881357503643,179.741630342279));
#32337=CARTESIAN_POINT('Ctrl Pts',(-33.682291766366,36.1173819195807,179.826657124525));
#32338=CARTESIAN_POINT('Ctrl Pts',(-33.4516565150989,36.6248074047886,179.491629509058));
#32339=CARTESIAN_POINT('Ctrl Pts',(-32.9232632882234,36.2665888893427,180.244482446977));
#32340=CARTESIAN_POINT('Ctrl Pts',(-33.5545758603726,36.3825939324359,180.329066002825));
#32341=CARTESIAN_POINT('Ctrl Pts',(-33.3378144598069,36.8927267103254,179.994482446977));
#47694=UNCERTAINTY_MEASURE_WITH_UNIT(LENGTH_MEASURE(0.01),#47718,
'DISTANCE_ACCURACY_VALUE',
'Maximum model space distance between geometric entities at asserted c
onnectivities');
#47703=UNCERTAINTY_MEASURE_WITH_UNIT(LENGTH_MEASURE(0.01),#47718,
'DISTANCE_ACCURACY_VALUE',
'Maximum model space distance between geometric entities at asserted c
onnectivities');
#47708=(
GEOMETRIC_REPRESENTATION_CONTEXT(3)
GLOBAL_UNCERTAINTY_ASSIGNED_CONTEXT((#47694))
GLOBAL_UNIT_ASSIGNED_CONTEXT((#47718,#47720,#47721))
REPRESENTATION_CONTEXT('','3D')
);
#47717=(
GEOMETRIC_REPRESENTATION_CONTEXT(3)
GLOBAL_UNCERTAINTY_ASSIGNED_CONTEXT((#47703))
GLOBAL_UNIT_ASSIGNED_CONTEXT((#47718,#47720,#47721))
REPRESENTATION_CONTEXT('','3D')
);
#47718=(
LENGTH_UNIT()
NAMED_UNIT(*)
SI_UNIT(.MILLI.,.METRE.)
);
#47720=(
NAMED_UNIT(*)
PLANE_ANGLE_UNIT()
SI_UNIT($,.RADIAN.)
);
#47721=(
NAMED_UNIT(*)
SI_UNIT($,.STERADIAN.)
SOLID_ANGLE_UNIT()
);
#47726=SHAPE_DEFINITION_REPRESENTATION(#47739,#47764);
#47739=PRODUCT_DEFINITION_SHAPE('',$,#47778);
#47764=SHAPE_REPRESENTATION('',(#9122),#47708);
#47773=PRODUCT_DEFINITION_CONTEXT('part definition',#47814,'design');
#47778=PRODUCT_DEFINITION('Upper Handle Fixed Jaw',
'Upper Handle Fixed Jaw',#47791,#47773);
#47791=PRODUCT_DEFINITION_FORMATION('',$,#47820);
#47814=APPLICATION_CONTEXT(
'Core Data for Automotive Mechanical Design Process');
#47815=PRODUCT_CONTEXT('part definition',#47814,'mechanical');
#47820=PRODUCT('Upper Handle Fixed Jaw','Upper Handle Fixed Jaw',$,(#47815));
#47830=PRESENTATION_STYLE_ASSIGNMENT((#47832));
#47832=SURFACE_STYLE_USAGE(.BOTH.,#47834);
#47834=SURFACE_SIDE_STYLE('',(#47836));
#47836=SURFACE_STYLE_FILL_AREA(#47838);
#47838=FILL_AREA_STYLE('Opaque(202,209,238)',(#47840));
#47840=FILL_AREA_STYLE_COLOUR('Opaque(202,209,238)',#47842);
#47842=COLOUR_RGB('Opaque(202,209,238)', 0.66274510, 0.83137255, 0.94901961);
ENDSEC;
END-ISO-10303-21;
